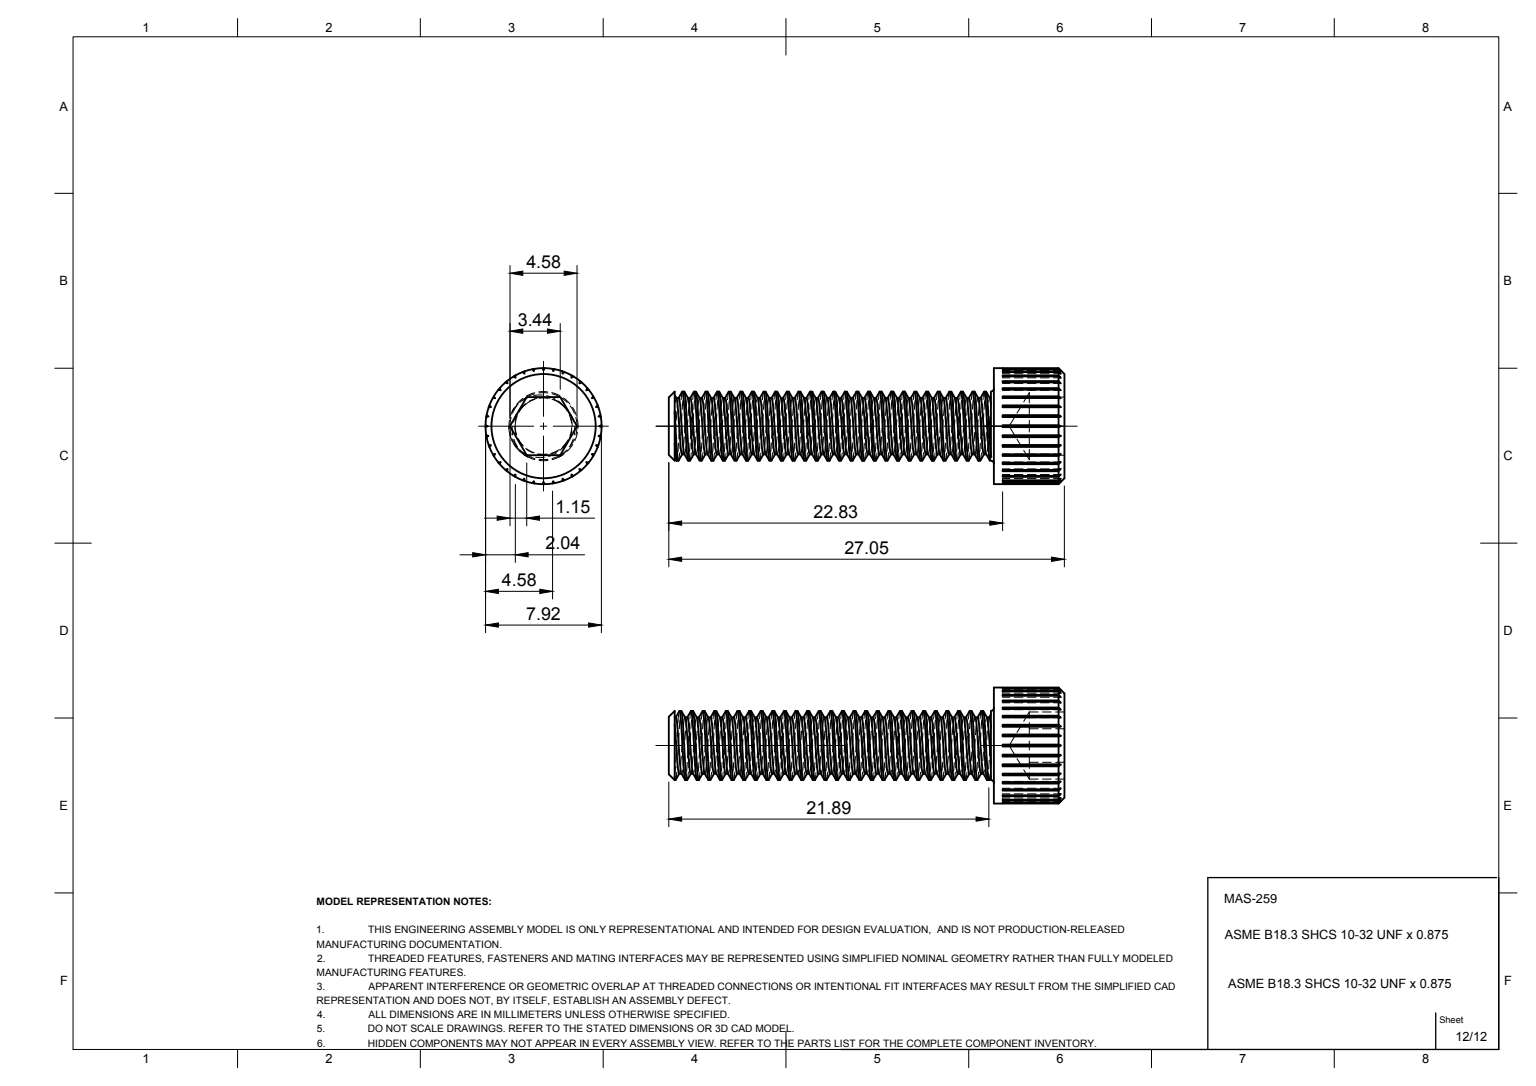
ISO-10303-21;
HEADER;
/* Generated by software containing ST-Developer
 * from STEP Tools, Inc. (www.steptools.com) 
 */

FILE_DESCRIPTION(
/* description */ (''),
/* implementation_level */ '2;1');

FILE_NAME(
/* name */ 'ASME B18.3 SHCS 10-32 UNF x 0.875.step',
/* time_stamp */ '2026-10-15T13:30:17-07:00',
/* author */ (''),
/* organization */ (''),
/* preprocessor_version */ 'ST-DEVELOPER v20.2',
/* originating_system */ 'Autodesk Translation Framework v15.15.0.0',
/* authorisation */ '');

FILE_SCHEMA (('AUTOMOTIVE_DESIGN { 1 0 10303 214 3 1 1 }'));
ENDSEC;

DATA;
#10=MECHANICAL_DESIGN_GEOMETRIC_PRESENTATION_REPRESENTATION('',(#1041),#71795);
#859=(
BOUNDED_CURVE()
B_SPLINE_CURVE(2,(#58913,#58914,#58915),.UNSPECIFIED.,.F.,.F.)
B_SPLINE_CURVE_WITH_KNOTS((3,3),(0.,0.0213887827154485),.UNSPECIFIED.)
CURVE()
GEOMETRIC_REPRESENTATION_ITEM()
RATIONAL_B_SPLINE_CURVE((1.,1.0006145366538,1.00078646015806))
REPRESENTATION_ITEM('')
);
#860=(
BOUNDED_CURVE()
B_SPLINE_CURVE(2,(#58918,#58919,#58920),.UNSPECIFIED.,.F.,.F.)
B_SPLINE_CURVE_WITH_KNOTS((3,3),(0.0380048027322743,0.0593935854477577),
 .UNSPECIFIED.)
CURVE()
GEOMETRIC_REPRESENTATION_ITEM()
RATIONAL_B_SPLINE_CURVE((1.00078646015726,1.00061453665318,1.))
REPRESENTATION_ITEM('')
);
#861=(
BOUNDED_CURVE()
B_SPLINE_CURVE(2,(#58929,#58930,#58931),.UNSPECIFIED.,.F.,.F.)
B_SPLINE_CURVE_WITH_KNOTS((3,3),(0.0380048027323083,0.0593935854477567),
 .UNSPECIFIED.)
CURVE()
GEOMETRIC_REPRESENTATION_ITEM()
RATIONAL_B_SPLINE_CURVE((1.00078646016055,1.00061453665575,1.))
REPRESENTATION_ITEM('')
);
#862=(
BOUNDED_CURVE()
B_SPLINE_CURVE(2,(#58935,#58936,#58937),.UNSPECIFIED.,.F.,.F.)
B_SPLINE_CURVE_WITH_KNOTS((3,3),(0.,0.0213887827154447),.UNSPECIFIED.)
CURVE()
GEOMETRIC_REPRESENTATION_ITEM()
RATIONAL_B_SPLINE_CURVE((1.,1.00061453665542,1.00078646016013))
REPRESENTATION_ITEM('')
);
#863=(
BOUNDED_CURVE()
B_SPLINE_CURVE(2,(#58939,#58940,#58941),.UNSPECIFIED.,.F.,.F.)
B_SPLINE_CURVE_WITH_KNOTS((3,3),(0.0380048027323192,0.0593935854477567),
 .UNSPECIFIED.)
CURVE()
GEOMETRIC_REPRESENTATION_ITEM()
RATIONAL_B_SPLINE_CURVE((1.0007864601593,1.00061453665477,1.))
REPRESENTATION_ITEM('')
);
#864=(
BOUNDED_CURVE()
B_SPLINE_CURVE(2,(#58945,#58946,#58947),.UNSPECIFIED.,.F.,.F.)
B_SPLINE_CURVE_WITH_KNOTS((3,3),(0.,0.0213887827154334),.UNSPECIFIED.)
CURVE()
GEOMETRIC_REPRESENTATION_ITEM()
RATIONAL_B_SPLINE_CURVE((1.,1.00061453665449,1.00078646015894))
REPRESENTATION_ITEM('')
);
#865=(
BOUNDED_CURVE()
B_SPLINE_CURVE(2,(#58949,#58950,#58951),.UNSPECIFIED.,.F.,.F.)
B_SPLINE_CURVE_WITH_KNOTS((3,3),(0.0380048027322763,0.0593935854477568),
 .UNSPECIFIED.)
CURVE()
GEOMETRIC_REPRESENTATION_ITEM()
RATIONAL_B_SPLINE_CURVE((1.00078646015818,1.00061453665389,1.))
REPRESENTATION_ITEM('')
);
#866=(
BOUNDED_CURVE()
B_SPLINE_CURVE(2,(#58955,#58956,#58957),.UNSPECIFIED.,.F.,.F.)
B_SPLINE_CURVE_WITH_KNOTS((3,3),(0.,0.0213887827154747),.UNSPECIFIED.)
CURVE()
GEOMETRIC_REPRESENTATION_ITEM()
RATIONAL_B_SPLINE_CURVE((1.,1.00061453665232,1.00078646015616))
REPRESENTATION_ITEM('')
);
#867=(
BOUNDED_CURVE()
B_SPLINE_CURVE(2,(#58959,#58960,#58961),.UNSPECIFIED.,.F.,.F.)
B_SPLINE_CURVE_WITH_KNOTS((3,3),(0.0380048027322871,0.0593935854477566),
 .UNSPECIFIED.)
CURVE()
GEOMETRIC_REPRESENTATION_ITEM()
RATIONAL_B_SPLINE_CURVE((1.00078646015913,1.00061453665464,1.))
REPRESENTATION_ITEM('')
);
#868=(
BOUNDED_CURVE()
B_SPLINE_CURVE(2,(#58965,#58966,#58967),.UNSPECIFIED.,.F.,.F.)
B_SPLINE_CURVE_WITH_KNOTS((3,3),(0.,0.0213887827154556),.UNSPECIFIED.)
CURVE()
GEOMETRIC_REPRESENTATION_ITEM()
RATIONAL_B_SPLINE_CURVE((1.,1.00061453665459,1.00078646015907))
REPRESENTATION_ITEM('')
);
#869=(
BOUNDED_CURVE()
B_SPLINE_CURVE(2,(#58969,#58970,#58971),.UNSPECIFIED.,.F.,.F.)
B_SPLINE_CURVE_WITH_KNOTS((3,3),(0.0380048027322698,0.0593935854477568),
 .UNSPECIFIED.)
CURVE()
GEOMETRIC_REPRESENTATION_ITEM()
RATIONAL_B_SPLINE_CURVE((1.000786460157,1.00061453665298,1.))
REPRESENTATION_ITEM('')
);
#870=(
BOUNDED_CURVE()
B_SPLINE_CURVE(2,(#58975,#58976,#58977),.UNSPECIFIED.,.F.,.F.)
B_SPLINE_CURVE_WITH_KNOTS((3,3),(0.,0.0213887827154226),.UNSPECIFIED.)
CURVE()
GEOMETRIC_REPRESENTATION_ITEM()
RATIONAL_B_SPLINE_CURVE((1.,1.00061453665557,1.00078646016033))
REPRESENTATION_ITEM('')
);
#871=(
BOUNDED_CURVE()
B_SPLINE_CURVE(2,(#58979,#58980,#58981),.UNSPECIFIED.,.F.,.F.)
B_SPLINE_CURVE_WITH_KNOTS((3,3),(0.0380048027322981,0.0593935854477561),
 .UNSPECIFIED.)
CURVE()
GEOMETRIC_REPRESENTATION_ITEM()
RATIONAL_B_SPLINE_CURVE((1.00078646015658,1.00061453665264,1.))
REPRESENTATION_ITEM('')
);
#872=(
BOUNDED_CURVE()
B_SPLINE_CURVE(2,(#58985,#58986,#58987),.UNSPECIFIED.,.F.,.F.)
B_SPLINE_CURVE_WITH_KNOTS((3,3),(0.,0.0213887827154885),.UNSPECIFIED.)
CURVE()
GEOMETRIC_REPRESENTATION_ITEM()
RATIONAL_B_SPLINE_CURVE((1.,1.00061453665414,1.00078646015849))
REPRESENTATION_ITEM('')
);
#873=(
BOUNDED_CURVE()
B_SPLINE_CURVE(2,(#58989,#58990,#58991),.UNSPECIFIED.,.F.,.F.)
B_SPLINE_CURVE_WITH_KNOTS((3,3),(0.0380048027323009,0.0593935854477566),
 .UNSPECIFIED.)
CURVE()
GEOMETRIC_REPRESENTATION_ITEM()
RATIONAL_B_SPLINE_CURVE((1.00078646015915,1.00061453665465,1.))
REPRESENTATION_ITEM('')
);
#874=(
BOUNDED_CURVE()
B_SPLINE_CURVE(2,(#58995,#58996,#58997),.UNSPECIFIED.,.F.,.F.)
B_SPLINE_CURVE_WITH_KNOTS((3,3),(0.,0.0213887827154357),.UNSPECIFIED.)
CURVE()
GEOMETRIC_REPRESENTATION_ITEM()
RATIONAL_B_SPLINE_CURVE((1.,1.00061453665688,1.000786460162))
REPRESENTATION_ITEM('')
);
#875=(
BOUNDED_CURVE()
B_SPLINE_CURVE(2,(#58999,#59000,#59001),.UNSPECIFIED.,.F.,.F.)
B_SPLINE_CURVE_WITH_KNOTS((3,3),(0.0380048027323154,0.059393585447756),
 .UNSPECIFIED.)
CURVE()
GEOMETRIC_REPRESENTATION_ITEM()
RATIONAL_B_SPLINE_CURVE((1.00078646016079,1.00061453665593,1.))
REPRESENTATION_ITEM('')
);
#876=(
BOUNDED_CURVE()
B_SPLINE_CURVE(2,(#59005,#59006,#59007),.UNSPECIFIED.,.F.,.F.)
B_SPLINE_CURVE_WITH_KNOTS((3,3),(0.,0.0213887827154912),.UNSPECIFIED.)
CURVE()
GEOMETRIC_REPRESENTATION_ITEM()
RATIONAL_B_SPLINE_CURVE((1.,1.00061453665086,1.0007864601543))
REPRESENTATION_ITEM('')
);
#877=(
BOUNDED_CURVE()
B_SPLINE_CURVE(2,(#59009,#59010,#59011),.UNSPECIFIED.,.F.,.F.)
B_SPLINE_CURVE_WITH_KNOTS((3,3),(0.0380048027322925,0.0593935854477561),
 .UNSPECIFIED.)
CURVE()
GEOMETRIC_REPRESENTATION_ITEM()
RATIONAL_B_SPLINE_CURVE((1.00078646015764,1.00061453665347,1.))
REPRESENTATION_ITEM('')
);
#878=(
BOUNDED_CURVE()
B_SPLINE_CURVE(2,(#59015,#59016,#59017),.UNSPECIFIED.,.F.,.F.)
B_SPLINE_CURVE_WITH_KNOTS((3,3),(0.,0.0213887827155107),.UNSPECIFIED.)
CURVE()
GEOMETRIC_REPRESENTATION_ITEM()
RATIONAL_B_SPLINE_CURVE((1.,1.00061453665119,1.00078646015471))
REPRESENTATION_ITEM('')
);
#879=(
BOUNDED_CURVE()
B_SPLINE_CURVE(2,(#59019,#59020,#59021),.UNSPECIFIED.,.F.,.F.)
B_SPLINE_CURVE_WITH_KNOTS((3,3),(0.038004802732295,0.0593935854477563),
 .UNSPECIFIED.)
CURVE()
GEOMETRIC_REPRESENTATION_ITEM()
RATIONAL_B_SPLINE_CURVE((1.00078646016111,1.00061453665618,1.))
REPRESENTATION_ITEM('')
);
#880=(
BOUNDED_CURVE()
B_SPLINE_CURVE(2,(#59025,#59026,#59027),.UNSPECIFIED.,.F.,.F.)
B_SPLINE_CURVE_WITH_KNOTS((3,3),(0.,0.0213887827154503),.UNSPECIFIED.)
CURVE()
GEOMETRIC_REPRESENTATION_ITEM()
RATIONAL_B_SPLINE_CURVE((1.,1.00061453665305,1.00078646015709))
REPRESENTATION_ITEM('')
);
#881=(
BOUNDED_CURVE()
B_SPLINE_CURVE(2,(#59029,#59030,#59031),.UNSPECIFIED.,.F.,.F.)
B_SPLINE_CURVE_WITH_KNOTS((3,3),(0.0380048027323246,0.059393585447756),
 .UNSPECIFIED.)
CURVE()
GEOMETRIC_REPRESENTATION_ITEM()
RATIONAL_B_SPLINE_CURVE((1.00078646015741,1.00061453665329,1.))
REPRESENTATION_ITEM('')
);
#882=(
BOUNDED_CURVE()
B_SPLINE_CURVE(2,(#59035,#59036,#59037),.UNSPECIFIED.,.F.,.F.)
B_SPLINE_CURVE_WITH_KNOTS((3,3),(0.,0.0213887827154455),.UNSPECIFIED.)
CURVE()
GEOMETRIC_REPRESENTATION_ITEM()
RATIONAL_B_SPLINE_CURVE((1.,1.00061453665435,1.00078646015877))
REPRESENTATION_ITEM('')
);
#883=(
BOUNDED_CURVE()
B_SPLINE_CURVE(2,(#59039,#59040,#59041),.UNSPECIFIED.,.F.,.F.)
B_SPLINE_CURVE_WITH_KNOTS((3,3),(0.0380048027322671,0.0593935854477559),
 .UNSPECIFIED.)
CURVE()
GEOMETRIC_REPRESENTATION_ITEM()
RATIONAL_B_SPLINE_CURVE((1.00078646015673,1.00061453665277,1.))
REPRESENTATION_ITEM('')
);
#884=(
BOUNDED_CURVE()
B_SPLINE_CURVE(2,(#59045,#59046,#59047),.UNSPECIFIED.,.F.,.F.)
B_SPLINE_CURVE_WITH_KNOTS((3,3),(0.,0.0213887827154328),.UNSPECIFIED.)
CURVE()
GEOMETRIC_REPRESENTATION_ITEM()
RATIONAL_B_SPLINE_CURVE((1.,1.0006145366569,1.00078646016203))
REPRESENTATION_ITEM('')
);
#885=(
BOUNDED_CURVE()
B_SPLINE_CURVE(2,(#59049,#59050,#59051),.UNSPECIFIED.,.F.,.F.)
B_SPLINE_CURVE_WITH_KNOTS((3,3),(0.0380048027322495,0.0593935854477564),
 .UNSPECIFIED.)
CURVE()
GEOMETRIC_REPRESENTATION_ITEM()
RATIONAL_B_SPLINE_CURVE((1.0007864601568,1.00061453665282,1.))
REPRESENTATION_ITEM('')
);
#886=(
BOUNDED_CURVE()
B_SPLINE_CURVE(2,(#59055,#59056,#59057),.UNSPECIFIED.,.F.,.F.)
B_SPLINE_CURVE_WITH_KNOTS((3,3),(0.,0.0213887827154736),.UNSPECIFIED.)
CURVE()
GEOMETRIC_REPRESENTATION_ITEM()
RATIONAL_B_SPLINE_CURVE((1.,1.0006145366516,1.00078646015525))
REPRESENTATION_ITEM('')
);
#887=(
BOUNDED_CURVE()
B_SPLINE_CURVE(2,(#59059,#59060,#59061),.UNSPECIFIED.,.F.,.F.)
B_SPLINE_CURVE_WITH_KNOTS((3,3),(0.0380048027322323,0.0593935854477557),
 .UNSPECIFIED.)
CURVE()
GEOMETRIC_REPRESENTATION_ITEM()
RATIONAL_B_SPLINE_CURVE((1.00078646015266,1.00061453664958,1.))
REPRESENTATION_ITEM('')
);
#888=(
BOUNDED_CURVE()
B_SPLINE_CURVE(2,(#59065,#59066,#59067),.UNSPECIFIED.,.F.,.F.)
B_SPLINE_CURVE_WITH_KNOTS((3,3),(0.,0.0213887827154861),.UNSPECIFIED.)
CURVE()
GEOMETRIC_REPRESENTATION_ITEM()
RATIONAL_B_SPLINE_CURVE((1.,1.00061453665221,1.00078646015603))
REPRESENTATION_ITEM('')
);
#889=(
BOUNDED_CURVE()
B_SPLINE_CURVE(2,(#59069,#59070,#59071),.UNSPECIFIED.,.F.,.F.)
B_SPLINE_CURVE_WITH_KNOTS((3,3),(0.038004802732259,0.0593935854477563),
 .UNSPECIFIED.)
CURVE()
GEOMETRIC_REPRESENTATION_ITEM()
RATIONAL_B_SPLINE_CURVE((1.00078646015598,1.00061453665218,1.))
REPRESENTATION_ITEM('')
);
#890=(
BOUNDED_CURVE()
B_SPLINE_CURVE(2,(#59075,#59076,#59077),.UNSPECIFIED.,.F.,.F.)
B_SPLINE_CURVE_WITH_KNOTS((3,3),(0.,0.0213887827154904),.UNSPECIFIED.)
CURVE()
GEOMETRIC_REPRESENTATION_ITEM()
RATIONAL_B_SPLINE_CURVE((1.,1.00061453665374,1.00078646015798))
REPRESENTATION_ITEM('')
);
#891=(
BOUNDED_CURVE()
B_SPLINE_CURVE(2,(#59079,#59080,#59081),.UNSPECIFIED.,.F.,.F.)
B_SPLINE_CURVE_WITH_KNOTS((3,3),(0.0380048027322369,0.0593935854477557),
 .UNSPECIFIED.)
CURVE()
GEOMETRIC_REPRESENTATION_ITEM()
RATIONAL_B_SPLINE_CURVE((1.00078646015409,1.0006145366507,1.))
REPRESENTATION_ITEM('')
);
#892=(
BOUNDED_CURVE()
B_SPLINE_CURVE(2,(#59085,#59086,#59087),.UNSPECIFIED.,.F.,.F.)
B_SPLINE_CURVE_WITH_KNOTS((3,3),(0.,0.0213887827154539),.UNSPECIFIED.)
CURVE()
GEOMETRIC_REPRESENTATION_ITEM()
RATIONAL_B_SPLINE_CURVE((1.,1.00061453665704,1.0007864601622))
REPRESENTATION_ITEM('')
);
#893=(
BOUNDED_CURVE()
B_SPLINE_CURVE(2,(#59089,#59090,#59091),.UNSPECIFIED.,.F.,.F.)
B_SPLINE_CURVE_WITH_KNOTS((3,3),(0.0380048027323148,0.0593935854477558),
 .UNSPECIFIED.)
CURVE()
GEOMETRIC_REPRESENTATION_ITEM()
RATIONAL_B_SPLINE_CURVE((1.00078646015925,1.00061453665473,1.))
REPRESENTATION_ITEM('')
);
#894=(
BOUNDED_CURVE()
B_SPLINE_CURVE(2,(#59095,#59096,#59097),.UNSPECIFIED.,.F.,.F.)
B_SPLINE_CURVE_WITH_KNOTS((3,3),(0.,0.0213887827154462),.UNSPECIFIED.)
CURVE()
GEOMETRIC_REPRESENTATION_ITEM()
RATIONAL_B_SPLINE_CURVE((1.,1.00061453665421,1.00078646015858))
REPRESENTATION_ITEM('')
);
#895=(
BOUNDED_CURVE()
B_SPLINE_CURVE(2,(#59099,#59100,#59101),.UNSPECIFIED.,.F.,.F.)
B_SPLINE_CURVE_WITH_KNOTS((3,3),(0.038004802732261,0.0593935854477558),
 .UNSPECIFIED.)
CURVE()
GEOMETRIC_REPRESENTATION_ITEM()
RATIONAL_B_SPLINE_CURVE((1.0007864601574,1.00061453665329,1.))
REPRESENTATION_ITEM('')
);
#896=(
BOUNDED_CURVE()
B_SPLINE_CURVE(2,(#59105,#59106,#59107),.UNSPECIFIED.,.F.,.F.)
B_SPLINE_CURVE_WITH_KNOTS((3,3),(0.,0.021388782715505),.UNSPECIFIED.)
CURVE()
GEOMETRIC_REPRESENTATION_ITEM()
RATIONAL_B_SPLINE_CURVE((1.,1.00061453665229,1.00078646015612))
REPRESENTATION_ITEM('')
);
#897=(
BOUNDED_CURVE()
B_SPLINE_CURVE(2,(#59109,#59110,#59111),.UNSPECIFIED.,.F.,.F.)
B_SPLINE_CURVE_WITH_KNOTS((3,3),(0.0380048027323058,0.0593935854477558),
 .UNSPECIFIED.)
CURVE()
GEOMETRIC_REPRESENTATION_ITEM()
RATIONAL_B_SPLINE_CURVE((1.00078646016102,1.00061453665611,1.))
REPRESENTATION_ITEM('')
);
#898=(
BOUNDED_CURVE()
B_SPLINE_CURVE(2,(#59116,#59117,#59118),.UNSPECIFIED.,.F.,.F.)
B_SPLINE_CURVE_WITH_KNOTS((3,3),(0.,0.0213887827154293),.UNSPECIFIED.)
CURVE()
GEOMETRIC_REPRESENTATION_ITEM()
RATIONAL_B_SPLINE_CURVE((1.,1.00061453665639,1.00078646016138))
REPRESENTATION_ITEM('')
);
#899=(
BOUNDED_CURVE()
B_SPLINE_CURVE(2,(#59120,#59121,#59122),.UNSPECIFIED.,.F.,.F.)
B_SPLINE_CURVE_WITH_KNOTS((3,3),(0.0380048027323149,0.0593935854477581),
 .UNSPECIFIED.)
CURVE()
GEOMETRIC_REPRESENTATION_ITEM()
RATIONAL_B_SPLINE_CURVE((1.00078646016138,1.0006145366564,1.))
REPRESENTATION_ITEM('')
);
#900=(
BOUNDED_CURVE()
B_SPLINE_CURVE(2,(#59126,#59127,#59128),.UNSPECIFIED.,.F.,.F.)
B_SPLINE_CURVE_WITH_KNOTS((3,3),(0.,0.0213887827154979),.UNSPECIFIED.)
CURVE()
GEOMETRIC_REPRESENTATION_ITEM()
RATIONAL_B_SPLINE_CURVE((1.,1.00061453665225,1.00078646015608))
REPRESENTATION_ITEM('')
);
#901=(
BOUNDED_CURVE()
B_SPLINE_CURVE(2,(#59130,#59131,#59132),.UNSPECIFIED.,.F.,.F.)
B_SPLINE_CURVE_WITH_KNOTS((3,3),(0.0380048027322422,0.059393585447758),
 .UNSPECIFIED.)
CURVE()
GEOMETRIC_REPRESENTATION_ITEM()
RATIONAL_B_SPLINE_CURVE((1.00078646015494,1.00061453665137,1.))
REPRESENTATION_ITEM('')
);
#902=(
BOUNDED_CURVE()
B_SPLINE_CURVE(2,(#59136,#59137,#59138),.UNSPECIFIED.,.F.,.F.)
B_SPLINE_CURVE_WITH_KNOTS((3,3),(0.,0.0213887827154959),.UNSPECIFIED.)
CURVE()
GEOMETRIC_REPRESENTATION_ITEM()
RATIONAL_B_SPLINE_CURVE((1.,1.00061453665238,1.00078646015624))
REPRESENTATION_ITEM('')
);
#903=(
BOUNDED_CURVE()
B_SPLINE_CURVE(2,(#59140,#59141,#59142),.UNSPECIFIED.,.F.,.F.)
B_SPLINE_CURVE_WITH_KNOTS((3,3),(0.0380048027323219,0.0593935854477577),
 .UNSPECIFIED.)
CURVE()
GEOMETRIC_REPRESENTATION_ITEM()
RATIONAL_B_SPLINE_CURVE((1.00078646016013,1.00061453665542,1.))
REPRESENTATION_ITEM('')
);
#904=(
BOUNDED_CURVE()
B_SPLINE_CURVE(2,(#59146,#59147,#59148),.UNSPECIFIED.,.F.,.F.)
B_SPLINE_CURVE_WITH_KNOTS((3,3),(0.,0.021388782715533),.UNSPECIFIED.)
CURVE()
GEOMETRIC_REPRESENTATION_ITEM()
RATIONAL_B_SPLINE_CURVE((1.,1.00061453664963,1.00078646015272))
REPRESENTATION_ITEM('')
);
#905=(
BOUNDED_CURVE()
B_SPLINE_CURVE(2,(#59150,#59151,#59152),.UNSPECIFIED.,.F.,.F.)
B_SPLINE_CURVE_WITH_KNOTS((3,3),(0.0380048027324089,0.0593935854477567),
 .UNSPECIFIED.)
CURVE()
GEOMETRIC_REPRESENTATION_ITEM()
RATIONAL_B_SPLINE_CURVE((1.00078646016585,1.00061453665989,1.))
REPRESENTATION_ITEM('')
);
#906=(
BOUNDED_CURVE()
B_SPLINE_CURVE(2,(#59156,#59157,#59158),.UNSPECIFIED.,.F.,.F.)
B_SPLINE_CURVE_WITH_KNOTS((3,3),(0.,0.0213887827154936),.UNSPECIFIED.)
CURVE()
GEOMETRIC_REPRESENTATION_ITEM()
RATIONAL_B_SPLINE_CURVE((1.,1.00061453665172,1.00078646015539))
REPRESENTATION_ITEM('')
);
#907=(
BOUNDED_CURVE()
B_SPLINE_CURVE(2,(#59160,#59161,#59162),.UNSPECIFIED.,.F.,.F.)
B_SPLINE_CURVE_WITH_KNOTS((3,3),(0.038004802732325,0.0593935854477579),
 .UNSPECIFIED.)
CURVE()
GEOMETRIC_REPRESENTATION_ITEM()
RATIONAL_B_SPLINE_CURVE((1.00078646016394,1.0006145366584,1.))
REPRESENTATION_ITEM('')
);
#908=(
BOUNDED_CURVE()
B_SPLINE_CURVE(2,(#59166,#59167,#59168),.UNSPECIFIED.,.F.,.F.)
B_SPLINE_CURVE_WITH_KNOTS((3,3),(0.,0.0213887827154531),.UNSPECIFIED.)
CURVE()
GEOMETRIC_REPRESENTATION_ITEM()
RATIONAL_B_SPLINE_CURVE((1.,1.00061453665483,1.00078646015938))
REPRESENTATION_ITEM('')
);
#909=(
BOUNDED_CURVE()
B_SPLINE_CURVE(2,(#59170,#59171,#59172),.UNSPECIFIED.,.F.,.F.)
B_SPLINE_CURVE_WITH_KNOTS((3,3),(0.03800480273219,0.0593935854477586),
 .UNSPECIFIED.)
CURVE()
GEOMETRIC_REPRESENTATION_ITEM()
RATIONAL_B_SPLINE_CURVE((1.00078646015297,1.00061453664982,1.))
REPRESENTATION_ITEM('')
);
#910=(
BOUNDED_CURVE()
B_SPLINE_CURVE(2,(#59176,#59177,#59178),.UNSPECIFIED.,.F.,.F.)
B_SPLINE_CURVE_WITH_KNOTS((3,3),(0.,0.0213887827154683),.UNSPECIFIED.)
CURVE()
GEOMETRIC_REPRESENTATION_ITEM()
RATIONAL_B_SPLINE_CURVE((1.,1.00061453665169,1.00078646015536))
REPRESENTATION_ITEM('')
);
#911=(
BOUNDED_CURVE()
B_SPLINE_CURVE(2,(#59180,#59181,#59182),.UNSPECIFIED.,.F.,.F.)
B_SPLINE_CURVE_WITH_KNOTS((3,3),(0.0380048027322755,0.0593935854477574),
 .UNSPECIFIED.)
CURVE()
GEOMETRIC_REPRESENTATION_ITEM()
RATIONAL_B_SPLINE_CURVE((1.00078646016181,1.00061453665673,1.))
REPRESENTATION_ITEM('')
);
#912=(
BOUNDED_CURVE()
B_SPLINE_CURVE(2,(#59186,#59187,#59188),.UNSPECIFIED.,.F.,.F.)
B_SPLINE_CURVE_WITH_KNOTS((3,3),(0.,0.0213887827154684),.UNSPECIFIED.)
CURVE()
GEOMETRIC_REPRESENTATION_ITEM()
RATIONAL_B_SPLINE_CURVE((1.,1.0006145366546,1.00078646015908))
REPRESENTATION_ITEM('')
);
#913=(
BOUNDED_CURVE()
B_SPLINE_CURVE(2,(#59190,#59191,#59192),.UNSPECIFIED.,.F.,.F.)
B_SPLINE_CURVE_WITH_KNOTS((3,3),(0.0380048027323105,0.0593935854477581),
 .UNSPECIFIED.)
CURVE()
GEOMETRIC_REPRESENTATION_ITEM()
RATIONAL_B_SPLINE_CURVE((1.00078646015979,1.00061453665516,1.))
REPRESENTATION_ITEM('')
);
#914=(
BOUNDED_CURVE()
B_SPLINE_CURVE(2,(#59196,#59197,#59198),.UNSPECIFIED.,.F.,.F.)
B_SPLINE_CURVE_WITH_KNOTS((3,3),(0.,0.0213887827154438),.UNSPECIFIED.)
CURVE()
GEOMETRIC_REPRESENTATION_ITEM()
RATIONAL_B_SPLINE_CURVE((1.,1.00061453665793,1.00078646016334))
REPRESENTATION_ITEM('')
);
#915=(
BOUNDED_CURVE()
B_SPLINE_CURVE(2,(#59200,#59201,#59202),.UNSPECIFIED.,.F.,.F.)
B_SPLINE_CURVE_WITH_KNOTS((3,3),(0.0380048027322779,0.0593935854477573),
 .UNSPECIFIED.)
CURVE()
GEOMETRIC_REPRESENTATION_ITEM()
RATIONAL_B_SPLINE_CURVE((1.00078646015484,1.00061453665129,1.))
REPRESENTATION_ITEM('')
);
#916=(
BOUNDED_CURVE()
B_SPLINE_CURVE(2,(#59206,#59207,#59208),.UNSPECIFIED.,.F.,.F.)
B_SPLINE_CURVE_WITH_KNOTS((3,3),(0.,0.0213887827154012),.UNSPECIFIED.)
CURVE()
GEOMETRIC_REPRESENTATION_ITEM()
RATIONAL_B_SPLINE_CURVE((1.,1.00061453665908,1.00078646016482))
REPRESENTATION_ITEM('')
);
#917=(
BOUNDED_CURVE()
B_SPLINE_CURVE(2,(#59210,#59211,#59212),.UNSPECIFIED.,.F.,.F.)
B_SPLINE_CURVE_WITH_KNOTS((3,3),(0.0380048027322933,0.0593935854477573),
 .UNSPECIFIED.)
CURVE()
GEOMETRIC_REPRESENTATION_ITEM()
RATIONAL_B_SPLINE_CURVE((1.00078646015827,1.00061453665397,1.))
REPRESENTATION_ITEM('')
);
#918=(
BOUNDED_CURVE()
B_SPLINE_CURVE(2,(#59216,#59217,#59218),.UNSPECIFIED.,.F.,.F.)
B_SPLINE_CURVE_WITH_KNOTS((3,3),(0.,0.0213887827154559),.UNSPECIFIED.)
CURVE()
GEOMETRIC_REPRESENTATION_ITEM()
RATIONAL_B_SPLINE_CURVE((1.,1.00061453665602,1.0007864601609))
REPRESENTATION_ITEM('')
);
#919=(
BOUNDED_CURVE()
B_SPLINE_CURVE(2,(#59220,#59221,#59222),.UNSPECIFIED.,.F.,.F.)
B_SPLINE_CURVE_WITH_KNOTS((3,3),(0.038004802732396,0.0593935854477571),
 .UNSPECIFIED.)
CURVE()
GEOMETRIC_REPRESENTATION_ITEM()
RATIONAL_B_SPLINE_CURVE((1.00078646016815,1.00061453666168,1.))
REPRESENTATION_ITEM('')
);
#920=(
BOUNDED_CURVE()
B_SPLINE_CURVE(2,(#59226,#59227,#59228),.UNSPECIFIED.,.F.,.F.)
B_SPLINE_CURVE_WITH_KNOTS((3,3),(0.,0.0213887827154657),.UNSPECIFIED.)
CURVE()
GEOMETRIC_REPRESENTATION_ITEM()
RATIONAL_B_SPLINE_CURVE((1.,1.00061453665296,1.00078646015698))
REPRESENTATION_ITEM('')
);
#921=(
BOUNDED_CURVE()
B_SPLINE_CURVE(2,(#59230,#59231,#59232),.UNSPECIFIED.,.F.,.F.)
B_SPLINE_CURVE_WITH_KNOTS((3,3),(0.0380048027322985,0.059393585447757),
 .UNSPECIFIED.)
CURVE()
GEOMETRIC_REPRESENTATION_ITEM()
RATIONAL_B_SPLINE_CURVE((1.00078646016081,1.00061453665595,1.))
REPRESENTATION_ITEM('')
);
#922=(
BOUNDED_CURVE()
B_SPLINE_CURVE(2,(#59236,#59237,#59238),.UNSPECIFIED.,.F.,.F.)
B_SPLINE_CURVE_WITH_KNOTS((3,3),(0.,0.0213887827154679),.UNSPECIFIED.)
CURVE()
GEOMETRIC_REPRESENTATION_ITEM()
RATIONAL_B_SPLINE_CURVE((1.,1.00061453665517,1.00078646015981))
REPRESENTATION_ITEM('')
);
#923=(
BOUNDED_CURVE()
B_SPLINE_CURVE(2,(#59240,#59241,#59242),.UNSPECIFIED.,.F.,.F.)
B_SPLINE_CURVE_WITH_KNOTS((3,3),(0.0380048027322456,0.0593935854477571),
 .UNSPECIFIED.)
CURVE()
GEOMETRIC_REPRESENTATION_ITEM()
RATIONAL_B_SPLINE_CURVE((1.00078646015223,1.00061453664925,1.))
REPRESENTATION_ITEM('')
);
#924=(
BOUNDED_CURVE()
B_SPLINE_CURVE(2,(#59246,#59247,#59248),.UNSPECIFIED.,.F.,.F.)
B_SPLINE_CURVE_WITH_KNOTS((3,3),(0.,0.0213887827154763),.UNSPECIFIED.)
CURVE()
GEOMETRIC_REPRESENTATION_ITEM()
RATIONAL_B_SPLINE_CURVE((1.,1.00061453665236,1.00078646015621))
REPRESENTATION_ITEM('')
);
#925=(
BOUNDED_CURVE()
B_SPLINE_CURVE(2,(#59250,#59251,#59252),.UNSPECIFIED.,.F.,.F.)
B_SPLINE_CURVE_WITH_KNOTS((3,3),(0.0380048027323043,0.0593935854477561),
 .UNSPECIFIED.)
CURVE()
GEOMETRIC_REPRESENTATION_ITEM()
RATIONAL_B_SPLINE_CURVE((1.00078646015985,1.0006145366552,1.))
REPRESENTATION_ITEM('')
);
#926=(
BOUNDED_CURVE()
B_SPLINE_CURVE(2,(#59256,#59257,#59258),.UNSPECIFIED.,.F.,.F.)
B_SPLINE_CURVE_WITH_KNOTS((3,3),(0.,0.0213887827154303),.UNSPECIFIED.)
CURVE()
GEOMETRIC_REPRESENTATION_ITEM()
RATIONAL_B_SPLINE_CURVE((1.,1.00061453665563,1.0007864601604))
REPRESENTATION_ITEM('')
);
#927=(
BOUNDED_CURVE()
B_SPLINE_CURVE(2,(#59260,#59261,#59262),.UNSPECIFIED.,.F.,.F.)
B_SPLINE_CURVE_WITH_KNOTS((3,3),(0.0380048027323154,0.0593935854477565),
 .UNSPECIFIED.)
CURVE()
GEOMETRIC_REPRESENTATION_ITEM()
RATIONAL_B_SPLINE_CURVE((1.00078646015761,1.00061453665345,1.))
REPRESENTATION_ITEM('')
);
#928=(
BOUNDED_CURVE()
B_SPLINE_CURVE(2,(#59266,#59267,#59268),.UNSPECIFIED.,.F.,.F.)
B_SPLINE_CURVE_WITH_KNOTS((3,3),(0.,0.0213887827154477),.UNSPECIFIED.)
CURVE()
GEOMETRIC_REPRESENTATION_ITEM()
RATIONAL_B_SPLINE_CURVE((1.,1.00061453665389,1.00078646015818))
REPRESENTATION_ITEM('')
);
#929=(
BOUNDED_CURVE()
B_SPLINE_CURVE(2,(#59270,#59271,#59272),.UNSPECIFIED.,.F.,.F.)
B_SPLINE_CURVE_WITH_KNOTS((3,3),(0.0380048027322823,0.0593935854477568),
 .UNSPECIFIED.)
CURVE()
GEOMETRIC_REPRESENTATION_ITEM()
RATIONAL_B_SPLINE_CURVE((1.00078646015752,1.00061453665338,1.))
REPRESENTATION_ITEM('')
);
#930=(
BOUNDED_CURVE()
B_SPLINE_CURVE(2,(#59275,#59276,#59277),.UNSPECIFIED.,.F.,.F.)
B_SPLINE_CURVE_WITH_KNOTS((3,3),(0.,0.0213887827154623),.UNSPECIFIED.)
CURVE()
GEOMETRIC_REPRESENTATION_ITEM()
RATIONAL_B_SPLINE_CURVE((1.,1.00061453665359,1.00078646015779))
REPRESENTATION_ITEM('')
);
#1004=TOROIDAL_SURFACE('',#14398,2.56347,0.2);
#1008=B_SPLINE_SURFACE_WITH_KNOTS('',3,3,((#57303,#57304,#57305,#57306,
#57307,#57308,#57309,#57310,#57311,#57312,#57313,#57314,#57315,#57316,#57317,
#57318,#57319,#57320,#57321,#57322,#57323,#57324,#57325,#57326,#57327,#57328,
#57329,#57330,#57331,#57332,#57333,#57334,#57335,#57336,#57337,#57338,#57339,
#57340,#57341,#57342,#57343,#57344,#57345,#57346,#57347,#57348,#57349,#57350,
#57351,#57352,#57353,#57354,#57355,#57356,#57357,#57358,#57359,#57360,#57361,
#57362,#57363,#57364,#57365,#57366,#57367,#57368,#57369,#57370,#57371,#57372,
#57373,#57374,#57375,#57376,#57377,#57378,#57379,#57380,#57381,#57382,#57383,
#57384,#57385,#57386,#57387,#57388,#57389,#57390,#57391,#57392,#57393,#57394,
#57395,#57396,#57397,#57398,#57399,#57400,#57401,#57402,#57403,#57404,#57405,
#57406,#57407,#57408,#57409,#57410,#57411,#57412,#57413,#57414,#57415,#57416,
#57417,#57418,#57419,#57420,#57421,#57422,#57423,#57424,#57425,#57426,#57427,
#57428,#57429,#57430,#57431,#57432,#57433,#57434,#57435,#57436,#57437,#57438,
#57439,#57440,#57441,#57442,#57443,#57444,#57445,#57446,#57447,#57448,#57449,
#57450,#57451,#57452,#57453,#57454,#57455,#57456,#57457,#57458,#57459,#57460,
#57461,#57462,#57463,#57464,#57465,#57466,#57467,#57468,#57469,#57470,#57471,
#57472,#57473,#57474,#57475,#57476,#57477,#57478,#57479),(#57480,#57481,
#57482,#57483,#57484,#57485,#57486,#57487,#57488,#57489,#57490,#57491,#57492,
#57493,#57494,#57495,#57496,#57497,#57498,#57499,#57500,#57501,#57502,#57503,
#57504,#57505,#57506,#57507,#57508,#57509,#57510,#57511,#57512,#57513,#57514,
#57515,#57516,#57517,#57518,#57519,#57520,#57521,#57522,#57523,#57524,#57525,
#57526,#57527,#57528,#57529,#57530,#57531,#57532,#57533,#57534,#57535,#57536,
#57537,#57538,#57539,#57540,#57541,#57542,#57543,#57544,#57545,#57546,#57547,
#57548,#57549,#57550,#57551,#57552,#57553,#57554,#57555,#57556,#57557,#57558,
#57559,#57560,#57561,#57562,#57563,#57564,#57565,#57566,#57567,#57568,#57569,
#57570,#57571,#57572,#57573,#57574,#57575,#57576,#57577,#57578,#57579,#57580,
#57581,#57582,#57583,#57584,#57585,#57586,#57587,#57588,#57589,#57590,#57591,
#57592,#57593,#57594,#57595,#57596,#57597,#57598,#57599,#57600,#57601,#57602,
#57603,#57604,#57605,#57606,#57607,#57608,#57609,#57610,#57611,#57612,#57613,
#57614,#57615,#57616,#57617,#57618,#57619,#57620,#57621,#57622,#57623,#57624,
#57625,#57626,#57627,#57628,#57629,#57630,#57631,#57632,#57633,#57634,#57635,
#57636,#57637,#57638,#57639,#57640,#57641,#57642,#57643,#57644,#57645,#57646,
#57647,#57648,#57649,#57650,#57651,#57652,#57653,#57654,#57655,#57656),
(#57657,#57658,#57659,#57660,#57661,#57662,#57663,#57664,#57665,#57666,
#57667,#57668,#57669,#57670,#57671,#57672,#57673,#57674,#57675,#57676,#57677,
#57678,#57679,#57680,#57681,#57682,#57683,#57684,#57685,#57686,#57687,#57688,
#57689,#57690,#57691,#57692,#57693,#57694,#57695,#57696,#57697,#57698,#57699,
#57700,#57701,#57702,#57703,#57704,#57705,#57706,#57707,#57708,#57709,#57710,
#57711,#57712,#57713,#57714,#57715,#57716,#57717,#57718,#57719,#57720,#57721,
#57722,#57723,#57724,#57725,#57726,#57727,#57728,#57729,#57730,#57731,#57732,
#57733,#57734,#57735,#57736,#57737,#57738,#57739,#57740,#57741,#57742,#57743,
#57744,#57745,#57746,#57747,#57748,#57749,#57750,#57751,#57752,#57753,#57754,
#57755,#57756,#57757,#57758,#57759,#57760,#57761,#57762,#57763,#57764,#57765,
#57766,#57767,#57768,#57769,#57770,#57771,#57772,#57773,#57774,#57775,#57776,
#57777,#57778,#57779,#57780,#57781,#57782,#57783,#57784,#57785,#57786,#57787,
#57788,#57789,#57790,#57791,#57792,#57793,#57794,#57795,#57796,#57797,#57798,
#57799,#57800,#57801,#57802,#57803,#57804,#57805,#57806,#57807,#57808,#57809,
#57810,#57811,#57812,#57813,#57814,#57815,#57816,#57817,#57818,#57819,#57820,
#57821,#57822,#57823,#57824,#57825,#57826,#57827,#57828,#57829,#57830,#57831,
#57832,#57833),(#57834,#57835,#57836,#57837,#57838,#57839,#57840,#57841,
#57842,#57843,#57844,#57845,#57846,#57847,#57848,#57849,#57850,#57851,#57852,
#57853,#57854,#57855,#57856,#57857,#57858,#57859,#57860,#57861,#57862,#57863,
#57864,#57865,#57866,#57867,#57868,#57869,#57870,#57871,#57872,#57873,#57874,
#57875,#57876,#57877,#57878,#57879,#57880,#57881,#57882,#57883,#57884,#57885,
#57886,#57887,#57888,#57889,#57890,#57891,#57892,#57893,#57894,#57895,#57896,
#57897,#57898,#57899,#57900,#57901,#57902,#57903,#57904,#57905,#57906,#57907,
#57908,#57909,#57910,#57911,#57912,#57913,#57914,#57915,#57916,#57917,#57918,
#57919,#57920,#57921,#57922,#57923,#57924,#57925,#57926,#57927,#57928,#57929,
#57930,#57931,#57932,#57933,#57934,#57935,#57936,#57937,#57938,#57939,#57940,
#57941,#57942,#57943,#57944,#57945,#57946,#57947,#57948,#57949,#57950,#57951,
#57952,#57953,#57954,#57955,#57956,#57957,#57958,#57959,#57960,#57961,#57962,
#57963,#57964,#57965,#57966,#57967,#57968,#57969,#57970,#57971,#57972,#57973,
#57974,#57975,#57976,#57977,#57978,#57979,#57980,#57981,#57982,#57983,#57984,
#57985,#57986,#57987,#57988,#57989,#57990,#57991,#57992,#57993,#57994,#57995,
#57996,#57997,#57998,#57999,#58000,#58001,#58002,#58003,#58004,#58005,#58006,
#58007,#58008,#58009,#58010)),.UNSPECIFIED.,.F.,.F.,.F.,(4,4),(4,1,1,1,
1,1,1,1,1,1,1,1,1,1,1,1,1,1,1,1,1,1,1,1,1,1,1,1,1,1,1,1,1,1,1,1,1,1,1,1,
1,1,1,1,1,1,1,1,1,1,1,1,1,1,1,1,1,1,1,1,1,1,1,1,1,1,1,1,1,1,1,1,1,1,1,1,
1,1,1,1,1,1,1,1,1,1,1,1,1,1,1,1,1,1,1,1,1,1,1,1,1,1,1,1,1,1,1,1,1,1,1,1,
1,1,1,1,1,1,1,1,1,1,1,1,1,1,1,1,1,1,1,1,1,1,1,1,1,1,1,1,1,1,1,1,1,1,1,1,
1,1,1,1,1,1,1,1,1,1,1,1,1,1,1,1,1,1,1,1,1,1,1,1,1,1,4),(-0.000395455933507198,
0.0505042896976108),(8.33359626324614,9.32879578175085,10.3239953002556,
11.3191948187603,12.314394337265,13.3095938557697,14.3047933742744,15.2999928927791,
16.2951924112838,17.2903919297885,18.2855914482932,19.2807909667979,20.2759904853026,
21.2711900038073,22.2663895223121,23.2615890408168,24.2567885593215,25.2519880778262,
26.2471875963309,27.2423871148356,28.2375866333403,29.232786151845,30.2279856703497,
31.2231851888544,32.2183847073591,33.2135842258639,34.2087837443686,35.2039832628733,
36.199182781378,37.1943822998827,38.1895818183874,39.1847813368921,40.1799808553968,
41.1751803739015,42.1703798924062,43.1655794109109,44.1607789294156,45.1559784479203,
46.1511779664251,47.1463774849298,48.1415770034345,49.1367765219392,50.1319760404439,
51.1271755589486,52.1223750774533,53.117574595958,54.1127741144627,55.1079736329674,
56.1031731514721,57.0983726699769,58.0935721884816,59.0887717069863,60.083971225491,
61.0791707439957,62.0743702625004,63.0695697810051,64.0647692995098,65.0599688180145,
66.0551683365192,67.0503678550239,68.0455673735286,69.0407668920334,70.0359664105381,
71.0311659290428,72.0263654475475,73.0215649660522,74.0167644845569,75.0119640030616,
76.0071635215663,77.002363040071,77.9975625585757,78.9927620770804,79.9879615955851,
80.9831611140899,81.9783606325946,82.9735601510993,83.968759669604,84.9639591881087,
85.9591587066134,86.9543582251181,87.9495577436228,88.9447572621275,89.9399567806322,
90.9351562991369,91.9303558176416,92.9255553361464,93.9207548546511,94.9159543731558,
95.9111538916605,96.9063534101652,97.9015529286699,98.8967524471746,99.8919519656793,
100.887151484184,101.882351002689,102.877550521193,103.872750039698,104.867949558203,
105.863149076708,106.858348595212,107.853548113717,108.848747632222,109.843947150726,
110.839146669231,111.834346187736,112.829545706241,113.824745224745,114.81994474325,
115.815144261755,116.810343780259,117.805543298764,118.800742817269,119.795942335773,
120.791141854278,121.786341372783,122.781540891288,123.776740409792,124.771939928297,
125.767139446802,126.762338965306,127.757538483811,128.752738002316,129.747937520821,
130.743137039325,131.73833655783,132.733536076335,133.728735594839,134.723935113344,
135.719134631849,136.714334150354,137.709533668858,138.704733187363,139.699932705868,
140.695132224372,141.690331742877,142.685531261382,143.680730779886,144.675930298391,
145.671129816896,146.666329335401,147.661528853905,148.65672837241,149.651927890915,
150.647127409419,151.642326927924,152.637526446429,153.632725964934,154.627925483438,
155.623125001943,156.618324520448,157.613524038952,158.608723557457,159.603923075962,
160.599122594467,161.594322112971,162.589521631476,163.584721149981,164.579920668485,
165.57512018699,166.570319705495,167.565519224,168.560718742504,169.555918261009,
170.551117779514,171.546317298018,172.541516816523,173.536716335028,174.531915853532,
175.527115372037,176.522314890542,177.517514409047,178.512713927551,179.507913446056,
180.503112964561,181.498707938999),.UNSPECIFIED.);
#1009=B_SPLINE_SURFACE_WITH_KNOTS('',3,3,((#58181,#58182,#58183,#58184,
#58185,#58186,#58187,#58188,#58189,#58190,#58191,#58192,#58193,#58194,#58195,
#58196,#58197,#58198,#58199,#58200,#58201,#58202,#58203,#58204,#58205,#58206,
#58207,#58208,#58209,#58210,#58211,#58212,#58213,#58214,#58215,#58216,#58217,
#58218,#58219,#58220,#58221,#58222,#58223,#58224,#58225,#58226,#58227,#58228,
#58229,#58230,#58231,#58232,#58233,#58234,#58235,#58236,#58237,#58238,#58239,
#58240,#58241,#58242,#58243,#58244,#58245,#58246,#58247,#58248,#58249,#58250,
#58251,#58252,#58253,#58254,#58255,#58256,#58257,#58258,#58259,#58260,#58261,
#58262,#58263,#58264,#58265,#58266,#58267,#58268,#58269,#58270,#58271,#58272,
#58273,#58274,#58275,#58276,#58277,#58278,#58279,#58280,#58281,#58282,#58283,
#58284,#58285,#58286,#58287,#58288,#58289,#58290,#58291,#58292,#58293,#58294,
#58295,#58296,#58297,#58298,#58299,#58300,#58301,#58302,#58303,#58304,#58305,
#58306,#58307,#58308,#58309,#58310,#58311,#58312,#58313,#58314,#58315,#58316,
#58317,#58318,#58319,#58320,#58321,#58322,#58323,#58324,#58325,#58326,#58327,
#58328,#58329,#58330,#58331,#58332,#58333,#58334,#58335,#58336,#58337,#58338,
#58339,#58340,#58341,#58342,#58343,#58344,#58345,#58346,#58347,#58348,#58349,
#58350,#58351,#58352,#58353,#58354,#58355,#58356,#58357),(#58358,#58359,
#58360,#58361,#58362,#58363,#58364,#58365,#58366,#58367,#58368,#58369,#58370,
#58371,#58372,#58373,#58374,#58375,#58376,#58377,#58378,#58379,#58380,#58381,
#58382,#58383,#58384,#58385,#58386,#58387,#58388,#58389,#58390,#58391,#58392,
#58393,#58394,#58395,#58396,#58397,#58398,#58399,#58400,#58401,#58402,#58403,
#58404,#58405,#58406,#58407,#58408,#58409,#58410,#58411,#58412,#58413,#58414,
#58415,#58416,#58417,#58418,#58419,#58420,#58421,#58422,#58423,#58424,#58425,
#58426,#58427,#58428,#58429,#58430,#58431,#58432,#58433,#58434,#58435,#58436,
#58437,#58438,#58439,#58440,#58441,#58442,#58443,#58444,#58445,#58446,#58447,
#58448,#58449,#58450,#58451,#58452,#58453,#58454,#58455,#58456,#58457,#58458,
#58459,#58460,#58461,#58462,#58463,#58464,#58465,#58466,#58467,#58468,#58469,
#58470,#58471,#58472,#58473,#58474,#58475,#58476,#58477,#58478,#58479,#58480,
#58481,#58482,#58483,#58484,#58485,#58486,#58487,#58488,#58489,#58490,#58491,
#58492,#58493,#58494,#58495,#58496,#58497,#58498,#58499,#58500,#58501,#58502,
#58503,#58504,#58505,#58506,#58507,#58508,#58509,#58510,#58511,#58512,#58513,
#58514,#58515,#58516,#58517,#58518,#58519,#58520,#58521,#58522,#58523,#58524,
#58525,#58526,#58527,#58528,#58529,#58530,#58531,#58532,#58533,#58534),
(#58535,#58536,#58537,#58538,#58539,#58540,#58541,#58542,#58543,#58544,
#58545,#58546,#58547,#58548,#58549,#58550,#58551,#58552,#58553,#58554,#58555,
#58556,#58557,#58558,#58559,#58560,#58561,#58562,#58563,#58564,#58565,#58566,
#58567,#58568,#58569,#58570,#58571,#58572,#58573,#58574,#58575,#58576,#58577,
#58578,#58579,#58580,#58581,#58582,#58583,#58584,#58585,#58586,#58587,#58588,
#58589,#58590,#58591,#58592,#58593,#58594,#58595,#58596,#58597,#58598,#58599,
#58600,#58601,#58602,#58603,#58604,#58605,#58606,#58607,#58608,#58609,#58610,
#58611,#58612,#58613,#58614,#58615,#58616,#58617,#58618,#58619,#58620,#58621,
#58622,#58623,#58624,#58625,#58626,#58627,#58628,#58629,#58630,#58631,#58632,
#58633,#58634,#58635,#58636,#58637,#58638,#58639,#58640,#58641,#58642,#58643,
#58644,#58645,#58646,#58647,#58648,#58649,#58650,#58651,#58652,#58653,#58654,
#58655,#58656,#58657,#58658,#58659,#58660,#58661,#58662,#58663,#58664,#58665,
#58666,#58667,#58668,#58669,#58670,#58671,#58672,#58673,#58674,#58675,#58676,
#58677,#58678,#58679,#58680,#58681,#58682,#58683,#58684,#58685,#58686,#58687,
#58688,#58689,#58690,#58691,#58692,#58693,#58694,#58695,#58696,#58697,#58698,
#58699,#58700,#58701,#58702,#58703,#58704,#58705,#58706,#58707,#58708,#58709,
#58710,#58711),(#58712,#58713,#58714,#58715,#58716,#58717,#58718,#58719,
#58720,#58721,#58722,#58723,#58724,#58725,#58726,#58727,#58728,#58729,#58730,
#58731,#58732,#58733,#58734,#58735,#58736,#58737,#58738,#58739,#58740,#58741,
#58742,#58743,#58744,#58745,#58746,#58747,#58748,#58749,#58750,#58751,#58752,
#58753,#58754,#58755,#58756,#58757,#58758,#58759,#58760,#58761,#58762,#58763,
#58764,#58765,#58766,#58767,#58768,#58769,#58770,#58771,#58772,#58773,#58774,
#58775,#58776,#58777,#58778,#58779,#58780,#58781,#58782,#58783,#58784,#58785,
#58786,#58787,#58788,#58789,#58790,#58791,#58792,#58793,#58794,#58795,#58796,
#58797,#58798,#58799,#58800,#58801,#58802,#58803,#58804,#58805,#58806,#58807,
#58808,#58809,#58810,#58811,#58812,#58813,#58814,#58815,#58816,#58817,#58818,
#58819,#58820,#58821,#58822,#58823,#58824,#58825,#58826,#58827,#58828,#58829,
#58830,#58831,#58832,#58833,#58834,#58835,#58836,#58837,#58838,#58839,#58840,
#58841,#58842,#58843,#58844,#58845,#58846,#58847,#58848,#58849,#58850,#58851,
#58852,#58853,#58854,#58855,#58856,#58857,#58858,#58859,#58860,#58861,#58862,
#58863,#58864,#58865,#58866,#58867,#58868,#58869,#58870,#58871,#58872,#58873,
#58874,#58875,#58876,#58877,#58878,#58879,#58880,#58881,#58882,#58883,#58884,
#58885,#58886,#58887,#58888)),.UNSPECIFIED.,.F.,.F.,.F.,(4,4),(4,1,1,1,
1,1,1,1,1,1,1,1,1,1,1,1,1,1,1,1,1,1,1,1,1,1,1,1,1,1,1,1,1,1,1,1,1,1,1,1,
1,1,1,1,1,1,1,1,1,1,1,1,1,1,1,1,1,1,1,1,1,1,1,1,1,1,1,1,1,1,1,1,1,1,1,1,
1,1,1,1,1,1,1,1,1,1,1,1,1,1,1,1,1,1,1,1,1,1,1,1,1,1,1,1,1,1,1,1,1,1,1,1,
1,1,1,1,1,1,1,1,1,1,1,1,1,1,1,1,1,1,1,1,1,1,1,1,1,1,1,1,1,1,1,1,1,1,1,1,
1,1,1,1,1,1,1,1,1,1,1,1,1,1,1,1,1,1,1,1,1,1,1,1,1,1,4),(-0.000351020118781134,
0.0505486889477217),(11.6721348619008,12.6677298061693,13.662929324674,
14.6581288431788,15.6533283616835,16.6485278801882,17.6437273986929,18.6389269171976,
19.6341264357023,20.629325954207,21.6245254727117,22.6197249912164,23.6149245097211,
24.6101240282258,25.6053235467305,26.6005230652353,27.59572258374,28.5909221022447,
29.5861216207494,30.5813211392541,31.5765206577588,32.5717201762635,33.5669196947682,
34.5621192132729,35.5573187317776,36.5525182502823,37.5477177687871,38.5429172872918,
39.5381168057965,40.5333163243012,41.5285158428059,42.5237153613106,43.5189148798153,
44.51411439832,45.5093139168247,46.5045134353294,47.4997129538341,48.4949124723388,
49.4901119908436,50.4853115093483,51.480511027853,52.4757105463577,53.4709100648624,
54.4661095833671,55.4613091018718,56.4565086203765,57.4517081388812,58.4469076573859,
59.4421071758906,60.4373066943953,61.4325062129001,62.4277057314048,63.4229052499095,
64.4181047684142,65.4133042869189,66.4085038054236,67.4037033239283,68.398902842433,
69.3941023609377,70.3893018794424,71.3845013979471,72.3797009164519,73.3749004349566,
74.3700999534613,75.365299471966,76.3604989904707,77.3556985089754,78.3508980274801,
79.3460975459848,80.3412970644895,81.3364965829942,82.3316961014989,83.3268956200036,
84.3220951385084,85.3172946570131,86.3124941755178,87.3076936940225,88.3028932125272,
89.2980927310319,90.2932922495366,91.2884917680413,92.283691286546,93.2788908050507,
94.2740903235554,95.2692898420601,96.2644893605649,97.2596888790696,98.2548883975743,
99.250087916079,100.245287434584,101.240486953088,102.235686471593,103.230885990098,
104.226085508603,105.221285027107,106.216484545612,107.211684064117,108.206883582621,
109.202083101126,110.197282619631,111.192482138135,112.18768165664,113.182881175145,
114.17808069365,115.173280212154,116.168479730659,117.163679249164,118.158878767668,
119.154078286173,120.149277804678,121.144477323183,122.139676841687,123.134876360192,
124.130075878697,125.125275397201,126.120474915706,127.115674434211,128.110873952716,
129.10607347122,130.101272989725,131.09647250823,132.091672026734,133.086871545239,
134.082071063744,135.077270582249,136.072470100753,137.067669619258,138.062869137763,
139.058068656267,140.053268174772,141.048467693277,142.043667211781,143.038866730286,
144.034066248791,145.029265767296,146.0244652858,147.019664804305,148.01486432281,
149.010063841314,150.005263359819,151.000462878324,151.995662396829,152.990861915333,
153.986061433838,154.981260952343,155.976460470847,156.971659989352,157.966859507857,
158.962059026361,159.957258544866,160.952458063371,161.947657581876,162.94285710038,
163.938056618885,164.93325613739,165.928455655894,166.923655174399,167.918854692904,
168.914054211409,169.909253729913,170.904453248418,171.899652766923,172.894852285427,
173.890051803932,174.885251322437,175.880450840942,176.875650359446,177.870849877951,
178.866049396456,179.86124891496,180.856448433465,181.85164795197,182.846847470474,
183.842046988979,184.837597527603),.UNSPECIFIED.);
#1021=SHAPE_REPRESENTATION_RELATIONSHIP('SRR','None',#72025,#1031);
#1031=ADVANCED_BREP_SHAPE_REPRESENTATION('',(#1051),#71793);
#1041=STYLED_ITEM('',(#72084),#1051);
#1051=MANIFOLD_SOLID_BREP('Body1',#13643);
#1097=CONICAL_SURFACE('',#14403,2.16347,0.785398163397448);
#1098=CONICAL_SURFACE('',#14410,3.7624,0.785398163397448);
#1099=CONICAL_SURFACE('',#14603,1.14567944042316,1.02974425867665);
#1250=B_SPLINE_CURVE_WITH_KNOTS('',3,(#37380,#37381,#37382,#37383,#37384,
#37385,#37386,#37387,#37388,#37389,#37390,#37391,#37392,#37393,#37394,#37395,
#37396,#37397,#37398,#37399,#37400,#37401,#37402,#37403,#37404,#37405,#37406,
#37407,#37408,#37409,#37410,#37411,#37412,#37413,#37414,#37415,#37416,#37417,
#37418,#37419,#37420,#37421,#37422,#37423,#37424,#37425,#37426,#37427,#37428,
#37429,#37430,#37431,#37432,#37433,#37434,#37435,#37436,#37437,#37438,#37439,
#37440,#37441,#37442,#37443,#37444,#37445,#37446,#37447,#37448,#37449,#37450,
#37451,#37452,#37453,#37454,#37455,#37456,#37457,#37458,#37459,#37460,#37461,
#37462,#37463,#37464,#37465,#37466,#37467,#37468,#37469,#37470,#37471,#37472,
#37473,#37474,#37475,#37476,#37477,#37478,#37479,#37480,#37481,#37482,#37483,
#37484,#37485,#37486,#37487,#37488,#37489,#37490,#37491,#37492,#37493,#37494,
#37495,#37496,#37497,#37498,#37499,#37500,#37501,#37502,#37503,#37504,#37505,
#37506,#37507,#37508,#37509),.UNSPECIFIED.,.F.,.F.,(4,3,3,3,3,3,3,3,3,3,
3,3,3,3,3,3,3,3,3,3,3,3,3,3,3,3,3,3,3,3,3,3,3,3,3,3,3,3,3,3,3,3,3,4),(10.3186182874641,
10.3239953002556,10.4300038943101,10.5411527598664,10.6468733851658,10.7525295886974,
10.8581575555237,10.9637934277648,11.0695404627179,11.1753522010957,11.2813394755448,
11.3191948187603,11.4252459288507,11.5363894799025,11.6421623944753,11.74787433385,
11.8535614052088,11.9592596763638,12.065073665625,12.1709550724332,12.2770154594751,
12.314394337265,12.4201373345448,12.5257192007202,12.6311751710519,12.7365642163835,
12.8419229525085,12.9472879499407,13.0527650948566,13.1583061525316,13.2640283089846,
13.3095938557697,13.4154942679295,13.5266566562226,13.6322701065976,13.7378198081219,
13.8433421239847,13.9488733752784,14.0545180315408,14.1602285717525,14.2661173730005,
14.3047933742744,14.4106730427761,14.457190242259),.UNSPECIFIED.);
#1251=B_SPLINE_CURVE_WITH_KNOTS('',3,(#37512,#37513,#37514,#37515,#37516,
#37517,#37518,#37519,#37520,#37521,#37522,#37523,#37524,#37525,#37526,#37527,
#37528,#37529,#37530,#37531,#37532,#37533,#37534,#37535,#37536,#37537,#37538,
#37539,#37540,#37541,#37542,#37543,#37544,#37545,#37546,#37547,#37548,#37549,
#37550,#37551,#37552,#37553,#37554,#37555,#37556,#37557,#37558,#37559,#37560,
#37561,#37562,#37563,#37564,#37565,#37566,#37567,#37568,#37569,#37570,#37571,
#37572,#37573,#37574,#37575,#37576,#37577,#37578,#37579,#37580,#37581,#37582,
#37583,#37584,#37585,#37586,#37587,#37588,#37589,#37590,#37591,#37592,#37593,
#37594,#37595,#37596),.UNSPECIFIED.,.F.,.F.,(4,3,3,3,3,3,3,3,3,3,3,3,3,
3,3,3,3,3,3,3,3,3,3,3,3,3,3,3,4),(11.6725302876646,11.7808330913471,11.8916951806998,
11.9999183950615,12.1081436308134,12.2164003956853,12.3292327483063,12.4377217360197,
12.5463108432516,12.6550959203905,12.6677298061693,12.7725797148627,12.8772543949575,
12.9817864245415,13.0862414773316,13.1906574122375,13.295072030404,13.3995935079154,
13.5041742946929,13.6089390469749,13.662929324674,13.768906453379,13.8747386674348,
13.9804623817128,14.0861138807601,14.1917607912468,14.297403516148,14.4031294877355,
14.4560348278906),.UNSPECIFIED.);
#1252=B_SPLINE_CURVE_WITH_KNOTS('',3,(#37602,#37603,#37604,#37605,#37606,
#37607,#37608,#37609,#37610,#37611,#37612,#37613,#37614,#37615,#37616,#37617,
#37618,#37619,#37620,#37621,#37622,#37623,#37624,#37625,#37626,#37627,#37628,
#37629,#37630,#37631,#37632,#37633,#37634,#37635,#37636,#37637,#37638,#37639,
#37640,#37641,#37642,#37643,#37644,#37645,#37646,#37647,#37648,#37649,#37650,
#37651,#37652,#37653,#37654,#37655,#37656,#37657,#37658,#37659,#37660,#37661,
#37662,#37663,#37664,#37665,#37666,#37667,#37668,#37669,#37670,#37671,#37672,
#37673,#37674,#37675,#37676,#37677,#37678,#37679,#37680,#37681,#37682,#37683,
#37684,#37685,#37686,#37687,#37688,#37689,#37690,#37691,#37692,#37693,#37694,
#37695,#37696,#37697,#37698,#37699,#37700,#37701,#37702,#37703,#37704,#37705,
#37706,#37707,#37708,#37709,#37710,#37711,#37712,#37713,#37714,#37715,#37716,
#37717,#37718,#37719,#37720,#37721,#37722,#37723,#37724,#37725,#37726,#37727,
#37728,#37729,#37730,#37731,#37732,#37733,#37734,#37735,#37736,#37737,#37738,
#37739,#37740,#37741,#37742,#37743,#37744,#37745,#37746,#37747,#37748,#37749,
#37750,#37751,#37752,#37753,#37754,#37755),.UNSPECIFIED.,.F.,.F.,(4,3,3,
3,3,3,3,3,3,3,3,3,3,3,3,3,3,3,3,3,3,3,3,3,3,3,3,3,3,3,3,3,3,3,3,3,3,3,3,
3,3,3,3,3,3,3,3,3,3,3,3,4),(15.707963267949,15.8151330995317,15.9223517262571,
16.0297361942916,16.1372132458269,16.2449080240999,16.2951924112838,16.4010712431056,
16.5122363289409,16.6178281121499,16.7233561737618,16.8288569113081,16.9343666802768,
17.0399901377781,17.1456796180955,17.2515477643943,17.2903919297885,17.3962679028274,
17.5074333460106,17.6130223227781,17.7185476047815,17.8240455940151,17.9295526504612,
18.0351734668675,18.1408603442465,18.2467259693383,18.2855914482932,18.3914628384719,
18.5026288545127,18.6082130240858,18.7137334296441,18.8192264806583,18.924728544519,
19.0303443187165,19.1360261191755,19.241886662104,19.2807909667979,19.3866656920306,
19.4978312911896,19.6034189078599,19.7089427922628,19.814439348484,19.9199449385594,
20.0255642478333,20.1312495927124,20.2371136612566,20.2759904853026,20.3818694039373,
20.4875658530965,20.5931570867173,20.698678083258,20.7399394645196),
 .UNSPECIFIED.);
#1253=B_SPLINE_CURVE_WITH_KNOTS('',3,(#37756,#37757,#37758,#37759,#37760,
#37761,#37762,#37763,#37764,#37765,#37766,#37767,#37768,#37769,#37770,#37771,
#37772,#37773,#37774,#37775,#37776,#37777,#37778,#37779,#37780,#37781,#37782,
#37783,#37784,#37785,#37786,#37787,#37788,#37789,#37790,#37791,#37792),
 .UNSPECIFIED.,.F.,.F.,(4,3,3,3,3,3,3,3,3,3,3,3,4),(14.457190242259,14.562854862703,
14.6684337986202,14.7739634667209,14.8794802188877,14.9850965746116,15.0907591877488,
15.1966208740822,15.2999928927791,15.4167046733531,15.5330578786748,15.6488271475791,
15.7079632676211),.UNSPECIFIED.);
#1254=B_SPLINE_CURVE_WITH_KNOTS('',3,(#37794,#37795,#37796,#37797,#37798,
#37799,#37800,#37801,#37802,#37803,#37804,#37805,#37806,#37807,#37808,#37809,
#37810,#37811,#37812,#37813,#37814,#37815,#37816,#37817,#37818,#37819,#37820,
#37821,#37822,#37823,#37824,#37825,#37826,#37827,#37828,#37829,#37830,#37831,
#37832,#37833),.UNSPECIFIED.,.F.,.F.,(4,3,3,3,3,3,3,3,3,3,3,3,3,4),(14.4560348278906,
14.562000547318,14.6581288431788,14.7641800030469,14.8753235478765,14.9810965159128,
15.0868085099609,15.1924956371218,15.2981939651273,15.4040080124557,15.509889478102,
15.6159499246049,15.6533283616835,15.707963267949),.UNSPECIFIED.);
#1255=B_SPLINE_CURVE_WITH_KNOTS('',3,(#37834,#37835,#37836,#37837,#37838,
#37839,#37840,#37841,#37842,#37843,#37844,#37845,#37846,#37847,#37848,#37849,
#37850,#37851,#37852,#37853,#37854,#37855,#37856,#37857,#37858,#37859,#37860,
#37861,#37862,#37863,#37864,#37865,#37866,#37867,#37868,#37869,#37870,#37871,
#37872,#37873,#37874,#37875,#37876,#37877,#37878,#37879,#37880,#37881,#37882,
#37883,#37884,#37885,#37886,#37887,#37888,#37889,#37890,#37891,#37892,#37893,
#37894,#37895,#37896,#37897,#37898,#37899,#37900,#37901,#37902,#37903,#37904,
#37905,#37906,#37907,#37908,#37909,#37910,#37911,#37912,#37913,#37914,#37915,
#37916,#37917,#37918,#37919,#37920,#37921,#37922,#37923,#37924,#37925,#37926,
#37927,#37928,#37929,#37930,#37931,#37932,#37933,#37934,#37935,#37936,#37937,
#37938,#37939,#37940,#37941,#37942,#37943,#37944,#37945,#37946,#37947,#37948,
#37949,#37950,#37951,#37952,#37953,#37954,#37955,#37956,#37957,#37958,#37959,
#37960,#37961,#37962,#37963,#37964,#37965,#37966,#37967,#37968,#37969,#37970,
#37971,#37972,#37973,#37974,#37975,#37976,#37977,#37978,#37979,#37980,#37981,
#37982,#37983,#37984,#37985,#37986,#37987,#37988,#37989,#37990,#37991,#37992,
#37993,#37994,#37995,#37996,#37997,#37998,#37999,#38000,#38001,#38002,#38003,
#38004,#38005,#38006,#38007,#38008,#38009,#38010,#38011),.UNSPECIFIED.,
 .F.,.F.,(4,2,2,2,2,2,2,2,2,2,2,2,2,2,2,2,2,2,2,2,2,2,2,2,2,2,2,2,2,2,2,
2,2,2,2,2,2,2,2,2,2,2,2,2,2,2,2,2,2,2,2,2,2,2,2,2,2,2,2,2,2,2,2,2,2,2,2,
2,2,2,2,2,2,2,2,2,2,2,2,2,2,2,2,2,2,2,2,2,4),(-2.43133029467023,-2.38045001641935,
-2.35582585487554,-2.34996458315354,-2.34737231509244,-2.34544514087839,
-2.34364787513912,-2.34117544414635,-2.33486585233081,-2.28574937995146,
-2.26320221662845,-2.25641259847009,-2.25337582158693,-2.25165987492902,
-2.25015458445799,-2.24908376645736,-2.24807298134615,-2.24639599349135,
-2.2420617591264,-2.20459396018532,-2.20325870874998,-2.16114216120753,
-2.15647733790003,-2.15409971006157,-2.15220279008586,-2.15002604328546,
-2.14630497841577,-2.1327292995895,-2.12305786403638,-2.0723386663915,-2.06093177442003,
-2.05865927109117,-2.05740262436177,-2.0563309285897,-2.05497533199509,
-2.05221788883994,-2.03150830505557,-1.99827162636792,-1.97841989445824,
-1.96681044873025,-1.96343346403003,-1.96133520783537,-1.95940855322915,
-1.95693657970761,-1.95286438517933,-1.92477504883846,-1.87686021439252,
-1.86815836690016,-1.86606893828926,-1.86485555255859,-1.86378135222052,
-1.86239428053879,-1.86008446922467,-1.84548994150369,-1.84188271978142,
-1.83737314524978,-1.78735171086278,-1.77449287947572,-1.77099907195111,
-1.76887677773858,-1.76695963469935,-1.76450247220002,-1.76056358161632,
-1.73709776247759,-1.68729728933206,-1.67596246878737,-1.67370142540451,
-1.67245099739686,-1.67138219433715,-1.67002849029079,-1.66727639878152,
-1.63428435466996,-1.60904546014541,-1.58569358874201,-1.57997665320094,
-1.57739888543641,-1.57546262700068,-1.5736423375891,-1.57111494340174,
-1.56453208978344,-1.51953315279275,-1.49439804095941,-1.48351717476073,
-1.48127975245331,-1.48003320198764,-1.47896300189892,-1.47760087849872,
-1.47480684896619,-1.45825318070351),.UNSPECIFIED.);
#1256=B_SPLINE_CURVE_WITH_KNOTS('',3,(#38017,#38018,#38019,#38020,#38021,
#38022,#38023,#38024,#38025,#38026,#38027,#38028,#38029,#38030,#38031,#38032,
#38033,#38034,#38035,#38036,#38037,#38038,#38039,#38040,#38041,#38042,#38043,
#38044,#38045,#38046,#38047,#38048,#38049,#38050,#38051,#38052,#38053,#38054,
#38055,#38056,#38057,#38058,#38059,#38060,#38061,#38062,#38063,#38064,#38065,
#38066,#38067,#38068,#38069,#38070,#38071,#38072,#38073,#38074,#38075,#38076,
#38077,#38078,#38079,#38080,#38081,#38082,#38083,#38084,#38085,#38086,#38087,
#38088,#38089,#38090,#38091,#38092,#38093,#38094,#38095,#38096,#38097,#38098,
#38099,#38100,#38101,#38102,#38103,#38104,#38105,#38106,#38107,#38108,#38109,
#38110,#38111,#38112,#38113,#38114,#38115,#38116,#38117,#38118,#38119,#38120,
#38121,#38122,#38123,#38124,#38125,#38126,#38127,#38128,#38129,#38130,#38131,
#38132,#38133,#38134,#38135,#38136,#38137,#38138,#38139,#38140,#38141,#38142,
#38143,#38144,#38145,#38146,#38147,#38148,#38149,#38150,#38151,#38152,#38153,
#38154,#38155,#38156,#38157,#38158,#38159,#38160,#38161,#38162,#38163,#38164,
#38165,#38166,#38167,#38168,#38169,#38170,#38171,#38172,#38173,#38174,#38175,
#38176,#38177,#38178,#38179,#38180,#38181,#38182,#38183,#38184,#38185,#38186,
#38187,#38188,#38189,#38190,#38191,#38192,#38193,#38194,#38195,#38196,#38197,
#38198,#38199,#38200),.UNSPECIFIED.,.F.,.F.,(4,2,2,2,2,2,2,2,2,2,2,2,2,
2,2,2,2,2,2,2,2,2,2,2,2,2,2,2,2,2,2,2,2,2,2,2,2,2,2,2,2,2,2,2,2,2,2,2,2,
2,2,2,2,2,2,2,2,2,2,2,2,2,2,2,2,2,2,2,2,2,2,2,2,2,2,2,2,2,2,2,2,2,2,2,2,
2,2,2,2,2,2,4),(-0.973731012778231,-0.955750958635197,-0.927909947755372,
-0.923844024993355,-0.921373817980455,-0.919447326652216,-0.917348026432846,
-0.913966681351581,-0.902316084334358,-0.882364141007552,-0.846990293236625,
-0.842697461103928,-0.828114535608816,-0.825803131074563,-0.824414718568904,
-0.82333944937632,-0.822125063138687,-0.820033087835368,-0.811307980630995,
-0.763285194946165,-0.735403154309707,-0.731336423695054,-0.728866047581838,
-0.726939616766068,-0.724840576847746,-0.721460080022725,-0.709816718998952,
-0.689882362547447,-0.670522457648294,-0.63846656759735,-0.634012125360898,
-0.632315970877924,-0.631301323134629,-0.630204156020763,-0.628653925132381,
-0.624810025087573,-0.605890794874009,-0.580447336426393,-0.569174825301193,
-0.542898176919398,-0.538863974553914,-0.536403146008452,-0.534478019893663,
-0.53237416812308,-0.528972086168774,-0.517113257272782,-0.467748584387895,
-0.443502234065478,-0.440697060970407,-0.439332560367093,-0.438262155148899,
-0.437017434643968,-0.434787607278837,-0.424028574732282,-0.39939235477578,
-0.353670719479631,-0.347123507531396,-0.344601732751843,-0.342782934594833,
-0.34084590276073,-0.338263073718374,-0.332518166164782,-0.324799974382857,
-0.304815429683866,-0.260585220866742,-0.250183900526884,-0.248090563291109,
-0.246752913181188,-0.245684319785793,-0.244419147477469,-0.242095000800413,
-0.229725171460215,-0.197764680691731,-0.160971399894507,-0.154554730935017,
-0.152053934683415,-0.150240545456253,-0.148300202652094,-0.146394599564277,
-0.142044179569303,-0.118569620754311,-0.0985583869616866,-0.0813296821625467,
-0.0793844099193463,-0.0584312395777052,-0.0556646330183186,-0.0543077968269223,
-0.0532380215325895,-0.051987825727483,-0.0497327075339078,-0.0469305815507994,
-0.000564225491686792),.UNSPECIFIED.);
#1257=B_SPLINE_CURVE_WITH_KNOTS('',3,(#38201,#38202,#38203,#38204,#38205,
#38206,#38207,#38208,#38209,#38210,#38211,#38212,#38213,#38214,#38215,#38216,
#38217,#38218,#38219,#38220,#38221,#38222,#38223,#38224,#38225,#38226,#38227,
#38228,#38229,#38230,#38231,#38232,#38233,#38234,#38235,#38236,#38237),
 .UNSPECIFIED.,.F.,.F.,(4,3,3,3,3,3,3,3,3,3,3,3,4),(20.7399394645196,20.8454343576969,
20.9518732692245,21.0575111976985,21.1643506007529,21.2711900038073,21.3761014635548,
21.480866411635,21.5855227766783,21.6901309418475,21.7947058019396,21.8993450709265,
21.9911485751286),.UNSPECIFIED.);
#1258=B_SPLINE_CURVE_WITH_KNOTS('',3,(#38238,#38239,#38240,#38241,#38242,
#38243,#38244,#38245,#38246,#38247,#38248,#38249,#38250,#38251,#38252,#38253,
#38254,#38255,#38256,#38257,#38258,#38259,#38260,#38261,#38262,#38263,#38264,
#38265,#38266,#38267,#38268,#38269,#38270,#38271,#38272,#38273,#38274,#38275,
#38276,#38277,#38278,#38279,#38280,#38281,#38282,#38283,#38284,#38285,#38286,
#38287,#38288,#38289,#38290,#38291,#38292,#38293,#38294,#38295,#38296,#38297,
#38298,#38299,#38300,#38301,#38302,#38303,#38304,#38305,#38306,#38307,#38308,
#38309,#38310,#38311,#38312,#38313,#38314,#38315,#38316,#38317,#38318,#38319,
#38320,#38321,#38322,#38323,#38324,#38325,#38326,#38327,#38328,#38329,#38330,
#38331,#38332,#38333,#38334,#38335,#38336,#38337,#38338,#38339,#38340,#38341,
#38342,#38343,#38344,#38345,#38346,#38347,#38348,#38349,#38350,#38351,#38352,
#38353,#38354,#38355,#38356,#38357,#38358,#38359,#38360,#38361,#38362,#38363,
#38364,#38365,#38366,#38367,#38368,#38369,#38370,#38371,#38372,#38373,#38374,
#38375,#38376,#38377,#38378,#38379,#38380,#38381,#38382,#38383,#38384,#38385,
#38386,#38387,#38388,#38389,#38390,#38391,#38392,#38393,#38394,#38395,#38396,
#38397,#38398,#38399,#38400,#38401,#38402,#38403,#38404,#38405,#38406,#38407,
#38408,#38409,#38410,#38411,#38412,#38413,#38414,#38415,#38416,#38417,#38418,
#38419,#38420,#38421,#38422,#38423,#38424,#38425,#38426,#38427,#38428,#38429,
#38430,#38431,#38432,#38433,#38434,#38435,#38436,#38437,#38438,#38439,#38440,
#38441,#38442,#38443,#38444,#38445,#38446,#38447),.UNSPECIFIED.,.F.,.F.,
(4,2,2,2,2,2,2,2,2,2,2,2,2,2,2,2,2,2,2,2,2,2,2,2,2,2,2,2,2,2,2,2,2,2,2,
2,2,2,2,2,2,2,2,2,2,2,2,2,2,2,2,2,2,2,2,2,2,2,2,2,2,2,2,2,2,2,2,2,2,2,2,
2,2,2,2,2,2,2,2,2,2,2,2,2,2,2,2,2,2,2,2,2,2,2,2,2,2,2,2,2,2,2,2,2,4),(-1.45825318070351,
-1.45156178778247,-1.42090792497479,-1.40102276261981,-1.38939887848518,
-1.38602083639596,-1.38392262513754,-1.38199648791495,-1.37952584138216,
-1.37545724963582,-1.34748120068021,-1.29950333832415,-1.29079437424628,
-1.28870398222319,-1.28749014757655,-1.28641514699885,-1.28502680057963,
-1.28271489394581,-1.2681049786494,-1.26053267416157,-1.21637831561782,
-1.19820627391089,-1.19452940480568,-1.19215069055576,-1.19023982714425,
-1.18806589020858,-1.18434464466145,-1.16872170824729,-1.10977602424721,
-1.09873956671539,-1.0966071259162,-1.09525768936263,-1.09418855470572,
-1.0929330402689,-1.09065330185538,-1.07901753526725,-1.02564218440679,
-1.00579633564512,-1.00202362975111,-0.999615218290805,-0.997701221088182,
-0.995545782674325,-0.991910100888293,-0.977418749284369,-0.949515751727793,
-0.909099786448388,-0.904865961813497,-0.903205015183827,-0.902197083093176,
-0.901094145324588,-0.899513702299606,-0.895479460004572,-0.874680517282409,
-0.832977281385335,-0.813300926898741,-0.809536708368696,-0.807130920758082,
-0.805217220821617,-0.803060222208958,-0.799417318693306,-0.784834337890712,
-0.73530540501547,-0.714355716199509,-0.711589300202888,-0.710232547595368,
-0.709162826002879,-0.7079126754028,-0.705657631261806,-0.694465257317898,
-0.646214321686994,-0.621179007803346,-0.617190326586427,-0.614716520525246,
-0.612795209862247,-0.610677226762678,-0.607210898824432,-0.594682526475048,
-0.54429322378361,-0.541775326839909,-0.534962483064637,-0.521403817291864,
-0.519138492929374,-0.517763632053185,-0.516690000901088,-0.515467352430039,
-0.513338033538654,-0.504109563266951,-0.455558614375983,-0.428725696984432,
-0.424685281485952,-0.422222638518982,-0.420297280843739,-0.418194382487543,
-0.41479652381461,-0.402979963969508,-0.353683036759244,-0.329323022126649,
-0.326516834600987,-0.325152143085468,-0.324081736938291,-0.32283718818749,
-0.320608075622083,-0.309860402849404,-0.285269174135166,-0.242759173181297),
 .UNSPECIFIED.);
#1259=B_SPLINE_CURVE_WITH_KNOTS('',3,(#38452,#38453,#38454,#38455,#38456,
#38457,#38458,#38459,#38460,#38461,#38462,#38463,#38464,#38465,#38466,#38467,
#38468,#38469,#38470,#38471,#38472,#38473,#38474,#38475,#38476,#38477,#38478,
#38479,#38480,#38481,#38482,#38483,#38484,#38485,#38486,#38487,#38488,#38489,
#38490,#38491,#38492,#38493,#38494,#38495,#38496,#38497,#38498,#38499,#38500,
#38501,#38502,#38503,#38504,#38505,#38506,#38507,#38508,#38509,#38510,#38511,
#38512,#38513,#38514,#38515,#38516,#38517,#38518,#38519,#38520,#38521,#38522,
#38523,#38524,#38525,#38526,#38527,#38528,#38529,#38530,#38531,#38532,#38533,
#38534,#38535,#38536,#38537,#38538,#38539,#38540,#38541,#38542,#38543,#38544,
#38545,#38546,#38547,#38548,#38549,#38550,#38551,#38552,#38553,#38554,#38555,
#38556,#38557,#38558,#38559,#38560,#38561,#38562,#38563,#38564,#38565,#38566,
#38567,#38568,#38569,#38570,#38571,#38572,#38573,#38574,#38575,#38576,#38577,
#38578,#38579,#38580,#38581,#38582,#38583,#38584,#38585,#38586,#38587,#38588,
#38589,#38590,#38591,#38592,#38593,#38594,#38595,#38596,#38597,#38598,#38599,
#38600,#38601,#38602,#38603,#38604,#38605,#38606,#38607,#38608,#38609,#38610,
#38611,#38612,#38613,#38614,#38615,#38616,#38617,#38618,#38619,#38620,#38621,
#38622,#38623,#38624,#38625,#38626,#38627,#38628,#38629,#38630,#38631,#38632,
#38633,#38634,#38635,#38636,#38637,#38638,#38639,#38640,#38641,#38642,#38643,
#38644,#38645,#38646,#38647,#38648,#38649,#38650,#38651,#38652,#38653,#38654,
#38655,#38656,#38657,#38658,#38659,#38660,#38661,#38662,#38663,#38664,#38665,
#38666,#38667,#38668,#38669,#38670,#38671,#38672,#38673,#38674,#38675,#38676,
#38677,#38678,#38679),.UNSPECIFIED.,.F.,.F.,(4,2,2,2,2,2,2,2,2,2,2,2,2,
2,2,2,2,2,2,2,2,2,2,2,2,2,2,2,2,2,2,2,2,2,2,2,2,2,2,2,2,2,2,2,2,2,2,2,2,
2,2,2,2,2,2,2,2,2,2,2,2,2,2,2,2,2,2,2,2,2,2,2,2,2,2,2,2,2,2,2,2,2,2,2,2,
2,2,2,2,2,2,2,2,2,2,2,2,2,2,2,2,2,2,2,2,2,2,2,2,2,2,2,2,4),(-2.18907843185636,
-2.1839306013294,-2.17485020575198,-2.17273199547205,-2.17151200523755,
-2.17043821167424,-2.1690599687162,-2.16678258086056,-2.15298325962618,
-2.14407336322025,-2.09404474057858,-2.08113083700294,-2.07762964538173,
-2.07550427092731,-2.07358523571058,-2.07112686624626,-2.06718845219888,
-2.04352277838749,-1.99392469203216,-1.98260702366587,-1.9803451476513,
-1.97909365696134,-1.97802428852795,-1.97666991122767,-1.97391466295616,
-1.94102259251772,-1.91596288141848,-1.8923771341101,-1.88663055052084,
-1.88404773803523,-1.88211102295667,-1.88029273909076,-1.87777202276496,
-1.87122963832237,-1.82541566561039,-1.80082765372363,-1.79008210236407,
-1.7878533619564,-1.78660902981171,-1.78553881750097,-1.78417438900382,
-1.78136876502146,-1.75699340207282,-1.70774602364499,-1.69594469696769,
-1.69254873306982,-1.69044647398244,-1.68852134558622,-1.68605850477318,
-1.68201668517563,-1.65511711555205,-1.60638806299799,-1.59735403843273,
-1.59523899949626,-1.5940195897443,-1.59294547489239,-1.59156575312678,
-1.5892837254437,-1.57538620389586,-1.53753193309329,-1.5052955359033,-1.50087091112575,
-1.49854547458503,-1.49663774468201,-1.49442304134062,-1.49061937817887,
-1.47559385812967,-1.46762063018482,-1.4297860559281,-1.41322955288997,
-1.40479868284896,-1.40272975314678,-1.40152054116425,-1.40044422584235,
-1.39904717505007,-1.39670603320875,-1.38135480916071,-1.34231200871113,
-1.31548288268737,-1.30933359090502,-1.30667934594091,-1.3047306205867,
-1.30293049425767,-1.30048066331338,-1.29436616552681,-1.24352118243223,
-1.22232034260141,-1.21576905562745,-1.21148236839234,-1.20981285835396,
-1.20880331644811,-1.20770183331242,-1.20612900255011,-1.20214357010386,
-1.18183778006478,-1.14511941468412,-1.12031081678326,-1.11632887885858,
-1.11385702466666,-1.11193586457025,-1.10981666469395,-1.10634518918034,
-1.09376300387386,-1.04341552098978,-1.03992207094416,-1.03518427337638,
-1.02062666848119,-1.01831619305407,-1.0169280136395,-1.01585272486253,
-1.01463809124073,-1.01254517944843,-1.00380882148382,-0.973731012778231),
 .UNSPECIFIED.);
#1260=B_SPLINE_CURVE_WITH_KNOTS('',3,(#38681,#38682,#38683,#38684,#38685,
#38686,#38687,#38688,#38689,#38690,#38691,#38692,#38693,#38694,#38695,#38696,
#38697,#38698,#38699,#38700,#38701,#38702,#38703,#38704,#38705,#38706,#38707,
#38708,#38709,#38710,#38711,#38712,#38713,#38714,#38715,#38716,#38717,#38718,
#38719,#38720,#38721,#38722,#38723,#38724,#38725,#38726,#38727,#38728,#38729,
#38730,#38731,#38732,#38733,#38734,#38735,#38736),.UNSPECIFIED.,.F.,.F.,
(4,2,2,2,2,2,2,2,2,2,2,2,2,2,2,2,2,2,2,2,2,2,2,2,2,2,2,4),(-0.242759173181297,
-0.239484908413729,-0.232942998134359,-0.230422100898547,-0.228603562991515,
-0.226666463115397,-0.224134462219529,-0.218612162294353,-0.211204854271706,
-0.192410102059554,-0.15099184128989,-0.136420870478374,-0.134109912752697,
-0.132721617013,-0.131646344922579,-0.130431850700236,-0.128339453177511,
-0.119609190654219,-0.0749861339708847,-0.0622325535010866,-0.0431063276215727,
-0.0393705230611759,-0.036973320299747,-0.0350602865874416,-0.0332660364412645,
-0.0311437737735425,-0.0280691132243875,-0.000562207713922817),
 .UNSPECIFIED.);
#1261=B_SPLINE_CURVE_WITH_KNOTS('',3,(#38737,#38738,#38739,#38740,#38741,
#38742,#38743,#38744,#38745,#38746,#38747,#38748,#38749,#38750,#38751,#38752,
#38753,#38754,#38755,#38756,#38757,#38758,#38759,#38760,#38761,#38762,#38763,
#38764,#38765,#38766,#38767,#38768,#38769,#38770,#38771,#38772,#38773,#38774,
#38775,#38776,#38777,#38778,#38779,#38780,#38781,#38782,#38783,#38784,#38785,
#38786,#38787,#38788,#38789,#38790,#38791,#38792,#38793,#38794,#38795,#38796,
#38797,#38798,#38799,#38800,#38801,#38802,#38803,#38804,#38805,#38806,#38807,
#38808,#38809,#38810,#38811,#38812,#38813,#38814,#38815,#38816,#38817,#38818,
#38819,#38820,#38821,#38822,#38823,#38824,#38825,#38826,#38827,#38828,#38829,
#38830,#38831,#38832,#38833,#38834,#38835,#38836,#38837,#38838,#38839,#38840,
#38841,#38842,#38843,#38844,#38845,#38846,#38847,#38848,#38849,#38850,#38851,
#38852,#38853,#38854,#38855,#38856,#38857,#38858,#38859,#38860,#38861,#38862,
#38863,#38864,#38865,#38866,#38867,#38868,#38869,#38870,#38871,#38872,#38873,
#38874,#38875,#38876,#38877,#38878,#38879,#38880,#38881,#38882,#38883,#38884,
#38885,#38886,#38887,#38888,#38889,#38890,#38891,#38892,#38893,#38894,#38895,
#38896,#38897,#38898,#38899,#38900,#38901,#38902,#38903,#38904,#38905,#38906,
#38907,#38908),.UNSPECIFIED.,.F.,.F.,(4,2,2,2,2,2,2,2,2,2,2,2,2,2,2,2,2,
2,2,2,2,2,2,2,2,2,2,2,2,2,2,2,2,2,2,2,2,2,2,2,2,2,2,2,2,2,2,2,2,2,2,2,2,
2,2,2,2,2,2,2,2,2,2,2,2,2,2,2,2,2,2,2,2,2,2,2,2,2,2,2,2,2,2,2,2,4),(-2.43106450421894,
-2.39856083670546,-2.37674236244877,-2.37260994751277,-2.37101451032931,
-2.36990877942184,-2.36890423794777,-2.36726031490655,-2.36312756464469,
-2.32129209831977,-2.29974641558412,-2.28724398588586,-2.27896222066677,
-2.27605490535705,-2.27426731044241,-2.27234199218159,-2.26987731557179,
-2.2658290795459,-2.23915429692451,-2.19091947104382,-2.18126430669329,
-2.17910533358957,-2.17787627917333,-2.17680395021957,-2.17541678511089,
-2.17315947718651,-2.15975564875051,-2.11477183353478,-2.09118845382734,
-2.08544213871858,-2.08285935469182,-2.0809226242386,-2.07910429922532,
-2.07658348332363,-2.07004059226666,-2.02422976751882,-1.9996387147458,
-1.98889233519711,-1.98666352473376,-1.9854191676788,-1.98434894271607,
-1.98298450976323,-1.9801789165061,-1.95581080779381,-1.90655821994549,
-1.89475388316804,-1.89135759085117,-1.8892552415537,-1.887330105921,-1.88486735962884,
-1.88082591679901,-1.85394312515226,-1.80526015606077,-1.79616893882391,
-1.79404968714631,-1.79282933765577,-1.79175538811095,-1.79037715036878,
-1.78810019381254,-1.77431691885455,-1.76539662913765,-1.71538404556458,
-1.70243737393402,-1.69893281989934,-1.69680646879669,-1.69488723702736,
-1.69242956686465,-1.6884941987051,-1.66525029266196,-1.61524846150961,
-1.6038931854412,-1.60162891305741,-1.60037676902164,-1.59930725544581,
-1.59795322331895,-1.59520041140823,-1.56220203872801,-1.53696107782019,
-1.51359987938577,-1.50788181747465,-1.50530390649304,-1.50336769639834,
-1.50154757213365,-1.49902060750673,-1.49244015029847,-1.45788973492034),
 .UNSPECIFIED.);
#1262=B_SPLINE_CURVE_WITH_KNOTS('',3,(#38914,#38915,#38916,#38917,#38918,
#38919,#38920,#38921,#38922,#38923,#38924,#38925,#38926,#38927,#38928,#38929,
#38930,#38931,#38932,#38933,#38934,#38935,#38936,#38937,#38938,#38939,#38940,
#38941,#38942,#38943,#38944,#38945,#38946,#38947,#38948,#38949,#38950,#38951,
#38952,#38953,#38954,#38955,#38956,#38957,#38958,#38959,#38960,#38961,#38962,
#38963,#38964,#38965,#38966,#38967,#38968,#38969,#38970,#38971,#38972,#38973,
#38974,#38975,#38976,#38977,#38978,#38979,#38980,#38981,#38982,#38983,#38984,
#38985,#38986,#38987,#38988,#38989,#38990,#38991,#38992,#38993,#38994,#38995,
#38996,#38997,#38998,#38999,#39000,#39001,#39002,#39003,#39004,#39005,#39006,
#39007,#39008,#39009,#39010,#39011,#39012,#39013,#39014,#39015,#39016,#39017,
#39018,#39019,#39020,#39021,#39022,#39023,#39024,#39025,#39026,#39027,#39028,
#39029,#39030,#39031,#39032,#39033,#39034,#39035,#39036,#39037,#39038,#39039,
#39040,#39041,#39042,#39043,#39044,#39045,#39046,#39047,#39048,#39049,#39050,
#39051,#39052,#39053,#39054,#39055,#39056,#39057,#39058,#39059,#39060,#39061,
#39062,#39063,#39064,#39065,#39066,#39067,#39068,#39069,#39070,#39071,#39072,
#39073,#39074,#39075,#39076,#39077,#39078,#39079,#39080,#39081,#39082,#39083,
#39084,#39085,#39086,#39087,#39088,#39089,#39090,#39091,#39092,#39093,#39094,
#39095,#39096,#39097,#39098,#39099,#39100,#39101,#39102,#39103,#39104,#39105,
#39106,#39107,#39108,#39109,#39110,#39111,#39112,#39113,#39114,#39115,#39116,
#39117,#39118,#39119,#39120,#39121,#39122,#39123,#39124,#39125,#39126,#39127,
#39128,#39129,#39130,#39131,#39132,#39133,#39134,#39135,#39136,#39137),
 .UNSPECIFIED.,.F.,.F.,(4,2,2,2,2,2,2,2,2,2,2,2,2,2,2,2,2,2,2,2,2,2,2,2,
2,2,2,2,2,2,2,2,2,2,2,2,2,2,2,2,2,2,2,2,2,2,2,2,2,2,2,2,2,2,2,2,2,2,2,2,
2,2,2,2,2,2,2,2,2,2,2,2,2,2,2,2,2,2,2,2,2,2,2,2,2,2,2,2,2,2,2,2,2,2,2,2,
2,2,2,2,2,2,2,2,2,2,2,2,2,2,2,4),(-0.974049502300515,-0.939668666783827,
-0.902923410451016,-0.898553856892679,-0.896870898180754,-0.895858753339227,
-0.894759439644448,-0.893198082359334,-0.889285261111349,-0.86969915682471,
-0.844667352004037,-0.83514015638519,-0.807510274807168,-0.803449377040111,
-0.800980594572217,-0.799054239182555,-0.796954101036965,-0.793569227282947,
-0.781884496908835,-0.76184752887367,-0.723102133264661,-0.707765142038601,
-0.705424196294939,-0.704027102049918,-0.702950652573362,-0.701741163373514,
-0.699671497935943,-0.691233737908456,-0.674660025196731,-0.636815037360663,
-0.628950834903638,-0.613886812162755,-0.610079586229558,-0.607863844696181,
-0.605955842977444,-0.603630854330446,-0.599209479812135,-0.567162280502796,
-0.527685699697228,-0.515040673177024,-0.512820090426797,-0.511443784707103,
-0.510372303045744,-0.509135641296099,-0.506942831513843,-0.496781460444001,
-0.474445634807406,-0.425382181390631,-0.419088858583707,-0.416608623625157,
-0.414800587748342,-0.412856970027851,-0.410233845880524,-0.404263746921691,
-0.378908104764982,-0.338480098460455,-0.322748848151743,-0.320166781566477,
-0.318830188286942,-0.317761660335839,-0.316495652641563,-0.314167567347622,
-0.301598113336664,-0.270736343622129,-0.230053644983765,-0.225940254321415,
-0.223456038041966,-0.221527427290404,-0.221482185472768,-0.221442324415341,
-0.221407200191162,-0.221376245849259,-0.221348962512488,-0.221324912356767,
-0.221303710325948,-0.221285015497597,-0.221262112677871,-0.221239852690074,
-0.221218216089607,-0.221197183392619,-0.221176735743261,-0.221156854892689,
-0.221137524412802,-0.221118728486339,-0.221100448669947,-0.221082669150805,
-0.221065374626108,-0.221048550273309,-0.221032181853345,-0.218813215100687,
-0.214830735898025,-0.209901542601693,-0.199420047216925,-0.168749462403717,
-0.132935679079068,-0.128539983970839,-0.126852896933998,-0.12583996423875,
-0.124741321061993,-0.123183460576993,-0.119292453273063,-0.0999190980505376,
-0.0617594859685334,-0.049449157600044,-0.0360612075894408,-0.0323616080679501,
-0.0301919801619317,-0.0284710675814616,-0.0266505210595801,-0.0244014998863868,
-0.0210199944006751,-0.000563417466375508),.UNSPECIFIED.);
#1263=B_SPLINE_CURVE_WITH_KNOTS('',3,(#39138,#39139,#39140,#39141,#39142,
#39143,#39144,#39145,#39146,#39147,#39148,#39149,#39150,#39151,#39152,#39153,
#39154,#39155,#39156,#39157,#39158,#39159,#39160,#39161,#39162,#39163,#39164,
#39165,#39166,#39167,#39168,#39169,#39170,#39171,#39172,#39173,#39174,#39175,
#39176,#39177,#39178,#39179,#39180,#39181,#39182,#39183,#39184,#39185,#39186,
#39187,#39188,#39189,#39190,#39191,#39192,#39193,#39194,#39195,#39196,#39197,
#39198,#39199,#39200,#39201,#39202,#39203,#39204,#39205,#39206,#39207,#39208,
#39209,#39210,#39211,#39212,#39213,#39214,#39215,#39216,#39217),
 .UNSPECIFIED.,.F.,.F.,(4,2,2,2,2,2,2,2,2,2,2,2,2,2,2,2,2,2,2,2,2,2,2,2,
2,2,2,2,2,2,2,2,2,2,2,2,2,2,2,4),(-2.43093834628344,-2.39397070051664,-2.37058048796982,
-2.36630170697331,-2.36468428417007,-2.36357423807792,-2.36257404593918,
-2.3609530259101,-2.35695582068091,-2.31400700300329,-2.29197204327885,
-2.28032579948885,-2.27501349318285,-2.27079475016954,-2.26851854724156,
-2.26850354307076,-2.26848760853789,-2.26847067571557,-2.26845267052536,
-2.26843351207262,-2.26841311178053,-2.26839137246683,-2.26836818735123,
-2.26834343885347,-2.26831699720751,-2.2682887188571,-2.26825844457562,
-2.26822599736379,-2.26819117997167,-2.26815377194733,-2.26811352626145,
-2.26807016525541,-2.26803603321207,-2.26798677368753,-2.2679150619848,
-2.26598972177671,-2.26352362362469,-2.25947007117894,-2.23261266108948,
-2.18907843185636),.UNSPECIFIED.);
#1264=B_SPLINE_CURVE_WITH_KNOTS('',3,(#39218,#39219,#39220,#39221,#39222,
#39223,#39224,#39225,#39226,#39227,#39228,#39229,#39230,#39231,#39232,#39233,
#39234,#39235,#39236,#39237,#39238,#39239,#39240,#39241,#39242,#39243,#39244,
#39245,#39246,#39247,#39248,#39249,#39250,#39251,#39252,#39253,#39254,#39255,
#39256,#39257,#39258,#39259,#39260,#39261,#39262,#39263,#39264,#39265,#39266,
#39267,#39268,#39269,#39270,#39271,#39272,#39273,#39274,#39275,#39276,#39277,
#39278,#39279,#39280,#39281,#39282,#39283,#39284,#39285,#39286,#39287,#39288,
#39289,#39290,#39291,#39292,#39293,#39294,#39295,#39296,#39297,#39298,#39299,
#39300,#39301,#39302,#39303,#39304,#39305,#39306,#39307,#39308,#39309,#39310,
#39311,#39312,#39313,#39314,#39315,#39316,#39317,#39318,#39319,#39320,#39321,
#39322,#39323,#39324,#39325,#39326,#39327,#39328,#39329,#39330,#39331,#39332,
#39333,#39334,#39335,#39336,#39337,#39338,#39339,#39340,#39341,#39342,#39343,
#39344,#39345,#39346,#39347,#39348,#39349,#39350,#39351,#39352,#39353,#39354,
#39355,#39356,#39357,#39358,#39359,#39360,#39361,#39362,#39363,#39364,#39365,
#39366,#39367,#39368,#39369,#39370,#39371,#39372,#39373,#39374,#39375,#39376,
#39377,#39378,#39379,#39380,#39381,#39382,#39383,#39384,#39385,#39386,#39387,
#39388,#39389,#39390,#39391,#39392,#39393,#39394,#39395,#39396,#39397,#39398,
#39399,#39400,#39401,#39402,#39403,#39404,#39405,#39406,#39407,#39408,#39409,
#39410,#39411,#39412,#39413,#39414,#39415,#39416,#39417,#39418,#39419,#39420,
#39421,#39422,#39423,#39424,#39425,#39426,#39427,#39428,#39429,#39430,#39431,
#39432,#39433,#39434,#39435,#39436,#39437,#39438,#39439,#39440,#39441,#39442,
#39443,#39444,#39445,#39446,#39447),.UNSPECIFIED.,.F.,.F.,(4,2,2,2,2,2,
2,2,2,2,2,2,2,2,2,2,2,2,2,2,2,2,2,2,2,2,2,2,2,2,2,2,2,2,2,2,2,2,2,2,2,2,
2,2,2,2,2,2,2,2,2,2,2,2,2,2,2,2,2,2,2,2,2,2,2,2,2,2,2,2,2,2,2,2,2,2,2,2,
2,2,2,2,2,2,2,2,2,2,2,2,2,2,2,2,2,2,2,2,2,2,2,2,2,2,2,2,2,2,2,2,2,2,2,2,
4),(-1.45788973492034,-1.44728121954649,-1.42221084849868,-1.41134474520948,
-1.40910854636243,-1.40786245858797,-1.40679223899318,-1.40542973937949,
-1.40263457398283,-1.37934069475602,-1.34776007851332,-1.32850668156247,
-1.31713696169503,-1.31378416547413,-1.31169109939208,-1.30976257782796,
-1.30727897943553,-1.30316766916123,-1.27332662366873,-1.24564104468246,
-1.2372790077656,-1.22094418203882,-1.21738131340196,-1.21587764868769,
-1.21478874498355,-1.21361746837589,-1.21171940356069,-1.20517837232685,
-1.19380092690107,-1.16600778296183,-1.12688622356108,-1.12274113106383,
-1.12024767241467,-1.118317729489,-1.11622933928657,-1.11289754020751,-1.10172889385284,
-1.08296142385611,-1.04164101264389,-1.03783609150706,-1.02662417221638,
-1.02447889653974,-1.02312541105238,-1.02205586028173,-1.02080312246978,
-1.01853640295204,-1.00713899693282,-0.95665389978429,-0.945426749053942,
-0.932671842151801,-0.929034758466654,-0.926878944805138,-0.925156315206015,
-0.922839388460946,-0.918456085130867,-0.888030943507583,-0.851998564480172,
-0.848374980401106,-0.834363354910915,-0.832076060398842,-0.830694727931788,
-0.829620337708081,-0.828401715525089,-0.826290571027713,-0.817310809208004,
-0.76855785615866,-0.741649187938735,-0.737606931111413,-0.735143775907819,
-0.733218384570893,-0.731115821977663,-0.727719333659612,-0.715916034779185,
-0.666641219987156,-0.642244417329993,-0.639437952269776,-0.63807322854585,
-0.637002842435684,-0.635758366491829,-0.633529526385042,-0.622785929600139,
-0.598210684958713,-0.552407673828893,-0.545865416441603,-0.543344486491743,
-0.541525957326011,-0.539588896706328,-0.537005487422589,-0.531257023365038,
-0.507657095268978,-0.482576703113886,-0.449664012275572,-0.446907720230216,
-0.445552982054528,-0.444483405761475,-0.443231754005791,-0.440969806764859,
-0.429655661080284,-0.38009810743266,-0.356425316092589,-0.352477419128838,
-0.350015888108703,-0.348096098033331,-0.345971635337019,-0.342475977572016,
-0.329629296459239,-0.279504223382021,-0.270580722951042,-0.256753974007734,
-0.254474890966415,-0.253095979900508,-0.252021886514772,-0.250801794960802,
-0.24868397461504,-0.242450017710487),.UNSPECIFIED.);
#1265=B_SPLINE_CURVE_WITH_KNOTS('',3,(#39452,#39453,#39454,#39455,#39456,
#39457,#39458,#39459,#39460,#39461,#39462,#39463,#39464,#39465,#39466,#39467,
#39468,#39469,#39470,#39471,#39472,#39473,#39474,#39475,#39476,#39477,#39478,
#39479,#39480,#39481,#39482,#39483,#39484,#39485,#39486,#39487,#39488,#39489,
#39490,#39491,#39492,#39493,#39494,#39495,#39496,#39497,#39498,#39499,#39500,
#39501,#39502,#39503,#39504,#39505,#39506,#39507,#39508,#39509,#39510,#39511,
#39512,#39513,#39514,#39515,#39516,#39517,#39518,#39519,#39520,#39521,#39522,
#39523,#39524,#39525,#39526,#39527,#39528,#39529,#39530,#39531,#39532,#39533,
#39534,#39535,#39536,#39537,#39538,#39539,#39540,#39541,#39542,#39543,#39544,
#39545,#39546,#39547,#39548,#39549,#39550,#39551,#39552,#39553,#39554,#39555,
#39556,#39557,#39558,#39559,#39560,#39561,#39562,#39563,#39564,#39565,#39566,
#39567,#39568,#39569,#39570,#39571,#39572,#39573,#39574,#39575,#39576,#39577,
#39578,#39579,#39580,#39581,#39582,#39583,#39584,#39585,#39586,#39587,#39588,
#39589,#39590,#39591,#39592,#39593,#39594,#39595,#39596,#39597,#39598,#39599,
#39600,#39601,#39602,#39603,#39604,#39605,#39606,#39607,#39608,#39609,#39610,
#39611,#39612,#39613,#39614,#39615,#39616,#39617,#39618,#39619,#39620,#39621,
#39622,#39623,#39624,#39625,#39626,#39627,#39628,#39629,#39630,#39631,#39632,
#39633,#39634,#39635,#39636,#39637,#39638,#39639,#39640,#39641,#39642,#39643,
#39644,#39645,#39646,#39647,#39648,#39649,#39650,#39651,#39652,#39653,#39654,
#39655,#39656,#39657,#39658,#39659,#39660,#39661,#39662,#39663,#39664,#39665,
#39666,#39667,#39668,#39669,#39670,#39671,#39672,#39673,#39674,#39675,#39676,
#39677,#39678,#39679,#39680,#39681,#39682,#39683,#39684,#39685),
 .UNSPECIFIED.,.F.,.F.,(4,2,2,2,2,2,2,2,2,2,2,2,2,2,2,2,2,2,2,2,2,2,2,2,
2,2,2,2,2,2,2,2,2,2,2,2,2,2,2,2,2,2,2,2,2,2,2,2,2,2,2,2,2,2,2,2,2,2,2,2,
2,2,2,2,2,2,2,2,2,2,2,2,2,2,2,2,2,2,2,2,2,2,2,2,2,2,2,2,2,2,2,2,2,2,2,2,
2,2,2,2,2,2,2,2,2,2,2,2,2,2,2,2,2,2,2,2,4),(-2.18935248187665,-2.18060066749766,
-2.15694016658323,-2.15118407272377,-2.14859960122188,-2.14666268406757,
-2.14484496893962,-2.14232624925915,-2.13579608245308,-2.08978493478155,
-2.06533993589874,-2.05463044068599,-2.05240392987667,-2.05116011334871,
-2.05008988780738,-2.04872485222336,-2.0459159945143,-2.01731507032644,
-1.96501096126273,-1.95884776140898,-1.95619137442189,-1.95424252348692,
-1.95244329808938,-1.94999625583526,-1.94389681699885,-1.89293421326724,
-1.87181669331227,-1.86199324095131,-1.85982296362902,-1.85859145419472,
-1.85751956066189,-1.8561363427705,-1.85389212123688,-1.84075767891242,
-1.83663677628878,-1.79739848954192,-1.77890347580332,-1.76784751087897,
-1.76452805143229,-1.76244264719452,-1.76051222081093,-1.7580135702108,
-1.75384981185473,-1.71962175099484,-1.69700106213779,-1.67043416967073,
-1.6677376184964,-1.66639499276351,-1.66532638013963,-1.66406581435144,
-1.66182497834639,-1.65217686663973,-1.64668268224548,-1.64343190088964,
-1.6071309288505,-1.58718087532719,-1.57553045135644,-1.57214954096179,
-1.57005058069742,-1.56812444738517,-1.56565476177136,-1.5615897988422,
-1.53377242182849,-1.48567445613213,-1.47692957908397,-1.47483618816815,
-1.47362155248537,-1.47254644189409,-1.47115873906295,-1.46884957918566,
-1.45431683617923,-1.41310881236197,-1.3941816503753,-1.38294619856559,
-1.37960763855067,-1.37751789578559,-1.37558866205773,-1.37309886484303,
-1.36896580734986,-1.32913662252565,-1.29758323813264,-1.28487092155145,
-1.28253604786515,-1.28126868035578,-1.28020038155685,-1.27886581316868,
-1.27678224874297,-1.26652794218534,-1.26169040461733,-1.25848401248425,
-1.21625766280637,-1.19236615165704,-1.18841185403942,-1.18594838990454,
-1.18402835893277,-1.18190492033105,-1.17841391748335,-1.1656183993103,
-1.1154512933227,-1.10655266306099,-1.09769458274199,-1.09160171006255,
-1.08967988583714,-1.08850333668462,-1.08741668501776,-1.08592632933243,
-1.08244081493993,-1.07756942812815,-1.0641969279115,-1.01260095594681,
-0.998688442087327,-0.994983744058309,-0.992791771793684,-0.990882235579823,
-0.988527333152801,-0.983960819019553,-0.974049502300515),.UNSPECIFIED.);
#1266=B_SPLINE_CURVE_WITH_KNOTS('',3,(#39687,#39688,#39689,#39690,#39691,
#39692,#39693,#39694,#39695,#39696,#39697,#39698,#39699,#39700,#39701,#39702,
#39703,#39704,#39705,#39706,#39707,#39708,#39709,#39710,#39711,#39712,#39713,
#39714,#39715,#39716,#39717,#39718,#39719,#39720,#39721,#39722,#39723,#39724,
#39725,#39726,#39727,#39728),.UNSPECIFIED.,.F.,.F.,(4,2,2,2,2,2,2,2,2,2,
2,2,2,2,2,2,2,2,2,2,4),(-0.242450017710487,-0.239613473062178,-0.190935717053101,
-0.164054434004285,-0.160012895157732,-0.157549959845364,-0.155624609592036,
-0.153836590607114,-0.150925281606183,-0.142625917540657,-0.130083569029777,
-0.108179587073087,-0.0668015315072034,-0.0626017132925774,-0.0609463002630057,
-0.0599394409044324,-0.0588355042916628,-0.0572500557751757,-0.0531838315658337,
-0.0320590766620085,-0.000564309293417658),.UNSPECIFIED.);
#1267=B_SPLINE_CURVE_WITH_KNOTS('',3,(#39729,#39730,#39731,#39732,#39733,
#39734,#39735,#39736,#39737,#39738,#39739,#39740,#39741,#39742,#39743,#39744,
#39745,#39746,#39747,#39748,#39749,#39750,#39751,#39752,#39753,#39754,#39755,
#39756,#39757,#39758,#39759,#39760,#39761,#39762,#39763,#39764,#39765,#39766,
#39767,#39768,#39769,#39770,#39771,#39772,#39773,#39774,#39775,#39776,#39777,
#39778,#39779,#39780,#39781,#39782,#39783,#39784,#39785,#39786,#39787,#39788,
#39789,#39790,#39791,#39792,#39793,#39794,#39795,#39796,#39797,#39798,#39799,
#39800,#39801,#39802,#39803,#39804,#39805,#39806,#39807,#39808,#39809,#39810,
#39811,#39812,#39813,#39814,#39815,#39816,#39817,#39818,#39819,#39820,#39821,
#39822,#39823,#39824,#39825,#39826,#39827,#39828,#39829,#39830,#39831,#39832,
#39833,#39834,#39835,#39836,#39837,#39838,#39839,#39840,#39841,#39842,#39843,
#39844,#39845,#39846,#39847,#39848,#39849,#39850,#39851,#39852,#39853,#39854,
#39855,#39856,#39857,#39858,#39859,#39860,#39861,#39862,#39863,#39864,#39865,
#39866,#39867,#39868,#39869,#39870,#39871,#39872,#39873,#39874,#39875,#39876,
#39877,#39878,#39879,#39880,#39881,#39882,#39883,#39884,#39885,#39886,#39887,
#39888,#39889,#39890,#39891,#39892,#39893,#39894,#39895,#39896,#39897,#39898,
#39899,#39900,#39901,#39902,#39903,#39904,#39905,#39906,#39907,#39908,#39909,
#39910),.UNSPECIFIED.,.F.,.F.,(4,2,2,2,2,2,2,2,2,2,2,2,2,2,2,2,2,2,2,2,
2,2,2,2,2,2,2,2,2,2,2,2,2,2,2,2,2,2,2,2,2,2,2,2,2,2,2,2,2,2,2,2,2,2,2,2,
2,2,2,2,2,2,2,2,2,2,2,2,2,2,2,2,2,2,2,2,2,2,2,2,2,2,2,2,2,2,2,2,2,2,4),
(-2.43147070535632,-2.40300556094277,-2.39963156188484,-2.39738592739693,
-2.39556668374874,-2.39367853485371,-2.39144549981715,-2.38756058344078,
-2.37147569928083,-2.36550631723452,-2.35221906982282,-2.31294397103424,
-2.3021952056922,-2.29996651027028,-2.29872230187077,-2.29765225773529,
-2.29628812360843,-2.29348337379555,-2.26427055269208,-2.23793401837194,
-2.21916095273017,-2.21175959069598,-2.20624169758611,-2.20371034602944,
-2.20177374242271,-2.19995566421347,-2.19743539402241,-2.19089510865308,
-2.14508228266071,-2.12049602366336,-2.10975125662286,-2.10752268455289,
-2.10627844725858,-2.10520831710629,-2.10384399431071,-2.10103859108146,
-2.07666592890003,-2.02742166491021,-2.01562086601409,-2.0122251247061,
-2.01012301841169,-2.00819803996524,-2.00573540483696,-2.00169395249485,
-1.97479880611712,-1.92608023587121,-1.91703857223042,-1.91492308250195,
-1.91370363088909,-1.91262962485615,-1.91125022976533,-1.90896912756493,
-1.89508957154718,-1.85425176992584,-1.82760849123504,-1.82148173486223,
-1.81883154172982,-1.81688365480492,-1.81508279798496,-1.81262965525182,
-1.80649483109552,-1.75584471168521,-1.73452469544941,-1.72464410995741,
-1.72246991923611,-1.72123749704616,-1.72016565358985,-1.71878360770034,
-1.71654346073459,-1.70349530646087,-1.69586373357149,-1.65962603782693,
-1.63479319467049,-1.62888809174351,-1.62627671094222,-1.62433525630996,
-1.62252453751998,-1.62003325829708,-1.61367269863085,-1.56534582288567,
-1.54249751157193,-1.53220006802035,-1.52999877622483,-1.52876036673041,
-1.5276892968553,-1.52631603775879,-1.52410525764287,-1.51164787092179,
-1.50692332461291,-1.46352326967845,-1.45811225063465),.UNSPECIFIED.);
#1268=B_SPLINE_CURVE_WITH_KNOTS('',3,(#39916,#39917,#39918,#39919,#39920,
#39921,#39922,#39923,#39924,#39925,#39926,#39927,#39928,#39929,#39930,#39931,
#39932,#39933,#39934,#39935,#39936,#39937,#39938,#39939,#39940,#39941,#39942,
#39943,#39944,#39945,#39946,#39947,#39948,#39949,#39950,#39951,#39952,#39953,
#39954,#39955,#39956,#39957,#39958,#39959,#39960,#39961,#39962,#39963,#39964,
#39965,#39966,#39967,#39968,#39969,#39970,#39971,#39972,#39973,#39974,#39975,
#39976,#39977,#39978,#39979,#39980,#39981,#39982,#39983,#39984,#39985,#39986,
#39987,#39988,#39989,#39990,#39991,#39992,#39993,#39994,#39995,#39996,#39997,
#39998,#39999,#40000,#40001,#40002,#40003,#40004,#40005,#40006,#40007,#40008,
#40009,#40010,#40011,#40012,#40013,#40014,#40015,#40016,#40017,#40018,#40019,
#40020,#40021,#40022,#40023,#40024,#40025,#40026,#40027,#40028,#40029,#40030,
#40031,#40032,#40033,#40034,#40035,#40036,#40037,#40038,#40039,#40040,#40041,
#40042,#40043,#40044,#40045,#40046,#40047,#40048,#40049,#40050,#40051,#40052,
#40053,#40054,#40055,#40056,#40057,#40058,#40059,#40060,#40061,#40062,#40063,
#40064,#40065,#40066,#40067,#40068,#40069,#40070,#40071,#40072,#40073,#40074,
#40075,#40076,#40077,#40078,#40079,#40080,#40081,#40082,#40083,#40084,#40085,
#40086,#40087,#40088,#40089,#40090,#40091,#40092,#40093,#40094,#40095,#40096,
#40097,#40098,#40099,#40100,#40101,#40102,#40103,#40104,#40105),
 .UNSPECIFIED.,.F.,.F.,(4,2,2,2,2,2,2,2,2,2,2,2,2,2,2,2,2,2,2,2,2,2,2,2,
2,2,2,2,2,2,2,2,2,2,2,2,2,2,2,2,2,2,2,2,2,2,2,2,2,2,2,2,2,2,2,2,2,2,2,2,
2,2,2,2,2,2,2,2,2,2,2,2,2,2,2,2,2,2,2,2,2,2,2,2,2,2,2,2,2,2,2,2,2,2,4),
(-0.973880464698564,-0.972269911093484,-0.969457378845782,-0.968091411426718,
-0.967020867405405,-0.96577714487014,-0.963551956960564,-0.952870471028589,
-0.928543279543384,-0.882387778249055,-0.875866516807864,-0.873348841111349,
-0.871531099753036,-0.869593431561668,-0.867006721865821,-0.861240473108374,
-0.837503321861841,-0.805408902237263,-0.779763040997667,-0.776947041813183,
-0.775580422480422,-0.774509861087641,-0.773266683782313,-0.771043858624368,
-0.760400345293145,-0.736222472933244,-0.689859125910439,-0.683351558937275,
-0.680836131057608,-0.679019024004365,-0.677081113987435,-0.674492499333955,
-0.668715352300812,-0.64489232770314,-0.612518230785388,-0.587253647670481,
-0.584440197257536,-0.583074112974796,-0.582003634870122,-0.580760169417441,
-0.578535884619285,-0.567867258045739,-0.543589536267181,-0.497370624181562,
-0.490854124820034,-0.488337326480139,-0.486519906768528,-0.484582292073066,
-0.481995155339175,-0.476225861051315,-0.452463280515828,-0.420277869357716,
-0.416501889836401,-0.394702732168843,-0.391925571083226,-0.390566707532061,
-0.389496856009609,-0.388248321095346,-0.386000598833899,-0.37493474536427,
-0.349041885940512,-0.305052298328393,-0.298418648747195,-0.295883577305447,
-0.294061405077351,-0.292126509122557,-0.289556322752951,-0.283880113573802,
-0.260836545559236,-0.235320547067467,-0.202177715473949,-0.199426441543799,
-0.198072752606125,-0.19702906937169,-0.195814034912246,-0.194510415399186,
-0.192500346305293,-0.188709621849118,-0.177852689857685,-0.123605809715138,
-0.10807550640261,-0.104233390007135,-0.102009954033067,-0.100102833316269,
-0.0977882547111115,-0.0934150861284736,-0.0633686667400292,-0.0132863794194273,
-0.00797944871388667,-0.0061591313381461,-0.00512003665360846,-0.00408773129344569,
-0.00302632206325726,-0.00169493168175966,-0.000563682644051655),
 .UNSPECIFIED.);
#1269=B_SPLINE_CURVE_WITH_KNOTS('',3,(#40106,#40107,#40108,#40109,#40110,
#40111,#40112,#40113,#40114,#40115,#40116,#40117,#40118,#40119,#40120,#40121,
#40122,#40123,#40124,#40125,#40126,#40127,#40128,#40129,#40130,#40131,#40132,
#40133,#40134,#40135,#40136,#40137,#40138,#40139,#40140,#40141,#40142,#40143,
#40144,#40145,#40146,#40147,#40148,#40149,#40150,#40151,#40152,#40153,#40154,
#40155,#40156,#40157,#40158,#40159,#40160,#40161,#40162,#40163,#40164,#40165,
#40166,#40167,#40168,#40169,#40170,#40171,#40172,#40173,#40174,#40175,#40176,
#40177,#40178,#40179,#40180,#40181,#40182,#40183,#40184,#40185),
 .UNSPECIFIED.,.F.,.F.,(4,2,2,2,2,2,2,2,2,2,2,2,2,2,2,2,2,2,2,2,2,2,2,2,
2,2,2,2,2,2,2,2,2,2,2,2,2,2,2,4),(-2.4313535774442,-2.42510807129326,-2.39735431592081,
-2.37085249543322,-2.34904123187566,-2.34352840192528,-2.34098866370796,
-2.33905874223842,-2.33722792421159,-2.33414261554579,-2.32583364557825,
-2.32481127129679,-2.27582979560085,-2.24834597515755,-2.24625271318251,
-2.24491477371547,-2.24367413235542,-2.24366896022422,-2.24366374095101,
-2.24365847351217,-2.24365315693452,-2.24364779010072,-2.24364237193938,
-2.24363690125186,-2.24363137687909,-2.24362579761802,-2.2436201623626,
-2.24361446970691,-2.2436087184551,-2.24360290725867,-2.24359703462071,
-2.24359109923169,-2.24358509947373,-2.24357903387616,-2.24357290098285,
-2.24253144952348,-2.24115684924962,-2.23845773220675,-2.20560943320674,
-2.18935248187665),.UNSPECIFIED.);
#1270=B_SPLINE_CURVE_WITH_KNOTS('',3,(#40186,#40187,#40188,#40189,#40190,
#40191,#40192,#40193,#40194,#40195,#40196,#40197,#40198,#40199,#40200,#40201,
#40202,#40203,#40204,#40205,#40206,#40207,#40208,#40209,#40210,#40211,#40212,
#40213,#40214,#40215,#40216,#40217,#40218,#40219,#40220,#40221,#40222,#40223,
#40224,#40225,#40226,#40227,#40228,#40229,#40230,#40231,#40232,#40233,#40234,
#40235,#40236,#40237,#40238,#40239,#40240,#40241,#40242,#40243,#40244,#40245,
#40246,#40247,#40248,#40249,#40250,#40251,#40252,#40253,#40254,#40255,#40256,
#40257,#40258,#40259,#40260,#40261,#40262,#40263,#40264,#40265,#40266,#40267,
#40268,#40269,#40270,#40271,#40272,#40273,#40274,#40275,#40276,#40277,#40278,
#40279,#40280,#40281,#40282,#40283,#40284,#40285,#40286,#40287,#40288,#40289,
#40290,#40291,#40292,#40293,#40294,#40295,#40296,#40297,#40298,#40299,#40300,
#40301,#40302,#40303,#40304,#40305,#40306,#40307,#40308,#40309,#40310,#40311,
#40312,#40313,#40314,#40315,#40316,#40317,#40318,#40319,#40320,#40321,#40322,
#40323,#40324,#40325,#40326,#40327,#40328,#40329,#40330,#40331,#40332,#40333,
#40334,#40335,#40336,#40337,#40338,#40339,#40340,#40341,#40342,#40343,#40344,
#40345,#40346,#40347,#40348,#40349,#40350,#40351,#40352,#40353,#40354,#40355,
#40356,#40357,#40358,#40359,#40360,#40361,#40362,#40363,#40364,#40365,#40366,
#40367,#40368,#40369,#40370,#40371,#40372,#40373,#40374,#40375,#40376,#40377,
#40378,#40379,#40380,#40381,#40382,#40383,#40384,#40385,#40386,#40387,#40388,
#40389,#40390,#40391,#40392,#40393,#40394,#40395,#40396,#40397,#40398,#40399,
#40400,#40401,#40402,#40403,#40404,#40405,#40406,#40407,#40408,#40409,#40410,
#40411,#40412,#40413),.UNSPECIFIED.,.F.,.F.,(4,2,2,2,2,2,2,2,2,2,2,2,2,
2,2,2,2,2,2,2,2,2,2,2,2,2,2,2,2,2,2,2,2,2,2,2,2,2,2,2,2,2,2,2,2,2,2,2,2,
2,2,2,2,2,2,2,2,2,2,2,2,2,2,2,2,2,2,2,2,2,2,2,2,2,2,2,2,2,2,2,2,2,2,2,2,
2,2,2,2,2,2,2,2,2,2,2,2,2,2,2,2,2,2,2,2,2,2,2,2,2,2,2,2,4),(-1.45811225063465,
-1.44170082180132,-1.43618582134325,-1.43364528846694,-1.43171484819826,
-1.42988360138484,-1.42679772386231,-1.41848826947098,-1.4165222193944,
-1.36594710220237,-1.34827985806994,-1.33948849992986,-1.33739143884113,
-1.33617592121108,-1.33510087351288,-1.33371433877708,-1.33140938767511,
-1.3169826198997,-1.31323902374403,-1.30961068878169,-1.26511237152881,
-1.24656587566988,-1.24265254902188,-1.24043611814186,-1.23872004850519,
-1.23647768428818,-1.23255374644359,-1.21593802447899,-1.1793488152984,
-1.16009498377915,-1.14762034011282,-1.145408571095,-1.14403499457011,-1.14296386468914,
-1.14172559042497,-1.13952504904511,-1.12923985212111,-1.10644047917935,
-1.05807986143029,-1.05172470419247,-1.04923426983626,-1.04742372312006,
-1.04548203791393,-1.04286963059341,-1.03695912812163,-1.0120807065289,
-0.975526007447791,-0.968861951198427,-0.955222582590498,-0.952952885198095,
-0.951576775429746,-0.950503058319238,-0.949281334180986,-0.947155945638413,
-0.937980459394101,-0.889391010616536,-0.862543504115506,-0.858502987268429,
-0.85604041671282,-0.854115196466913,-0.852012530416708,-0.848615230141997,
-0.836802501174192,-0.787514522134391,-0.763146661402301,-0.760340605634563,
-0.758976008164643,-0.757905686150994,-0.756661244654995,-0.754432367584388,
-0.743686675979851,-0.719102034132714,-0.67331664825625,-0.666773868535854,
-0.664252939054944,-0.662434474839119,-0.66049754325791,-0.657914408952143,
-0.652166987107334,-0.628573976464478,-0.603490708992825,-0.570577345053661,
-0.567821288068995,-0.566466641813923,-0.565397126535096,-0.564145532806228,
-0.561883656827096,-0.550569161633893,-0.501003570372116,-0.47734334827208,
-0.473396000960714,-0.470934706787354,-0.469015036185457,-0.466890639150764,
-0.463394936107679,-0.450546324335389,-0.400426224341905,-0.37809074440209,
-0.375302693741566,-0.373941669709287,-0.372871649728039,-0.37162468239229,
-0.369384164216112,-0.358441940004316,-0.333061062736163,-0.288376260763831,
-0.281774636441631,-0.279244502087781,-0.27742363244446,-0.275488048658781,
-0.272913409092824,-0.267212729661355,-0.243981066307571,-0.242694324494143),
 .UNSPECIFIED.);
#1271=B_SPLINE_CURVE_WITH_KNOTS('',3,(#40418,#40419,#40420,#40421,#40422,
#40423,#40424,#40425,#40426,#40427,#40428,#40429,#40430,#40431,#40432,#40433,
#40434,#40435,#40436,#40437,#40438,#40439,#40440,#40441,#40442,#40443,#40444,
#40445,#40446,#40447,#40448,#40449,#40450,#40451,#40452,#40453,#40454,#40455,
#40456,#40457,#40458,#40459,#40460,#40461,#40462,#40463,#40464,#40465,#40466,
#40467,#40468,#40469,#40470,#40471,#40472,#40473,#40474,#40475,#40476,#40477,
#40478,#40479,#40480,#40481,#40482,#40483,#40484,#40485,#40486,#40487,#40488,
#40489,#40490,#40491,#40492,#40493,#40494,#40495,#40496,#40497,#40498,#40499,
#40500,#40501,#40502,#40503,#40504,#40505,#40506,#40507,#40508,#40509,#40510,
#40511,#40512,#40513,#40514,#40515,#40516,#40517,#40518,#40519,#40520,#40521,
#40522,#40523,#40524,#40525,#40526,#40527,#40528,#40529,#40530,#40531,#40532,
#40533,#40534,#40535,#40536,#40537,#40538,#40539,#40540,#40541,#40542,#40543,
#40544,#40545,#40546,#40547,#40548,#40549,#40550,#40551,#40552,#40553,#40554,
#40555,#40556,#40557,#40558,#40559,#40560,#40561,#40562,#40563,#40564,#40565,
#40566,#40567,#40568,#40569,#40570,#40571,#40572,#40573,#40574,#40575,#40576,
#40577,#40578,#40579,#40580,#40581,#40582,#40583,#40584,#40585,#40586,#40587,
#40588,#40589,#40590,#40591,#40592,#40593,#40594,#40595,#40596,#40597,#40598,
#40599,#40600,#40601,#40602,#40603,#40604,#40605,#40606,#40607,#40608,#40609,
#40610,#40611,#40612,#40613,#40614,#40615,#40616,#40617,#40618,#40619,#40620,
#40621,#40622,#40623,#40624,#40625,#40626,#40627,#40628,#40629,#40630,#40631,
#40632,#40633),.UNSPECIFIED.,.F.,.F.,(4,2,2,2,2,2,2,2,2,2,2,2,2,2,2,2,2,
2,2,2,2,2,2,2,2,2,2,2,2,2,2,2,2,2,2,2,2,2,2,2,2,2,2,2,2,2,2,2,2,2,2,2,2,
2,2,2,2,2,2,2,2,2,2,2,2,2,2,2,2,2,2,2,2,2,2,2,2,2,2,2,2,2,2,2,2,2,2,2,2,
2,2,2,2,2,2,2,2,2,2,2,2,2,2,2,2,2,2,4),(-2.18940658193359,-2.16144257327339,
-2.13712099329524,-2.12644165044395,-2.12421662887569,-2.12297297834277,
-2.1219024780941,-2.12053655223453,-2.11772404374133,-2.0925695938446,-2.06014355461465,
-2.03630392865665,-2.03052412119434,-2.02793495096009,-2.02599687479963,
-2.02417978858807,-2.02166466999551,-2.01515955612574,-1.96870351955098,
-1.94455905100501,-1.93392429751389,-1.93170188152769,-1.9304587522863,
-1.92938811365604,-1.92802125155263,-1.92520425142244,-1.89935050708435,
-1.8703445606534,-1.84420648875698,-1.83813988678378,-1.83549970273249,
-1.8335530958362,-1.83174912232173,-1.82928508310506,-1.8230881048389,-1.77299492340303,
-1.75448464401906,-1.74160149573924,-1.73925804394325,-1.73798866066294,
-1.73692021949006,-1.73558742889287,-1.73351017519861,-1.72335655509252,
-1.68067243928948,-1.6490806007065,-1.64466924860686,-1.64234623579676,
-1.64043817531106,-1.63822046295688,-1.63440514597119,-1.61924535681772,
-1.61150245729804,-1.57361820968498,-1.55702718568849,-1.54858416943477,
-1.5465139282218,-1.54530423929898,-1.5442276986449,-1.54283061388871,-1.54048996215428,
-1.52516330792117,-1.51783757855562,-1.46768342936896,-1.4548923192832,
-1.45140132442633,-1.44927764382689,-1.44735723351125,-1.44489305927805,
-1.44093713374117,-1.41702272421784,-1.38100908984842,-1.36446838835635,
-1.35604213761666,-1.35397328633343,-1.35276393683969,-1.35168737320398,
-1.35028983644486,-1.34794753345849,-1.33257510891003,-1.2918535263551,
-1.27319073354756,-1.2620639423948,-1.25873635117821,-1.25664875288808,
-1.25471828327463,-1.25222237371355,-1.24806930345205,-1.21578564165102,
-1.19326211510147,-1.16479918968955,-1.16198137568129,-1.16061433404227,
-1.15954366092882,-1.15830060481519,-1.15607861145084,-1.14545084611257,
-1.12133637463227,-1.07487668668413,-1.06837469763743,-1.06586004743169,
-1.0640430517866,-1.06210484214885,-1.05951510558615,-1.05373241602226,
-1.0298677757197,-0.997378655514071,-0.973880464698564),.UNSPECIFIED.);
#1272=B_SPLINE_CURVE_WITH_KNOTS('',3,(#40635,#40636,#40637,#40638,#40639,
#40640,#40641,#40642,#40643,#40644,#40645,#40646,#40647,#40648,#40649,#40650,
#40651,#40652,#40653,#40654,#40655,#40656,#40657,#40658,#40659,#40660,#40661,
#40662,#40663,#40664,#40665,#40666,#40667,#40668,#40669,#40670,#40671,#40672,
#40673,#40674,#40675,#40676,#40677,#40678,#40679,#40680,#40681,#40682,#40683,
#40684,#40685,#40686,#40687,#40688,#40689,#40690,#40691,#40692,#40693,#40694,
#40695,#40696),.UNSPECIFIED.,.F.,.F.,(4,2,2,2,2,2,2,2,2,2,2,2,2,2,2,2,2,
2,2,2,2,2,2,2,2,2,2,2,2,2,4),(-0.242694324494143,-0.218605650932494,-0.185552121754827,
-0.182797511274354,-0.181443159544478,-0.180406009161524,-0.180400810290624,
-0.180395681461162,-0.180390621373856,-0.180385628707869,-0.180380702107863,
-0.180375840415643,-0.18037104225267,-0.180366306480232,-0.180361631974136,
-0.180357017665444,-0.179123693304752,-0.177796221260034,-0.175728472628226,
-0.1717832401797,-0.161960968930813,-0.115026663723998,-0.103806571378454,
-0.0910204854260511,-0.087380530540636,-0.0852242461373569,-0.0835019252520926,
-0.0811862994677313,-0.0768084010236629,-0.0465816149829859,-0.000564402028610045),
 .UNSPECIFIED.);
#1273=B_SPLINE_CURVE_WITH_KNOTS('',3,(#40697,#40698,#40699,#40700,#40701,
#40702,#40703,#40704,#40705,#40706,#40707,#40708,#40709,#40710,#40711,#40712,
#40713,#40714,#40715,#40716,#40717,#40718,#40719,#40720,#40721,#40722,#40723,
#40724,#40725,#40726,#40727,#40728,#40729,#40730,#40731,#40732,#40733,#40734,
#40735,#40736,#40737,#40738,#40739,#40740,#40741,#40742,#40743,#40744,#40745,
#40746,#40747,#40748,#40749,#40750,#40751,#40752,#40753,#40754,#40755,#40756,
#40757,#40758,#40759,#40760,#40761,#40762,#40763,#40764,#40765,#40766,#40767,
#40768,#40769,#40770,#40771,#40772,#40773,#40774,#40775,#40776,#40777,#40778,
#40779,#40780,#40781,#40782,#40783,#40784,#40785,#40786,#40787,#40788,#40789,
#40790,#40791,#40792,#40793,#40794,#40795,#40796,#40797,#40798,#40799,#40800,
#40801,#40802,#40803,#40804,#40805,#40806,#40807,#40808,#40809,#40810,#40811,
#40812,#40813,#40814,#40815,#40816,#40817,#40818,#40819,#40820,#40821,#40822,
#40823,#40824,#40825,#40826,#40827,#40828,#40829,#40830,#40831,#40832,#40833,
#40834,#40835,#40836,#40837,#40838,#40839,#40840,#40841,#40842,#40843,#40844,
#40845,#40846,#40847,#40848,#40849,#40850,#40851,#40852,#40853,#40854,#40855,
#40856,#40857,#40858,#40859,#40860,#40861,#40862,#40863,#40864,#40865,#40866,
#40867,#40868,#40869,#40870,#40871,#40872,#40873,#40874,#40875,#40876,#40877,
#40878,#40879,#40880,#40881,#40882,#40883,#40884,#40885,#40886,#40887,#40888,
#40889,#40890),.UNSPECIFIED.,.F.,.F.,(4,2,2,2,2,2,2,2,2,2,2,2,2,2,2,2,2,
2,2,2,2,2,2,2,2,2,2,2,2,2,2,2,2,2,2,2,2,2,2,2,2,2,2,2,2,2,2,2,2,2,2,2,2,
2,2,2,2,2,2,2,2,2,2,2,2,2,2,2,2,2,2,2,2,2,2,2,2,2,2,2,2,2,2,2,2,2,2,2,2,
2,2,2,2,2,2,2,4),(-2.4317062866866,-2.42631946932063,-2.42284242681522,
-2.42138712823313,-2.42030635631367,-2.41929078546131,-2.41827619804741,
-2.41658068528834,-2.412131014088,-2.4042631093833,-2.35755483301902,-2.33076585912172,
-2.32648682003991,-2.32419183435477,-2.32230310789888,-2.32006893514292,
-2.31618089233947,-2.30006479595078,-2.29414997942651,-2.25400673339955,
-2.23851616165929,-2.2331462770639,-2.2305711188579,-2.22848372097956,-2.22728189948522,
-2.2272783209793,-2.22727472446683,-2.22727111019277,-2.22726707779843,
-2.22726295734438,-2.22627413439945,-2.2249248760073,-2.22219608205174,
-2.20297217965708,-2.16689246046896,-2.14785413817739,-2.13657261230876,
-2.13322903487839,-2.1311380516908,-2.12920896144971,-2.12672115297072,
-2.12259531964831,-2.09204332782668,-2.06523540897104,-2.04143514287707,
-2.0371183630271,-2.03549492471133,-2.03438335856718,-2.03338376108912,
-2.03176742393232,-2.02780017460041,-1.98463327652318,-1.94618210521712,
-1.94165667913121,-1.93931021770443,-1.93740119453352,-1.93520279048105,
-1.93147034085856,-1.91724937590887,-1.90784956577158,-1.85723685355633,
-1.84582687396493,-1.84355937852569,-1.84230645713313,-1.8412368955595,
-1.8398835907454,-1.83713483704096,-1.80394389373345,-1.77834739718764,
-1.75543209513847,-1.74977179704114,-1.74720425223577,-1.74526949748954,
-1.74344609704551,-1.74090712924979,-1.73424975188637,-1.69074788332287,
-1.66445024573998,-1.65328764777817,-1.65103403222151,-1.64978408218889,
-1.64871416178508,-1.64735668774601,-1.64458723953504,-1.62351387319986,
-1.57412066204767,-1.55955581103137,-1.55591398846505,-1.55375701717094,
-1.55184296172285,-1.54943621994816,-1.5456694924275,-1.52595351827851,
-1.4842401133961,-1.46343816530266,-1.4594035702923,-1.45835777854406),
 .UNSPECIFIED.);
#1274=B_SPLINE_CURVE_WITH_KNOTS('',3,(#40896,#40897,#40898,#40899,#40900,
#40901,#40902,#40903,#40904,#40905,#40906,#40907,#40908,#40909,#40910,#40911,
#40912,#40913,#40914,#40915,#40916,#40917,#40918,#40919,#40920,#40921,#40922,
#40923,#40924,#40925,#40926,#40927,#40928,#40929,#40930,#40931,#40932,#40933,
#40934,#40935,#40936,#40937,#40938,#40939,#40940,#40941,#40942,#40943,#40944,
#40945,#40946,#40947,#40948,#40949,#40950,#40951,#40952,#40953,#40954,#40955,
#40956,#40957,#40958,#40959,#40960,#40961,#40962,#40963,#40964,#40965,#40966,
#40967,#40968,#40969,#40970,#40971,#40972,#40973,#40974,#40975,#40976,#40977,
#40978,#40979,#40980,#40981,#40982,#40983,#40984,#40985,#40986,#40987,#40988,
#40989,#40990,#40991,#40992,#40993,#40994,#40995,#40996,#40997,#40998,#40999,
#41000,#41001,#41002,#41003,#41004,#41005,#41006,#41007,#41008,#41009,#41010,
#41011,#41012,#41013,#41014,#41015,#41016,#41017,#41018,#41019,#41020,#41021,
#41022,#41023,#41024,#41025,#41026,#41027,#41028,#41029,#41030,#41031,#41032,
#41033,#41034,#41035,#41036,#41037,#41038,#41039,#41040,#41041,#41042,#41043,
#41044,#41045,#41046,#41047,#41048,#41049,#41050,#41051,#41052,#41053,#41054,
#41055,#41056,#41057,#41058,#41059,#41060,#41061,#41062,#41063,#41064,#41065,
#41066,#41067,#41068,#41069,#41070,#41071),.UNSPECIFIED.,.F.,.F.,(4,2,2,
2,2,2,2,2,2,2,2,2,2,2,2,2,2,2,2,2,2,2,2,2,2,2,2,2,2,2,2,2,2,2,2,2,2,2,2,
2,2,2,2,2,2,2,2,2,2,2,2,2,2,2,2,2,2,2,2,2,2,2,2,2,2,2,2,2,2,2,2,2,2,2,2,
2,2,2,2,2,2,2,2,2,2,2,2,4),(-0.973977657370886,-0.973066225395767,-0.96462553205897,
-0.949890383429859,-0.946108799913681,-0.943898938423955,-0.941990547568084,
-0.939658230341248,-0.93520175623725,-0.901423061709051,-0.864052893434362,
-0.851119013078597,-0.848884067143519,-0.847503440760412,-0.846431544150649,
-0.845197744158303,-0.843018001083116,-0.833057749166896,-0.811456952073632,
-0.761268981829781,-0.755085959307637,-0.752624381878774,-0.75082112682837,
-0.748874263048361,-0.746231906474935,-0.740152187499536,-0.685673665951278,
-0.65907084035136,-0.656250944266086,-0.654883472690943,-0.65381273992442,
-0.652569931773576,-0.650349158675844,-0.639742052545,-0.615709127911285,
-0.569131526530966,-0.562637200983748,-0.560123747126126,-0.558307036457941,
-0.556368592141944,-0.553777612379373,-0.547988227727931,-0.524071730661645,
-0.491451887208981,-0.466531110152501,-0.463719962171692,-0.462354248606782,
-0.461283703094992,-0.460039749030071,-0.457813582313128,-0.447116515032338,
-0.422727974885078,-0.376658171476533,-0.370130551098277,-0.367611826710242,
-0.365793782987993,-0.363856214310271,-0.361270363610149,-0.355509076252417,
-0.331811084214977,-0.299860253176341,-0.274023829522888,-0.271206733979273,
-0.269839878994731,-0.268769274689338,-0.267526209836558,-0.265303983616606,
-0.254670951810799,-0.230534782273424,-0.184107317859786,-0.177605661939579,
-0.175091146612725,-0.173274250402615,-0.171388887920209,-0.168909579784115,
-0.166151510114064,-0.161541700153478,-0.152000034598465,-0.124139661679705,
-0.0836544184238998,-0.0794162098931193,-0.0777545015696333,-0.076746390053646,
-0.0756434506032181,-0.0740634455314549,-0.0700327318928364,-0.0492720935334833,
-0.000564379274226552),.UNSPECIFIED.);
#1275=B_SPLINE_CURVE_WITH_KNOTS('',3,(#41072,#41073,#41074,#41075,#41076,
#41077,#41078,#41079,#41080,#41081,#41082,#41083,#41084,#41085,#41086,#41087,
#41088,#41089,#41090,#41091,#41092,#41093,#41094,#41095,#41096,#41097,#41098,
#41099,#41100,#41101,#41102,#41103,#41104,#41105,#41106,#41107,#41108,#41109,
#41110,#41111,#41112,#41113,#41114,#41115,#41116,#41117,#41118,#41119,#41120,
#41121,#41122,#41123,#41124,#41125,#41126,#41127,#41128,#41129,#41130,#41131),
 .UNSPECIFIED.,.F.,.F.,(4,2,2,2,2,2,2,2,2,2,2,2,2,2,2,2,2,2,2,2,2,2,2,2,
2,2,2,2,2,4),(-2.43155191913647,-2.42280426928896,-2.41717915570413,-2.41472977602384,
-2.4128483970087,-2.4110144659602,-2.40919597385053,-2.40667538762493,-2.4001357854956,
-2.38765704245933,-2.34967338981676,-2.32867441764294,-2.31888358202122,
-2.31671515539217,-2.31548388580663,-2.31441167645972,-2.31302736228571,
-2.31078000750653,-2.29758812567188,-2.2901962096612,-2.24000035791993,
-2.23033265395902,-2.22567929295,-2.22290341575571,-2.22039871392486,-2.21849988363351,
-2.21668231804465,-2.21416509433217,-2.20764625756361,-2.18940658193359),
 .UNSPECIFIED.);
#1276=B_SPLINE_CURVE_WITH_KNOTS('',3,(#41132,#41133,#41134,#41135,#41136,
#41137,#41138,#41139,#41140,#41141,#41142,#41143,#41144,#41145,#41146,#41147,
#41148,#41149,#41150,#41151,#41152,#41153,#41154,#41155,#41156,#41157,#41158,
#41159,#41160,#41161,#41162,#41163,#41164,#41165,#41166,#41167,#41168,#41169,
#41170,#41171,#41172,#41173,#41174,#41175,#41176,#41177,#41178,#41179,#41180,
#41181,#41182,#41183,#41184,#41185,#41186,#41187,#41188,#41189,#41190,#41191,
#41192,#41193,#41194,#41195,#41196,#41197,#41198,#41199,#41200,#41201,#41202,
#41203,#41204,#41205,#41206,#41207,#41208,#41209,#41210,#41211,#41212,#41213,
#41214,#41215,#41216,#41217,#41218,#41219,#41220,#41221,#41222,#41223,#41224,
#41225,#41226,#41227,#41228,#41229,#41230,#41231,#41232,#41233,#41234,#41235,
#41236,#41237,#41238,#41239,#41240,#41241,#41242,#41243,#41244,#41245,#41246,
#41247,#41248,#41249,#41250,#41251,#41252,#41253,#41254,#41255,#41256,#41257,
#41258,#41259,#41260,#41261,#41262,#41263,#41264,#41265,#41266,#41267,#41268,
#41269,#41270,#41271,#41272,#41273,#41274,#41275,#41276,#41277,#41278,#41279,
#41280,#41281,#41282,#41283,#41284,#41285,#41286,#41287,#41288,#41289,#41290,
#41291,#41292,#41293,#41294,#41295,#41296,#41297,#41298,#41299,#41300,#41301,
#41302,#41303,#41304,#41305,#41306,#41307,#41308,#41309,#41310,#41311,#41312,
#41313,#41314,#41315,#41316,#41317,#41318,#41319,#41320,#41321,#41322,#41323,
#41324,#41325,#41326,#41327,#41328,#41329,#41330,#41331,#41332,#41333,#41334,
#41335,#41336,#41337,#41338,#41339,#41340,#41341,#41342,#41343,#41344,#41345,
#41346,#41347,#41348,#41349),.UNSPECIFIED.,.F.,.F.,(4,2,2,2,2,2,2,2,2,2,
2,2,2,2,2,2,2,2,2,2,2,2,2,2,2,2,2,2,2,2,2,2,2,2,2,2,2,2,2,2,2,2,2,2,2,2,
2,2,2,2,2,2,2,2,2,2,2,2,2,2,2,2,2,2,2,2,2,2,2,2,2,2,2,2,2,2,2,2,2,2,2,2,
2,2,2,2,2,2,2,2,2,2,2,2,2,2,2,2,2,2,2,2,2,2,2,2,2,2,4),(-1.45835777854406,
-1.45782292134003,-1.45671982849219,-1.45571180378477,-1.45405068696945,
-1.44981633975645,-1.40941409136322,-1.38151665039056,-1.36702465517826,
-1.36338856292279,-1.36123282708679,-1.35931853250336,-1.35690970377132,
-1.35313623226168,-1.33328607259331,-1.2916715978068,-1.27091053315857,
-1.26687992104755,-1.2652998732437,-1.26419688058157,-1.26318870015759,
-1.26152684151105,-1.25728805457661,-1.21645982195293,-1.17610577553567,
-1.17199274716033,-1.16950859901695,-1.16757995187486,-1.1654870523497,
-1.16213518611104,-1.15077524554465,-1.13154304754217,-1.1093393364444,
-1.07653295911687,-1.07377260196959,-1.07241697662387,-1.0713472429167,
-1.07009603487008,-1.06783646579505,-1.05656721586208,-1.00750575847676,
-0.983309320391648,-0.979345735708968,-0.976879356296229,-0.974958817363028,
-0.972836611528421,-0.969351756039008,-0.956625709477781,-0.906395563822677,
-0.899001585570265,-0.883708004291678,-0.881368651676051,-0.879972002196811,
-0.878895586663093,-0.877685788952901,-0.875614827186638,-0.867161218921143,
-0.850539790563458,-0.81262176389978,-0.805139220166297,-0.78985891896541,
-0.78603554928505,-0.783816063930652,-0.781908216251608,-0.779587630864457,
-0.775187516610344,-0.744082816337828,-0.699986725742051,-0.690597403163341,
-0.688376255545713,-0.687119929725613,-0.686050573033518,-0.684701493744927,
-0.681974206919407,-0.652315578287309,-0.600933311411062,-0.594876274383381,
-0.592438712173165,-0.590641471414158,-0.58868996983462,-0.586021344200863,
-0.579790268987491,-0.55227256029989,-0.532096881767296,-0.498876658231994,
-0.496127792706804,-0.494774448438069,-0.493704865817538,-0.492451924507258,
-0.490184417884345,-0.478774147393955,-0.428145293785074,-0.405566535049798,
-0.401655738212274,-0.399205269930749,-0.397286622876708,-0.395155746347279,
-0.391631723900853,-0.378471888084394,-0.328593100266154,-0.319666177026502,
-0.30594849068588,-0.303673254608417,-0.302295404604407,-0.301221344249222,
-0.300000385996226,-0.297878987119962,-0.288761531407757,-0.242729697819112),
 .UNSPECIFIED.);
#1277=B_SPLINE_CURVE_WITH_KNOTS('',3,(#41354,#41355,#41356,#41357,#41358,
#41359,#41360,#41361,#41362,#41363,#41364,#41365,#41366,#41367,#41368,#41369,
#41370,#41371,#41372,#41373,#41374,#41375,#41376,#41377,#41378,#41379,#41380,
#41381,#41382,#41383,#41384,#41385,#41386,#41387,#41388,#41389,#41390,#41391,
#41392,#41393,#41394,#41395,#41396,#41397,#41398,#41399,#41400,#41401,#41402,
#41403,#41404,#41405,#41406,#41407,#41408,#41409,#41410,#41411,#41412,#41413,
#41414,#41415,#41416,#41417,#41418,#41419,#41420,#41421,#41422,#41423,#41424,
#41425,#41426,#41427,#41428,#41429,#41430,#41431,#41432,#41433,#41434,#41435,
#41436,#41437,#41438,#41439,#41440,#41441,#41442,#41443,#41444,#41445,#41446,
#41447,#41448,#41449,#41450,#41451,#41452,#41453,#41454,#41455,#41456,#41457,
#41458,#41459,#41460,#41461,#41462,#41463,#41464,#41465,#41466,#41467,#41468,
#41469,#41470,#41471,#41472,#41473,#41474,#41475,#41476,#41477,#41478,#41479,
#41480,#41481,#41482,#41483,#41484,#41485,#41486,#41487,#41488,#41489,#41490,
#41491,#41492,#41493,#41494,#41495,#41496,#41497,#41498,#41499,#41500,#41501,
#41502,#41503,#41504,#41505,#41506,#41507,#41508,#41509,#41510,#41511,#41512,
#41513,#41514,#41515,#41516,#41517,#41518,#41519,#41520,#41521,#41522,#41523,
#41524,#41525,#41526,#41527,#41528,#41529,#41530,#41531,#41532,#41533,#41534,
#41535,#41536,#41537,#41538,#41539,#41540,#41541,#41542,#41543,#41544,#41545,
#41546,#41547,#41548,#41549,#41550,#41551,#41552,#41553,#41554,#41555,#41556,
#41557,#41558,#41559,#41560,#41561),.UNSPECIFIED.,.F.,.F.,(4,2,2,2,2,2,
2,2,2,2,2,2,2,2,2,2,2,2,2,2,2,2,2,2,2,2,2,2,2,2,2,2,2,2,2,2,2,2,2,2,2,2,
2,2,2,2,2,2,2,2,2,2,2,2,2,2,2,2,2,2,2,2,2,2,2,2,2,2,2,2,2,2,2,2,2,2,2,2,
2,2,2,2,2,2,2,2,2,2,2,2,2,2,2,2,2,2,2,2,2,2,2,2,2,4),(-2.18956623962693,
-2.18041265317692,-2.13479112283698,-2.11558000051423,-2.10806267563156,
-2.10249362892436,-2.09991061012686,-2.09797378248252,-2.09615542362863,
-2.09363465227258,-2.08709241093975,-2.04127798422216,-2.01668662835424,
-2.00593999991555,-2.00371111203506,-2.00246670807316,-2.0013964405585,
-2.00003195016963,-1.99722622749472,-1.97285484915736,-1.92360185617187,
-1.91179798530528,-1.90840165225533,-1.90629924087623,-1.90437402379684,
-1.90191113941125,-1.89786939745731,-1.87097988132194,-1.82227944897952,
-1.81320701320005,-1.81108907851394,-1.80986899017584,-1.80879493893445,
-1.80741614584906,-1.80513739766206,-1.7913846509769,-1.78245491750448,
-1.73248156176817,-1.71948358905235,-1.71597432518676,-1.71384687906953,
-1.71192779210242,-1.70947187810071,-1.70554249779532,-1.68249449319403,
-1.6323005931622,-1.62092793367482,-1.61866262219051,-1.61741022173571,
-1.61634068419027,-1.61498687122962,-1.61223532245761,-1.57918186518307,
-1.55384116306093,-1.53060519866613,-1.52490326666873,-1.52232822463779,
-1.52039240101882,-1.51857134679561,-1.51604102130604,-1.50943936924016,
-1.46469168750852,-1.43029296130569,-1.42682568940314,-1.42533842521348,
-1.42425221684062,-1.42307425013789,-1.42114633521858,-1.41500392814279,
-1.36095873132179,-1.33797549667318,-1.33230655794222,-1.32973757283408,
-1.32780273420643,-1.32597998967863,-1.32344311596424,-1.3167986002539,
-1.2729999316692,-1.24692916359499,-1.23582081263044,-1.23357045616619,
-1.23232128218876,-1.23125138826584,-1.22989312832399,-1.2277321321533,
-1.21620561414111,-1.16169534723097,-1.14295010261025,-1.1392392790364,
-1.13684979219599,-1.1349375347666,-1.13276982262447,-1.12907855463261,
-1.1138696923037,-1.05923312898293,-1.04382162424118,-1.04147786111809,
-1.04007993791724,-1.0390033692011,-1.03779432903114,-1.03572672259374,
-1.02731503206474,-1.01082014887421,-0.973977657370886),.UNSPECIFIED.);
#1278=B_SPLINE_CURVE_WITH_KNOTS('',3,(#41563,#41564,#41565,#41566,#41567,
#41568,#41569,#41570,#41571,#41572,#41573,#41574,#41575,#41576,#41577,#41578,
#41579,#41580,#41581,#41582,#41583,#41584,#41585,#41586,#41587,#41588,#41589,
#41590,#41591,#41592,#41593,#41594,#41595,#41596,#41597,#41598,#41599,#41600,
#41601,#41602,#41603,#41604,#41605,#41606,#41607,#41608,#41609,#41610,#41611,
#41612,#41613,#41614,#41615,#41616),.UNSPECIFIED.,.F.,.F.,(4,2,2,2,2,2,
2,2,2,2,2,2,2,2,2,2,2,2,2,2,2,2,2,2,2,2,4),(-0.242729697819112,-0.240116437798231,
-0.213250307360193,-0.209206621585435,-0.206742923171201,-0.204871176334209,
-0.202830447661773,-0.200707670511219,-0.197631835711563,-0.192234493795022,
-0.152249128627421,-0.116231805408894,-0.111837027572666,-0.11014999390269,
-0.109137008829852,-0.108038232994759,-0.106480058163093,-0.102587620031566,
-0.0832020359993201,-0.0292996200280103,-0.0187066474130954,-0.0153142652421365,
-0.0132125172705519,-0.0113620376163737,-0.00949737249079776,-0.00709833961708263,
-0.000563576427226659),.UNSPECIFIED.);
#1279=B_SPLINE_CURVE_WITH_KNOTS('',3,(#41617,#41618,#41619,#41620,#41621,
#41622,#41623,#41624,#41625,#41626,#41627,#41628,#41629,#41630,#41631,#41632,
#41633,#41634,#41635,#41636,#41637,#41638,#41639,#41640,#41641,#41642,#41643,
#41644,#41645,#41646,#41647,#41648,#41649,#41650,#41651,#41652,#41653,#41654,
#41655,#41656,#41657,#41658,#41659,#41660,#41661,#41662,#41663,#41664,#41665,
#41666,#41667,#41668,#41669,#41670,#41671,#41672,#41673,#41674,#41675,#41676,
#41677,#41678,#41679,#41680,#41681,#41682,#41683,#41684,#41685,#41686,#41687,
#41688,#41689,#41690,#41691,#41692,#41693,#41694,#41695,#41696,#41697,#41698,
#41699,#41700,#41701,#41702,#41703,#41704,#41705,#41706,#41707,#41708,#41709,
#41710,#41711,#41712,#41713,#41714,#41715,#41716,#41717,#41718,#41719,#41720,
#41721,#41722,#41723,#41724,#41725,#41726,#41727,#41728,#41729,#41730,#41731,
#41732,#41733,#41734,#41735,#41736,#41737,#41738,#41739,#41740,#41741,#41742,
#41743,#41744,#41745,#41746,#41747,#41748,#41749,#41750,#41751,#41752,#41753,
#41754,#41755,#41756,#41757,#41758,#41759,#41760,#41761,#41762,#41763,#41764,
#41765,#41766,#41767,#41768,#41769,#41770,#41771,#41772,#41773,#41774,#41775,
#41776,#41777,#41778,#41779,#41780,#41781,#41782,#41783,#41784,#41785,#41786,
#41787,#41788,#41789,#41790,#41791,#41792),.UNSPECIFIED.,.F.,.F.,(4,2,2,
2,2,2,2,2,2,2,2,2,2,2,2,2,2,2,2,2,2,2,2,2,2,2,2,2,2,2,2,2,2,2,2,2,2,2,2,
2,2,2,2,2,2,2,2,2,2,2,2,2,2,2,2,2,2,2,2,2,2,2,2,2,2,2,2,2,2,2,2,2,2,2,2,
2,2,2,2,2,2,2,2,2,2,2,2,4),(-2.43098705841732,-2.37325618589629,-2.35138393235581,
-2.34875985260428,-2.34743194285922,-2.34646736735063,-2.3452364712295,
-2.34312480058049,-2.33501171342135,-2.27302956465628,-2.26259037357187,
-2.25767556453552,-2.25479368631527,-2.25228619365899,-2.25038948750831,
-2.24860670909135,-2.2457786052043,-2.23907951341181,-2.19696091665691,
-2.18432879521766,-2.16671728089558,-2.15794472848786,-2.15584958042758,
-2.15463474084651,-2.15356000158624,-2.15217348935786,-2.14986779371891,
-2.13540917988652,-2.13123953293945,-2.09601883338496,-2.07583864161764,
-2.06409693795727,-2.06070716390939,-2.05860642407425,-2.05668114419651,
-2.05421598368269,-2.05016581307431,-2.02329630499217,-1.97460122937902,
-1.96553340523322,-1.96341604761062,-1.96219621060087,-1.96112232655666,
-1.95974367908389,-1.95746502960675,-1.94363919822089,-1.93474313249465,
-1.88468173806665,-1.87180449230982,-1.86830651259571,-1.8661817859668,
-1.86426249635717,-1.86180263470978,-1.85785946586743,-1.834341149538,-1.7846128941192,
-1.77328309330995,-1.77102045824447,-1.76976876684499,-1.76869936167858,
-1.76734511062723,-1.76459068609666,-1.73166584694355,-1.70655132012922,
-1.68303418847249,-1.67729631933894,-1.67471501209352,-1.67277846273196,
-1.67095963252408,-1.66843703924917,-1.66188321649084,-1.61625853492399,
-1.59153190985087,-1.58075152837653,-1.57852062830689,-1.57727579023372,
-1.57620558036129,-1.57484172014555,-1.57203916236646,-1.54800005779068,
-1.49855239847719,-1.48662910198961,-1.48322097845794,-1.48111597163792,
-1.479191501112,-1.47673385895048,-1.47270984440081,-1.45772415786055),
 .UNSPECIFIED.);
#1280=B_SPLINE_CURVE_WITH_KNOTS('',3,(#41798,#41799,#41800,#41801,#41802,
#41803,#41804,#41805,#41806,#41807,#41808,#41809,#41810,#41811,#41812,#41813,
#41814,#41815,#41816,#41817,#41818,#41819,#41820,#41821,#41822,#41823,#41824,
#41825,#41826,#41827,#41828,#41829,#41830,#41831,#41832,#41833,#41834,#41835,
#41836,#41837,#41838,#41839,#41840,#41841,#41842,#41843,#41844,#41845,#41846,
#41847,#41848,#41849,#41850,#41851,#41852,#41853,#41854,#41855,#41856,#41857,
#41858,#41859,#41860,#41861,#41862,#41863,#41864,#41865,#41866,#41867,#41868,
#41869,#41870,#41871,#41872,#41873,#41874,#41875,#41876,#41877,#41878,#41879,
#41880,#41881,#41882,#41883,#41884,#41885,#41886,#41887,#41888,#41889,#41890,
#41891,#41892,#41893,#41894,#41895,#41896,#41897,#41898,#41899,#41900,#41901,
#41902,#41903,#41904,#41905,#41906,#41907,#41908,#41909,#41910,#41911,#41912,
#41913,#41914,#41915,#41916,#41917,#41918,#41919,#41920,#41921,#41922,#41923,
#41924,#41925,#41926,#41927,#41928,#41929,#41930,#41931,#41932,#41933,#41934,
#41935,#41936,#41937,#41938,#41939,#41940,#41941,#41942,#41943,#41944,#41945,
#41946,#41947,#41948,#41949,#41950,#41951,#41952,#41953,#41954,#41955,#41956,
#41957,#41958,#41959,#41960,#41961,#41962,#41963,#41964,#41965,#41966,#41967,
#41968,#41969,#41970,#41971,#41972,#41973,#41974,#41975,#41976,#41977,#41978,
#41979),.UNSPECIFIED.,.F.,.F.,(4,2,2,2,2,2,2,2,2,2,2,2,2,2,2,2,2,2,2,2,
2,2,2,2,2,2,2,2,2,2,2,2,2,2,2,2,2,2,2,2,2,2,2,2,2,2,2,2,2,2,2,2,2,2,2,2,
2,2,2,2,2,2,2,2,2,2,2,2,2,2,2,2,2,2,2,2,2,2,2,2,2,2,2,2,2,2,2,2,2,2,4),
(-0.97400982262004,-0.939077207573621,-0.923181086866272,-0.920592913881418,
-0.919255111714498,-0.918186661183434,-0.916921971078261,-0.914599507770575,
-0.902139044537373,-0.869753821135637,-0.830541542481921,-0.826400310588078,
-0.823908117647993,-0.821978531220479,-0.819889906012371,-0.816556386446665,
-0.805369159224853,-0.786555882087239,-0.745091495181054,-0.730596384167335,
-0.728288657443566,-0.726901365223826,-0.725826291228361,-0.724611365664025,
-0.722516746509033,-0.713755870225364,-0.696186004762857,-0.666729273318793,
-0.637976146905596,-0.633889137744435,-0.631412792417983,-0.629485492526718,
-0.6273893194661,-0.624021829572349,-0.612506891380457,-0.592891960217706,
-0.551826433120587,-0.538073516635675,-0.535794992344142,-0.534416253167552,
-0.533342189652874,-0.532122013407345,-0.530003774144425,-0.520927345024398,
-0.472255137139017,-0.445376108802911,-0.441334664061433,-0.438871769675417,
-0.436946441493308,-0.434843804970809,-0.431446879756632,-0.419638807746116,
-0.370357049030402,-0.345974416967848,-0.343168126153214,-0.341803450348783,
-0.340733084123659,-0.339488610814658,-0.337259724835709,-0.326514921370215,
-0.301934525120386,-0.256146755451947,-0.249599617232489,-0.247077940087878,
-0.245259234433548,-0.243322321543413,-0.240739686153191,-0.235184684216764,
-0.22768443090503,-0.208537529894372,-0.176131543099938,-0.169617438007437,
-0.153220540271922,-0.150613800178691,-0.149271979345731,-0.148203282914577,
-0.146941770713721,-0.145599792217739,-0.140316164913045,-0.117843485008567,
-0.0976712951451026,-0.0872716329576706,-0.0603973523829484,-0.0563558450857691,
-0.0538928630504517,-0.051967436578634,-0.0498646624896345,-0.0477046383277412,
-0.0445379818388593,-0.0338137111492761,-0.000563923203056516),
 .UNSPECIFIED.);
#1281=B_SPLINE_CURVE_WITH_KNOTS('',3,(#41980,#41981,#41982,#41983,#41984,
#41985,#41986,#41987,#41988,#41989,#41990,#41991,#41992,#41993,#41994,#41995,
#41996,#41997,#41998,#41999,#42000,#42001,#42002,#42003,#42004,#42005,#42006,
#42007,#42008,#42009,#42010,#42011,#42012,#42013,#42014,#42015,#42016,#42017,
#42018,#42019,#42020,#42021,#42022,#42023,#42024,#42025,#42026,#42027,#42028,
#42029,#42030,#42031,#42032,#42033,#42034,#42035),.UNSPECIFIED.,.F.,.F.,
(4,2,2,2,2,2,2,2,2,2,2,2,2,2,2,2,2,2,2,2,2,2,2,2,2,2,2,4),(-2.43140076039871,
-2.39440475956086,-2.39129067200828,-2.38954019459536,-2.38799018084422,
-2.38689320294571,-2.38587875790501,-2.38418299704171,-2.37972988241132,
-2.34792437241353,-2.32909866248134,-2.30836358721486,-2.29682048211597,
-2.29431824636313,-2.29197312934567,-2.29006450344343,-2.28786578274992,
-2.28413092789478,-2.26987859822957,-2.26054060536068,-2.20991829103546,
-2.19852196334369,-2.19629771777738,-2.1950285003781,-2.19396036929867,
-2.1926281795813,-2.19055224883826,-2.18956623962693),.UNSPECIFIED.);
#1282=B_SPLINE_CURVE_WITH_KNOTS('',3,(#42036,#42037,#42038,#42039,#42040,
#42041,#42042,#42043,#42044,#42045,#42046,#42047,#42048,#42049,#42050,#42051,
#42052,#42053,#42054,#42055,#42056,#42057,#42058,#42059,#42060,#42061,#42062,
#42063,#42064,#42065,#42066,#42067,#42068,#42069,#42070,#42071,#42072,#42073,
#42074,#42075,#42076,#42077,#42078,#42079,#42080,#42081,#42082,#42083,#42084,
#42085,#42086,#42087,#42088,#42089,#42090,#42091,#42092,#42093,#42094,#42095,
#42096,#42097,#42098,#42099,#42100,#42101,#42102,#42103,#42104,#42105,#42106,
#42107,#42108,#42109,#42110,#42111,#42112,#42113,#42114,#42115,#42116,#42117,
#42118,#42119,#42120,#42121,#42122,#42123,#42124,#42125,#42126,#42127,#42128,
#42129,#42130,#42131,#42132,#42133,#42134,#42135,#42136,#42137,#42138,#42139,
#42140,#42141,#42142,#42143,#42144,#42145,#42146,#42147,#42148,#42149,#42150,
#42151,#42152,#42153,#42154,#42155,#42156,#42157,#42158,#42159,#42160,#42161,
#42162,#42163,#42164,#42165,#42166,#42167,#42168,#42169,#42170,#42171,#42172,
#42173,#42174,#42175,#42176,#42177,#42178,#42179,#42180,#42181,#42182,#42183,
#42184,#42185,#42186,#42187,#42188,#42189,#42190,#42191,#42192,#42193,#42194,
#42195,#42196,#42197,#42198,#42199,#42200,#42201,#42202,#42203,#42204,#42205,
#42206,#42207,#42208,#42209,#42210,#42211,#42212,#42213,#42214,#42215,#42216,
#42217,#42218,#42219,#42220,#42221,#42222,#42223,#42224,#42225,#42226,#42227,
#42228,#42229,#42230,#42231,#42232,#42233,#42234,#42235,#42236,#42237,#42238,
#42239,#42240,#42241,#42242,#42243,#42244,#42245,#42246,#42247,#42248,#42249,
#42250,#42251),.UNSPECIFIED.,.F.,.F.,(4,2,2,2,2,2,2,2,2,2,2,2,2,2,2,2,2,
2,2,2,2,2,2,2,2,2,2,2,2,2,2,2,2,2,2,2,2,2,2,2,2,2,2,2,2,2,2,2,2,2,2,2,2,
2,2,2,2,2,2,2,2,2,2,2,2,2,2,2,2,2,2,2,2,2,2,2,2,2,2,2,2,2,2,2,2,2,2,2,2,
2,2,2,2,2,2,2,2,2,2,2,2,2,2,2,2,2,2,4),(-1.45772415786055,-1.44648434475585,
-1.43513039397568,-1.40967403196687,-1.39074676278327,-1.38690250508643,
-1.38535233027771,-1.38425527651423,-1.38324079143602,-1.38154502484505,
-1.37709224739574,-1.3449684202107,-1.31108999243359,-1.29486807041862,
-1.29110383623707,-1.28892025104236,-1.28701015439179,-1.28464439998024,
-1.28101018914932,-1.26346220473926,-1.2155886220444,-1.21093664919579,
-1.19636012794277,-1.19404918426374,-1.1926609905796,-1.19158585557495,
-1.1903715819739,-1.1882797105454,-1.17955374255117,-1.1315309774056,-1.1036593126324,
-1.09959323249244,-1.09712319924799,-1.09519700462702,-1.09309819062394,
-1.08971798837394,-1.07807494897275,-1.05814031916614,-1.04074491082258,
-1.00670630617543,-1.00227142637631,-1.00057839813368,-0.999564432201041,
-0.998466938314348,-0.996914481307998,-0.993056149466106,-0.973996176335221,
-0.948646457345167,-0.937299141324565,-0.911151612309999,-0.907129967764425,
-0.904672987294396,-0.902748572346378,-0.900643156020368,-0.897233322069521,
-0.885293358341514,-0.835797164451535,-0.81178497768871,-0.808982338963741,
-0.807618426931977,-0.806548173500303,-0.805303273309203,-0.803072247896647,
-0.792290346122666,-0.7675604210291,-0.721978599471011,-0.715424152550581,
-0.712901398121786,-0.711082469351578,-0.709145831571899,-0.706564443645755,
-0.700826566101351,-0.677307378585801,-0.652167948477815,-0.619222189382195,
-0.616467190145176,-0.615112764116153,-0.614043276000622,-0.612791544283018,
-0.610528992148389,-0.599202139297834,-0.549499317175386,-0.525982640659287,
-0.522039541800048,-0.519579543467754,-0.517660048940116,-0.515534994928404,
-0.512036246785498,-0.499153791500606,-0.449062050911271,-0.440125765073548,
-0.426324651551249,-0.424046827146197,-0.42266833520035,-0.421594353973553,
-0.420374145751427,-0.418255563646169,-0.409173297016571,-0.360509019333671,
-0.33363333921505,-0.329592172348819,-0.327129433694186,-0.325204219123834,
-0.323101698460661,-0.319704942270411,-0.308665781953824,-0.289895743865608,
-0.242394817054379),.UNSPECIFIED.);
#1283=B_SPLINE_CURVE_WITH_KNOTS('',3,(#42256,#42257,#42258,#42259,#42260,
#42261,#42262,#42263,#42264,#42265,#42266,#42267,#42268,#42269,#42270,#42271,
#42272,#42273,#42274,#42275,#42276,#42277,#42278,#42279,#42280,#42281,#42282,
#42283,#42284,#42285,#42286,#42287,#42288,#42289,#42290,#42291,#42292,#42293,
#42294,#42295,#42296,#42297,#42298,#42299,#42300,#42301,#42302,#42303,#42304,
#42305,#42306,#42307,#42308,#42309,#42310,#42311,#42312,#42313,#42314,#42315,
#42316,#42317,#42318,#42319,#42320,#42321,#42322,#42323,#42324,#42325,#42326,
#42327,#42328,#42329,#42330,#42331,#42332,#42333,#42334,#42335,#42336,#42337,
#42338,#42339,#42340,#42341,#42342,#42343,#42344,#42345,#42346,#42347,#42348,
#42349,#42350,#42351,#42352,#42353,#42354,#42355,#42356,#42357,#42358,#42359,
#42360,#42361,#42362,#42363,#42364,#42365,#42366,#42367,#42368,#42369,#42370,
#42371,#42372,#42373,#42374,#42375,#42376,#42377,#42378,#42379,#42380,#42381,
#42382,#42383,#42384,#42385,#42386,#42387,#42388,#42389,#42390,#42391,#42392,
#42393,#42394,#42395,#42396,#42397,#42398,#42399,#42400,#42401,#42402,#42403,
#42404,#42405,#42406,#42407,#42408,#42409,#42410,#42411,#42412,#42413,#42414,
#42415,#42416,#42417,#42418,#42419,#42420,#42421,#42422,#42423,#42424,#42425,
#42426,#42427,#42428,#42429,#42430,#42431,#42432,#42433,#42434,#42435,#42436,
#42437,#42438,#42439,#42440,#42441,#42442,#42443,#42444,#42445,#42446,#42447,
#42448,#42449,#42450,#42451,#42452,#42453,#42454,#42455,#42456,#42457,#42458,
#42459,#42460,#42461,#42462,#42463,#42464,#42465,#42466,#42467,#42468,#42469,
#42470,#42471,#42472,#42473,#42474,#42475,#42476,#42477,#42478,#42479,#42480,
#42481,#42482,#42483),.UNSPECIFIED.,.F.,.F.,(4,2,2,2,2,2,2,2,2,2,2,2,2,
2,2,2,2,2,2,2,2,2,2,2,2,2,2,2,2,2,2,2,2,2,2,2,2,2,2,2,2,2,2,2,2,2,2,2,2,
2,2,2,2,2,2,2,2,2,2,2,2,2,2,2,2,2,2,2,2,2,2,2,2,2,2,2,2,2,2,2,2,2,2,2,2,
2,2,2,2,2,2,2,2,2,2,2,2,2,2,2,2,2,2,2,2,2,2,2,2,2,2,2,2,4),(-2.18931141726403,
-2.17971667832203,-2.1740160498697,-2.17144169112358,-2.16950641917689,
-2.16768591172043,-2.16515639046521,-2.15855710585837,-2.11381318737296,
-2.08845504588565,-2.07751962371634,-2.07527973837221,-2.07403303835293,
-2.07296319011424,-2.07160231875026,-2.06881434908441,-2.04651619031018,
-1.99647970394439,-1.98357334229189,-1.98007276618586,-1.97794748921928,
-1.97602836410324,-1.97356963236718,-1.96963013729441,-1.94623392849253,
-1.89638959941177,-1.88504946072947,-1.88278627299703,-1.88153447453714,
-1.88046509985247,-1.87911104334982,-1.87635752577091,-1.84340404869804,
-1.81823856230869,-1.79478852897057,-1.78905936872617,-1.78647966632284,
-1.78454339589489,-1.78272415279415,-1.78019990948715,-1.77363543732423,
-1.72820385303824,-1.70333934205701,-1.69252478179074,-1.69029187121616,
-1.68904660853373,-1.68797646898426,-1.68661326000842,-1.68381392304517,
-1.66009019981957,-1.62676371955206,-1.60247045374809,-1.5966332703778,
-1.59403400930359,-1.59209453001447,-1.59028057654964,-1.58777683567353,
-1.581340693591,-1.53394559694203,-1.51046266617043,-1.49999852998953,-1.49778680719362,
-1.49654611858245,-1.49547534836201,-1.49410542088859,-1.49190568130833,
-1.47966149467538,-1.47672048794915,-1.4356436480993,-1.41692899715293,
-1.40578127281034,-1.40245184674131,-1.40036407711228,-1.39843411649277,
-1.39593980305544,-1.3917914385534,-1.35985865087689,-1.35502115868795,
-1.33287401204694,-1.31050544791138,-1.30632060236034,-1.30471701458361,
-1.30360952762794,-1.30260636232229,-1.30097041016749,-1.29688593766107,
-1.25474407604486,-1.21610189115401,-1.21116629859234,-1.20873697248221,
-1.20682091850222,-1.20467841387701,-1.20110095985851,-1.18731908359201,
-1.13793039812803,-1.1297063610522,-1.12806946511162,-1.11543397322218,
-1.11321409396405,-1.11183809978535,-1.11076678014907,-1.10953021389148,
-1.10733735324484,-1.09717180774499,-1.07481837312228,-1.02579318475135,
-1.01949783413441,-1.01701745831222,-1.0152095509318,-1.01326628957882,
-1.01064402995532,-1.00467757573562,-0.979348183379391,-0.97400982262004),
 .UNSPECIFIED.);
#1284=B_SPLINE_CURVE_WITH_KNOTS('',3,(#42485,#42486,#42487,#42488,#42489,
#42490,#42491,#42492,#42493,#42494,#42495,#42496,#42497,#42498,#42499,#42500,
#42501,#42502,#42503,#42504,#42505,#42506,#42507,#42508,#42509,#42510,#42511,
#42512,#42513,#42514,#42515,#42516,#42517,#42518,#42519,#42520,#42521,#42522,
#42523,#42524,#42525,#42526,#42527,#42528,#42529,#42530,#42531,#42532,#42533,
#42534,#42535,#42536,#42537,#42538,#42539,#42540),.UNSPECIFIED.,.F.,.F.,
(4,2,2,2,2,2,2,2,2,2,2,2,2,2,2,2,2,2,2,2,2,2,2,2,2,2,2,4),(-0.242394817054379,
-0.239477933129532,-0.232834969013898,-0.230848793020402,-0.229657925746363,
-0.228576461818301,-0.227148180620264,-0.224012380099846,-0.21970251570913,
-0.208538470225524,-0.176092779368492,-0.141350239810987,-0.137184531408027,
-0.134685091467156,-0.132754290951723,-0.130668717402813,-0.1273494967973,
-0.116541451371545,-0.0910614130852629,-0.0701399243704446,-0.0417834508299576,
-0.0389659377043969,-0.0375990719874846,-0.0365285510021365,-0.035285688115564,
-0.0339701702088994,-0.0319313914060394,-0.000563637760111814),
 .UNSPECIFIED.);
#1285=B_SPLINE_CURVE_WITH_KNOTS('',3,(#42541,#42542,#42543,#42544,#42545,
#42546,#42547,#42548,#42549,#42550,#42551,#42552,#42553,#42554,#42555,#42556,
#42557,#42558,#42559,#42560,#42561,#42562,#42563,#42564,#42565,#42566,#42567,
#42568,#42569,#42570,#42571,#42572,#42573,#42574,#42575,#42576,#42577,#42578,
#42579,#42580,#42581,#42582,#42583,#42584,#42585,#42586,#42587,#42588,#42589,
#42590,#42591,#42592,#42593,#42594,#42595,#42596,#42597,#42598,#42599,#42600,
#42601,#42602,#42603,#42604,#42605,#42606,#42607,#42608,#42609,#42610,#42611,
#42612,#42613,#42614,#42615,#42616,#42617,#42618,#42619,#42620,#42621,#42622,
#42623,#42624,#42625,#42626,#42627,#42628,#42629,#42630,#42631,#42632,#42633,
#42634,#42635,#42636,#42637,#42638,#42639,#42640,#42641,#42642,#42643,#42644,
#42645,#42646,#42647,#42648,#42649,#42650,#42651,#42652,#42653,#42654,#42655,
#42656,#42657,#42658,#42659,#42660,#42661,#42662,#42663,#42664,#42665,#42666,
#42667,#42668,#42669,#42670,#42671,#42672,#42673,#42674,#42675,#42676,#42677,
#42678,#42679,#42680,#42681,#42682,#42683,#42684,#42685,#42686,#42687,#42688,
#42689,#42690,#42691,#42692,#42693,#42694,#42695,#42696,#42697,#42698,#42699,
#42700,#42701,#42702,#42703,#42704,#42705,#42706,#42707,#42708,#42709,#42710,
#42711,#42712,#42713,#42714,#42715,#42716,#42717,#42718,#42719,#42720),
 .UNSPECIFIED.,.F.,.F.,(4,2,2,2,2,2,2,2,2,2,2,2,2,2,2,2,2,2,2,2,2,2,2,2,
2,2,2,2,2,2,2,2,2,2,2,2,2,2,2,2,2,2,2,2,2,2,2,2,2,2,2,2,2,2,2,2,2,2,2,2,
2,2,2,2,2,2,2,2,2,2,2,2,2,2,2,2,2,2,2,2,2,2,2,2,2,2,2,2,2,4),(-2.43111332147802,
-2.38917177521858,-2.37884381470538,-2.37580751112802,-2.37308011772945,
-2.37111920558706,-2.36933623067966,-2.36650413856717,-2.35976992812447,
-2.32022875543692,-2.29877245339659,-2.28568114122789,-2.27850715033665,
-2.27654687080474,-2.27553356051292,-2.27446559778252,-2.2731247373101,
-2.27051997682063,-2.25413707293724,-2.21586026107291,-2.19633288980105,
-2.18488724238658,-2.18150859397224,-2.17941088462658,-2.17748579658507,
-2.17501730932659,-2.17095401451103,-2.14312784627585,-2.09507485649955,
-2.08634084768317,-2.0842490787659,-2.08303521959261,-2.08196068488694,
-2.08057358187924,-2.07826512068986,-2.06372609292791,-2.06029014083134,
-2.02810348766952,-1.99442956914285,-1.98997799626856,-1.98764768423892,
-1.98575840755453,-1.98355640874775,-1.97980490657129,-1.96535729195556,
-1.95637900899021,-1.9187883770378,-1.9023298071914,-1.89393293524496,-1.89186744927816,
-1.89065939691659,-1.88958352682837,-1.88818629131251,-1.8858432234415,
-1.87041570169094,-1.83244271815857,-1.80480911101898,-1.79856606812766,
-1.79589652110466,-1.7939458995574,-1.79215054933956,-1.7892510245597,-1.78210809499121,
-1.78069897318267,-1.7142709818317,-1.70188807520945,-1.6995699185117,-1.6983063758211,
-1.69723817732583,-1.69589979053953,-1.69330788042781,-1.67729613578746,
-1.67070292700316,-1.62055405819952,-1.60779490314547,-1.60430804402985,
-1.60218598415125,-1.60026646040368,-1.59780261663732,-1.59384557993601,
-1.56983497879135,-1.52059092707837,-1.50930636683371,-1.50704653351831,
-1.50579556926187,-1.50472627945938,-1.50337152633243,-1.50061395219292,
-1.48014739334638,-1.45804903820686),.UNSPECIFIED.);
#1286=B_SPLINE_CURVE_WITH_KNOTS('',3,(#42726,#42727,#42728,#42729,#42730,
#42731,#42732,#42733,#42734,#42735,#42736,#42737,#42738,#42739,#42740,#42741,
#42742,#42743,#42744,#42745,#42746,#42747,#42748,#42749,#42750,#42751,#42752,
#42753,#42754,#42755,#42756,#42757,#42758,#42759,#42760,#42761,#42762,#42763,
#42764,#42765,#42766,#42767,#42768,#42769,#42770,#42771,#42772,#42773,#42774,
#42775,#42776,#42777,#42778,#42779,#42780,#42781,#42782,#42783,#42784,#42785,
#42786,#42787,#42788,#42789,#42790,#42791,#42792,#42793,#42794,#42795,#42796,
#42797,#42798,#42799,#42800,#42801,#42802,#42803,#42804,#42805,#42806,#42807,
#42808,#42809,#42810,#42811,#42812,#42813,#42814,#42815,#42816,#42817,#42818,
#42819,#42820,#42821,#42822,#42823,#42824,#42825,#42826,#42827,#42828,#42829,
#42830,#42831,#42832,#42833,#42834,#42835,#42836,#42837,#42838,#42839,#42840,
#42841,#42842,#42843,#42844,#42845,#42846,#42847,#42848,#42849,#42850,#42851,
#42852,#42853,#42854,#42855,#42856,#42857,#42858,#42859,#42860,#42861,#42862,
#42863,#42864,#42865,#42866,#42867,#42868,#42869,#42870,#42871,#42872,#42873,
#42874,#42875,#42876,#42877,#42878,#42879,#42880,#42881,#42882,#42883,#42884,
#42885,#42886,#42887,#42888,#42889,#42890,#42891,#42892,#42893,#42894,#42895,
#42896,#42897,#42898,#42899,#42900,#42901,#42902,#42903,#42904,#42905,#42906,
#42907),.UNSPECIFIED.,.F.,.F.,(4,2,2,2,2,2,2,2,2,2,2,2,2,2,2,2,2,2,2,2,
2,2,2,2,2,2,2,2,2,2,2,2,2,2,2,2,2,2,2,2,2,2,2,2,2,2,2,2,2,2,2,2,2,2,2,2,
2,2,2,2,2,2,2,2,2,2,2,2,2,2,2,2,2,2,2,2,2,2,2,2,2,2,2,2,2,2,2,2,2,2,4),
(-0.973731148246856,-0.951279812783102,-0.905142557312427,-0.898619654373167,
-0.896101639113266,-0.894283747865263,-0.892346008287853,-0.889759355501773,
-0.883993872523863,-0.86026380526683,-0.828197165487885,-0.802510932731893,
-0.799694562950635,-0.798327827824749,-0.797257206352008,-0.79601399436364,
-0.793791193224789,-0.783149442324522,-0.758979449522965,-0.712600691950234,
-0.706093629737283,-0.703578205223135,-0.701761038045641,-0.699823005805383,
-0.697234127711926,-0.691455971181448,-0.667626182897352,-0.635234174815842,
-0.609990764968893,-0.607177324877824,-0.605811199954283,-0.604740668152728,
-0.603497115284924,-0.601272612648773,-0.590601759538253,-0.566316174829597,
-0.520104127674435,-0.513586693973118,-0.511069668712476,-0.509252128619224,
-0.507314425935313,-0.504727241235337,-0.498958132026518,-0.475198112371053,
-0.443023778988662,-0.417481873302499,-0.414669410318262,-0.413303510126237,
-0.412233034873776,-0.410989410663569,-0.408764443935391,-0.39808489115552,
-0.373764168679482,-0.327604860820988,-0.321084461622554,-0.318567021058041,
-0.316749417787192,-0.314811867403475,-0.31222526435995,-0.306459040839527,
-0.282720685501049,-0.248079315716744,-0.224952367324629,-0.22215746487591,
-0.220795062430265,-0.219724907147974,-0.218503915405194,-0.216363456341239,
-0.21369578096127,-0.208053508523378,-0.191338861194781,-0.154619482139047,
-0.131651989982077,-0.127725350969118,-0.125270166743044,-0.123351054218838,
-0.121222969280775,-0.117711239986985,-0.104687879315528,-0.0677131483839322,
-0.0520824168507651,-0.0460575312679607,-0.03206964115021,-0.0297834579716761,
-0.0284024794595397,-0.0273281666610978,-0.0263227736782593,-0.0251172576095525,
-0.0233453054434443,-0.0170509377124757,-0.000563395908633966),
 .UNSPECIFIED.);
#1287=B_SPLINE_CURVE_WITH_KNOTS('',3,(#42908,#42909,#42910,#42911,#42912,
#42913,#42914,#42915,#42916,#42917,#42918,#42919,#42920,#42921,#42922,#42923,
#42924,#42925,#42926,#42927,#42928,#42929,#42930,#42931,#42932,#42933,#42934,
#42935,#42936,#42937,#42938,#42939,#42940,#42941,#42942,#42943,#42944,#42945,
#42946,#42947,#42948,#42949,#42950,#42951),.UNSPECIFIED.,.F.,.F.,(4,2,2,
2,2,2,2,2,2,2,2,2,2,2,2,2,2,2,2,2,2,4),(-2.43151735467866,-2.38290482253618,
-2.37358794232629,-2.36693454650074,-2.36419561173252,-2.3622317610133,
-2.36044974366734,-2.35762693889216,-2.35095445542579,-2.30791896744605,
-2.28692218296531,-2.27580139030319,-2.27150343763058,-2.26838780436255,
-2.26695602206332,-2.26587417418831,-2.26468527150582,-2.26270735505003,
-2.25613545544025,-2.25465941024578,-2.20294860238536,-2.18931141726403),
 .UNSPECIFIED.);
#1288=B_SPLINE_CURVE_WITH_KNOTS('',3,(#42952,#42953,#42954,#42955,#42956,
#42957,#42958,#42959,#42960,#42961,#42962,#42963,#42964,#42965,#42966,#42967,
#42968,#42969,#42970,#42971,#42972,#42973,#42974,#42975,#42976,#42977,#42978,
#42979,#42980,#42981,#42982,#42983,#42984,#42985,#42986,#42987,#42988,#42989,
#42990,#42991,#42992,#42993,#42994,#42995,#42996,#42997,#42998,#42999,#43000,
#43001,#43002,#43003,#43004,#43005,#43006,#43007,#43008,#43009,#43010,#43011,
#43012,#43013,#43014,#43015,#43016,#43017,#43018,#43019,#43020,#43021,#43022,
#43023,#43024,#43025,#43026,#43027,#43028,#43029,#43030,#43031,#43032,#43033,
#43034,#43035,#43036,#43037,#43038,#43039,#43040,#43041,#43042,#43043,#43044,
#43045,#43046,#43047,#43048,#43049,#43050,#43051,#43052,#43053,#43054,#43055,
#43056,#43057,#43058,#43059,#43060,#43061,#43062,#43063,#43064,#43065,#43066,
#43067,#43068,#43069,#43070,#43071,#43072,#43073,#43074,#43075,#43076,#43077,
#43078,#43079,#43080,#43081,#43082,#43083,#43084,#43085,#43086,#43087,#43088,
#43089,#43090,#43091,#43092,#43093,#43094,#43095,#43096,#43097,#43098,#43099,
#43100,#43101,#43102,#43103,#43104,#43105,#43106,#43107,#43108,#43109,#43110,
#43111,#43112,#43113,#43114,#43115,#43116,#43117,#43118,#43119,#43120,#43121,
#43122,#43123,#43124,#43125,#43126,#43127,#43128,#43129,#43130,#43131,#43132,
#43133,#43134,#43135,#43136,#43137,#43138,#43139,#43140,#43141,#43142,#43143,
#43144,#43145,#43146,#43147,#43148,#43149,#43150,#43151,#43152,#43153,#43154,
#43155,#43156,#43157,#43158,#43159,#43160,#43161,#43162,#43163,#43164,#43165,
#43166,#43167,#43168,#43169,#43170,#43171,#43172,#43173,#43174,#43175,#43176,
#43177),.UNSPECIFIED.,.F.,.F.,(4,2,2,2,2,2,2,2,2,2,2,2,2,2,2,2,2,2,2,2,
2,2,2,2,2,2,2,2,2,2,2,2,2,2,2,2,2,2,2,2,2,2,2,2,2,2,2,2,2,2,2,2,2,2,2,2,
2,2,2,2,2,2,2,2,2,2,2,2,2,2,2,2,2,2,2,2,2,2,2,2,2,2,2,2,2,2,2,2,2,2,2,2,
2,2,2,2,2,2,2,2,2,2,2,2,2,2,2,2,2,2,2,2,4),(-1.45804903820686,-1.44411603124442,
-1.41931364947825,-1.41341293944206,-1.41080266413045,-1.40886170535669,
-1.40705121483662,-1.40455988171319,-1.39819720383853,-1.34992058120615,
-1.32704990428333,-1.31674740446581,-1.31454611555658,-1.31330786400848,
-1.31223703005821,-1.31086420267533,-1.30865436736672,-1.29620903696286,
-1.29147679578464,-1.25491697527206,-1.22448400536502,-1.22010159717905,
-1.21778520182247,-1.21606298734725,-1.21390772642402,-1.21027164814994,
-1.19576936065448,-1.16782955717974,-1.12746451440361,-1.12323445350922,
-1.12157433395621,-1.12056671343561,-1.11946387646818,-1.11788328292449,
-1.11384713031036,-1.0930257268107,-1.05130305455471,-1.03167762524489,
-1.02791629846846,-1.02551156463125,-1.02359819413678,-1.02144102670644,
-1.01779652651438,-1.00318901473943,-0.95347066733627,-0.932750620208573,
-0.929985602457105,-0.928629224592126,-0.927559646597564,-0.926309486657909,
-0.924053979952481,-0.912850070776156,-0.864469000500925,-0.839580014824916,
-0.835596204323731,-0.833124017428689,-0.831203106510309,-0.829084695636985,
-0.825615686110968,-0.813055540777542,-0.762700454526518,-0.759610199259253,
-0.754164578701645,-0.739887822884978,-0.73758930351271,-0.736204759388913,
-0.735130087216258,-0.733913657859962,-0.731812017309895,-0.722957160454548,
-0.705090431905975,-0.676230134081205,-0.647297656289903,-0.643206856889482,
-0.640729480188029,-0.638802131026579,-0.63670666226202,-0.633341967401709,
-0.621853038839032,-0.602301877085459,-0.561006757549835,-0.54737630866855,
-0.545107171359372,-0.543731243198401,-0.542657568539581,-0.541435779445196,
-0.53931001710087,-0.530128889112639,-0.481545305103937,-0.454700250067968,
-0.450659873189332,-0.448197373453389,-0.446272199864192,-0.444169575928009,
-0.44077232405153,-0.428959561920595,-0.37967224122419,-0.355305788630056,
-0.352499805782322,-0.351135241544172,-0.350064944526133,-0.348820530864299,
-0.346591700623393,-0.335846176064526,-0.31126177525271,-0.265477914632111,
-0.258935259735816,-0.256414384522101,-0.254595961428509,-0.252659075479142,
-0.250076005176255,-0.244328738901846,-0.242792485946247),.UNSPECIFIED.);
#1289=B_SPLINE_CURVE_WITH_KNOTS('',3,(#43182,#43183,#43184,#43185,#43186,
#43187,#43188,#43189,#43190,#43191,#43192,#43193,#43194,#43195,#43196,#43197,
#43198,#43199,#43200,#43201,#43202,#43203,#43204,#43205,#43206,#43207,#43208,
#43209,#43210,#43211,#43212,#43213,#43214,#43215,#43216,#43217,#43218,#43219,
#43220,#43221,#43222,#43223,#43224,#43225,#43226,#43227,#43228,#43229,#43230,
#43231,#43232,#43233,#43234,#43235,#43236,#43237,#43238,#43239,#43240,#43241,
#43242,#43243,#43244,#43245,#43246,#43247,#43248,#43249,#43250,#43251,#43252,
#43253,#43254,#43255,#43256,#43257,#43258,#43259,#43260,#43261,#43262,#43263,
#43264,#43265,#43266,#43267,#43268,#43269,#43270,#43271,#43272,#43273,#43274,
#43275,#43276,#43277,#43278,#43279,#43280,#43281,#43282,#43283,#43284,#43285,
#43286,#43287,#43288,#43289,#43290,#43291,#43292,#43293,#43294,#43295,#43296,
#43297,#43298,#43299,#43300,#43301,#43302,#43303,#43304,#43305,#43306,#43307,
#43308,#43309,#43310,#43311,#43312,#43313,#43314,#43315,#43316,#43317,#43318,
#43319,#43320,#43321,#43322,#43323,#43324,#43325,#43326,#43327,#43328,#43329,
#43330,#43331,#43332,#43333,#43334,#43335,#43336,#43337,#43338,#43339,#43340,
#43341,#43342,#43343,#43344,#43345,#43346,#43347,#43348,#43349,#43350,#43351,
#43352,#43353,#43354,#43355,#43356,#43357,#43358,#43359,#43360,#43361,#43362,
#43363,#43364,#43365,#43366,#43367,#43368,#43369,#43370,#43371,#43372,#43373,
#43374,#43375,#43376,#43377,#43378,#43379,#43380,#43381,#43382,#43383,#43384,
#43385,#43386,#43387,#43388,#43389,#43390,#43391,#43392,#43393,#43394,#43395,
#43396,#43397,#43398,#43399,#43400,#43401,#43402,#43403,#43404,#43405,#43406,
#43407),.UNSPECIFIED.,.F.,.F.,(4,2,2,2,2,2,2,2,2,2,2,2,2,2,2,2,2,2,2,2,
2,2,2,2,2,2,2,2,2,2,2,2,2,2,2,2,2,2,2,2,2,2,2,2,2,2,2,2,2,2,2,2,2,2,2,2,
2,2,2,2,2,2,2,2,2,2,2,2,2,2,2,2,2,2,2,2,2,2,2,2,2,2,2,2,2,2,2,2,2,2,2,2,
2,2,2,2,2,2,2,2,2,2,2,2,2,2,2,2,2,2,2,2,4),(-2.1891488065354,-2.18407159117508,
-2.15979983031995,-2.14913383485187,-2.14690988386288,-2.14566659310058,
-2.14459625283958,-2.14323033751547,-2.1404171979368,-2.11511152414759,
-2.0828027222587,-2.05900520967905,-2.053231249635,-2.05064339136501,-2.04870577796628,
-2.0468887483205,-2.04437310819771,-2.03786320923401,-1.99150154532939,
-1.96730017783045,-1.95665173129801,-1.9544287463143,-1.95318561927294,
-1.95211518375039,-1.95074884127597,-1.94793379090312,-1.9223556952876,
-1.89024525756908,-1.86650790491974,-1.86074148965835,-1.85815489694462,
-1.85621738975707,-1.85439984798862,-1.85188252569995,-1.84536267515809,
-1.79916055671009,-1.77484177475619,-1.76416333267218,-1.76193843312834,
-1.76069484164971,-1.75962438649371,-1.75825851074869,-1.75544608042783,
-1.73028692675401,-1.69786638536991,-1.67402924025756,-1.66824986706944,
-1.66566084130567,-1.66372285341205,-1.66190583552197,-1.65939078855576,
-1.65288572872909,-1.60644531195937,-1.58229151716934,-1.5716545869198,
-1.5694321061222,-1.56818899521187,-1.5671184066517,-1.565751652834,-1.56293502569036,
-1.53713253224363,-1.50518579944361,-1.48149220271351,-1.47573106818268,
-1.47314523773344,-1.47120766213391,-1.46938959103355,-1.46687079517596,
-1.46034284864737,-1.41425149688032,-1.38984698160783,-1.3791463523992,
-1.37691991724136,-1.37567589707743,-1.37460534222759,-1.37323968742848,
-1.37105445594421,-1.35908847320552,-1.35390478039994,-1.31033055912168,
-1.28857470422758,-1.28306825710304,-1.28052907871686,-1.27859859569926,
-1.27676650936933,-1.27367727812995,-1.26575457493155,-1.21565024412149,
-1.18756778685796,-1.18474933794885,-1.18338212841215,-1.18231139074868,
-1.18106833635763,-1.17884653393905,-1.16822327014345,-1.14412742366844,
-1.09763702710024,-1.09113657392201,-1.08862209291068,-1.08680508048344,
-1.08486672374035,-1.0822765677241,-1.07649200246857,-1.05261382074484,
-1.02009029026644,-0.99502696360631,-0.992214634511519,-0.990848664520793,
-0.98977807000532,-0.988534233238302,-0.986308704469612,-0.975622953818306,
-0.973731148246856),.UNSPECIFIED.);
#1290=B_SPLINE_CURVE_WITH_KNOTS('',3,(#43409,#43410,#43411,#43412,#43413,
#43414,#43415,#43416,#43417,#43418,#43419,#43420,#43421,#43422,#43423,#43424,
#43425,#43426,#43427,#43428,#43429,#43430,#43431,#43432,#43433,#43434,#43435,
#43436,#43437,#43438,#43439,#43440,#43441,#43442,#43443,#43444,#43445,#43446,
#43447,#43448,#43449,#43450),.UNSPECIFIED.,.F.,.F.,(4,2,2,2,2,2,2,2,2,2,
2,2,2,2,2,2,2,2,2,2,4),(-0.242792485946247,-0.236606260475716,-0.216603844230613,
-0.177600472048637,-0.162467956475159,-0.160135070365004,-0.158740433278701,
-0.157664438586877,-0.156660436687939,-0.154845479375884,-0.14911953504362,
-0.139586203035983,-0.114635212441782,-0.0732474400545378,-0.0665302659882875,
-0.0636998826889005,-0.0619163984637437,-0.0599536284970733,-0.0572212430688076,
-0.0506087548470122,-0.000564233396250174),.UNSPECIFIED.);
#1291=B_SPLINE_CURVE_WITH_KNOTS('',3,(#43451,#43452,#43453,#43454,#43455,
#43456,#43457,#43458,#43459,#43460,#43461,#43462,#43463,#43464,#43465,#43466,
#43467,#43468,#43469,#43470,#43471,#43472,#43473,#43474,#43475,#43476,#43477,
#43478,#43479,#43480,#43481,#43482,#43483,#43484,#43485,#43486,#43487,#43488,
#43489,#43490,#43491,#43492,#43493,#43494,#43495,#43496,#43497,#43498,#43499,
#43500,#43501,#43502,#43503,#43504,#43505,#43506,#43507,#43508,#43509,#43510,
#43511,#43512,#43513,#43514,#43515,#43516,#43517,#43518,#43519,#43520,#43521,
#43522,#43523,#43524,#43525,#43526,#43527,#43528,#43529,#43530,#43531,#43532,
#43533,#43534,#43535,#43536,#43537,#43538,#43539,#43540,#43541,#43542,#43543,
#43544,#43545,#43546,#43547,#43548,#43549,#43550,#43551,#43552,#43553,#43554,
#43555,#43556,#43557,#43558,#43559,#43560,#43561,#43562,#43563,#43564,#43565,
#43566,#43567,#43568,#43569,#43570,#43571,#43572,#43573,#43574,#43575,#43576,
#43577,#43578,#43579,#43580,#43581,#43582,#43583,#43584,#43585,#43586,#43587,
#43588,#43589,#43590,#43591,#43592,#43593,#43594,#43595,#43596,#43597,#43598,
#43599,#43600,#43601,#43602,#43603,#43604,#43605,#43606,#43607,#43608,#43609,
#43610,#43611,#43612,#43613,#43614,#43615,#43616,#43617,#43618,#43619,#43620,
#43621,#43622,#43623,#43624,#43625,#43626),.UNSPECIFIED.,.F.,.F.,(4,2,2,
2,2,2,2,2,2,2,2,2,2,2,2,2,2,2,2,2,2,2,2,2,2,2,2,2,2,2,2,2,2,2,2,2,2,2,2,
2,2,2,2,2,2,2,2,2,2,2,2,2,2,2,2,2,2,2,2,2,2,2,2,2,2,2,2,2,2,2,2,2,2,2,2,
2,2,2,2,2,2,2,2,2,2,2,2,4),(-2.43144843030508,-2.40785000583015,-2.40081715584106,
-2.39898955012162,-2.39776127716115,-2.3967514418594,-2.3956810271092,-2.39431407568053,
-2.39149562376289,-2.36415626395074,-2.3429661710446,-2.31721727850622,
-2.3060587865771,-2.30270362049879,-2.30061026573823,-2.2986822823544,-2.29620049811193,
-2.29209461855544,-2.26247961134774,-2.21309749852176,-2.20704719263268,
-2.20523873696824,-2.20423118381301,-2.20315890103114,-2.20177342189852,
-2.1995220676231,-2.18630323603844,-2.17896668854862,-2.15998733635828,
-2.11753435018015,-2.11178986444075,-2.10920716907905,-2.10727021236919,
-2.10545146162796,-2.10292971542693,-2.09638241916073,-2.050624999603,-2.02598654668394,
-2.01522759358309,-2.01299778004289,-2.01175308504504,-2.01068270850339,
-2.00931826178519,-2.00651324271827,-1.98225073594355,-1.93292688948208,
-1.9210808995237,-1.91768012732984,-1.91557657668874,-1.91365138680606,
-1.91119000910201,-1.90715387836146,-1.88071562406883,-1.86976129225014,
-1.84451043018516,-1.82524940226418,-1.82137031370429,-1.81981441394241,
-1.81871618686855,-1.81770287689808,-1.81601363388956,-1.81160379997301,
-1.77640226859393,-1.73071783308773,-1.72611796769222,-1.72375628374654,
-1.72184635426832,-1.71965954041639,-1.7159769004447,-1.70230398963697,
-1.64234000250745,-1.63025924291869,-1.62795571378017,-1.62669498537163,
-1.62562607093029,-1.62428286458477,-1.62167018288379,-1.6051099103036,
-1.56739941498058,-1.54051901546667,-1.53436308508751,-1.53170741605176,
-1.5297581860298,-1.5279579738794,-1.52550861096656,-1.51939831583559,-1.46849685491709,
-1.45815955314769),.UNSPECIFIED.);
#1292=B_SPLINE_CURVE_WITH_KNOTS('',3,(#43632,#43633,#43634,#43635,#43636,
#43637,#43638,#43639,#43640,#43641,#43642,#43643,#43644,#43645,#43646,#43647,
#43648,#43649,#43650,#43651,#43652,#43653,#43654,#43655,#43656,#43657,#43658,
#43659,#43660,#43661,#43662,#43663,#43664,#43665,#43666,#43667,#43668,#43669,
#43670,#43671,#43672,#43673,#43674,#43675,#43676,#43677,#43678,#43679,#43680,
#43681,#43682,#43683,#43684,#43685,#43686,#43687,#43688,#43689,#43690,#43691,
#43692,#43693,#43694,#43695,#43696,#43697,#43698,#43699,#43700,#43701,#43702,
#43703,#43704,#43705,#43706,#43707,#43708,#43709,#43710,#43711,#43712,#43713,
#43714,#43715,#43716,#43717,#43718,#43719,#43720,#43721,#43722,#43723,#43724,
#43725,#43726,#43727,#43728,#43729,#43730,#43731,#43732,#43733,#43734,#43735,
#43736,#43737,#43738,#43739,#43740,#43741,#43742,#43743,#43744,#43745,#43746,
#43747,#43748,#43749,#43750,#43751,#43752,#43753,#43754,#43755,#43756,#43757,
#43758,#43759,#43760,#43761,#43762,#43763,#43764,#43765,#43766,#43767,#43768,
#43769,#43770,#43771,#43772,#43773,#43774,#43775,#43776,#43777,#43778,#43779,
#43780,#43781,#43782,#43783,#43784,#43785,#43786,#43787,#43788,#43789,#43790,
#43791,#43792,#43793,#43794,#43795,#43796,#43797,#43798,#43799,#43800,#43801,
#43802,#43803,#43804,#43805,#43806,#43807,#43808,#43809,#43810,#43811,#43812,
#43813,#43814,#43815,#43816,#43817),.UNSPECIFIED.,.F.,.F.,(4,2,2,2,2,2,
2,2,2,2,2,2,2,2,2,2,2,2,2,2,2,2,2,2,2,2,2,2,2,2,2,2,2,2,2,2,2,2,2,2,2,2,
2,2,2,2,2,2,2,2,2,2,2,2,2,2,2,2,2,2,2,2,2,2,2,2,2,2,2,2,2,2,2,2,2,2,2,2,
2,2,2,2,2,2,2,2,2,2,2,2,2,2,4),(-0.974056705393386,-0.970767599827482,-0.968248849743031,
-0.966430598933844,-0.964492634670361,-0.961905954975287,-0.956141557687982,
-0.932423006446969,-0.90040565164778,-0.874644663389221,-0.871827496807036,
-0.870460487489761,-0.869389705003979,-0.868146367639386,-0.865923493353298,
-0.855284282705457,-0.831126855210087,-0.784718647842081,-0.778212138159034,
-0.77569658979416,-0.773879222992864,-0.771940875529662,-0.769351399913293,
-0.763571167113192,-0.739728233207329,-0.707303473089765,-0.68209559271628,
-0.679282025970213,-0.677915759069537,-0.676845077488844,-0.675601306485995,
-0.67337630525633,-0.662700976143061,-0.638400270170196,-0.592197954215753,
-0.585678539654812,-0.583160985107273,-0.581343139305016,-0.579405181685472,
-0.576817778872307,-0.571048696888105,-0.547291951846117,-0.515135657007328,
-0.489564133311662,-0.486748260051386,-0.485381570228107,-0.484310890681449,
-0.483067504073187,-0.480844127845821,-0.470194587867565,-0.445995046599982,
-0.399654341647386,-0.393143278441079,-0.390627117579252,-0.388809682585953,
-0.386871609996702,-0.384283100823115,-0.378507546406061,-0.354699458675277,
-0.322375054238652,-0.297033738475139,-0.294219448791694,-0.292853103622761,
-0.291782491249627,-0.290538950233659,-0.28831472761058,-0.277650190713819,
-0.25339073855881,-0.207134540309728,-0.200620242929509,-0.197880099369848,
-0.195947412270461,-0.194001118338801,-0.192026745997686,-0.186780676933051,
-0.179902354445663,-0.163049726484927,-0.137558298351062,-0.104416941036746,
-0.101666486621136,-0.100312839959541,-0.0992432537594365,-0.0979905807456046,
-0.0957242462049522,-0.084334456591408,-0.0339378912075332,-0.0199576090708968,
-0.0140702961719974,-0.00792603025400796,-0.00525623048890964,-0.00332710256047799,
-0.00169315958314438,-0.000563811939861371),.UNSPECIFIED.);
#1293=B_SPLINE_CURVE_WITH_KNOTS('',3,(#43818,#43819,#43820,#43821,#43822,
#43823,#43824,#43825,#43826,#43827,#43828,#43829,#43830,#43831,#43832,#43833,
#43834,#43835,#43836,#43837,#43838,#43839,#43840,#43841,#43842,#43843,#43844,
#43845,#43846,#43847,#43848,#43849,#43850,#43851,#43852,#43853,#43854,#43855,
#43856,#43857,#43858,#43859),.UNSPECIFIED.,.F.,.F.,(4,2,2,2,2,2,2,2,2,2,
2,2,2,2,2,2,2,2,2,2,4),(-2.43117239107418,-2.4290930149489,-2.42472570548591,
-2.40006531117722,-2.3614222198719,-2.34391340408118,-2.34022028516732,
-2.33869485427737,-2.33760229782761,-2.33658159640704,-2.33485398169207,
-2.33019147478549,-2.28681939009497,-2.2531026138123,-2.24618984956439,
-2.24347381374301,-2.24152886814728,-2.23958583461733,-2.23684613990076,
-2.23033209340117,-2.1891488065354),.UNSPECIFIED.);
#1294=B_SPLINE_CURVE_WITH_KNOTS('',3,(#43860,#43861,#43862,#43863,#43864,
#43865,#43866,#43867,#43868,#43869,#43870,#43871,#43872,#43873,#43874,#43875,
#43876,#43877,#43878,#43879,#43880,#43881,#43882,#43883,#43884,#43885,#43886,
#43887,#43888,#43889,#43890,#43891,#43892,#43893,#43894,#43895,#43896,#43897,
#43898,#43899,#43900,#43901,#43902,#43903,#43904,#43905,#43906,#43907,#43908,
#43909,#43910,#43911,#43912,#43913,#43914,#43915,#43916,#43917,#43918,#43919,
#43920,#43921,#43922,#43923,#43924,#43925,#43926,#43927,#43928,#43929,#43930,
#43931,#43932,#43933,#43934,#43935,#43936,#43937,#43938,#43939,#43940,#43941,
#43942,#43943,#43944,#43945,#43946,#43947,#43948,#43949,#43950,#43951,#43952,
#43953,#43954,#43955,#43956,#43957,#43958,#43959,#43960,#43961,#43962,#43963,
#43964,#43965,#43966,#43967,#43968,#43969,#43970,#43971,#43972,#43973,#43974,
#43975,#43976,#43977,#43978,#43979,#43980,#43981,#43982,#43983,#43984,#43985,
#43986,#43987,#43988,#43989,#43990,#43991,#43992,#43993,#43994,#43995,#43996,
#43997,#43998,#43999,#44000,#44001,#44002,#44003,#44004,#44005,#44006,#44007,
#44008,#44009,#44010,#44011,#44012,#44013,#44014,#44015,#44016,#44017,#44018,
#44019,#44020,#44021,#44022,#44023,#44024,#44025,#44026,#44027,#44028,#44029,
#44030,#44031,#44032,#44033,#44034,#44035,#44036,#44037,#44038,#44039,#44040,
#44041,#44042,#44043,#44044,#44045,#44046,#44047,#44048,#44049,#44050,#44051,
#44052,#44053,#44054,#44055,#44056,#44057,#44058,#44059,#44060,#44061,#44062,
#44063,#44064,#44065,#44066,#44067,#44068,#44069,#44070,#44071,#44072,#44073,
#44074,#44075,#44076,#44077,#44078,#44079,#44080,#44081,#44082,#44083,#44084,
#44085,#44086,#44087,#44088,#44089),.UNSPECIFIED.,.F.,.F.,(4,2,2,2,2,2,
2,2,2,2,2,2,2,2,2,2,2,2,2,2,2,2,2,2,2,2,2,2,2,2,2,2,2,2,2,2,2,2,2,2,2,2,
2,2,2,2,2,2,2,2,2,2,2,2,2,2,2,2,2,2,2,2,2,2,2,2,2,2,2,2,2,2,2,2,2,2,2,2,
2,2,2,2,2,2,2,2,2,2,2,2,2,2,2,2,2,2,2,2,2,2,2,2,2,2,2,2,2,2,2,2,2,2,2,2,
4),(-1.45815955314769,-1.44732239483162,-1.4374815980845,-1.43530965035556,
-1.43407751885901,-1.43300529456673,-1.43162192643633,-1.42937800453873,
-1.41626097458002,-1.37521302751139,-1.34801416757412,-1.34182015784328,
-1.33915781988152,-1.33720733922246,-1.33540852808946,-1.33296499174635,
-1.32686946064739,-1.27577362846622,-1.25471878594145,-1.24491146276283,
-1.24274165989903,-1.24150995294707,-1.24043758552606,-1.23905335993059,
-1.2368067246399,-1.22363569591481,-1.21620278656998,-1.19055413225765,
-1.18075585925275,-1.1529041864578,-1.14883716538906,-1.14636632028527,
-1.14443934880887,-1.14233954307896,-1.13895742295031,-1.12730455185172,
-1.10734920133301,-1.0720558348165,-1.06769069478283,-1.05308523263596,
-1.05077249566933,-1.04938351750842,-1.04830795561214,-1.04709340405836,
-1.0450015131953,-1.03628206747524,-0.988270978654193,-0.960350687990752,
-0.956282198022534,-0.953810991505604,-0.951884055767852,-0.949784609839112,
-0.946403777433049,-0.934762463204984,-0.914835477492735,-0.888896014969876,
-0.86094318007732,-0.858124467330395,-0.856757192695807,-0.855686434128333,
-0.854443390088617,-0.852221691153655,-0.841600547227164,-0.817513338268695,
-0.771009110740899,-0.76450940249591,-0.761995017413554,-0.760178011403446,
-0.758239603075399,-0.75564927736428,-0.749863908874753,-0.725979799604828,
-0.693441324549237,-0.668398089841144,-0.665585869300714,-0.664219907676432,
-0.663149298508304,-0.661905420581649,-0.65967975904056,-0.648992234575457,
-0.624642378329538,-0.578513036397747,-0.571989464154865,-0.569471318334955,
-0.567653374251944,-0.565715616815219,-0.563129006459453,-0.557363896546726,
-0.533637087329864,-0.501583030661506,-0.475878850358701,-0.473062334996994,
-0.471695558087341,-0.470624917716716,-0.469381699807339,-0.467158927530579,
-0.456518072773769,-0.432351920759021,-0.385967102003845,-0.379459667396208,
-0.376944159485018,-0.375126951867793,-0.373188894923825,-0.370600015649461,
-0.364821990738335,-0.340993582725157,-0.308606257880663,-0.283354963533916,
-0.280541423394484,-0.279175265685267,-0.278104715785658,-0.276861150774939,
-0.274636648374459,-0.263966221290074,-0.242629061483656),.UNSPECIFIED.);
#1295=B_SPLINE_CURVE_WITH_KNOTS('',3,(#44094,#44095,#44096,#44097,#44098,
#44099,#44100,#44101,#44102,#44103,#44104,#44105,#44106,#44107,#44108,#44109,
#44110,#44111,#44112,#44113,#44114,#44115,#44116,#44117,#44118,#44119,#44120,
#44121,#44122,#44123,#44124,#44125,#44126,#44127,#44128,#44129,#44130,#44131,
#44132,#44133,#44134,#44135,#44136,#44137,#44138,#44139,#44140,#44141,#44142,
#44143,#44144,#44145,#44146,#44147,#44148,#44149,#44150,#44151,#44152,#44153,
#44154,#44155,#44156,#44157,#44158,#44159,#44160,#44161,#44162,#44163,#44164,
#44165,#44166,#44167,#44168,#44169,#44170,#44171,#44172,#44173,#44174,#44175,
#44176,#44177,#44178,#44179,#44180,#44181,#44182,#44183,#44184,#44185,#44186,
#44187,#44188,#44189,#44190,#44191,#44192,#44193,#44194,#44195,#44196,#44197,
#44198,#44199,#44200,#44201,#44202,#44203,#44204,#44205,#44206,#44207,#44208,
#44209,#44210,#44211,#44212,#44213,#44214,#44215,#44216,#44217,#44218,#44219,
#44220,#44221,#44222,#44223,#44224,#44225,#44226,#44227,#44228,#44229,#44230,
#44231,#44232,#44233,#44234,#44235,#44236,#44237,#44238,#44239,#44240,#44241,
#44242,#44243,#44244,#44245,#44246,#44247,#44248,#44249,#44250,#44251,#44252,
#44253,#44254,#44255,#44256,#44257,#44258,#44259,#44260,#44261,#44262,#44263,
#44264,#44265,#44266,#44267,#44268,#44269,#44270,#44271,#44272,#44273,#44274,
#44275,#44276,#44277,#44278,#44279,#44280,#44281,#44282,#44283,#44284,#44285,
#44286,#44287,#44288,#44289,#44290,#44291,#44292,#44293,#44294,#44295,#44296,
#44297,#44298,#44299,#44300,#44301,#44302,#44303,#44304,#44305),
 .UNSPECIFIED.,.F.,.F.,(4,2,2,2,2,2,2,2,2,2,2,2,2,2,2,2,2,2,2,2,2,2,2,2,
2,2,2,2,2,2,2,2,2,2,2,2,2,2,2,2,2,2,2,2,2,2,2,2,2,2,2,2,2,2,2,2,2,2,2,2,
2,2,2,2,2,2,2,2,2,2,2,2,2,2,2,2,2,2,2,2,2,2,2,2,2,2,2,2,2,2,2,2,2,2,2,2,
2,2,2,2,2,2,2,2,2,4),(-2.18988230660751,-2.18020862884737,-2.15522474485167,
-2.13149902818363,-2.12573340665907,-2.12314655975065,-2.12120861939381,
-2.11939049471598,-2.11687208411056,-2.11034779308784,-2.06417767717913,
-2.03982150278388,-2.02913245352607,-2.02690650664556,-2.0256624917424,
-2.02459177367733,-2.02322569379073,-2.02041328568376,-1.99604239516536,
-1.9467732584526,-1.93496561450914,-1.93156816678215,-1.92946505929063,
-1.9275392007042,-1.92507549006123,-1.92103238023235,-1.8941329993509,-1.84541388260516,
-1.83634145487599,-1.83422303722388,-1.83300259187793,-1.83192817379636,
-1.83054884247138,-1.82826906621039,-1.81443650002443,-1.80553599538707,
-1.75544982617297,-1.74256616896649,-1.73906644883103,-1.73694066510838,
-1.73502042061606,-1.73255933509714,-1.72861420416093,-1.70508409941534,
-1.65533141517052,-1.64399602008472,-1.64173226192497,-1.64047994836713,
-1.63941001106574,-1.63805508519747,-1.63529928491342,-1.60235842677999,
-1.57723192580991,-1.55370258545975,-1.54796179730585,-1.54537919422741,
-1.54344167957483,-1.54162194773606,-1.53909811186514,-1.53254110687688,
-1.48689272750605,-1.46215469980333,-1.45136918546287,-1.44913718945494,
-1.44789173510909,-1.44682099239685,-1.44545644904185,-1.44265247361283,
-1.41859883477889,-1.36912828860013,-1.35720003965533,-1.35379031711478,
-1.35168428436138,-1.34975885042809,-1.34729994298328,-1.34327378224955,
-1.31703011668517,-1.30567420457458,-1.28020291482538,-1.26126991671715,
-1.25742413169721,-1.2558732479088,-1.25477565994706,-1.25376065521533,
-1.25206396782874,-1.24760847225538,-1.21635576050806,-1.1698077613698,
-1.1633097746501,-1.16079547791974,-1.15897834638018,-1.1570396280807,-1.15444858428883,
-1.14866033077609,-1.1247563834069,-1.09217127843988,-1.06718673213728,
-1.06437463042073,-1.06300858835561,-1.06193784993263,-1.06069374575655,
-1.05846749233913,-1.04777351747286,-1.02340036986222,-0.977293775021958,
-0.974056705393386),.UNSPECIFIED.);
#1296=B_SPLINE_CURVE_WITH_KNOTS('',3,(#44307,#44308,#44309,#44310,#44311,
#44312,#44313,#44314,#44315,#44316,#44317,#44318,#44319,#44320,#44321,#44322,
#44323,#44324,#44325,#44326,#44327,#44328,#44329,#44330,#44331,#44332,#44333,
#44334,#44335,#44336,#44337,#44338,#44339,#44340,#44341,#44342,#44343,#44344,
#44345,#44346),.UNSPECIFIED.,.F.,.F.,(4,2,2,2,2,2,2,2,2,2,2,2,2,2,2,2,2,
2,2,4),(-0.242629061483656,-0.239682634531744,-0.1934641037118,-0.186947916218177,
-0.184431248901112,-0.182613783776822,-0.18074272676804,-0.178246011784779,
-0.175487868287805,-0.170877890135219,-0.13846529255783,-0.0991266652829539,
-0.0898702697162213,-0.0876598718599338,-0.0864060717597737,-0.0853365957900867,
-0.0839844673452894,-0.0812415895493274,-0.0491039633603923,-0.000564216032066522),
 .UNSPECIFIED.);
#1297=B_SPLINE_CURVE_WITH_KNOTS('',3,(#44347,#44348,#44349,#44350,#44351,
#44352,#44353,#44354,#44355,#44356,#44357,#44358,#44359,#44360,#44361,#44362,
#44363,#44364,#44365,#44366,#44367,#44368,#44369,#44370,#44371,#44372,#44373,
#44374,#44375,#44376,#44377,#44378,#44379,#44380,#44381,#44382,#44383,#44384,
#44385,#44386,#44387,#44388,#44389,#44390,#44391,#44392,#44393,#44394,#44395,
#44396,#44397,#44398,#44399,#44400,#44401,#44402,#44403,#44404,#44405,#44406,
#44407,#44408,#44409,#44410,#44411,#44412,#44413,#44414,#44415,#44416,#44417,
#44418,#44419,#44420,#44421,#44422,#44423,#44424,#44425,#44426,#44427,#44428,
#44429,#44430,#44431,#44432,#44433,#44434,#44435,#44436,#44437,#44438,#44439,
#44440,#44441,#44442,#44443,#44444,#44445,#44446,#44447,#44448,#44449,#44450,
#44451,#44452,#44453,#44454,#44455,#44456,#44457,#44458,#44459,#44460,#44461,
#44462,#44463,#44464,#44465,#44466,#44467,#44468,#44469,#44470,#44471,#44472,
#44473,#44474,#44475,#44476,#44477,#44478,#44479,#44480,#44481,#44482,#44483,
#44484,#44485,#44486,#44487,#44488,#44489,#44490,#44491,#44492,#44493,#44494,
#44495,#44496,#44497,#44498,#44499,#44500,#44501,#44502,#44503,#44504,#44505,
#44506,#44507,#44508,#44509,#44510,#44511,#44512,#44513,#44514,#44515,#44516,
#44517,#44518,#44519,#44520,#44521,#44522,#44523,#44524,#44525,#44526),
 .UNSPECIFIED.,.F.,.F.,(4,2,2,2,2,2,2,2,2,2,2,2,2,2,2,2,2,2,2,2,2,2,2,2,
2,2,2,2,2,2,2,2,2,2,2,2,2,2,2,2,2,2,2,2,2,2,2,2,2,2,2,2,2,2,2,2,2,2,2,2,
2,2,2,2,2,2,2,2,2,2,2,2,2,2,2,2,2,2,2,2,2,2,2,2,2,2,2,2,2,4),(-2.43140689233801,
-2.42730802413046,-2.42384966764435,-2.42197678520656,-2.42013632541179,
-2.41805381072676,-2.41474657866191,-2.40482494816618,-2.35006798177995,
-2.33068438956821,-2.32679299369968,-2.32523527200865,-2.3241368317781,
-2.3231241666317,-2.32143768962451,-2.31704448475864,-2.28112899585354,
-2.24110509170697,-2.23570914056281,-2.23263405531163,-2.23051182522825,
-2.22847121329233,-2.22659964598011,-2.22413640967445,-2.22009303974486,
-2.1932117185811,-2.14452097237056,-2.13544349917663,-2.13332534236296,
-2.1321052809959,-2.13103135690177,-2.12965285963222,-2.12737487317794,
-2.1135662627697,-2.10465940377763,-2.05461570128677,-2.04171198600117,
-2.03821145889551,-2.03608608258357,-2.03416678461417,-2.03170771598067,
-2.02776744732415,-2.00410984452807,-1.95449874146468,-1.94317912566083,
-1.94091696075749,-1.93966532352435,-1.93859583811702,-1.93724132341471,
-1.93448583098649,-1.90158806500461,-1.87652216896889,-1.85293812903845,
-1.84719146553272,-1.84460846852694,-1.84267155586909,-1.84085304339472,
-1.83833194146579,-1.83178815509688,-1.78598031300878,-1.7613814106052,
-1.75063262164552,-1.74840351230983,-1.74715901618346,-1.74608868915105,
-1.74472414859095,-1.74191840928341,-1.71756171542954,-1.66829638977874,
-1.6564858775608,-1.65308875597319,-1.65098609224484,-1.64906080114486,
-1.64659803823337,-1.64255695708556,-1.61570163208136,-1.56709302049328,
-1.55790361113352,-1.55577708686118,-1.5545550599976,-1.55348130266044,
-1.55210544329499,-1.54983678596374,-1.53621703957684,-1.49492499433258,
-1.47538716047664,-1.46390196080592,-1.4605373999802,-1.45844179702659,
-1.45799153533436),.UNSPECIFIED.);
#1298=B_SPLINE_CURVE_WITH_KNOTS('',3,(#44532,#44533,#44534,#44535,#44536,
#44537,#44538,#44539,#44540,#44541,#44542,#44543,#44544,#44545,#44546,#44547,
#44548,#44549,#44550,#44551,#44552,#44553,#44554,#44555,#44556,#44557,#44558,
#44559,#44560,#44561,#44562,#44563,#44564,#44565,#44566,#44567,#44568,#44569,
#44570,#44571,#44572,#44573,#44574,#44575,#44576,#44577,#44578,#44579,#44580,
#44581,#44582,#44583,#44584,#44585,#44586,#44587,#44588,#44589,#44590,#44591,
#44592,#44593,#44594,#44595,#44596,#44597,#44598,#44599,#44600,#44601,#44602,
#44603,#44604,#44605,#44606,#44607,#44608,#44609,#44610,#44611,#44612,#44613,
#44614,#44615,#44616,#44617,#44618,#44619,#44620,#44621,#44622,#44623,#44624,
#44625,#44626,#44627,#44628,#44629,#44630,#44631,#44632,#44633,#44634,#44635,
#44636,#44637,#44638,#44639,#44640,#44641,#44642,#44643,#44644,#44645,#44646,
#44647,#44648,#44649,#44650,#44651,#44652,#44653,#44654,#44655,#44656,#44657,
#44658,#44659,#44660,#44661,#44662,#44663,#44664,#44665,#44666,#44667,#44668,
#44669,#44670,#44671,#44672,#44673,#44674,#44675,#44676,#44677,#44678,#44679,
#44680,#44681,#44682,#44683,#44684,#44685,#44686,#44687,#44688,#44689,#44690,
#44691,#44692,#44693,#44694,#44695,#44696,#44697,#44698,#44699,#44700,#44701,
#44702,#44703,#44704,#44705,#44706,#44707,#44708,#44709,#44710,#44711,#44712,
#44713,#44714,#44715,#44716,#44717,#44718,#44719,#44720,#44721,#44722,#44723,
#44724,#44725,#44726,#44727,#44728,#44729,#44730,#44731),.UNSPECIFIED.,
 .F.,.F.,(4,2,2,2,2,2,2,2,2,2,2,2,2,2,2,2,2,2,2,2,2,2,2,2,2,2,2,2,2,2,2,
2,2,2,2,2,2,2,2,2,2,2,2,2,2,2,2,2,2,2,2,2,2,2,2,2,2,2,2,2,2,2,2,2,2,2,2,
2,2,2,2,2,2,2,2,2,2,2,2,2,2,2,2,2,2,2,2,2,2,2,2,2,2,2,2,2,2,2,2,4),(-0.97398342740053,
-0.968789361277668,-0.965266725663231,-0.960570416671455,-0.946002141715252,
-0.943691261956634,-0.942302975570392,-0.941227687795161,-0.94001314994702,
-0.937920616691668,-0.929188913039654,-0.881145465576063,-0.853287025028794,
-0.849220735468894,-0.846750441118566,-0.84482396273153,-0.84272475851091,
-0.839343748850874,-0.82769612619938,-0.80775146912542,-0.77275384054031,
-0.768060200998447,-0.753492154119069,-0.751181382289118,-0.749793168302248,
-0.748717941271087,-0.747503477310026,-0.745411083233981,-0.736680131350044,
-0.688640198281378,-0.660782354850949,-0.656716274212725,-0.65424611436532,
-0.652319745407183,-0.65022066500978,-0.646839864898028,-0.635193065905695,
-0.615249941840422,-0.58027423357657,-0.575552480206659,-0.560992661202858,
-0.558682321382804,-0.557294274842584,-0.556219120642795,-0.555004674660426,
-0.552912166829224,-0.544178656171066,-0.496132215096054,-0.468288168448986,
-0.464222616924401,-0.461752686018684,-0.459826440263581,-0.457727438197202,
-0.454346640793039,-0.442698609209978,-0.422751877753202,-0.3822367226858,
-0.368432767544484,-0.366154858310516,-0.364776359165642,-0.363702399926604,
-0.362482247943189,-0.360363834948695,-0.351283378875099,-0.302619137294814,
-0.275743799216676,-0.271702727583868,-0.269240048974191,-0.26731488249938,
-0.265212415497841,-0.26181574843141,-0.250008412649237,-0.200730365289813,
-0.17635237101312,-0.173545085341349,-0.172180280486157,-0.171109983227981,
-0.171104885878602,-0.17109985722943,-0.171094896126241,-0.171090001282427,
-0.171085171468235,-0.171080405514773,-0.171075702294062,-0.171071060659346,
-0.169836383949264,-0.167670621475185,-0.164939434463173,-0.159107639417711,
-0.141509908166866,-0.112041215706876,-0.0833372334848896,-0.0792513797624821,
-0.0767753920112682,-0.0748481662874705,-0.0727518684183954,-0.069383726633986,
-0.0578620861435787,-0.0382304328438444,-0.000564480343473832),
 .UNSPECIFIED.);
#1299=B_SPLINE_CURVE_WITH_KNOTS('',3,(#44732,#44733,#44734,#44735,#44736,
#44737,#44738,#44739,#44740,#44741,#44742,#44743,#44744,#44745,#44746,#44747,
#44748,#44749,#44750,#44751,#44752,#44753,#44754,#44755,#44756,#44757,#44758,
#44759,#44760,#44761,#44762,#44763,#44764,#44765,#44766,#44767,#44768,#44769,
#44770,#44771,#44772,#44773,#44774,#44775,#44776,#44777,#44778,#44779,#44780,
#44781,#44782,#44783,#44784,#44785,#44786,#44787),.UNSPECIFIED.,.F.,.F.,
(4,2,2,2,2,2,2,2,2,2,2,2,2,2,2,2,2,2,2,2,2,2,2,2,2,2,2,4),(-2.43183342158011,
-2.41479196364183,-2.41296275867932,-2.41173372599316,-2.41072356638809,
-2.40965298480507,-2.40828648451585,-2.40609834958051,-2.39407687652996,
-2.3855012686747,-2.35151229207745,-2.33166344231834,-2.32005262071449,
-2.31667513422864,-2.31457657965056,-2.31264966593554,-2.31017738443359,
-2.30610472255568,-2.27800301443796,-2.23010211394347,-2.22433170748115,
-2.22162094479725,-2.2194489721092,-2.21822263232837,-2.21715280704875,
-2.21579726637834,-2.21303773047925,-2.18988230660751),.UNSPECIFIED.);
#1300=B_SPLINE_CURVE_WITH_KNOTS('',3,(#44788,#44789,#44790,#44791,#44792,
#44793,#44794,#44795,#44796,#44797,#44798,#44799,#44800,#44801,#44802,#44803,
#44804,#44805,#44806,#44807,#44808,#44809,#44810,#44811,#44812,#44813,#44814,
#44815,#44816,#44817,#44818,#44819,#44820,#44821,#44822,#44823,#44824,#44825,
#44826,#44827,#44828,#44829,#44830,#44831,#44832,#44833,#44834,#44835,#44836,
#44837,#44838,#44839,#44840,#44841,#44842,#44843,#44844,#44845,#44846,#44847,
#44848,#44849,#44850,#44851,#44852,#44853,#44854,#44855,#44856,#44857,#44858,
#44859,#44860,#44861,#44862,#44863,#44864,#44865,#44866,#44867,#44868,#44869,
#44870,#44871,#44872,#44873,#44874,#44875,#44876,#44877,#44878,#44879,#44880,
#44881,#44882,#44883,#44884,#44885,#44886,#44887,#44888,#44889,#44890,#44891,
#44892,#44893,#44894,#44895,#44896,#44897,#44898,#44899,#44900,#44901,#44902,
#44903,#44904,#44905,#44906,#44907,#44908,#44909,#44910,#44911,#44912,#44913,
#44914,#44915,#44916,#44917,#44918,#44919,#44920,#44921,#44922,#44923,#44924,
#44925,#44926,#44927,#44928,#44929,#44930,#44931,#44932,#44933,#44934,#44935,
#44936,#44937,#44938,#44939,#44940,#44941,#44942,#44943,#44944,#44945,#44946,
#44947,#44948,#44949,#44950,#44951,#44952,#44953,#44954,#44955,#44956,#44957,
#44958,#44959,#44960,#44961,#44962,#44963,#44964,#44965,#44966,#44967,#44968,
#44969,#44970,#44971,#44972,#44973,#44974,#44975,#44976,#44977,#44978,#44979,
#44980,#44981,#44982,#44983,#44984,#44985,#44986,#44987,#44988,#44989,#44990,
#44991,#44992,#44993,#44994,#44995,#44996,#44997,#44998,#44999,#45000,#45001,
#45002,#45003,#45004,#45005,#45006,#45007),.UNSPECIFIED.,.F.,.F.,(4,2,2,
2,2,2,2,2,2,2,2,2,2,2,2,2,2,2,2,2,2,2,2,2,2,2,2,2,2,2,2,2,2,2,2,2,2,2,2,
2,2,2,2,2,2,2,2,2,2,2,2,2,2,2,2,2,2,2,2,2,2,2,2,2,2,2,2,2,2,2,2,2,2,2,2,
2,2,2,2,2,2,2,2,2,2,2,2,2,2,2,2,2,2,2,2,2,2,2,2,2,2,2,2,2,2,2,2,2,2,4),
(-1.45799153533436,-1.45651417706466,-1.45403624613571,-1.44994405409045,
-1.42097709480293,-1.39209919572151,-1.36867732705061,-1.36439485985391,
-1.362776523103,-1.36166600052332,-1.3606654929809,-1.35904417830258,-1.3550473207155,
-1.312064391649,-1.28580827308421,-1.27660644739737,-1.27001644747882,-1.26728761919184,
-1.26532537659116,-1.26354098881585,-1.26070621604771,-1.25396336127136,
-1.21576901676488,-1.17622344647632,-1.17197318108443,-1.17030952396949,
-1.16930104917613,-1.168198464086,-1.16662023684018,-1.16260083811927,-1.14195464856034,
-1.10018730489828,-1.08040023259733,-1.07663015773493,-1.07422242216828,
-1.07230832110076,-1.07015208760232,-1.0665134259311,-1.05198792680941,
-1.02398010559419,-0.983675247784505,-0.979450802613525,-0.977791304773497,
-0.976783596635041,-0.975680235883655,-0.974098167166473,-0.970054359585526,
-0.921162681269848,-0.88856605718916,-0.884410662117065,-0.88191416045053,
-0.87998371854712,-0.877896633990358,-0.874570909331996,-0.863460421535659,
-0.844833376384835,-0.804420847416611,-0.788672332436125,-0.786089591973712,
-0.784752853919872,-0.783684319587785,-0.782418433068192,-0.780090907330598,
-0.767532812312541,-0.736725087439566,-0.695994912039856,-0.691871033066363,
-0.689383743796099,-0.687454677948254,-0.685363344218717,-0.682018387597583,
-0.670724481050623,-0.651653325621746,-0.612535221539828,-0.59619701944811,
-0.593592138557923,-0.592250623469297,-0.59118182495394,-0.589919787918668,
-0.587610145699826,-0.575409100155573,-0.513140824030563,-0.501526108351775,
-0.49801047818145,-0.495881615044767,-0.493962817257088,-0.49150944246179,
-0.48645173660807,-0.479883294958928,-0.464121348109848,-0.42038480522287,
-0.415022082955552,-0.403241580038739,-0.401066651294722,-0.399704232860486,
-0.398634098053535,-0.397388125173552,-0.395152186636372,-0.384287760935015,
-0.359224624415685,-0.314103749499636,-0.307524123919663,-0.304997410533382,
-0.3031774375461,-0.301241361157506,-0.298663590341235,-0.292945697496344,
-0.269581291711543,-0.244309336638491,-0.242475885032187),.UNSPECIFIED.);
#1301=B_SPLINE_CURVE_WITH_KNOTS('',3,(#45012,#45013,#45014,#45015,#45016,
#45017,#45018,#45019,#45020,#45021,#45022,#45023,#45024,#45025,#45026,#45027,
#45028,#45029,#45030,#45031,#45032,#45033,#45034,#45035,#45036,#45037,#45038,
#45039,#45040,#45041,#45042,#45043,#45044,#45045,#45046,#45047,#45048,#45049,
#45050,#45051,#45052,#45053,#45054,#45055,#45056,#45057,#45058,#45059,#45060,
#45061,#45062,#45063,#45064,#45065,#45066,#45067,#45068,#45069,#45070,#45071,
#45072,#45073,#45074,#45075,#45076,#45077,#45078,#45079,#45080,#45081,#45082,
#45083,#45084,#45085,#45086,#45087,#45088,#45089,#45090,#45091,#45092,#45093,
#45094,#45095,#45096,#45097,#45098,#45099,#45100,#45101,#45102,#45103,#45104,
#45105,#45106,#45107,#45108,#45109,#45110,#45111,#45112,#45113,#45114,#45115,
#45116,#45117,#45118,#45119,#45120,#45121,#45122,#45123,#45124,#45125,#45126,
#45127,#45128,#45129,#45130,#45131,#45132,#45133,#45134,#45135,#45136,#45137,
#45138,#45139,#45140,#45141,#45142,#45143,#45144,#45145,#45146,#45147,#45148,
#45149,#45150,#45151,#45152,#45153,#45154,#45155,#45156,#45157,#45158,#45159,
#45160,#45161,#45162,#45163,#45164,#45165,#45166,#45167,#45168,#45169,#45170,
#45171,#45172,#45173,#45174,#45175,#45176,#45177,#45178,#45179,#45180,#45181,
#45182,#45183,#45184,#45185,#45186,#45187,#45188,#45189,#45190,#45191,#45192,
#45193,#45194,#45195,#45196,#45197,#45198,#45199,#45200,#45201,#45202,#45203,
#45204,#45205,#45206,#45207,#45208,#45209,#45210,#45211,#45212,#45213,#45214,
#45215,#45216,#45217,#45218,#45219,#45220,#45221,#45222,#45223,#45224,#45225,
#45226,#45227),.UNSPECIFIED.,.F.,.F.,(4,2,2,2,2,2,2,2,2,2,2,2,2,2,2,2,2,
2,2,2,2,2,2,2,2,2,2,2,2,2,2,2,2,2,2,2,2,2,2,2,2,2,2,2,2,2,2,2,2,2,2,2,2,
2,2,2,2,2,2,2,2,2,2,2,2,2,2,2,2,2,2,2,2,2,2,2,2,2,2,2,2,2,2,2,2,2,2,2,2,
2,2,2,2,2,2,2,2,2,2,2,2,2,2,2,2,2,2,4),(-2.18954711984868,-2.18843508427736,
-2.18217025824943,-2.13183465909379,-2.11041638015107,-2.10062439548328,
-2.09839846759916,-2.09714683209159,-2.09607728962157,-2.09472262747542,
-2.09196658823948,-2.05908052686512,-2.03399035419614,-2.01041420920415,
-2.004668434598,-2.00208552494448,-2.000148553169,-1.99832989437154,-1.99580844475497,
-1.98926290823627,-1.9434473845648,-1.91885340361622,-1.90810563330579,
-1.90587650964589,-1.90463197419128,-1.90356159367554,-1.90219695933854,
-1.89939094106571,-1.8750170619244,-1.82575882625216,-1.81395368239914,
-1.81055698808115,-1.8084543541203,-1.80652893391879,-1.80406579064773,
-1.80002362590504,-1.77313142876445,-1.7244262815198,-1.71535236617163,
-1.71323416964948,-1.71201394404838,-1.71093978102919,-1.7095608560479,
-1.70728191373387,-1.69352812041669,-1.68459733085101,-1.63461952082228,
-1.62161915620125,-1.61810943021373,-1.61598173919837,-1.61406245397801,
-1.61160631766428,-1.60767664512738,-1.58463005044965,-1.53442712766417,
-1.5230529366638,-1.52078736744537,-1.51953483070341,-1.51846518057668,
-1.51711122998332,-1.51435941743451,-1.48130136576737,-1.45595594057811,
-1.43272012602413,-1.42701792996058,-1.42444267747988,-1.42250665901046,
-1.42068539468321,-1.41815473433718,-1.41155194896732,-1.36660946282598,
-1.34138433543342,-1.3304795426544,-1.32824082624815,-1.32699407969633,
-1.32592375764581,-1.32456172450014,-1.32176950947304,-1.298758299962,-1.26487566894333,
-1.24695088769403,-1.23977632115703,-1.2343519312359,-1.2318279227496,-1.22989946552966,
-1.2280621674189,-1.22494669344176,-1.21644189586132,-1.2159940573012,-1.20206001071282,
-1.17281884631323,-1.15957262311967,-1.13887344489183,-1.13610865929863,
-1.13475219517047,-1.13368245149794,-1.13243198490166,-1.13017564181538,
-1.11896171069095,-1.07048639413291,-1.04568353353247,-1.04170182323602,
-1.03923005824389,-1.03730893557505,-1.03518974466993,-1.03171821005687,
-1.01913498544038,-0.97398342740053),.UNSPECIFIED.);
#1302=B_SPLINE_CURVE_WITH_KNOTS('',3,(#45229,#45230,#45231,#45232,#45233,
#45234,#45235,#45236,#45237,#45238,#45239,#45240,#45241,#45242,#45243,#45244,
#45245,#45246,#45247,#45248,#45249,#45250,#45251,#45252,#45253,#45254,#45255,
#45256,#45257,#45258,#45259,#45260,#45261,#45262,#45263,#45264,#45265,#45266,
#45267,#45268,#45269,#45270,#45271,#45272,#45273,#45274,#45275,#45276,#45277,
#45278,#45279,#45280,#45281,#45282,#45283,#45284,#45285,#45286,#45287,#45288,
#45289,#45290,#45291,#45292,#45293,#45294,#45295,#45296,#45297,#45298,#45299,
#45300,#45301,#45302,#45303,#45304,#45305,#45306,#45307,#45308,#45309,#45310,
#45311,#45312,#45313,#45314,#45315,#45316,#45317,#45318,#45319,#45320,#45321,
#45322),.UNSPECIFIED.,.F.,.F.,(4,2,2,2,2,2,2,2,2,2,2,2,2,2,2,2,2,2,2,2,
2,2,2,2,2,2,2,2,2,2,2,2,2,2,2,2,2,2,2,2,2,2,2,2,2,2,4),(-0.242475885032187,
-0.211311516992314,-0.208556292319953,-0.207201817003389,-0.206208042780248,
-0.206203817915274,-0.206199683161047,-0.206195636544027,-0.206192019441469,
-0.206188420176096,-0.206184838611877,-0.206181274743271,-0.206177728430791,
-0.206174199566654,-0.206170688246241,-0.206167194404566,-0.206163717687113,
-0.20616025810502,-0.206156815386804,-0.206153389527791,-0.206149980554044,
-0.206146588168098,-0.204925604908831,-0.20276948903304,-0.200088336227301,
-0.194405976488265,-0.177506579186398,-0.159876697351341,-0.121865362242285,
-0.11512466485239,-0.112290320204464,-0.110506058339158,-0.108543830494773,
-0.105814801981801,-0.0992232583093638,-0.0900175597048242,-0.0637414610418433,
-0.030333017612405,-0.0224419710486729,-0.0186641397871498,-0.0160563233359045,
-0.0147142666500038,-0.0137075916180399,-0.0126989203002053,-0.0114764548261663,
-0.00966312529024703,-0.000563390165638188),.UNSPECIFIED.);
#1303=B_SPLINE_CURVE_WITH_KNOTS('',3,(#45323,#45324,#45325,#45326,#45327,
#45328,#45329,#45330,#45331,#45332,#45333,#45334,#45335,#45336,#45337,#45338,
#45339,#45340,#45341,#45342,#45343,#45344,#45345,#45346,#45347,#45348,#45349,
#45350,#45351,#45352,#45353,#45354,#45355,#45356,#45357,#45358,#45359,#45360,
#45361,#45362,#45363,#45364,#45365,#45366,#45367,#45368,#45369,#45370,#45371,
#45372,#45373,#45374,#45375,#45376,#45377,#45378,#45379,#45380,#45381,#45382,
#45383,#45384,#45385,#45386,#45387,#45388,#45389,#45390,#45391,#45392,#45393,
#45394,#45395,#45396,#45397,#45398,#45399,#45400,#45401,#45402,#45403,#45404,
#45405,#45406,#45407,#45408,#45409,#45410,#45411,#45412,#45413,#45414,#45415,
#45416,#45417,#45418,#45419,#45420,#45421,#45422,#45423,#45424,#45425,#45426,
#45427,#45428,#45429,#45430,#45431,#45432,#45433,#45434,#45435,#45436,#45437,
#45438,#45439,#45440,#45441,#45442,#45443,#45444,#45445,#45446,#45447,#45448,
#45449,#45450,#45451,#45452,#45453,#45454,#45455,#45456,#45457,#45458,#45459,
#45460,#45461,#45462,#45463,#45464,#45465,#45466,#45467,#45468,#45469,#45470,
#45471,#45472,#45473,#45474,#45475,#45476,#45477,#45478,#45479,#45480,#45481,
#45482,#45483,#45484,#45485,#45486,#45487,#45488,#45489,#45490,#45491,#45492,
#45493,#45494,#45495,#45496,#45497,#45498),.UNSPECIFIED.,.F.,.F.,(4,2,2,
2,2,2,2,2,2,2,2,2,2,2,2,2,2,2,2,2,2,2,2,2,2,2,2,2,2,2,2,2,2,2,2,2,2,2,2,
2,2,2,2,2,2,2,2,2,2,2,2,2,2,2,2,2,2,2,2,2,2,2,2,2,2,2,2,2,2,2,2,2,2,2,2,
2,2,2,2,2,2,2,2,2,2,2,2,4),(-2.43201023192336,-2.41829679723027,-2.36793049198057,
-2.35539612686519,-2.35192890121182,-2.34981050631577,-2.34788890998877,
-2.34541485945137,-2.34142600117818,-2.31640932036142,-2.27985334704831,
-2.26453959265631,-2.25920982259474,-2.25664833554951,-2.25459398025459,
-2.2533838605833,-2.25234705228238,-2.25098690718971,-2.24820391392017,
-2.22587235576064,-2.17578201699542,-2.16291765311221,-2.15942013393211,
-2.15729509797618,-2.15537514895323,-2.15291391380682,-2.14896747144052,
-2.125371311619,-2.07569592984939,-2.06436883949363,-2.062105862622,-2.06085386588979,
-2.05978412844462,-2.05842936515504,-2.05567359874798,-2.02276743251201,
-1.99769575491309,-1.97410569598012,-1.96835760453313,-1.9657739773459,
-1.96383659677978,-1.96201764838483,-1.95949594751044,-1.95295063806469,
-1.90713085053513,-1.88252667180167,-1.8717754558079,-1.86954581916108,
-1.86830102531784,-1.86723044015574,-1.86586556782549,-1.86305913731539,
-1.83869492073372,-1.78941868214392,-1.7776059289547,-1.7742080489118,-1.7721048918289,
-1.77017913307196,-1.76771575004489,-1.76367360461862,-1.73680818062124,
-1.68817847211972,-1.67899846068376,-1.67687226288339,-1.67565012657541,
-1.67457607582821,-1.67319958845993,-1.67092937937136,-1.65728919869154,
-1.61602007559205,-1.59646825030886,-1.58497652423159,-1.58161076819369,
-1.57951457513966,-1.5775865162642,-1.57510816548938,-1.57101559162511,
-1.5420689196837,-1.51317274152033,-1.49528784424624,-1.48642682118663,
-1.48432416439205,-1.48310723498795,-1.48203217347373,-1.48064720948833,
-1.47834817101076,-1.46407236322947,-1.45834644240502),.UNSPECIFIED.);
#1304=B_SPLINE_CURVE_WITH_KNOTS('',3,(#45504,#45505,#45506,#45507,#45508,
#45509,#45510,#45511,#45512,#45513,#45514,#45515,#45516,#45517,#45518,#45519,
#45520,#45521,#45522,#45523,#45524,#45525,#45526,#45527,#45528,#45529,#45530,
#45531,#45532,#45533,#45534,#45535,#45536,#45537,#45538,#45539,#45540,#45541,
#45542,#45543,#45544,#45545,#45546,#45547,#45548,#45549,#45550,#45551,#45552,
#45553,#45554,#45555,#45556,#45557,#45558,#45559,#45560,#45561,#45562,#45563,
#45564,#45565,#45566,#45567,#45568,#45569,#45570,#45571,#45572,#45573,#45574,
#45575,#45576,#45577,#45578,#45579,#45580,#45581,#45582,#45583,#45584,#45585,
#45586,#45587,#45588,#45589,#45590,#45591,#45592,#45593,#45594,#45595,#45596,
#45597,#45598,#45599,#45600,#45601,#45602,#45603,#45604,#45605,#45606,#45607,
#45608,#45609,#45610,#45611,#45612,#45613,#45614,#45615,#45616,#45617,#45618,
#45619,#45620,#45621,#45622,#45623,#45624,#45625,#45626,#45627,#45628,#45629,
#45630,#45631,#45632,#45633,#45634,#45635,#45636,#45637,#45638,#45639,#45640,
#45641,#45642,#45643,#45644,#45645,#45646,#45647,#45648,#45649,#45650,#45651,
#45652,#45653,#45654,#45655,#45656,#45657,#45658,#45659,#45660,#45661,#45662,
#45663,#45664,#45665,#45666,#45667,#45668,#45669,#45670,#45671,#45672,#45673,
#45674,#45675,#45676,#45677,#45678,#45679,#45680,#45681),.UNSPECIFIED.,
 .F.,.F.,(4,2,2,2,2,2,2,2,2,2,2,2,2,2,2,2,2,2,2,2,2,2,2,2,2,2,2,2,2,2,2,
2,2,2,2,2,2,2,2,2,2,2,2,2,2,2,2,2,2,2,2,2,2,2,2,2,2,2,2,2,2,2,2,2,2,2,2,
2,2,2,2,2,2,2,2,2,2,2,2,2,2,2,2,2,2,2,2,2,4),(-0.973746388460305,-0.964026499357242,
-0.925008914880137,-0.920865169477403,-0.918372219975626,-0.916442493527153,
-0.914354160686515,-0.911022069794456,-0.899848797001676,-0.88106940061312,
-0.839700173427234,-0.833881447720076,-0.824522836744943,-0.822304412055297,
-0.821048852704035,-0.819979656117997,-0.81863015094139,-0.815899968897619,
-0.785792992478453,-0.734974663461587,-0.728860798445624,-0.726411095616516,
-0.724611015576052,-0.722662294579658,-0.720007982801653,-0.713858226769834,
-0.687021263813445,-0.64776263229401,-0.632581134377751,-0.630246352083531,
-0.628851155971027,-0.627775081247309,-0.626564790244736,-0.624491037538719,
-0.615999144676198,-0.599259944139691,-0.562511411147729,-0.539607283698179,
-0.535682879100219,-0.533228434301822,-0.531309492542256,-0.529181179666661,
-0.525668107005635,-0.512628410796253,-0.462660004739359,-0.45370597408244,
-0.439975617433199,-0.437699381671416,-0.43632131094361,-0.435247319506291,
-0.434026713992213,-0.431906557439573,-0.422804055243892,-0.374152722725726,
-0.3472814055064,-0.343240129129532,-0.340777274139774,-0.338851938760359,
-0.336749255803814,-0.333352169891232,-0.321732819678866,-0.301779703417091,
-0.257494562288134,-0.247107054256051,-0.245014733199427,-0.243677455637427,
-0.242608974608807,-0.241343720371571,-0.23901884340004,-0.226644628619756,
-0.194653327343986,-0.160038725792635,-0.15207563127623,-0.149041812479143,
-0.147220511019105,-0.14528495563211,-0.143388340674838,-0.139122847388627,
-0.113835882725883,-0.0937843897785946,-0.0578023244281912,-0.0534078898783422,
-0.0517209993357558,-0.0507081033863247,-0.0496094269939885,-0.0480513976124226,
-0.0462896458552489,-0.0431471780912219,-0.000564085736078712),
 .UNSPECIFIED.);
#1305=B_SPLINE_CURVE_WITH_KNOTS('',3,(#45682,#45683,#45684,#45685,#45686,
#45687,#45688,#45689,#45690,#45691,#45692,#45693,#45694,#45695,#45696,#45697,
#45698,#45699,#45700,#45701,#45702,#45703,#45704,#45705,#45706,#45707,#45708,
#45709,#45710,#45711,#45712,#45713,#45714,#45715,#45716,#45717,#45718,#45719,
#45720,#45721,#45722,#45723,#45724,#45725,#45726,#45727,#45728,#45729,#45730,
#45731,#45732,#45733,#45734,#45735),.UNSPECIFIED.,.F.,.F.,(4,2,2,2,2,2,
2,2,2,2,2,2,2,2,2,2,2,2,2,2,2,2,2,2,2,2,4),(-2.43166641639941,-2.4035822623252,
-2.39321099227628,-2.39010269405064,-2.38796676598012,-2.38588059230468,
-2.38395033182375,-2.38145313275954,-2.37729450241099,-2.34422996694495,
-2.32249358193877,-2.29712234873137,-2.29217173168749,-2.29085510082182,
-2.28961152279337,-2.28854122649356,-2.28717574386714,-2.28436476465057,
-2.25935341469091,-2.23098557959375,-2.21075322911876,-2.20297145278707,
-2.19723601869153,-2.19466096879313,-2.19271686184005,-2.19091029731729,
-2.18954711984868),.UNSPECIFIED.);
#1306=B_SPLINE_CURVE_WITH_KNOTS('',3,(#45736,#45737,#45738,#45739,#45740,
#45741,#45742,#45743,#45744,#45745,#45746,#45747,#45748,#45749,#45750,#45751,
#45752,#45753,#45754,#45755,#45756,#45757,#45758,#45759,#45760,#45761,#45762,
#45763,#45764,#45765,#45766,#45767,#45768,#45769,#45770,#45771,#45772,#45773,
#45774,#45775,#45776,#45777,#45778,#45779,#45780,#45781,#45782,#45783,#45784,
#45785,#45786,#45787,#45788,#45789,#45790,#45791,#45792,#45793,#45794,#45795,
#45796,#45797,#45798,#45799,#45800,#45801,#45802,#45803,#45804,#45805,#45806,
#45807,#45808,#45809,#45810,#45811,#45812,#45813,#45814,#45815,#45816,#45817,
#45818,#45819,#45820,#45821,#45822,#45823,#45824,#45825,#45826,#45827,#45828,
#45829,#45830,#45831,#45832,#45833,#45834,#45835,#45836,#45837,#45838,#45839,
#45840,#45841,#45842,#45843,#45844,#45845,#45846,#45847,#45848,#45849,#45850,
#45851,#45852,#45853,#45854,#45855,#45856,#45857,#45858,#45859,#45860,#45861,
#45862,#45863,#45864,#45865,#45866,#45867,#45868,#45869,#45870,#45871,#45872,
#45873,#45874,#45875,#45876,#45877,#45878,#45879,#45880,#45881,#45882,#45883,
#45884,#45885,#45886,#45887,#45888,#45889,#45890,#45891,#45892,#45893,#45894,
#45895,#45896,#45897,#45898,#45899,#45900,#45901,#45902,#45903,#45904,#45905,
#45906,#45907,#45908,#45909,#45910,#45911,#45912,#45913,#45914,#45915,#45916,
#45917,#45918,#45919,#45920,#45921,#45922,#45923,#45924,#45925,#45926,#45927,
#45928,#45929,#45930,#45931,#45932,#45933,#45934,#45935,#45936,#45937,#45938,
#45939,#45940,#45941,#45942,#45943),.UNSPECIFIED.,.F.,.F.,(4,2,2,2,2,2,
2,2,2,2,2,2,2,2,2,2,2,2,2,2,2,2,2,2,2,2,2,2,2,2,2,2,2,2,2,2,2,2,2,2,2,2,
2,2,2,2,2,2,2,2,2,2,2,2,2,2,2,2,2,2,2,2,2,2,2,2,2,2,2,2,2,2,2,2,2,2,2,2,
2,2,2,2,2,2,2,2,2,2,2,2,2,2,2,2,2,2,2,2,2,2,2,2,2,4),(-1.45834644240502,
-1.42374471371173,-1.39700114213766,-1.39086112834712,-1.38820797082164,
-1.38625894713713,-1.38445777320206,-1.38200532844103,-1.37587813168322,
-1.3251133445948,-1.3222390361035,-1.29486859212337,-1.29216182246573,-1.29081674281652,
-1.28974749362049,-1.28848771402035,-1.28625195090993,-1.27667900905391,
-1.216226484536,-1.20075922531249,-1.19692105602227,-1.1946980654169,-1.19279023294875,
-1.19047343204715,-1.18609194423199,-1.15576595879912,-1.12851542892481,
-1.10243564931261,-1.09961715089813,-1.09824993184173,-1.09717919368131,
-1.09593614685932,-1.09371437808789,-1.08309166203224,-1.05899798684945,
-1.01250427586629,-1.00600402375574,-1.00348957544059,-1.00167257192859,
-0.999734211052079,-0.997144026022698,-0.991359297349661,-0.967479841021998,
-0.934952977495644,-0.909894206510875,-0.907081910778686,-0.905715947616078,
-0.904645353996951,-0.90340151334074,-0.901175965658991,-0.890489896755449,
-0.866145513954071,-0.820009780551091,-0.813486763016654,-0.810968729891711,
-0.809150834333133,-0.807213098156615,-0.804626463728066,-0.798861080013256,
-0.775131789383233,-0.743067991407038,-0.717377792553701,-0.714561399194917,
-0.713194659663292,-0.712124038135746,-0.710880830152675,-0.708658046312723,
-0.698016575058588,-0.673847703047412,-0.627467128808157,-0.620960165856165,
-0.618444757656858,-0.616627595116704,-0.614689561211031,-0.6121006695439,
-0.606322435305216,-0.582492043188745,-0.550098296407065,-0.524857081595505,
-0.52204365583862,-0.52067753398953,-0.519607002770865,-0.518363448664692,
-0.516138939268841,-0.505467969160891,-0.481181940966927,-0.434971472167958,
-0.4284531672314,-0.425936003306884,-0.424118427322185,-0.42218074601925,
-0.419593692658138,-0.413825308436699,-0.39007094459325,-0.365100651915328,
-0.332263432392804,-0.329504468238845,-0.328149175243173,-0.327079531844555,
-0.325828230566595,-0.323567994022054,-0.312284983825815,-0.263069673735912,
-0.242708007470264),.UNSPECIFIED.);
#1307=B_SPLINE_CURVE_WITH_KNOTS('',3,(#45948,#45949,#45950,#45951,#45952,
#45953,#45954,#45955,#45956,#45957,#45958,#45959,#45960,#45961,#45962,#45963,
#45964,#45965,#45966,#45967,#45968,#45969,#45970,#45971,#45972,#45973,#45974,
#45975,#45976,#45977,#45978,#45979,#45980,#45981,#45982,#45983,#45984,#45985,
#45986,#45987,#45988,#45989,#45990,#45991,#45992,#45993,#45994,#45995,#45996,
#45997,#45998,#45999,#46000,#46001,#46002,#46003,#46004,#46005,#46006,#46007,
#46008,#46009,#46010,#46011,#46012,#46013,#46014,#46015,#46016,#46017,#46018,
#46019,#46020,#46021,#46022,#46023,#46024,#46025,#46026,#46027,#46028,#46029,
#46030,#46031,#46032,#46033,#46034,#46035,#46036,#46037,#46038,#46039,#46040,
#46041,#46042,#46043,#46044,#46045,#46046,#46047,#46048,#46049,#46050,#46051,
#46052,#46053,#46054,#46055,#46056,#46057,#46058,#46059,#46060,#46061,#46062,
#46063,#46064,#46065,#46066,#46067,#46068,#46069,#46070,#46071,#46072,#46073,
#46074,#46075,#46076,#46077,#46078,#46079,#46080,#46081,#46082,#46083,#46084,
#46085,#46086,#46087,#46088,#46089,#46090,#46091,#46092,#46093,#46094,#46095,
#46096,#46097,#46098,#46099,#46100,#46101,#46102,#46103,#46104,#46105,#46106,
#46107,#46108,#46109,#46110,#46111,#46112,#46113,#46114,#46115,#46116,#46117,
#46118,#46119,#46120,#46121,#46122,#46123,#46124,#46125,#46126,#46127,#46128,
#46129,#46130,#46131,#46132,#46133,#46134,#46135,#46136,#46137,#46138,#46139,
#46140,#46141,#46142,#46143,#46144,#46145,#46146,#46147,#46148,#46149,#46150,
#46151,#46152,#46153,#46154,#46155,#46156,#46157,#46158,#46159,#46160,#46161,
#46162,#46163,#46164,#46165,#46166,#46167,#46168,#46169,#46170,#46171,#46172,
#46173,#46174,#46175,#46176,#46177),.UNSPECIFIED.,.F.,.F.,(4,2,2,2,2,2,
2,2,2,2,2,2,2,2,2,2,2,2,2,2,2,2,2,2,2,2,2,2,2,2,2,2,2,2,2,2,2,2,2,2,2,2,
2,2,2,2,2,2,2,2,2,2,2,2,2,2,2,2,2,2,2,2,2,2,2,2,2,2,2,2,2,2,2,2,2,2,2,2,
2,2,2,2,2,2,2,2,2,2,2,2,2,2,2,2,2,2,2,2,2,2,2,2,2,2,2,2,2,2,2,2,2,2,2,2,
4),(-2.18892388094417,-2.1843488704546,-2.17199046622995,-2.16967335405779,
-2.16840995352589,-2.16734162029971,-2.16600274244,-2.16340894683327,-2.14735269665759,
-2.1407038627092,-2.09031069828951,-2.07783695997642,-2.07437631571477,
-2.07225991018016,-2.07033879336962,-2.06786349888921,-2.06386881771297,
-2.03877015875202,-1.99057038181363,-1.97938330526312,-1.97712884419471,
-1.97587897099879,-1.97480945309321,-1.97345292163124,-1.97068682159884,
-1.94992345679077,-1.91985680301451,-1.88711406842814,-1.88267922302751,
-1.88035180266203,-1.87844416353084,-1.87623150446256,-1.87243612394093,
-1.85752223922304,-1.84935861118924,-1.81155852248697,-1.78976721460458,
-1.78563730698772,-1.78404221216232,-1.78293651519665,-1.78193185046896,
-1.78028742345155,-1.77615192579642,-1.73433178542166,-1.69480400245381,
-1.69026818711351,-1.68791986831109,-1.68601108594607,-1.68381490241827,
-1.68009089967871,-1.66595926189511,-1.65640861839957,-1.60585411835963,
-1.59445066798587,-1.59218386973542,-1.59093125500479,-1.58986190700698,
-1.5885088105629,-1.58576027760468,-1.55259324215636,-1.52703410495093,
-1.5040829436025,-1.49841850040637,-1.49585051131698,-1.49391600210762,
-1.49209325908414,-1.48955589128635,-1.4829069899875,-1.43923754022666,
-1.41307723349706,-1.40194816402122,-1.3996968001989,-1.39844749429663,
-1.39737775150074,-1.39602002263345,-1.39324846733114,-1.37205880270645,
-1.33841266162355,-1.31911370763122,-1.3077258025411,-1.30437137600113,
-1.30227810235601,-1.30034993680233,-1.29786755992181,-1.29375992426504,
-1.26407275131254,-1.23619952520191,-1.2277150158654,-1.21569054920526,
-1.2090190516832,-1.2070297305276,-1.20583820086272,-1.2047570216075,-1.20330108139657,
-1.20001032803684,-1.19548653160004,-1.18350163005669,-1.14508698648702,
-1.11734597306032,-1.11328274193258,-1.11081342320432,-1.10888717753662,
-1.10678769304258,-1.10340505283826,-1.09173993784322,-1.07175099433473,
-1.03349084653365,-1.01764228267197,-1.01505590478967,-1.01371847762994,
-1.01265003097012,-1.01138499820538,-1.0090609999237,-0.996570127006823,
-0.973746388460305),.UNSPECIFIED.);
#1308=B_SPLINE_CURVE_WITH_KNOTS('',3,(#46179,#46180,#46181,#46182,#46183,
#46184,#46185,#46186,#46187,#46188,#46189,#46190,#46191,#46192,#46193,#46194,
#46195,#46196,#46197,#46198,#46199,#46200,#46201,#46202,#46203,#46204,#46205,
#46206,#46207,#46208,#46209,#46210,#46211,#46212,#46213,#46214,#46215,#46216,
#46217,#46218,#46219,#46220,#46221,#46222,#46223,#46224,#46225,#46226,#46227,
#46228,#46229,#46230,#46231,#46232,#46233,#46234,#46235,#46236),
 .UNSPECIFIED.,.F.,.F.,(4,2,2,2,2,2,2,2,2,2,2,2,2,2,2,2,2,2,2,2,2,2,2,2,
2,2,2,2,4),(-0.242708007470264,-0.239038576650452,-0.235080102347808,-0.232615348612138,
-0.230695119825303,-0.228905579258431,-0.225960965083586,-0.217282374486274,
-0.203984666361365,-0.173075737777023,-0.142287490478921,-0.137838005971676,
-0.136142596534498,-0.135128081889868,-0.13403077769428,-0.13247988995464,
-0.128632028598946,-0.112421686013435,-0.0933912558259936,-0.0727848811857325,
-0.0467009348712936,-0.0426806923945847,-0.0402239591333887,-0.03829937000933,
-0.0365110374283958,-0.0344440954814045,-0.0315055729894532,-0.0221457821256158,
-0.000563535122424079),.UNSPECIFIED.);
#1309=B_SPLINE_CURVE_WITH_KNOTS('',3,(#46237,#46238,#46239,#46240,#46241,
#46242,#46243,#46244,#46245,#46246,#46247,#46248,#46249,#46250,#46251,#46252,
#46253,#46254,#46255,#46256,#46257,#46258,#46259,#46260,#46261,#46262,#46263,
#46264,#46265,#46266,#46267,#46268,#46269,#46270,#46271,#46272,#46273,#46274,
#46275,#46276,#46277,#46278,#46279,#46280,#46281,#46282,#46283,#46284,#46285,
#46286,#46287,#46288,#46289,#46290,#46291,#46292,#46293,#46294,#46295,#46296,
#46297,#46298,#46299,#46300,#46301,#46302,#46303,#46304,#46305,#46306,#46307,
#46308,#46309,#46310,#46311,#46312,#46313,#46314,#46315,#46316,#46317,#46318,
#46319,#46320,#46321,#46322,#46323,#46324,#46325,#46326,#46327,#46328,#46329,
#46330,#46331,#46332,#46333,#46334,#46335,#46336,#46337,#46338,#46339,#46340,
#46341,#46342,#46343,#46344,#46345,#46346,#46347,#46348,#46349,#46350,#46351,
#46352,#46353,#46354,#46355,#46356,#46357,#46358,#46359,#46360,#46361,#46362,
#46363,#46364,#46365,#46366,#46367,#46368,#46369,#46370,#46371,#46372,#46373,
#46374,#46375,#46376,#46377,#46378,#46379,#46380,#46381,#46382,#46383,#46384,
#46385,#46386,#46387,#46388,#46389,#46390,#46391,#46392,#46393,#46394,#46395,
#46396,#46397,#46398,#46399,#46400,#46401,#46402,#46403,#46404,#46405,#46406,
#46407,#46408,#46409,#46410,#46411,#46412),.UNSPECIFIED.,.F.,.F.,(4,2,2,
2,2,2,2,2,2,2,2,2,2,2,2,2,2,2,2,2,2,2,2,2,2,2,2,2,2,2,2,2,2,2,2,2,2,2,2,
2,2,2,2,2,2,2,2,2,2,2,2,2,2,2,2,2,2,2,2,2,2,2,2,2,2,2,2,2,2,2,2,2,2,2,2,
2,2,2,2,2,2,2,2,2,2,2,2,4),(-2.43194619973958,-2.38643680506946,-2.38052321123352,
-2.37647803904974,-2.37489573106975,-2.37379230532373,-2.37278461431682,
-2.37112529738533,-2.36690211191859,-2.32662888658048,-2.306188174032,-2.28517197525235,
-2.28102647635352,-2.27914198623931,-2.27721235382981,-2.27537824489537,
-2.27227871178857,-2.26388014691298,-2.26313491361184,-2.26123166742741,
-2.22060196103296,-2.19600030640739,-2.1852500502366,-2.18302058437965,
-2.18177588197233,-2.18070537300041,-2.17934059463958,-2.1765343467141,
-2.1521699206584,-2.1028983301243,-2.09108713368274,-2.08768956717104,-2.08558657596555,
-2.08366095032344,-2.08119771174316,-2.07715574821591,-2.05028796985693,
-2.00165062761665,-1.99248499313785,-1.9903599399778,-1.98913810992845,
-1.98806409468184,-1.98668735416955,-1.98441611556206,-1.97075747964463,
-1.9616618011355,-1.91156201494552,-1.89870278912326,-1.89520553501889,
-1.89308044058222,-1.89116029706932,-1.88869861559295,-1.88475105782276,
-1.86112640155451,-1.81147215585378,-1.80014639200279,-1.79788334906934,
-1.79663127219778,-1.79556143949831,-1.79420652127494,-1.79145032717075,
-1.75853536815557,-1.73345028878398,-1.70987286559356,-1.70412616749733,
-1.7015426591062,-1.69960516512639,-1.69778596271455,-1.69526367446354,
-1.68871546402137,-1.64293149103429,-1.61829670759328,-1.60753744098217,
-1.60530718476164,-1.60406219037432,-1.60299152366787,-1.60162666482692,
-1.59882065663587,-1.5745261215384,-1.52520397167212,-1.51336406308118,
-1.50996329741003,-1.50785938644611,-1.50593362436087,-1.50347118179144,
-1.49943259432383,-1.47272844074429,-1.45847283624988),.UNSPECIFIED.);
#1310=B_SPLINE_CURVE_WITH_KNOTS('',3,(#46418,#46419,#46420,#46421,#46422,
#46423,#46424,#46425,#46426,#46427,#46428,#46429,#46430,#46431,#46432,#46433,
#46434,#46435,#46436,#46437,#46438,#46439,#46440,#46441,#46442,#46443,#46444,
#46445,#46446,#46447,#46448,#46449,#46450,#46451,#46452,#46453,#46454,#46455,
#46456,#46457,#46458,#46459,#46460,#46461,#46462,#46463,#46464,#46465,#46466,
#46467,#46468,#46469,#46470,#46471,#46472,#46473,#46474,#46475,#46476,#46477,
#46478,#46479,#46480,#46481,#46482,#46483,#46484,#46485,#46486,#46487,#46488,
#46489,#46490,#46491,#46492,#46493,#46494,#46495,#46496,#46497,#46498,#46499,
#46500,#46501,#46502,#46503,#46504,#46505,#46506,#46507,#46508,#46509,#46510,
#46511,#46512,#46513,#46514,#46515,#46516,#46517,#46518,#46519,#46520,#46521,
#46522,#46523,#46524,#46525,#46526,#46527,#46528,#46529,#46530,#46531,#46532,
#46533,#46534,#46535,#46536,#46537,#46538,#46539,#46540,#46541,#46542,#46543,
#46544,#46545,#46546,#46547,#46548,#46549,#46550,#46551,#46552,#46553,#46554,
#46555,#46556,#46557,#46558,#46559,#46560,#46561,#46562,#46563,#46564,#46565,
#46566,#46567,#46568),.UNSPECIFIED.,.F.,.F.,(4,3,3,3,3,3,3,3,3,3,3,3,3,
3,3,3,3,3,3,3,3,3,3,3,3,3,3,3,3,3,3,3,3,3,3,3,3,3,3,3,3,3,3,3,3,3,3,3,3,
3,4),(135.088484104361,135.19457077706,135.300665273228,135.406886595447,
135.513169775309,135.619670278263,135.719134631849,135.825008513915,135.93617421847,
136.041760973883,136.147283992731,136.25277968045,136.358284400424,136.463902842808,
136.569587321621,136.67545053338,136.714334150354,136.82020803242,136.931373736974,
137.036960492388,137.142483511235,137.247979198954,137.353483918929,137.459102361313,
137.564786840126,137.670650051885,137.709533668858,137.815407550924,137.926573255479,
138.032160010892,138.13768302974,138.243178717459,138.348683437433,138.454301879818,
138.55998635863,138.66584957039,138.704733187363,138.810607069429,138.921772773984,
139.027359529397,139.132882548245,139.238378235964,139.343882955938,139.449501398322,
139.555185877135,139.661049088894,139.699932705868,139.805771670952,139.911472047979,
140.017065096305,140.120587878827),.UNSPECIFIED.);
#1311=B_SPLINE_CURVE_WITH_KNOTS('',3,(#46569,#46570,#46571,#46572,#46573,
#46574,#46575,#46576,#46577,#46578,#46579,#46580,#46581,#46582,#46583,#46584,
#46585,#46586,#46587,#46588,#46589,#46590,#46591,#46592,#46593,#46594,#46595,
#46596,#46597,#46598,#46599,#46600,#46601,#46602,#46603,#46604,#46605,#46606,
#46607,#46608,#46609,#46610),.UNSPECIFIED.,.F.,.F.,(4,2,2,2,2,2,2,2,2,2,
2,2,2,2,2,2,2,2,2,2,4),(-2.43085120260907,-2.4218930692744,-2.3732304159689,
-2.36414340232433,-2.36202507088455,-2.36080524156356,-2.35973174341889,
-2.35835407650429,-2.35607804526844,-2.34229979991363,-2.33357368029187,
-2.29450145198639,-2.27936350646572,-2.27297675430417,-2.2680761656219,
-2.26566166773466,-2.26381204113711,-2.26197018280592,-2.25882689403973,
-2.25012351517351,-2.18892388094417),.UNSPECIFIED.);
#1312=B_SPLINE_CURVE_WITH_KNOTS('',3,(#46611,#46612,#46613,#46614,#46615,
#46616,#46617,#46618,#46619,#46620,#46621,#46622,#46623,#46624,#46625,#46626,
#46627,#46628,#46629,#46630,#46631,#46632,#46633,#46634,#46635,#46636,#46637,
#46638,#46639,#46640,#46641,#46642,#46643,#46644,#46645,#46646,#46647,#46648,
#46649,#46650,#46651,#46652,#46653,#46654,#46655,#46656,#46657,#46658,#46659,
#46660,#46661,#46662,#46663,#46664,#46665,#46666,#46667,#46668,#46669,#46670,
#46671,#46672,#46673,#46674,#46675,#46676,#46677,#46678,#46679,#46680,#46681,
#46682,#46683,#46684,#46685,#46686,#46687,#46688,#46689,#46690,#46691,#46692,
#46693,#46694,#46695,#46696,#46697,#46698,#46699,#46700,#46701,#46702,#46703,
#46704,#46705,#46706,#46707,#46708,#46709,#46710,#46711,#46712,#46713,#46714,
#46715,#46716,#46717,#46718,#46719,#46720,#46721,#46722,#46723,#46724,#46725,
#46726,#46727,#46728,#46729,#46730,#46731,#46732,#46733,#46734,#46735,#46736,
#46737,#46738,#46739,#46740,#46741,#46742,#46743,#46744,#46745,#46746,#46747,
#46748,#46749,#46750,#46751,#46752,#46753,#46754,#46755,#46756,#46757,#46758,
#46759,#46760,#46761,#46762,#46763,#46764,#46765,#46766,#46767,#46768,#46769,
#46770,#46771,#46772,#46773,#46774,#46775,#46776,#46777,#46778,#46779,#46780,
#46781,#46782,#46783,#46784,#46785,#46786,#46787,#46788,#46789,#46790,#46791,
#46792,#46793,#46794,#46795,#46796,#46797,#46798,#46799,#46800,#46801,#46802,
#46803,#46804,#46805,#46806,#46807,#46808,#46809,#46810,#46811,#46812,#46813,
#46814,#46815,#46816,#46817,#46818,#46819,#46820,#46821,#46822,#46823,#46824,
#46825,#46826,#46827,#46828,#46829,#46830,#46831,#46832,#46833,#46834,#46835,
#46836,#46837,#46838),.UNSPECIFIED.,.F.,.F.,(4,2,2,2,2,2,2,2,2,2,2,2,2,
2,2,2,2,2,2,2,2,2,2,2,2,2,2,2,2,2,2,2,2,2,2,2,2,2,2,2,2,2,2,2,2,2,2,2,2,
2,2,2,2,2,2,2,2,2,2,2,2,2,2,2,2,2,2,2,2,2,2,2,2,2,2,2,2,2,2,2,2,2,2,2,2,
2,2,2,2,2,2,2,2,2,2,2,2,2,2,2,2,2,2,2,2,2,2,2,2,2,2,2,2,4),(-1.45847283624988,
-1.42448104976427,-1.41480729857782,-1.41264633664841,-1.41141648204844,
-1.41034366997905,-1.40895616369512,-1.40669886288321,-1.39331110372,-1.38939161230587,
-1.35220191876228,-1.33235836169835,-1.32074869529503,-1.31737074171904,
-1.3152717257304,-1.31334427360727,-1.31087114249934,-1.30679673990829,
-1.27865968173235,-1.23076682075486,-1.22209487069045,-1.22000632946136,
-1.21879237462672,-1.21771641841138,-1.21632575396059,-1.21330956422072,
-1.18514208765776,-1.13244841661113,-1.12655765196056,-1.12414557315679,
-1.12235435477634,-1.12039696035579,-1.11769762176706,-1.11128841518579,
-1.08223935854675,-1.04294581977014,-1.03014229915132,-1.02791330905034,
-1.02653425910949,-1.02546223213671,-1.02422674637145,-1.0220403522293,
-1.01198545223261,-0.990045532705057,-0.94035466596778,-0.934117946781772,
-0.931646853860487,-0.929840811876034,-0.927894911801151,-0.925260896532167,
-0.919231601188733,-0.893401491294308,-0.852753394268094,-0.847835417932028,
-0.837305384501196,-0.835203382475635,-0.83386287443638,-0.832793836131314,
-0.831530294760042,-0.829214734453587,-0.81690711207722,-0.752415906348205,
-0.750508920171359,-0.742220614031927,-0.739137165946123,-0.737306079560877,
-0.735374861676985,-0.732831725764556,-0.727304785851107,-0.705395560581283,
-0.662189960510224,-0.658083806982385,-0.644917449006924,-0.642670973943648,
-0.641286796220091,-0.640214428578387,-0.63898266929941,-0.636812666993299,
-0.627002141650751,-0.60593849674924,-0.554897578235623,-0.548799145697978,
-0.546355118445305,-0.54455616808783,-0.54260575003587,-0.539943890108808,
-0.533752805864446,-0.50657520393874,-0.469630588248447,-0.465537757261919,
-0.452356649907539,-0.450109552699725,-0.448725228570267,-0.447652898983027,
-0.446421354464429,-0.444252135798799,-0.434452030859449,-0.413424504584609,
-0.362328485355368,-0.356238497188287,-0.353795949088853,-0.35199743903901,
-0.350046874928202,-0.347383695745733,-0.34118442484052,-0.313936337359388,
-0.286171739665607,-0.260335079083255,-0.257517883491338,-0.256150979568555,
-0.255080336776874,-0.253837227238005,-0.251614921289972,-0.242510440294479),
 .UNSPECIFIED.);
#1313=B_SPLINE_CURVE_WITH_KNOTS('',3,(#46844,#46845,#46846,#46847,#46848,
#46849,#46850,#46851,#46852,#46853,#46854,#46855,#46856,#46857,#46858,#46859,
#46860,#46861,#46862,#46863,#46864,#46865,#46866,#46867,#46868,#46869,#46870,
#46871,#46872,#46873,#46874,#46875,#46876,#46877,#46878,#46879,#46880,#46881,
#46882,#46883,#46884,#46885,#46886,#46887,#46888,#46889,#46890,#46891,#46892,
#46893,#46894,#46895,#46896,#46897,#46898,#46899,#46900,#46901,#46902,#46903,
#46904,#46905,#46906,#46907,#46908,#46909,#46910,#46911,#46912,#46913,#46914,
#46915,#46916,#46917,#46918,#46919,#46920,#46921,#46922,#46923,#46924,#46925,
#46926,#46927,#46928,#46929,#46930,#46931,#46932,#46933,#46934,#46935,#46936,
#46937,#46938,#46939,#46940,#46941,#46942,#46943,#46944,#46945,#46946,#46947,
#46948,#46949,#46950,#46951,#46952,#46953,#46954,#46955,#46956,#46957,#46958,
#46959,#46960,#46961,#46962,#46963,#46964,#46965,#46966,#46967,#46968,#46969,
#46970,#46971,#46972,#46973,#46974,#46975,#46976,#46977,#46978,#46979,#46980,
#46981,#46982,#46983,#46984,#46985,#46986,#46987,#46988,#46989,#46990,#46991,
#46992,#46993,#46994,#46995,#46996,#46997,#46998,#46999,#47000,#47001,#47002,
#47003,#47004,#47005,#47006,#47007,#47008,#47009,#47010,#47011,#47012,#47013,
#47014,#47015,#47016,#47017,#47018,#47019,#47020,#47021,#47022,#47023,#47024,
#47025),.UNSPECIFIED.,.F.,.F.,(4,2,2,2,2,2,2,2,2,2,2,2,2,2,2,2,2,2,2,2,
2,2,2,2,2,2,2,2,2,2,2,2,2,2,2,2,2,2,2,2,2,2,2,2,2,2,2,2,2,2,2,2,2,2,2,2,
2,2,2,2,2,2,2,2,2,2,2,2,2,2,2,2,2,2,2,2,2,2,2,2,2,2,2,2,2,2,2,2,2,2,4),
(-0.97396649970557,-0.963160677049242,-0.936493329974217,-0.932456435089873,
-0.92999466299771,-0.928069219250143,-0.925965447727417,-0.922564446150021,
-0.910719168795666,-0.861372828057179,-0.837082522994241,-0.834276636619951,
-0.832911899907758,-0.831841362256304,-0.830596547743831,-0.828366701262137,
-0.817610474823226,-0.792987604902333,-0.747238785022208,-0.740691912692005,
-0.73817001886883,-0.736351054949499,-0.734413772548259,-0.731830482143081,
-0.726084016251074,-0.702502908975983,-0.677401453655629,-0.644473610654205,
-0.641717208988461,-0.64036232220085,-0.639292582175733,-0.638040684943666,
-0.63577815854317,-0.624458264319718,-0.57484907492696,-0.55121838206422,
-0.547271206301607,-0.544809692621628,-0.542889649515154,-0.540764634857739,
-0.537267442119368,-0.524407900964139,-0.474283930768112,-0.465354681437526,
-0.451533540689114,-0.449254447227754,-0.447875421872581,-0.44680117185509,
-0.445580825225109,-0.44346238522139,-0.434386540518391,-0.38570445419734,
-0.358836444568864,-0.354785521745208,-0.35231961929378,-0.350393601061566,
-0.348291895541077,-0.344900210592264,-0.333148490768363,-0.31294369840165,
-0.277719852171861,-0.273534786846673,-0.259052848455541,-0.256745409839309,
-0.255358096443446,-0.254282885854908,-0.253067669961399,-0.250972243616042,
-0.242203552825536,-0.224610651414523,-0.175037354543392,-0.173210348356956,
-0.171921917447971,-0.170072966897399,-0.163187272095047,-0.160329254175153,
-0.158540649031897,-0.156725911650928,-0.154172490534364,-0.14854749344977,
-0.140942067916782,-0.121393663295704,-0.0800739361752444,-0.0664513076675939,
-0.064182412995454,-0.0628064564478728,-0.0617326493067222,-0.0605105833603781,
-0.0583840487260259,-0.0491950908041694,-0.000564353419034184),
 .UNSPECIFIED.);
#1314=B_SPLINE_CURVE_WITH_KNOTS('',3,(#47026,#47027,#47028,#47029,#47030,
#47031,#47032,#47033,#47034,#47035,#47036,#47037,#47038,#47039,#47040,#47041,
#47042,#47043,#47044,#47045,#47046,#47047,#47048,#47049,#47050,#47051,#47052,
#47053,#47054,#47055,#47056,#47057,#47058,#47059,#47060,#47061,#47062,#47063,
#47064,#47065),.UNSPECIFIED.,.F.,.F.,(4,3,3,3,3,3,3,3,3,3,3,3,3,4),(140.120587878827,
140.226084307905,140.331587186861,140.437202184293,140.542880897559,140.648740549922,
140.695132224372,140.800694341929,140.906103434911,141.011396551526,141.116620100793,
141.221803227789,141.327013037885,141.371669411541),.UNSPECIFIED.);
#1315=B_SPLINE_CURVE_WITH_KNOTS('',3,(#47067,#47068,#47069,#47070,#47071,
#47072,#47073,#47074,#47075,#47076,#47077,#47078,#47079,#47080,#47081,#47082,
#47083,#47084,#47085,#47086,#47087,#47088,#47089,#47090,#47091,#47092,#47093,
#47094,#47095,#47096,#47097,#47098,#47099,#47100,#47101,#47102,#47103,#47104,
#47105,#47106,#47107,#47108),.UNSPECIFIED.,.F.,.F.,(4,2,2,2,2,2,2,2,2,2,
2,2,2,2,2,2,2,2,2,2,4),(-0.242510440294479,-0.240981513752686,-0.21684452742106,
-0.169409698756096,-0.163471707480922,-0.161115789464972,-0.15916083636883,
-0.157365049449781,-0.15482361530898,-0.148704683956145,-0.140251434050436,
-0.117292739366224,-0.0803531418467185,-0.0672818280338345,-0.0650402297128775,
-0.0636576336542719,-0.0625855799040149,-0.0613531507775264,-0.0591795220341944,
-0.0493108473116508,-0.000564367400856858),.UNSPECIFIED.);
#1316=B_SPLINE_CURVE_WITH_KNOTS('',3,(#47109,#47110,#47111,#47112,#47113,
#47114,#47115,#47116,#47117,#47118,#47119,#47120,#47121,#47122,#47123,#47124,
#47125,#47126,#47127,#47128,#47129,#47130,#47131,#47132,#47133,#47134,#47135,
#47136,#47137,#47138,#47139,#47140,#47141,#47142,#47143,#47144,#47145,#47146,
#47147,#47148,#47149,#47150,#47151,#47152,#47153,#47154,#47155,#47156,#47157,
#47158,#47159,#47160,#47161,#47162,#47163,#47164,#47165,#47166,#47167,#47168,
#47169,#47170,#47171,#47172,#47173,#47174,#47175,#47176,#47177,#47178,#47179,
#47180,#47181,#47182,#47183,#47184,#47185,#47186,#47187,#47188,#47189,#47190,
#47191,#47192,#47193,#47194,#47195,#47196,#47197,#47198,#47199,#47200,#47201,
#47202,#47203,#47204,#47205,#47206,#47207,#47208,#47209,#47210,#47211,#47212,
#47213,#47214,#47215,#47216,#47217,#47218,#47219,#47220,#47221,#47222,#47223,
#47224,#47225,#47226,#47227,#47228,#47229,#47230,#47231,#47232,#47233,#47234,
#47235,#47236,#47237,#47238,#47239,#47240,#47241,#47242,#47243,#47244,#47245,
#47246,#47247,#47248,#47249,#47250,#47251,#47252,#47253,#47254,#47255,#47256,
#47257,#47258,#47259,#47260,#47261,#47262,#47263,#47264,#47265,#47266,#47267,
#47268,#47269,#47270,#47271,#47272,#47273,#47274,#47275,#47276,#47277,#47278,
#47279,#47280,#47281,#47282,#47283,#47284,#47285,#47286,#47287,#47288,#47289,
#47290,#47291,#47292,#47293,#47294,#47295,#47296,#47297,#47298,#47299,#47300,
#47301,#47302,#47303,#47304,#47305,#47306,#47307,#47308,#47309,#47310,#47311,
#47312,#47313,#47314,#47315,#47316,#47317,#47318,#47319,#47320,#47321,#47322,
#47323,#47324,#47325,#47326,#47327,#47328,#47329,#47330,#47331,#47332,#47333,
#47334,#47335,#47336,#47337,#47338),.UNSPECIFIED.,.F.,.F.,(4,2,2,2,2,2,
2,2,2,2,2,2,2,2,2,2,2,2,2,2,2,2,2,2,2,2,2,2,2,2,2,2,2,2,2,2,2,2,2,2,2,2,
2,2,2,2,2,2,2,2,2,2,2,2,2,2,2,2,2,2,2,2,2,2,2,2,2,2,2,2,2,2,2,2,2,2,2,2,
2,2,2,2,2,2,2,2,2,2,2,2,2,2,2,2,2,2,2,2,2,2,2,2,2,2,2,2,2,2,2,2,2,2,2,2,
4),(-2.43130179521416,-2.40521661328843,-2.40210741262236,-2.39997151240219,
-2.3981760791286,-2.39626619950669,-2.39389373123154,-2.39023600490332,
-2.37230348877159,-2.35969568972471,-2.31584478156482,-2.30511357571031,
-2.30288634235593,-2.30164264811573,-2.30057285711815,-2.29920880146605,
-2.29640339207263,-2.27193528943643,-2.25973863257918,-2.2275793913354,
-2.2171313737183,-2.21221386664805,-2.20824241610447,-2.20602490885012,
-2.20600881579687,-2.20599227243346,-2.20597526443617,-2.20595777695779,
-2.20593979463704,-2.20592130162841,-2.20590228038918,-2.20588271280846,
-2.2058625834411,-2.20584187399575,-2.20582056545482,-2.20579863810674,
-2.20577607186008,-2.20575886829018,-2.20573933453463,-2.20571715025449,
-2.20569195021371,-2.20566332153779,-2.20563079088278,-2.20559381851842,
-2.20555178906137,-2.20362595385859,-2.20115553039861,-2.19708694822443,
-2.16926467954086,-2.12119390049976,-2.11245615078168,-2.11036367085829,
-2.10914943017043,-2.10807457879296,-2.10668709414727,-2.10437805449337,
-2.08983741058363,-2.08559487402455,-2.07411127348399,-2.05073267941089,
-2.0304300153756,-2.01863966990622,-2.01524501322652,-2.01314317408843,
-2.01121817092183,-2.008755133366,-2.00471222892042,-1.97781857453458,-1.92909608301112,
-1.92006057449843,-1.91794556695003,-1.91672623711903,-1.91565223400078,
-1.9142727089416,-1.91199111632163,-1.89809976450573,-1.85728076763408,
-1.83763625946661,-1.82610867045518,-1.82274023405638,-1.82064405160731,
-1.81871713202263,-1.81624181394433,-1.81215762847284,-1.7835168878772,
-1.75406980019526,-1.73638282186629,-1.72758586797076,-1.72548868611437,
-1.72427330133332,-1.72319850816391,-1.72181247819941,-1.71950873369246,
-1.70510219572368,-1.70099261770262,-1.66547840417381,-1.6382961237278,
-1.63210507254481,-1.62944377751171,-1.62749397557211,-1.62569573055,-1.62325287152882,
-1.61715853509714,-1.56608715218077,-1.54503470288607,-1.53522934655712,
-1.53306018122405,-1.53182886676045,-1.53075686085098,-1.52937312788663,
-1.52712734324978,-1.51396277641544,-1.51293567800882,-1.47638090775202,
-1.45815515730985),.UNSPECIFIED.);
#1317=B_SPLINE_CURVE_WITH_KNOTS('',3,(#47343,#47344,#47345,#47346,#47347,
#47348,#47349,#47350,#47351,#47352,#47353,#47354,#47355,#47356,#47357,#47358,
#47359,#47360,#47361,#47362,#47363,#47364,#47365,#47366,#47367,#47368,#47369,
#47370,#47371,#47372,#47373,#47374,#47375,#47376,#47377,#47378,#47379,#47380,
#47381,#47382,#47383,#47384,#47385,#47386,#47387,#47388,#47389,#47390,#47391,
#47392,#47393,#47394,#47395,#47396,#47397,#47398,#47399,#47400,#47401,#47402,
#47403,#47404,#47405,#47406,#47407,#47408,#47409,#47410,#47411,#47412,#47413,
#47414,#47415,#47416,#47417,#47418,#47419,#47420,#47421,#47422,#47423,#47424,
#47425,#47426,#47427,#47428,#47429,#47430,#47431,#47432,#47433,#47434,#47435,
#47436,#47437,#47438,#47439,#47440,#47441,#47442,#47443,#47444,#47445,#47446,
#47447,#47448,#47449,#47450,#47451,#47452,#47453,#47454,#47455,#47456,#47457,
#47458,#47459,#47460,#47461,#47462,#47463,#47464,#47465,#47466,#47467,#47468,
#47469,#47470,#47471,#47472,#47473,#47474,#47475,#47476,#47477,#47478,#47479,
#47480,#47481,#47482,#47483,#47484,#47485,#47486,#47487,#47488,#47489,#47490,
#47491,#47492,#47493,#47494,#47495,#47496,#47497,#47498,#47499,#47500,#47501,
#47502,#47503,#47504,#47505,#47506,#47507,#47508,#47509,#47510,#47511,#47512,
#47513,#47514,#47515,#47516,#47517,#47518,#47519,#47520,#47521,#47522,#47523,
#47524,#47525,#47526,#47527,#47528,#47529,#47530,#47531,#47532,#47533,#47534,
#47535,#47536,#47537,#47538,#47539,#47540,#47541,#47542,#47543,#47544,#47545,
#47546,#47547,#47548,#47549,#47550,#47551,#47552,#47553,#47554,#47555,#47556,
#47557,#47558,#47559,#47560,#47561,#47562,#47563,#47564,#47565,#47566,#47567,
#47568),.UNSPECIFIED.,.F.,.F.,(4,2,2,2,2,2,2,2,2,2,2,2,2,2,2,2,2,2,2,2,
2,2,2,2,2,2,2,2,2,2,2,2,2,2,2,2,2,2,2,2,2,2,2,2,2,2,2,2,2,2,2,2,2,2,2,2,
2,2,2,2,2,2,2,2,2,2,2,2,2,2,2,2,2,2,2,2,2,2,2,2,2,2,2,2,2,2,2,2,2,2,2,2,
2,2,2,2,2,2,2,2,2,2,2,2,2,2,2,2,2,2,2,2,4),(-2.18949906292891,-2.1838650089922,
-2.18163622273672,-2.18039187561649,-2.17932165705407,-2.17795722915846,
-2.17515163526715,-2.15078142330274,-2.10153065279031,-2.08972730276351,
-2.08633112314776,-2.08422880749848,-2.08230367858015,-2.07984090766426,
-2.07579935338851,-2.04891117986127,-2.00021327939007,-1.99114088668074,
-1.98902302161969,-1.98780298306768,-1.98672898210937,-1.98535026184121,
-1.98307165100038,-1.96925110501733,-1.96033552537047,-1.91024334543028,
-1.89739515281065,-1.89389953573463,-1.89177517123471,-1.88985551632921,
-1.88739422344208,-1.8834468060302,-1.85979651054343,-1.81018684308953,
-1.79886699722579,-1.79660473021298,-1.79535302900298,-1.79428348427921,
-1.79292888830024,-1.79017321020061,-1.75727490009547,-1.73220967725323,
-1.70862182618849,-1.70287452413093,-1.70029132676813,-1.69835429837472,
-1.69653570234955,-1.69401452457364,-1.68747077470464,-1.64165405685319,
-1.6170585313395,-1.60631034109623,-1.60408118071565,-1.60283663173836,
-1.60176624395849,-1.60040160600074,-1.59759559923776,-1.57322502826008,
-1.52396442077986,-1.51215791530036,-1.5087610695415,-1.50665839230684,
-1.50473296609692,-1.50226986140283,-1.49822785870703,-1.47134306991988,
-1.42265799690053,-1.41355905152598,-1.41143901428331,-1.41021837699256,
-1.40914428396779,-1.40776600229934,-1.40548926104755,-1.39175626157772,
-1.38282361888464,-1.34832797823272,-1.33030636996907,-1.32310576586014,
-1.31766596056196,-1.31513921693266,-1.31321053141478,-1.31137441314844,
-1.30826436637587,-1.29979490709798,-1.29925333107365,-1.25003776607155,
-1.22305935265615,-1.21967214806597,-1.21819883416083,-1.2171148038492,
-1.21607845635969,-1.21427264755552,-1.20857237311552,-1.19919355257488,
-1.15742761264654,-1.1291123391115,-1.12503472450797,-1.12256091445563,
-1.12063370358738,-1.11853572832477,-1.11516116513808,-1.10358047589121,
-1.08380399239698,-1.0440534653287,-1.04245188977587,-1.0291650673599,-1.02691289616834,
-1.02552706368613,-1.02445459794764,-1.02322406119448,-1.02105937004265,
-1.01132613546075,-0.97396649970557),.UNSPECIFIED.);
#1318=B_SPLINE_CURVE_WITH_KNOTS('',3,(#47569,#47570,#47571,#47572,#47573,
#47574,#47575,#47576,#47577,#47578,#47579,#47580,#47581,#47582,#47583,#47584,
#47585,#47586,#47587,#47588,#47589,#47590,#47591,#47592,#47593,#47594,#47595,
#47596,#47597,#47598,#47599,#47600,#47601,#47602,#47603,#47604,#47605,#47606,
#47607,#47608,#47609,#47610,#47611,#47612,#47613,#47614,#47615,#47616,#47617,
#47618,#47619,#47620,#47621,#47622,#47623,#47624,#47625,#47626,#47627,#47628,
#47629,#47630,#47631,#47632,#47633,#47634,#47635,#47636,#47637,#47638,#47639,
#47640,#47641,#47642,#47643,#47644,#47645,#47646,#47647,#47648,#47649,#47650,
#47651,#47652,#47653,#47654,#47655,#47656,#47657,#47658,#47659,#47660,#47661,
#47662,#47663,#47664,#47665,#47666,#47667,#47668,#47669,#47670,#47671,#47672,
#47673,#47674,#47675,#47676,#47677,#47678,#47679,#47680,#47681,#47682,#47683,
#47684,#47685,#47686,#47687,#47688,#47689,#47690,#47691,#47692,#47693,#47694,
#47695,#47696,#47697,#47698,#47699,#47700,#47701,#47702,#47703,#47704,#47705,
#47706,#47707,#47708,#47709,#47710,#47711,#47712,#47713,#47714,#47715,#47716,
#47717,#47718,#47719,#47720,#47721,#47722,#47723,#47724,#47725,#47726,#47727,
#47728,#47729,#47730,#47731,#47732,#47733,#47734,#47735,#47736,#47737,#47738,
#47739,#47740,#47741,#47742,#47743,#47744,#47745,#47746,#47747,#47748,#47749,
#47750,#47751,#47752,#47753,#47754,#47755,#47756,#47757,#47758,#47759,#47760,
#47761,#47762,#47763,#47764,#47765,#47766,#47767,#47768,#47769,#47770,#47771,
#47772,#47773,#47774,#47775,#47776,#47777,#47778,#47779,#47780,#47781,#47782,
#47783,#47784,#47785,#47786,#47787,#47788,#47789,#47790),.UNSPECIFIED.,
 .F.,.F.,(4,2,2,2,2,2,2,2,2,2,2,2,2,2,2,2,2,2,2,2,2,2,2,2,2,2,2,2,2,2,2,
2,2,2,2,2,2,2,2,2,2,2,2,2,2,2,2,2,2,2,2,2,2,2,2,2,2,2,2,2,2,2,2,2,2,2,2,
2,2,2,2,2,2,2,2,2,2,2,2,2,2,2,2,2,2,2,2,2,2,2,2,2,2,2,2,2,2,2,2,2,2,2,2,
2,2,2,2,2,2,2,4),(-1.45815515730985,-1.44311106714501,-1.43866533437122,
-1.43633552712416,-1.43461173462009,-1.43246533009513,-1.42887016732215,
-1.41651973983777,-1.36941026717677,-1.35148688200421,-1.34261472047773,
-1.34051166933253,-1.33929488460142,-1.33822020196588,-1.33683604894193,
-1.33453902675744,-1.32029853381343,-1.31483766688885,-1.26395783223085,
-1.24919663170449,-1.24553987342171,-1.24337987025709,-1.2414667039106,
-1.23906584830869,-1.23531757631766,-1.21597119432106,-1.16386542523579,
-1.15073996967145,-1.14849586366893,-1.14711256823274,-1.14604051464259,
-1.14480869864457,-1.14263760631898,-1.13280530404366,-1.11166108054614,
-1.06076806319143,-1.05466226608335,-1.05221390748264,-1.05041414743598,
-1.0484651328367,-1.04580927574224,-1.03965074470046,-1.01274074458945,
-0.975751174046082,-0.972106143030279,-0.958288283245352,-0.956009703561393,
-0.954630986116154,-0.953556974136883,-0.952336896014332,-0.950218917922291,
-0.94114499006314,-0.892473640758535,-0.865595297937176,-0.861554049098209,
-0.859091280809838,-0.857166055288193,-0.855063535065136,-0.851666807129734,
-0.839859519543243,-0.790580579910545,-0.766198655561951,-0.763392508246637,
-0.762027904358827,-0.760957595598691,-0.759713190493695,-0.757484430253501,
-0.746740305406103,-0.722161659370576,-0.676369047836385,-0.669826827451264,
-0.667306007928953,-0.665487589227804,-0.663550674810742,-0.66096750956867,
-0.655219793739925,-0.63162419573825,-0.606543529041573,-0.573631955430268,
-0.570875896002742,-0.569521260885908,-0.568451760439797,-0.567200191055959,
-0.564938376631638,-0.553624558266521,-0.504065332566312,-0.480399575278229,
-0.476452113126949,-0.473990802682898,-0.472071153495024,-0.469946814942489,
-0.466451288270663,-0.453604246946545,-0.403483737066874,-0.381147891239907,
-0.378359998669721,-0.376999017612909,-0.37592901488986,-0.37468204864494,
-0.372441485254584,-0.361498098158943,-0.336112164974224,-0.291435410883938,
-0.284833521049669,-0.282303367205749,-0.280482509045716,-0.278546960999872,
-0.275972409223171,-0.270272090904166,-0.247042911606363,-0.242695174128374),
 .UNSPECIFIED.);
#1319=B_SPLINE_CURVE_WITH_KNOTS('',3,(#47796,#47797,#47798,#47799,#47800,
#47801,#47802,#47803,#47804,#47805,#47806,#47807,#47808,#47809,#47810,#47811,
#47812,#47813,#47814,#47815,#47816,#47817,#47818,#47819,#47820,#47821,#47822,
#47823,#47824,#47825,#47826,#47827,#47828,#47829,#47830,#47831,#47832,#47833,
#47834,#47835,#47836,#47837,#47838,#47839,#47840,#47841,#47842,#47843,#47844,
#47845,#47846,#47847,#47848,#47849,#47850,#47851,#47852,#47853,#47854,#47855,
#47856,#47857,#47858,#47859,#47860,#47861,#47862,#47863,#47864,#47865,#47866,
#47867,#47868,#47869,#47870,#47871,#47872,#47873,#47874,#47875,#47876,#47877,
#47878,#47879,#47880,#47881,#47882,#47883,#47884,#47885,#47886,#47887,#47888,
#47889,#47890,#47891,#47892,#47893,#47894,#47895,#47896,#47897,#47898,#47899,
#47900,#47901,#47902,#47903,#47904,#47905,#47906,#47907,#47908,#47909,#47910,
#47911,#47912,#47913,#47914,#47915,#47916,#47917,#47918,#47919,#47920,#47921,
#47922,#47923,#47924,#47925,#47926,#47927,#47928,#47929,#47930,#47931,#47932,
#47933,#47934,#47935,#47936,#47937,#47938,#47939,#47940,#47941,#47942,#47943,
#47944,#47945,#47946,#47947,#47948,#47949,#47950,#47951,#47952,#47953,#47954,
#47955,#47956,#47957,#47958,#47959,#47960,#47961,#47962,#47963,#47964,#47965,
#47966,#47967,#47968,#47969,#47970,#47971,#47972,#47973,#47974,#47975,#47976,
#47977),.UNSPECIFIED.,.F.,.F.,(4,2,2,2,2,2,2,2,2,2,2,2,2,2,2,2,2,2,2,2,
2,2,2,2,2,2,2,2,2,2,2,2,2,2,2,2,2,2,2,2,2,2,2,2,2,2,2,2,2,2,2,2,2,2,2,2,
2,2,2,2,2,2,2,2,2,2,2,2,2,2,2,2,2,2,2,2,2,2,2,2,2,2,2,2,2,2,2,2,2,2,4),
(-0.974174670753132,-0.9634387478963,-0.922534947998271,-0.908680419082317,
-0.906395898254317,-0.905015325265116,-0.903940954268919,-0.902721703837313,
-0.900607987060405,-0.89159499936821,-0.842865170768955,-0.815964168702849,
-0.811921841013154,-0.809458563378312,-0.80753302865571,-0.805430261039978,
-0.802033333848669,-0.790227404450901,-0.740946061260547,-0.716552111482368,
-0.713745467792079,-0.712380644009616,-0.711310173068138,-0.710065591037871,
-0.707836542352759,-0.697091576444547,-0.67251230267429,-0.626708770399057,
-0.620165826363481,-0.617644669076387,-0.615825987798593,-0.613888776131545,
-0.611305184223749,-0.605556392203509,-0.581955589606329,-0.556872547144106,
-0.523956906786774,-0.521200410334773,-0.519845567067463,-0.518775905501424,
-0.517524151110571,-0.515262011105729,-0.503946744883425,-0.454382696229716,
-0.430710883651648,-0.426762757290848,-0.424301055522499,-0.422381115143407,
-0.420256468606168,-0.416760467897113,-0.403912057978495,-0.353783679746306,
-0.344859167237714,-0.331031955283378,-0.328752719201692,-0.327373706518535,
-0.326299528299217,-0.32507933374179,-0.322961319235643,-0.313889751013021,
-0.265208494141045,-0.238325315169799,-0.23428346188979,-0.231820332296355,
-0.229894828515189,-0.228106666535456,-0.225163619444972,-0.216726004108841,
-0.203920218771785,-0.172858848314652,-0.158376967495467,-0.152739973468462,
-0.149077644592055,-0.138231396142488,-0.13611016384228,-0.134764044901729,
-0.133695047108698,-0.132436819832506,-0.130144541429449,-0.118274896887299,
-0.0813224857394244,-0.0677146962907497,-0.0597956969094492,-0.0447636751811699,
-0.0409592442672668,-0.0387442253970217,-0.0368363035725809,-0.0350092001075732,
-0.0327352983580613,-0.0292939652422515,-0.00056352101036781),
 .UNSPECIFIED.);
#1320=B_SPLINE_CURVE_WITH_KNOTS('',3,(#47978,#47979,#47980,#47981,#47982,
#47983,#47984,#47985,#47986,#47987,#47988,#47989,#47990,#47991,#47992,#47993,
#47994,#47995,#47996,#47997,#47998,#47999,#48000,#48001,#48002,#48003,#48004,
#48005,#48006,#48007,#48008,#48009,#48010,#48011,#48012,#48013,#48014,#48015,
#48016,#48017,#48018,#48019,#48020,#48021,#48022,#48023),.UNSPECIFIED.,
 .F.,.F.,(4,2,2,2,2,2,2,2,2,2,2,2,2,2,2,2,2,2,2,2,2,2,4),(-2.43136994263749,
-2.38857942322587,-2.37646857526415,-2.37416389819509,-2.37290310662602,
-2.37183447809935,-2.37049206108053,-2.36838263494433,-2.35772255734863,
-2.31573744321584,-2.294466988112,-2.28642387945132,-2.28054678715594,-2.27800435161223,
-2.27604735945959,-2.27425783159587,-2.27139336340267,-2.26446612094389,
-2.2627043812287,-2.26099926603054,-2.21920140266554,-2.19461115105961,
-2.18949906292891),.UNSPECIFIED.);
#1321=B_SPLINE_CURVE_WITH_KNOTS('',3,(#48025,#48026,#48027,#48028,#48029,
#48030,#48031,#48032,#48033,#48034,#48035,#48036,#48037,#48038,#48039,#48040,
#48041,#48042,#48043,#48044,#48045,#48046,#48047,#48048,#48049,#48050,#48051,
#48052,#48053,#48054,#48055,#48056,#48057,#48058,#48059,#48060,#48061,#48062,
#48063,#48064,#48065,#48066,#48067,#48068,#48069,#48070,#48071,#48072,#48073,
#48074,#48075,#48076,#48077,#48078,#48079,#48080,#48081,#48082,#48083,#48084),
 .UNSPECIFIED.,.F.,.F.,(4,2,2,2,2,2,2,2,2,2,2,2,2,2,2,2,2,2,2,2,2,2,2,2,
2,2,2,2,2,4),(-0.242695174128374,-0.221667875824946,-0.188612152567491,
-0.185857636448818,-0.184503315098143,-0.183464484460551,-0.183459264182677,
-0.183454111818551,-0.183449026147903,-0.183444005663323,-0.183439049352269,
-0.18343415586448,-0.183429324011531,-0.183424552649247,-0.183419840616554,
-0.183415186829067,-0.182181080759297,-0.180852488616711,-0.178781995938101,
-0.174829325467977,-0.128017800485001,-0.0957595023227357,-0.0916081614258372,
-0.0891131162241835,-0.0871832241910747,-0.0850961611120692,-0.0817692317479223,
-0.0706430063604701,-0.0519763481601277,-0.000564321818699808),
 .UNSPECIFIED.);
#1322=B_SPLINE_CURVE_WITH_KNOTS('',3,(#48085,#48086,#48087,#48088,#48089,
#48090,#48091,#48092,#48093,#48094,#48095,#48096,#48097,#48098,#48099,#48100,
#48101,#48102,#48103,#48104,#48105,#48106,#48107,#48108,#48109,#48110,#48111,
#48112,#48113,#48114,#48115,#48116,#48117,#48118,#48119,#48120,#48121,#48122,
#48123,#48124,#48125,#48126,#48127,#48128,#48129,#48130,#48131,#48132,#48133,
#48134,#48135,#48136,#48137,#48138,#48139,#48140,#48141,#48142,#48143,#48144,
#48145,#48146,#48147,#48148,#48149,#48150,#48151,#48152,#48153,#48154,#48155,
#48156,#48157,#48158,#48159,#48160,#48161,#48162,#48163,#48164,#48165,#48166,
#48167,#48168,#48169,#48170,#48171,#48172,#48173,#48174,#48175,#48176,#48177,
#48178,#48179,#48180,#48181,#48182,#48183,#48184,#48185,#48186,#48187,#48188,
#48189,#48190,#48191,#48192,#48193,#48194,#48195,#48196,#48197,#48198,#48199,
#48200,#48201,#48202,#48203,#48204,#48205,#48206,#48207,#48208,#48209,#48210,
#48211,#48212,#48213,#48214,#48215,#48216,#48217,#48218,#48219,#48220,#48221,
#48222,#48223,#48224,#48225,#48226,#48227,#48228,#48229,#48230,#48231,#48232,
#48233,#48234,#48235,#48236,#48237,#48238,#48239,#48240,#48241),
 .UNSPECIFIED.,.F.,.F.,(4,3,3,3,3,3,3,3,3,3,3,3,3,3,3,3,3,3,3,3,3,3,3,3,
3,3,3,3,3,3,3,3,3,3,3,3,3,3,3,3,3,3,3,3,3,3,3,3,3,3,3,3,4),(153.9380400259,
153.986061433838,154.091935315901,154.203101020456,154.308687775867,154.414210794711,
154.519706482428,154.625211202399,154.730829644781,154.836514123591,154.942377335347,
154.981260952343,155.087134834418,155.198300538972,155.303887294394,155.409410313251,
155.51490600098,155.620410720963,155.726029163356,155.831713642178,155.937576853946,
155.976460470847,156.082334352903,156.19350005746,156.299086812864,156.404609831702,
156.510105519413,156.615610239378,156.721228681754,156.826913160558,156.932776372309,
156.971659989352,157.077533871402,157.188699575959,157.294286331357,157.399809350189,
157.505305037892,157.610809757851,157.716428200219,157.822112679016,157.92797589076,
157.966859507857,158.07273338999,158.183899094536,158.289485850017,158.395008868932,
158.500504556718,158.606009276758,158.711627719208,158.817312198086,158.923175409909,
158.962059026361,158.969960932636),.UNSPECIFIED.);
#1323=B_SPLINE_CURVE_WITH_KNOTS('',3,(#48246,#48247,#48248,#48249,#48250,
#48251,#48252,#48253,#48254,#48255,#48256,#48257,#48258,#48259,#48260,#48261,
#48262,#48263,#48264,#48265,#48266,#48267,#48268,#48269,#48270,#48271,#48272,
#48273,#48274,#48275,#48276,#48277,#48278,#48279,#48280,#48281,#48282,#48283,
#48284,#48285,#48286,#48287,#48288,#48289,#48290,#48291,#48292,#48293,#48294,
#48295,#48296,#48297,#48298,#48299,#48300,#48301,#48302,#48303,#48304,#48305,
#48306,#48307,#48308,#48309,#48310,#48311,#48312,#48313,#48314,#48315,#48316,
#48317,#48318,#48319,#48320,#48321,#48322,#48323,#48324,#48325,#48326,#48327,
#48328,#48329,#48330,#48331,#48332,#48333,#48334,#48335,#48336,#48337,#48338,
#48339,#48340,#48341,#48342,#48343,#48344,#48345,#48346,#48347,#48348,#48349,
#48350,#48351,#48352,#48353,#48354,#48355,#48356,#48357,#48358,#48359,#48360,
#48361,#48362,#48363,#48364,#48365,#48366,#48367,#48368,#48369,#48370,#48371,
#48372,#48373,#48374,#48375,#48376,#48377,#48378,#48379,#48380,#48381,#48382,
#48383,#48384,#48385,#48386,#48387,#48388,#48389,#48390,#48391,#48392,#48393,
#48394,#48395,#48396,#48397,#48398,#48399,#48400,#48401,#48402,#48403,#48404,
#48405,#48406,#48407,#48408,#48409,#48410,#48411,#48412,#48413,#48414,#48415,
#48416,#48417,#48418,#48419,#48420,#48421,#48422,#48423,#48424,#48425,#48426,
#48427,#48428,#48429,#48430,#48431,#48432,#48433,#48434,#48435,#48436,#48437,
#48438,#48439,#48440,#48441,#48442,#48443,#48444,#48445,#48446,#48447,#48448,
#48449,#48450,#48451,#48452,#48453,#48454,#48455,#48456,#48457,#48458,#48459,
#48460,#48461,#48462,#48463,#48464,#48465,#48466,#48467,#48468,#48469,#48470,
#48471,#48472,#48473,#48474,#48475),.UNSPECIFIED.,.F.,.F.,(4,2,2,2,2,2,
2,2,2,2,2,2,2,2,2,2,2,2,2,2,2,2,2,2,2,2,2,2,2,2,2,2,2,2,2,2,2,2,2,2,2,2,
2,2,2,2,2,2,2,2,2,2,2,2,2,2,2,2,2,2,2,2,2,2,2,2,2,2,2,2,2,2,2,2,2,2,2,2,
2,2,2,2,2,2,2,2,2,2,2,2,2,2,2,2,2,2,2,2,2,2,2,2,2,2,2,2,2,2,2,2,2,2,2,2,
4),(-2.18940064281308,-2.17324077329001,-2.16143901298114,-2.15804337874734,
-2.15594141928606,-2.15401662894101,-2.15155430825681,-2.14751352942863,
-2.12063290814333,-2.07195154041407,-2.06287088315446,-2.0607526661771,
-2.05953268093726,-2.05845889606584,-2.05708067089078,-2.05480332804314,
-2.04106172224337,-2.02899930501495,-1.99673047286814,-1.97294744453886,
-1.96717565764364,-1.96458837116913,-1.9626510260713,-1.96083413186644,
-1.95831849451821,-1.95180754209415,-1.90549285637228,-1.88126409108669,
-1.87060922949552,-1.86838603843297,-1.86714295435572,-1.86607265609163,
-1.8647066178964,-1.86189262734673,-1.83643587887034,-1.8042409334404,-1.78048012410981,
-1.77471102086373,-1.77212412516464,-1.77018674989406,-1.7683695927781,
-1.76585321828434,-1.75933821327124,-1.71307730131563,-1.68880685303427,
-1.67814116167038,-1.67591722009928,-1.67467392709753,-1.67360358004846,
-1.6722376499123,-1.66942445955091,-1.64411367538752,-1.61180827260133,
-1.58801179027351,-1.58223794572398,-1.57965009899405,-1.57771247826308,
-1.57589543013712,-1.57337974598009,-1.56686962725001,-1.52052379582618,
-1.49630993073737,-1.48565828834039,-1.48343509997932,-1.4821919240161,
-1.4811214868796,-1.47975519484316,-1.47756743927912,-1.46554922553989,
-1.46041753794372,-1.42183749947843,-1.39590787138247,-1.38986717267425,
-1.38723180943733,-1.3852862970197,-1.38348159235791,-1.38101384680097,
-1.37479343072953,-1.32495224273226,-1.30630021147244,-1.29336314441733,
-1.29101746019944,-1.28974773989311,-1.28867952837314,-1.28734766856046,
-1.28527302782054,-1.2751548719539,-1.23243264931515,-1.21630057327133,
-1.20006270971042,-1.19616594145952,-1.19392979701521,-1.19221358907431,
-1.18999115510297,-1.18605015542787,-1.16702391464143,-1.11964043772659,
-1.11560984042451,-1.10120413887445,-1.09889995817399,-1.09751363668171,
-1.09643859637109,-1.09522289538876,-1.09312510277461,-1.08432429177742,
-1.066629920425,-1.03722858135862,-1.0085775388757,-1.00449249691808,-1.0020166049989,
-1.00008921775498,-0.99799250647038,-0.994623178058371,-0.983092297038724,
-0.974174670753132),.UNSPECIFIED.);
#1324=B_SPLINE_CURVE_WITH_KNOTS('',3,(#48477,#48478,#48479,#48480,#48481,
#48482,#48483,#48484,#48485,#48486,#48487,#48488,#48489,#48490,#48491,#48492,
#48493,#48494,#48495,#48496,#48497,#48498,#48499,#48500,#48501,#48502,#48503,
#48504,#48505,#48506,#48507,#48508,#48509,#48510,#48511,#48512,#48513),
 .UNSPECIFIED.,.F.,.F.,(4,3,3,3,3,3,3,3,3,3,3,3,4),(158.969960932636,159.075821542289,
159.186001167611,159.291582644725,159.397102766328,159.502597933955,159.608104509553,
159.713726266565,159.819416195121,159.925282860653,159.957258544866,160.090976876507,
160.22122533308),.UNSPECIFIED.);
#1325=B_SPLINE_CURVE_WITH_KNOTS('',3,(#48514,#48515,#48516,#48517,#48518,
#48519,#48520,#48521,#48522,#48523,#48524,#48525,#48526,#48527,#48528,#48529,
#48530,#48531,#48532,#48533,#48534,#48535,#48536,#48537,#48538,#48539,#48540,
#48541,#48542,#48543,#48544,#48545,#48546,#48547,#48548,#48549,#48550,#48551,
#48552,#48553,#48554,#48555,#48556,#48557,#48558,#48559,#48560,#48561,#48562,
#48563,#48564,#48565,#48566,#48567,#48568,#48569,#48570,#48571,#48572,#48573,
#48574,#48575,#48576,#48577,#48578,#48579,#48580,#48581,#48582,#48583,#48584,
#48585,#48586,#48587,#48588,#48589,#48590,#48591,#48592,#48593,#48594,#48595,
#48596,#48597,#48598,#48599,#48600,#48601,#48602,#48603,#48604,#48605,#48606,
#48607,#48608,#48609,#48610,#48611,#48612,#48613,#48614,#48615,#48616,#48617,
#48618,#48619,#48620,#48621,#48622,#48623,#48624,#48625,#48626,#48627,#48628,
#48629,#48630,#48631,#48632,#48633,#48634,#48635,#48636,#48637,#48638,#48639,
#48640,#48641,#48642,#48643,#48644,#48645,#48646,#48647,#48648,#48649,#48650,
#48651,#48652,#48653,#48654,#48655,#48656,#48657,#48658,#48659,#48660,#48661,
#48662,#48663,#48664,#48665,#48666,#48667,#48668,#48669,#48670,#48671,#48672,
#48673,#48674,#48675,#48676,#48677,#48678,#48679,#48680,#48681,#48682,#48683,
#48684,#48685,#48686,#48687,#48688,#48689,#48690,#48691,#48692,#48693),
 .UNSPECIFIED.,.F.,.F.,(4,2,2,2,2,2,2,2,2,2,2,2,2,2,2,2,2,2,2,2,2,2,2,2,
2,2,2,2,2,2,2,2,2,2,2,2,2,2,2,2,2,2,2,2,2,2,2,2,2,2,2,2,2,2,2,2,2,2,2,2,
2,2,2,2,2,2,2,2,2,2,2,2,2,2,2,2,2,2,2,2,2,2,2,2,2,2,2,2,2,4),(-2.43128894848558,
-2.40402165749699,-2.39373143610476,-2.39061926341053,-2.38848190111966,
-2.38639485731439,-2.38446536562597,-2.381971374362,-2.37782292549865,-2.34580085899753,
-2.32528912137062,-2.30423921586788,-2.29362190367919,-2.29139181401887,
-2.29014733693218,-2.28907738036556,-2.28771376932007,-2.28491147647599,
-2.2608355911699,-2.21142526738758,-2.20355201278584,-2.19776263617866,
-2.19517879997975,-2.19323359120059,-2.19142993049838,-2.18896479492237,
-2.18275705001053,-2.1324153038027,-2.11095636463804,-2.10118862433269,
-2.09892725589144,-2.09767596541003,-2.09660671859089,-2.09525243215069,
-2.09249716145065,-2.05961979425454,-2.03453719648145,-2.01096712398314,
-2.00522287890918,-2.00264067241323,-2.00070423422888,-1.9988860810328,
-1.99636533978075,-1.98982168574514,-1.94401719922651,-1.91943099357456,
-1.90868643179094,-1.90645793826304,-1.90521374980516,-1.90414366480947,
-1.90277940364899,-1.89997414073687,-1.87560501050664,-1.82636135044212,
-1.81456011900504,-1.81116442769963,-1.80906238900794,-1.80713749688047,
-1.80467500577902,-1.80063386151756,-1.77374535134339,-1.72504381292472,
-1.71598427736919,-1.71386753606527,-1.71264783961755,-1.71157393599248,
-1.71019507990167,-1.7079157081721,-1.69408155483174,-1.65317816574383,
-1.6335503869198,-1.62202963000177,-1.6186619369908,-1.61656594808735,-1.61463902552569,
-1.61216345251823,-1.60807830527806,-1.57939167990488,-1.54989364667247,
-1.53228040212644,-1.5235069661649,-1.52141160076482,-1.52019663410166,
-1.51912178188801,-1.51773512312131,-1.51542918186865,-1.50096896070186,
-1.49602903682948,-1.46162491485128,-1.45803638872278),.UNSPECIFIED.);
#1326=B_SPLINE_CURVE_WITH_KNOTS('',3,(#48699,#48700,#48701,#48702,#48703,
#48704,#48705,#48706,#48707,#48708,#48709,#48710,#48711,#48712,#48713,#48714,
#48715,#48716,#48717,#48718,#48719,#48720,#48721,#48722,#48723,#48724,#48725,
#48726,#48727,#48728,#48729,#48730,#48731,#48732,#48733,#48734,#48735,#48736,
#48737,#48738,#48739,#48740,#48741,#48742,#48743,#48744,#48745,#48746,#48747,
#48748,#48749,#48750,#48751,#48752,#48753,#48754,#48755,#48756,#48757,#48758,
#48759,#48760,#48761,#48762,#48763,#48764,#48765,#48766,#48767,#48768,#48769,
#48770,#48771,#48772,#48773,#48774,#48775,#48776,#48777,#48778,#48779,#48780,
#48781,#48782,#48783,#48784,#48785,#48786,#48787,#48788,#48789,#48790,#48791,
#48792,#48793,#48794,#48795,#48796,#48797,#48798,#48799,#48800,#48801,#48802,
#48803,#48804,#48805,#48806,#48807,#48808,#48809,#48810,#48811,#48812,#48813,
#48814,#48815,#48816,#48817,#48818,#48819,#48820,#48821,#48822,#48823,#48824,
#48825,#48826,#48827,#48828,#48829,#48830,#48831,#48832,#48833,#48834,#48835,
#48836,#48837,#48838,#48839,#48840,#48841,#48842,#48843,#48844,#48845,#48846,
#48847,#48848,#48849,#48850,#48851,#48852,#48853,#48854,#48855,#48856,#48857,
#48858,#48859,#48860,#48861,#48862,#48863,#48864,#48865,#48866,#48867,#48868,
#48869,#48870,#48871,#48872,#48873,#48874,#48875,#48876,#48877,#48878,#48879,
#48880,#48881,#48882,#48883,#48884,#48885,#48886,#48887,#48888,#48889,#48890,
#48891,#48892,#48893,#48894,#48895,#48896,#48897,#48898,#48899,#48900,#48901,
#48902,#48903,#48904),.UNSPECIFIED.,.F.,.F.,(4,2,2,2,2,2,2,2,2,2,2,2,2,
2,2,2,2,2,2,2,2,2,2,2,2,2,2,2,2,2,2,2,2,2,2,2,2,2,2,2,2,2,2,2,2,2,2,2,2,
2,2,2,2,2,2,2,2,2,2,2,2,2,2,2,2,2,2,2,2,2,2,2,2,2,2,2,2,2,2,2,2,2,2,2,2,
2,2,2,2,2,2,2,2,2,2,2,2,2,2,2,2,2,4),(-0.973787058187152,-0.971801940687298,
-0.960595339333787,-0.912180463585337,-0.887328913404492,-0.883346693228246,
-0.880875193661627,-0.878954635845838,-0.876836432945466,-0.873367354718714,
-0.86080253907915,-0.810461687935693,-0.807784069226913,-0.801407631248591,
-0.787603698148841,-0.785326082540803,-0.783947804096976,-0.782873995668262,
-0.781653932042932,-0.77953575922172,-0.770457641318477,-0.721794527897309,
-0.694920470067691,-0.690879506929976,-0.688416876728683,-0.686491736509972,
-0.684389285437468,-0.680992612966264,-0.669184854826154,-0.619903294147924,
-0.59553936461531,-0.592733518051818,-0.591368985761278,-0.590298723959279,
-0.589054378667964,-0.586825602932509,-0.576078994605386,-0.551488665258547,
-0.505721719980875,-0.499179053126231,-0.496658315310316,-0.4948400368633,
-0.492903347186302,-0.49032061117294,-0.484574393320205,-0.460988384462475,
-0.435903714829837,-0.402990880561689,-0.400235401362543,-0.398880976192795,
-0.397811604865909,-0.396560145736941,-0.394298429990437,-0.382983009438961,
-0.333398190501279,-0.309766546414575,-0.305820446084308,-0.303359692352746,
-0.301440297380349,-0.299316056740722,-0.29582026906562,-0.282967424203672,
-0.23285865727467,-0.210527785598441,-0.207739529436496,-0.206378568735993,
-0.20538523922618,-0.205380733840351,-0.205376324848768,-0.205372010222191,
-0.205367788043043,-0.205363656126608,-0.205359612456606,-0.205355996019009,
-0.205352397622671,-0.20534881725101,-0.205345254614244,-0.205341709628195,
-0.205338182293948,-0.204132906833308,-0.202029515594048,-0.199429825637415,
-0.193988040782058,-0.178178988109144,-0.136499636818045,-0.116920683751525,
-0.113161382794714,-0.110757150155002,-0.1088436693764,-0.106685836783518,
-0.10303889847966,-0.0884033904650566,-0.0384822875238028,-0.0286042439439895,
-0.020731486639263,-0.0161192246366164,-0.0143991075754617,-0.0133797956866168,
-0.0123611384337308,-0.0112848240284811,-0.00984155426457022,-0.00629937579403202,
-0.000566239655952785),.UNSPECIFIED.);
#1327=B_SPLINE_CURVE_WITH_KNOTS('',3,(#48905,#48906,#48907,#48908,#48909,
#48910,#48911,#48912,#48913,#48914,#48915,#48916,#48917,#48918,#48919,#48920,
#48921,#48922,#48923,#48924,#48925,#48926,#48927,#48928,#48929,#48930,#48931,
#48932,#48933,#48934,#48935,#48936,#48937,#48938,#48939,#48940,#48941,#48942,
#48943,#48944,#48945,#48946,#48947,#48948,#48949,#48950,#48951,#48952,#48953,
#48954,#48955,#48956,#48957,#48958,#48959,#48960,#48961,#48962,#48963,#48964,
#48965,#48966,#48967,#48968,#48969,#48970,#48971,#48972,#48973,#48974),
 .UNSPECIFIED.,.F.,.F.,(4,2,2,2,2,2,2,2,2,2,2,2,2,2,2,2,2,2,2,2,2,2,2,2,
2,2,2,2,2,2,2,2,2,2,4),(-2.43149354648851,-2.38992219825084,-2.35583090092751,
-2.35137061176593,-2.3490381223182,-2.34713050883852,-2.34492257878601,
-2.34114681995311,-2.32646952177799,-2.31789549330984,-2.27056566194237,
-2.26071202374391,-2.25675850045035,-2.25468785090749,-2.25335928637703,
-2.25212528419966,-2.25212070094854,-2.25211605802304,-2.25211135431886,
-2.25210658860967,-2.25210175976448,-2.25209686677358,-2.25209190816784,
-2.2520868826371,-2.25208178896488,-2.25207662590736,-2.25207139196767,
-2.2520660857715,-2.25206070583709,-2.25205525071632,-2.25101812014064,
-2.24965406848819,-2.24684966234465,-2.22248366788433,-2.18940064281308),
 .UNSPECIFIED.);
#1328=B_SPLINE_CURVE_WITH_KNOTS('',3,(#48975,#48976,#48977,#48978,#48979,
#48980,#48981,#48982,#48983,#48984,#48985,#48986,#48987,#48988,#48989,#48990,
#48991,#48992,#48993,#48994,#48995,#48996,#48997,#48998,#48999,#49000,#49001,
#49002,#49003,#49004,#49005,#49006,#49007,#49008,#49009,#49010,#49011,#49012,
#49013,#49014,#49015,#49016,#49017,#49018,#49019,#49020,#49021,#49022,#49023,
#49024,#49025,#49026,#49027,#49028,#49029,#49030,#49031,#49032,#49033,#49034,
#49035,#49036,#49037,#49038,#49039,#49040,#49041,#49042,#49043,#49044,#49045,
#49046,#49047,#49048,#49049,#49050,#49051,#49052,#49053,#49054,#49055,#49056,
#49057,#49058,#49059,#49060,#49061,#49062,#49063,#49064,#49065,#49066,#49067,
#49068,#49069,#49070,#49071,#49072,#49073,#49074,#49075,#49076,#49077,#49078,
#49079,#49080,#49081,#49082,#49083,#49084,#49085,#49086,#49087,#49088,#49089,
#49090,#49091,#49092,#49093,#49094,#49095,#49096,#49097,#49098,#49099,#49100,
#49101,#49102,#49103,#49104,#49105,#49106,#49107,#49108,#49109,#49110,#49111,
#49112,#49113,#49114,#49115,#49116,#49117,#49118,#49119,#49120,#49121,#49122,
#49123,#49124,#49125,#49126,#49127,#49128,#49129,#49130,#49131,#49132,#49133,
#49134,#49135,#49136,#49137,#49138,#49139,#49140,#49141,#49142,#49143,#49144,
#49145,#49146,#49147,#49148,#49149,#49150,#49151,#49152,#49153,#49154,#49155,
#49156,#49157,#49158,#49159,#49160,#49161,#49162,#49163,#49164,#49165,#49166,
#49167,#49168,#49169,#49170,#49171,#49172,#49173,#49174,#49175,#49176,#49177,
#49178,#49179,#49180,#49181,#49182,#49183,#49184,#49185,#49186,#49187,#49188,
#49189,#49190,#49191,#49192,#49193,#49194,#49195,#49196,#49197,#49198,#49199,
#49200),.UNSPECIFIED.,.F.,.F.,(4,2,2,2,2,2,2,2,2,2,2,2,2,2,2,2,2,2,2,2,
2,2,2,2,2,2,2,2,2,2,2,2,2,2,2,2,2,2,2,2,2,2,2,2,2,2,2,2,2,2,2,2,2,2,2,2,
2,2,2,2,2,2,2,2,2,2,2,2,2,2,2,2,2,2,2,2,2,2,2,2,2,2,2,2,2,2,2,2,2,2,2,2,
2,2,2,2,2,2,2,2,2,2,2,2,2,2,2,2,2,2,2,2,4),(-1.45803638872278,-1.44140955810846,
-1.4296534867198,-1.42626204032791,-1.42416078601136,-1.42223538283188,
-1.41977054438492,-1.41572192907757,-1.38905345093723,-1.34083188303034,
-1.33115650017217,-1.32899609162502,-1.32776669246211,-1.32669436926324,
-1.32530761571122,-1.32305177729499,-1.30967949560475,-1.27115914898039,
-1.24205315011539,-1.23563848956805,-1.23293901479649,-1.23098229959912,
-1.22919223408246,-1.22632517787012,-1.21938271153818,-1.21764312031094,
-1.21594715762074,-1.20052166719741,-1.15783440869433,-1.15376778767004,
-1.13935889970063,-1.13705478431023,-1.13566856520255,-1.13459364289385,
-1.13337811845707,-1.13128073068624,-1.12248307646172,-1.10479748624807,
-1.07538906341804,-1.04674257577078,-1.04265803567621,-1.04018243940552,
-1.03825527724496,-1.03615880572939,-1.0327898514745,-1.02126014157823,
-1.00160846489221,-0.960711118130644,-0.946850192664359,-0.944569636386252,
-0.943190312833635,-0.942116198371843,-0.940896425614768,-0.938779939005228,
-0.929726983933022,-0.881036635156126,-0.854150880649193,-0.850109336714403,
-0.847646441396319,-0.845721148342182,-0.843618586646655,-0.840221863469916,
-0.828415329485479,-0.779136643502452,-0.754750652140122,-0.75194438598397,
-0.750579733526155,-0.74950939152889,-0.748264953939066,-0.746036149132539,
-0.735292080389934,-0.71071426842235,-0.664917481742959,-0.658375171359847,
-0.655854289806948,-0.65403581763451,-0.652098838204596,-0.649515572455393,
-0.64376757539928,-0.620170461854027,-0.595089597553438,-0.56217733182469,
-0.559421166843357,-0.558066482533499,-0.556996940095799,-0.5557453144805,
-0.553483399505891,-0.542169078215479,-0.492606658186242,-0.46894245453169,
-0.46499491262841,-0.462533525070197,-0.460613798585893,-0.458489356844486,
-0.454993619330617,-0.442145320835569,-0.392023602689026,-0.369687981125468,
-0.366899631130225,-0.365538528973036,-0.364468487942502,-0.363221548241199,
-0.360981174973554,-0.350041577124906,-0.324671736470178,-0.279970060321373,
-0.273369105584581,-0.270839068375085,-0.269018219490698,-0.267082612598111,
-0.264507865315939,-0.258806630483864,-0.242686067170977),.UNSPECIFIED.);
#1329=B_SPLINE_CURVE_WITH_KNOTS('',3,(#49205,#49206,#49207,#49208,#49209,
#49210,#49211,#49212,#49213,#49214,#49215,#49216,#49217,#49218,#49219,#49220,
#49221,#49222,#49223,#49224,#49225,#49226,#49227,#49228,#49229,#49230,#49231,
#49232,#49233,#49234,#49235,#49236,#49237,#49238,#49239,#49240,#49241,#49242,
#49243,#49244,#49245,#49246,#49247,#49248,#49249,#49250,#49251,#49252,#49253,
#49254,#49255,#49256,#49257,#49258,#49259,#49260,#49261,#49262,#49263,#49264,
#49265,#49266,#49267,#49268,#49269,#49270,#49271,#49272,#49273,#49274,#49275,
#49276,#49277,#49278,#49279,#49280,#49281,#49282,#49283,#49284,#49285,#49286,
#49287,#49288,#49289,#49290,#49291,#49292,#49293,#49294,#49295,#49296,#49297,
#49298,#49299,#49300,#49301,#49302,#49303,#49304,#49305,#49306,#49307,#49308,
#49309,#49310,#49311,#49312,#49313,#49314,#49315,#49316,#49317,#49318,#49319,
#49320,#49321,#49322,#49323,#49324,#49325,#49326,#49327,#49328,#49329,#49330,
#49331,#49332,#49333,#49334,#49335,#49336,#49337,#49338,#49339,#49340,#49341,
#49342,#49343,#49344,#49345,#49346,#49347,#49348,#49349,#49350,#49351,#49352,
#49353,#49354,#49355,#49356,#49357,#49358,#49359,#49360,#49361,#49362,#49363,
#49364,#49365,#49366,#49367,#49368,#49369,#49370,#49371,#49372,#49373,#49374,
#49375,#49376,#49377,#49378,#49379,#49380,#49381,#49382,#49383,#49384,#49385,
#49386,#49387,#49388,#49389,#49390,#49391,#49392,#49393,#49394,#49395,#49396,
#49397,#49398,#49399,#49400,#49401,#49402,#49403,#49404,#49405,#49406,#49407,
#49408,#49409,#49410,#49411,#49412,#49413,#49414,#49415,#49416,#49417,#49418,
#49419,#49420,#49421,#49422,#49423,#49424,#49425,#49426,#49427,#49428,#49429,
#49430),.UNSPECIFIED.,.F.,.F.,(4,2,2,2,2,2,2,2,2,2,2,2,2,2,2,2,2,2,2,2,
2,2,2,2,2,2,2,2,2,2,2,2,2,2,2,2,2,2,2,2,2,2,2,2,2,2,2,2,2,2,2,2,2,2,2,2,
2,2,2,2,2,2,2,2,2,2,2,2,2,2,2,2,2,2,2,2,2,2,2,2,2,2,2,2,2,2,2,2,2,2,2,2,
2,2,2,2,2,2,2,2,2,2,2,2,2,2,2,2,2,2,2,2,4),(-2.18872254859161,-2.17002179167717,
-2.14518703702611,-2.13436880140523,-2.13213379750711,-2.13088725221948,
-2.1298202530721,-2.12846565382737,-2.12568523544807,-2.10286441602397,
-2.05273787376312,-2.04036827364099,-2.03693304534607,-2.0348319028284,
-2.03292456959959,-2.0304670764821,-2.02650167534777,-2.00157162747401,
-1.95288089662249,-1.94164785102387,-1.93940343155684,-1.93816201436535,
-1.93709567204078,-1.93574240420877,-1.93299254007081,-1.89988676028501,
-1.8744524822172,-1.85130855558775,-1.84561366357324,-1.84303709746159,
-1.84109817253612,-1.83927272957644,-1.83673388794344,-1.83009470939507,
-1.78675857011873,-1.76061031150067,-1.74948407283173,-1.74722745902251,
-1.74597424423193,-1.74490219310406,-1.74354187372541,-1.74137583650298,
-1.72977515162387,-1.72614881771714,-1.68511277778045,-1.65967148131973,
-1.65369141651281,-1.65106669689131,-1.64912295297693,-1.64731554730339,
-1.64483734031946,-1.63855528126412,-1.58929534984329,-1.56703951088787,
-1.55690152001526,-1.55471121639564,-1.55347563711939,-1.55240534684621,
-1.55103072082867,-1.54881253115325,-1.53617323809864,-1.53392130142186,
-1.52985906274059,-1.49432363324139,-1.47447130805812,-1.46286312171031,
-1.45948896163682,-1.45739307116101,-1.45546901860655,-1.45300100078151,
-1.44893669643834,-1.42102214697608,-1.3730010914805,-1.36426263461768,
-1.36217147279774,-1.36095827606882,-1.35988371443071,-1.3584964621511,
-1.35618846503178,-1.3416774818303,-1.33754025779713,-1.30077359602667,
-1.28164390005165,-1.27032487363905,-1.26697735413578,-1.26488545258997,
-1.26295655598157,-1.26047044261958,-1.25635052086089,-1.21563973324288,
-1.17521405567067,-1.1709811870584,-1.1693200889352,-1.16831190363125,-1.16720889430082,
-1.16562808483523,-1.16159118187243,-1.14076347097502,-1.09905033095437,
-1.07943385000551,-1.07567306488648,-1.07326852833733,-1.07135521780413,
-1.06919801497672,-1.06555320581034,-1.05094112500672,-1.0011947216004,
-0.980497079700009,-0.977732889705016,-0.976376773378501,-0.975307352126593,
-0.974057341062226,-0.973787058187152),.UNSPECIFIED.);
#1330=B_SPLINE_CURVE_WITH_KNOTS('',3,(#49432,#49433,#49434,#49435,#49436,
#49437,#49438,#49439,#49440,#49441,#49442,#49443,#49444,#49445,#49446,#49447,
#49448,#49449,#49450,#49451,#49452,#49453,#49454,#49455,#49456,#49457,#49458,
#49459,#49460,#49461,#49462,#49463,#49464,#49465,#49466,#49467,#49468,#49469,
#49470,#49471,#49472,#49473,#49474,#49475,#49476,#49477,#49478,#49479,#49480,
#49481,#49482,#49483),.UNSPECIFIED.,.F.,.F.,(4,2,2,2,2,2,2,2,2,2,2,2,2,
2,2,2,2,2,2,2,2,2,2,2,2,4),(-0.242686067170977,-0.235570833340653,-0.210241480296161,
-0.177143687126316,-0.174389806930583,-0.173035598851322,-0.17196612060904,
-0.171961294888966,-0.171956533088919,-0.171951833918979,-0.171947196490059,
-0.170712853535879,-0.168546913769349,-0.165816510750283,-0.159987017369551,
-0.142400060987175,-0.112933959948163,-0.0842115242191416,-0.0801252663193682,
-0.0776491721637786,-0.0757219466205869,-0.0736257326623009,-0.0702579098612493,
-0.0587391870800611,-0.0391146113794489,-0.000564882367464451),
 .UNSPECIFIED.);
#1331=B_SPLINE_CURVE_WITH_KNOTS('',3,(#49484,#49485,#49486,#49487,#49488,
#49489,#49490,#49491,#49492,#49493,#49494,#49495,#49496,#49497,#49498,#49499,
#49500,#49501,#49502,#49503,#49504,#49505,#49506,#49507,#49508,#49509,#49510,
#49511,#49512,#49513,#49514,#49515,#49516,#49517,#49518,#49519,#49520,#49521,
#49522,#49523,#49524,#49525,#49526,#49527,#49528,#49529,#49530,#49531,#49532,
#49533,#49534,#49535,#49536,#49537,#49538,#49539,#49540,#49541,#49542,#49543,
#49544,#49545,#49546,#49547,#49548,#49549,#49550,#49551,#49552,#49553,#49554,
#49555,#49556,#49557,#49558,#49559,#49560,#49561,#49562,#49563,#49564,#49565,
#49566,#49567,#49568,#49569,#49570,#49571,#49572,#49573,#49574,#49575,#49576,
#49577,#49578,#49579,#49580,#49581,#49582,#49583,#49584,#49585,#49586,#49587,
#49588,#49589,#49590,#49591,#49592,#49593,#49594,#49595,#49596,#49597,#49598,
#49599,#49600,#49601,#49602,#49603,#49604,#49605,#49606,#49607,#49608,#49609,
#49610,#49611,#49612,#49613,#49614,#49615,#49616,#49617,#49618,#49619,#49620,
#49621,#49622,#49623,#49624,#49625,#49626,#49627,#49628,#49629,#49630,#49631,
#49632,#49633,#49634),.UNSPECIFIED.,.F.,.F.,(4,3,3,3,3,3,3,3,3,3,3,3,3,
3,3,3,3,3,3,3,3,3,3,3,3,3,3,3,3,3,3,3,3,3,3,3,3,3,3,3,3,3,3,3,3,3,3,3,3,
3,4),(172.787595947439,172.894852285427,173.000727023252,173.111892620837,
173.217480244213,173.32300413316,173.428500691763,173.534006282056,173.639625588321,
173.745310928324,173.851174989247,173.890051803932,173.995923020582,174.107089058314,
174.212673151851,174.318193517071,174.423686563397,174.529188658208,174.63480451627,
174.740486431252,174.846347133457,174.885251322437,174.991127614625,175.102293017914,
175.207882130164,175.313407480416,175.418905470766,175.524412461228,175.63003311208,
175.735719766205,175.841585083887,175.880450840942,175.98632964872,176.097494737561,
176.203086517862,176.308614584271,176.414115334286,176.519625123373,176.625248612265,
176.730938130519,176.836806324186,176.875650359446,176.981508508061,177.0871824446,
177.192752734883,177.298255901997,177.403728384724,177.509271423133,177.61484564062,
177.720590257694,177.819192458502),.UNSPECIFIED.);
#1332=B_SPLINE_CURVE_WITH_KNOTS('',3,(#49638,#49639,#49640,#49641,#49642,
#49643,#49644,#49645,#49646,#49647,#49648,#49649,#49650,#49651,#49652,#49653,
#49654,#49655,#49656,#49657,#49658,#49659,#49660,#49661,#49662,#49663,#49664,
#49665,#49666,#49667,#49668,#49669,#49670,#49671,#49672,#49673,#49674,#49675,
#49676,#49677,#49678,#49679,#49680,#49681,#49682,#49683,#49684,#49685,#49686,
#49687,#49688,#49689,#49690,#49691,#49692,#49693,#49694,#49695,#49696,#49697,
#49698,#49699,#49700,#49701,#49702,#49703,#49704),.UNSPECIFIED.,.F.,.F.,
(4,3,3,3,3,3,3,3,3,3,3,3,3,3,3,3,3,3,3,3,3,3,4),(-4.03543298028442,-3.98079807401883,
-3.87997784099943,-3.77930285740571,-3.67874561621863,-3.57825284400111,
-3.47779351922475,-3.3773366620498,-3.27678386921224,-3.17618423154693,
-3.0754091542649,-2.98559855551413,-2.88484766263545,-2.78423921728324,
-2.68374404659775,-2.58331059978388,-2.48290779801925,-2.38250460150961,
-2.28200066564049,-2.18144732608841,-2.08071375859153,-1.99039903700942,
-1.98502202421793),.UNSPECIFIED.);
#1333=B_SPLINE_CURVE_WITH_KNOTS('',3,(#49708,#49709,#49710,#49711,#49712),
 .UNSPECIFIED.,.F.,.F.,(4,1,4),(0.,0.995199518504699,1.09118169752335),
 .UNSPECIFIED.);
#1334=B_SPLINE_CURVE_WITH_KNOTS('',3,(#49714,#49715,#49716,#49717,#49718,
#49719,#49720,#49721,#49722,#49723,#49724,#49725,#49726,#49727,#49728,#49729,
#49730,#49731,#49732,#49733,#49734,#49735,#49736,#49737,#49738,#49739,#49740,
#49741,#49742,#49743,#49744,#49745,#49746,#49747,#49748,#49749,#49750,#49751,
#49752,#49753,#49754,#49755,#49756,#49757,#49758,#49759,#49760,#49761,#49762,
#49763,#49764,#49765,#49766,#49767,#49768,#49769,#49770,#49771,#49772,#49773,
#49774,#49775,#49776,#49777,#49778,#49779,#49780,#49781,#49782,#49783,#49784,
#49785,#49786,#49787,#49788,#49789,#49790,#49791,#49792,#49793,#49794,#49795,
#49796,#49797,#49798,#49799,#49800,#49801,#49802,#49803,#49804,#49805,#49806,
#49807,#49808,#49809,#49810,#49811,#49812,#49813,#49814,#49815,#49816,#49817,
#49818,#49819,#49820,#49821,#49822,#49823,#49824,#49825,#49826,#49827,#49828,
#49829,#49830,#49831,#49832,#49833,#49834,#49835,#49836,#49837,#49838,#49839,
#49840,#49841,#49842,#49843,#49844,#49845,#49846,#49847,#49848,#49849,#49850,
#49851,#49852,#49853,#49854,#49855,#49856,#49857,#49858,#49859,#49860,#49861,
#49862,#49863,#49864,#49865,#49866,#49867,#49868,#49869,#49870,#49871,#49872,
#49873,#49874,#49875,#49876,#49877,#49878,#49879,#49880,#49881,#49882,#49883,
#49884,#49885,#49886,#49887,#49888,#49889,#49890,#49891,#49892,#49893,#49894,
#49895,#49896,#49897,#49898,#49899,#49900,#49901,#49902,#49903),
 .UNSPECIFIED.,.F.,.F.,(4,3,3,3,3,3,3,3,3,3,3,3,3,3,3,3,3,3,3,3,3,3,3,3,
3,3,3,3,3,3,3,3,3,3,3,3,3,3,3,3,3,3,3,3,3,3,3,3,3,3,3,3,3,3,3,3,3,3,3,3,
3,3,3,4),(1.09118169752335,1.18963615437418,1.28973151470358,1.38794123898432,
1.48609770063967,1.58423432078809,1.68577549984342,1.78403284001534,1.88721593851237,
1.99039903700941,2.09116037479013,2.19177691929166,2.29227662977098,2.39271244684173,
2.49311545338774,2.59351669119274,2.69401529414065,2.79456144284928,2.89528477765136,
2.98559855551411,3.08640030485475,3.18706082314412,3.28760969790442,3.38809782241632,
3.48855621210923,3.58901584426918,3.68957719963664,3.79018858726309,3.89098063411128,
3.98079807401882,4.08130696164147,4.18166936812423,4.28191363655008,4.38209334175167,
4.4822399338952,4.58238482155049,4.68262899353893,4.78292135853078,4.88339499444592,
4.97599759252353,5.07665610324085,5.17717000061932,5.27756785995971,5.37790236639782,
5.47820475574583,5.57850622331588,5.67890711758334,5.77935653576083,5.87998594870358,
5.97119711102824,6.07184943593958,6.17235746762015,6.27274997609054,6.3730794484051,
6.47337712835462,6.57367421953878,6.67407129617918,6.77451719672591,6.87514364485227,
6.96639662953295,7.077331363177,7.18794283858982,7.29800909371209,7.37436700431324),
 .UNSPECIFIED.);
#1335=B_SPLINE_CURVE_WITH_KNOTS('',3,(#49905,#49906,#49907,#49908,#49909,
#49910,#49911,#49912,#49913,#49914,#49915,#49916,#49917,#49918,#49919,#49920,
#49921,#49922,#49923,#49924,#49925,#49926,#49927,#49928,#49929,#49930,#49931,
#49932,#49933,#49934,#49935,#49936,#49937,#49938,#49939,#49940,#49941,#49942,
#49943,#49944,#49945,#49946,#49947,#49948,#49949,#49950,#49951,#49952,#49953,
#49954,#49955,#49956,#49957,#49958,#49959,#49960,#49961,#49962,#49963,#49964,
#49965,#49966,#49967,#49968,#49969,#49970,#49971,#49972,#49973,#49974,#49975,
#49976,#49977,#49978,#49979,#49980,#49981,#49982,#49983,#49984,#49985,#49986,
#49987,#49988,#49989,#49990,#49991,#49992,#49993,#49994,#49995,#49996,#49997,
#49998,#49999,#50000,#50001,#50002,#50003,#50004,#50005,#50006,#50007,#50008,
#50009,#50010,#50011,#50012,#50013,#50014,#50015,#50016,#50017,#50018,#50019,
#50020,#50021,#50022,#50023,#50024,#50025,#50026,#50027,#50028,#50029,#50030,
#50031,#50032,#50033,#50034,#50035,#50036,#50037,#50038,#50039,#50040,#50041,
#50042,#50043,#50044,#50045,#50046,#50047,#50048,#50049,#50050,#50051,#50052,
#50053,#50054,#50055,#50056,#50057,#50058,#50059,#50060,#50061,#50062,#50063,
#50064,#50065,#50066,#50067,#50068,#50069,#50070,#50071,#50072,#50073,#50074,
#50075,#50076,#50077,#50078,#50079,#50080,#50081,#50082,#50083,#50084,#50085,
#50086,#50087,#50088,#50089,#50090,#50091,#50092,#50093,#50094,#50095,#50096,
#50097),.UNSPECIFIED.,.F.,.F.,(4,3,3,3,3,3,3,3,3,3,3,3,3,3,3,3,3,3,3,3,
3,3,3,3,3,3,3,3,3,3,3,3,3,3,3,3,3,3,3,3,3,3,3,3,3,3,3,3,3,3,3,3,3,3,3,3,
3,3,3,3,3,3,3,3,4),(7.37436700470293,7.47623210060709,7.57814056338098,
7.68020247595503,7.78234477542899,7.88469717684685,7.96159614803766,8.06223414660923,
8.16272746632172,8.26310474994611,8.36341869192005,8.46370055755739,8.56398157169686,
8.66436226855847,8.76479159750012,8.86540134129867,8.95679566654237,9.05743094783625,
9.15792156441644,9.25829617966797,9.35860747576356,9.45888672184735,9.55916514661096,
9.65954332022051,9.75997015810087,9.86057749497037,9.95199518504709,10.0526261103251,
10.1531122834455,10.2534823443239,10.3537890205745,10.4540635877761,10.5543372809956,
10.6547106729914,10.7551326942182,10.8557352111616,10.9471947035518,11.0478287988039,
11.148318187236,11.2486915164575,11.3490014918313,11.4492793843046,11.54955642434,
11.6499331736749,11.7503585633559,11.8509644282025,11.9423942220565,12.0430276962745,
12.1435164614777,12.2438891671998,12.3441985192097,12.4444757893439,12.5447522089552,
12.6451283452818,12.7455531250382,12.8461583923753,12.9375937405612,13.0373122504327,
13.1368975488485,13.2363822102156,13.3357986874663,13.4352009865847,13.5345968719368,
13.6340503460223,13.6575523118825),.UNSPECIFIED.);
#1336=B_SPLINE_CURVE_WITH_KNOTS('',3,(#50099,#50100,#50101,#50102,#50103,
#50104,#50105,#50106,#50107,#50108,#50109,#50110,#50111,#50112,#50113,#50114,
#50115,#50116,#50117,#50118,#50119,#50120,#50121,#50122,#50123,#50124,#50125,
#50126,#50127,#50128,#50129,#50130,#50131,#50132,#50133,#50134,#50135,#50136,
#50137,#50138,#50139,#50140,#50141,#50142,#50143,#50144,#50145,#50146,#50147,
#50148,#50149,#50150,#50151,#50152,#50153,#50154,#50155,#50156,#50157,#50158,
#50159,#50160,#50161,#50162,#50163,#50164,#50165,#50166,#50167,#50168,#50169,
#50170,#50171,#50172,#50173,#50174,#50175,#50176,#50177,#50178,#50179,#50180,
#50181,#50182,#50183,#50184,#50185,#50186,#50187,#50188,#50189,#50190,#50191,
#50192,#50193,#50194,#50195,#50196,#50197,#50198,#50199,#50200,#50201,#50202,
#50203,#50204,#50205,#50206,#50207,#50208,#50209,#50210,#50211,#50212,#50213,
#50214,#50215,#50216,#50217,#50218,#50219,#50220,#50221,#50222,#50223,#50224,
#50225,#50226,#50227,#50228,#50229,#50230,#50231,#50232,#50233,#50234,#50235,
#50236,#50237,#50238,#50239,#50240,#50241,#50242,#50243,#50244,#50245,#50246,
#50247,#50248,#50249,#50250,#50251,#50252,#50253,#50254,#50255,#50256,#50257,
#50258,#50259,#50260,#50261,#50262,#50263,#50264,#50265,#50266,#50267,#50268,
#50269,#50270,#50271,#50272,#50273,#50274,#50275,#50276,#50277,#50278,#50279,
#50280,#50281,#50282,#50283,#50284,#50285,#50286,#50287,#50288,#50289,#50290,
#50291),.UNSPECIFIED.,.F.,.F.,(4,3,3,3,3,3,3,3,3,3,3,3,3,3,3,3,3,3,3,3,
3,3,3,3,3,3,3,3,3,3,3,3,3,3,3,3,3,3,3,3,3,3,3,3,3,3,3,3,3,3,3,3,3,3,3,3,
3,3,3,3,3,3,3,3,4),(13.6575523121158,13.7815219879644,13.9076259063269,
13.9327932590659,14.0334266816178,14.1339153909878,14.2342880348259,14.3345973212899,
14.4348745223014,14.5351508692947,14.6355269279752,14.7359516272088,14.8365568100598,
14.9279927775706,15.0286260828516,15.1291146740881,15.2294871990636,15.3297963662775,
15.4300734478205,15.5303496752957,15.6307256152235,15.7311501959341,15.8317552620445,
15.9231922960753,16.0238255491891,16.1243140869664,16.2246865567843,16.324995667831,
16.425272692275,16.525548861796,16.6259247428236,16.7263492640218,16.8269542702739,
16.9183918145801,17.019025128215,17.1195137274687,17.2198862599111,17.3201954342525,
17.4204725225729,17.5207487564637,17.6211247021888,17.7215492883672,17.8221543593193,
17.9135913330848,18.0142246266121,18.1147132055655,18.2150857175149,18.3153948712555,
18.4156719388965,18.5159481520584,18.6163240771223,18.7167486426438,18.8173536931884,
18.9087908515895,19.0094241403,19.1099127142906,19.2102852210797,19.3105943695423,
19.4108714317945,19.5111476394641,19.6115235589104,19.7119481187367,19.8125531635206,
19.9039903700942,19.9407376190621),.UNSPECIFIED.);
#1337=B_SPLINE_CURVE_WITH_KNOTS('',3,(#50293,#50294,#50295,#50296,#50297,
#50298,#50299,#50300,#50301,#50302,#50303,#50304,#50305,#50306,#50307,#50308,
#50309,#50310,#50311,#50312,#50313,#50314,#50315,#50316,#50317,#50318,#50319,
#50320,#50321,#50322,#50323,#50324,#50325,#50326,#50327,#50328,#50329,#50330,
#50331,#50332,#50333,#50334,#50335,#50336,#50337,#50338,#50339,#50340,#50341,
#50342,#50343,#50344,#50345,#50346,#50347,#50348,#50349,#50350,#50351,#50352,
#50353,#50354,#50355,#50356,#50357,#50358,#50359,#50360,#50361,#50362,#50363,
#50364,#50365,#50366,#50367,#50368,#50369,#50370,#50371,#50372,#50373,#50374,
#50375,#50376,#50377,#50378,#50379,#50380,#50381,#50382,#50383,#50384,#50385,
#50386,#50387,#50388,#50389,#50390,#50391,#50392,#50393,#50394,#50395,#50396,
#50397,#50398,#50399,#50400,#50401,#50402,#50403,#50404,#50405,#50406,#50407,
#50408,#50409,#50410,#50411,#50412,#50413,#50414,#50415,#50416,#50417,#50418,
#50419,#50420,#50421,#50422,#50423,#50424,#50425,#50426,#50427,#50428,#50429,
#50430,#50431,#50432,#50433,#50434,#50435,#50436,#50437,#50438,#50439,#50440,
#50441,#50442,#50443,#50444,#50445,#50446,#50447,#50448,#50449,#50450,#50451,
#50452,#50453,#50454,#50455,#50456,#50457,#50458,#50459,#50460,#50461,#50462,
#50463,#50464,#50465,#50466,#50467,#50468,#50469,#50470,#50471,#50472,#50473,
#50474,#50475,#50476,#50477,#50478,#50479,#50480,#50481,#50482),
 .UNSPECIFIED.,.F.,.F.,(4,3,3,3,3,3,3,3,3,3,3,3,3,3,3,3,3,3,3,3,3,3,3,3,
3,3,3,3,3,3,3,3,3,3,3,3,3,3,3,3,3,3,3,3,3,3,3,3,3,3,3,3,3,3,3,3,3,3,3,3,
3,3,3,4),(19.9407376193107,20.0407702233511,20.1406607870345,20.2404402949026,
20.3401604465629,20.4398532798881,20.539550795928,20.639349904067,20.739204086973,
20.8392274864441,20.8991898885989,20.9998231821237,21.1003117610257,21.2006842728501,
21.3009934264208,21.4012704938471,21.5015467067495,21.601922631485,21.7023471966396,
21.8029522467564,21.8943894071036,21.9950227003054,22.0955112788694,22.195883790334,
22.2961929435321,22.3964700105732,22.4967462230784,22.5971221474006,22.6975467121326,
22.7981517618153,22.8895889256083,22.990222219855,23.0907107994821,23.1910833120322,
23.2913924663288,23.3916695344803,23.4919457481059,23.5923216735563,23.6927462394227,
23.7933512902372,23.884788444113,23.9854217378588,24.0859103169787,24.1862828290149,
24.2865919827936,24.3868690504238,24.4871452635258,24.5875211884525,24.6879457537941,
24.7885508040885,24.8799879626177,24.9806212563667,25.0811098354885,25.1814823475244,
25.2817915013017,25.3820685689291,25.4823447820271,25.5827207069478,25.683145272282,
25.7837503225673,25.8751874811224,25.9913760242763,26.1076493578189,26.2239226913614),
 .UNSPECIFIED.);
#1338=B_SPLINE_CURVE_WITH_KNOTS('',3,(#50484,#50485,#50486,#50487,#50488,
#50489,#50490,#50491,#50492,#50493),.UNSPECIFIED.,.F.,.F.,(4,1,1,1,1,1,
1,4),(26.2239229262417,26.8703869996271,27.8655865181318,28.8607860366366,
29.8559855551413,30.851185073646,31.8463845921507,32.5071082334213),
 .UNSPECIFIED.);
#1339=B_SPLINE_CURVE_WITH_KNOTS('',3,(#50495,#50496,#50497,#50498,#50499,
#50500,#50501,#50502,#50503,#50504),.UNSPECIFIED.,.F.,.F.,(4,1,1,1,1,1,
1,4),(32.5071082334213,32.8415841106554,33.8367836291601,34.8319831476648,
35.8271826661695,36.8223821846742,37.8175817031789,38.7902935406009),
 .UNSPECIFIED.);
#1340=B_SPLINE_CURVE_WITH_KNOTS('',3,(#50506,#50507,#50508,#50509,#50510,
#50511,#50512,#50513,#50514,#50515,#50516),.UNSPECIFIED.,.F.,.F.,(4,1,1,
1,1,1,1,1,4),(38.7902935406009,38.8127812216836,39.8079807401883,40.803180258693,
41.7983797771977,42.7935792957025,43.7887788142072,44.7839783327119,45.0734788477805),
 .UNSPECIFIED.);
#1341=B_SPLINE_CURVE_WITH_KNOTS('',3,(#50518,#50519,#50520,#50521,#50522,
#50523,#50524,#50525,#50526,#50527),.UNSPECIFIED.,.F.,.F.,(4,1,1,1,1,1,
1,4),(45.0734788477805,45.7791778512166,46.7743773697213,47.769576888226,
48.7647764067307,49.7599759252354,50.7551754437401,51.35666415496),
 .UNSPECIFIED.);
#1342=B_SPLINE_CURVE_WITH_KNOTS('',3,(#50529,#50530,#50531,#50532,#50533,
#50534,#50535,#50536,#50537,#50538),.UNSPECIFIED.,.F.,.F.,(4,1,1,1,1,1,
1,4),(51.35666415496,51.7503749622449,52.7455744807496,53.7407739992543,
54.735973517759,55.7311730362637,56.7263725547684,57.6398494621397),
 .UNSPECIFIED.);
#1343=B_SPLINE_CURVE_WITH_KNOTS('',3,(#50540,#50541,#50542,#50543,#50544,
#50545,#50546,#50547,#50548,#50549,#50550),.UNSPECIFIED.,.F.,.F.,(4,1,1,
1,1,1,1,1,4),(57.6398494621397,57.7215720732731,58.7167715917778,59.7119711102825,
60.7071706287872,61.7023701472919,62.6975696657966,63.6927691843013,63.9230347693192),
 .UNSPECIFIED.);
#1344=B_SPLINE_CURVE_WITH_KNOTS('',3,(#50552,#50553,#50554,#50555,#50556,
#50557,#50558,#50559,#50560,#50561),.UNSPECIFIED.,.F.,.F.,(4,1,1,1,1,1,
1,4),(63.9230347693192,64.687968702806,65.6831682213108,66.6783677398155,
67.6735672583202,68.6687667768249,69.6639662953296,70.2062200764988),
 .UNSPECIFIED.);
#1345=B_SPLINE_CURVE_WITH_KNOTS('',3,(#50563,#50564,#50565,#50566,#50567,
#50568,#50569,#50570,#50571,#50572),.UNSPECIFIED.,.F.,.F.,(4,1,1,1,1,1,
1,4),(70.2062200764988,70.6591658138343,71.654365332339,72.6495648508437,
73.6447643693484,74.6399638878531,75.6351634063578,76.4893976728457),
 .UNSPECIFIED.);
#1346=B_SPLINE_CURVE_WITH_KNOTS('',3,(#50574,#50575,#50576,#50577,#50578,
#50579,#50580,#50581,#50582,#50583,#50584,#50585,#50586,#50587,#50588,#50589,
#50590,#50591,#50592,#50593,#50594,#50595,#50596,#50597,#50598,#50599,#50600,
#50601,#50602,#50603,#50604,#50605,#50606,#50607,#50608,#50609,#50610,#50611,
#50612,#50613,#50614,#50615,#50616,#50617,#50618,#50619,#50620,#50621,#50622,
#50623,#50624,#50625,#50626,#50627,#50628,#50629,#50630,#50631,#50632,#50633,
#50634,#50635,#50636,#50637,#50638,#50639,#50640,#50641,#50642,#50643,#50644,
#50645,#50646,#50647,#50648,#50649,#50650,#50651,#50652,#50653,#50654,#50655,
#50656,#50657,#50658,#50659,#50660,#50661,#50662,#50663,#50664,#50665,#50666,
#50667,#50668,#50669,#50670,#50671,#50672,#50673,#50674,#50675,#50676,#50677,
#50678,#50679,#50680,#50681,#50682,#50683,#50684,#50685,#50686,#50687,#50688,
#50689,#50690,#50691,#50692,#50693,#50694,#50695,#50696,#50697,#50698,#50699,
#50700,#50701,#50702,#50703,#50704,#50705,#50706,#50707,#50708,#50709,#50710,
#50711,#50712,#50713,#50714,#50715,#50716,#50717,#50718,#50719,#50720,#50721,
#50722,#50723,#50724,#50725,#50726,#50727,#50728,#50729,#50730,#50731,#50732,
#50733,#50734,#50735,#50736,#50737,#50738,#50739,#50740,#50741,#50742,#50743,
#50744,#50745,#50746,#50747,#50748,#50749,#50750,#50751,#50752,#50753,#50754,
#50755,#50756,#50757,#50758,#50759,#50760,#50761,#50762,#50763),
 .UNSPECIFIED.,.F.,.F.,(4,3,3,3,3,3,3,3,3,3,3,3,3,3,3,3,3,3,3,3,3,3,3,3,
3,3,3,3,3,3,3,3,3,3,3,3,3,3,3,3,3,3,3,3,3,3,3,3,3,3,3,3,3,3,3,3,3,3,3,3,
3,3,3,4),(76.4894053836784,76.6303629248626,76.7309962186831,76.8314847978778,
76.9318573099886,77.0321664638419,77.1324435315463,77.2327197447224,77.333095669722,
77.433520235136,77.534125285501,77.6255624433673,77.726195737188,77.826684316383,
77.9270568284941,78.0273659823476,78.1276430500524,78.2279192632286,78.3282951882285,
78.4287197536428,78.5293248040081,78.620761961872,78.7213952556924,78.8218838348872,
78.922256346998,79.0225655008513,79.1228425685558,79.2231187817318,79.3234947067314,
79.4239192721455,79.5245243225105,79.6159614803767,79.7165947741972,79.817083353392,
79.9174558655028,80.0177650193562,80.1180420870607,80.2183183002368,80.3186942252365,
80.4191187906506,80.5197238410157,80.6111609988814,80.711794292702,80.8122828718968,
80.9126553840076,81.0129645378611,81.1132416055656,81.2135178187418,81.3138937437415,
81.4143183091556,81.5149233595208,81.6063605173861,81.7069938112066,81.8074823904016,
81.9078549025124,82.0081640563658,82.1084411240703,82.2087173372464,82.309093262246,
82.4095178276602,82.5101228780253,82.6015600358908,82.7574881024976,82.772590690858),
 .UNSPECIFIED.);
#1347=B_SPLINE_CURVE_WITH_KNOTS('',3,(#50765,#50766,#50767,#50768,#50769,
#50770,#50771,#50772,#50773,#50774,#50775,#50776,#50777,#50778,#50779,#50780,
#50781,#50782,#50783,#50784,#50785,#50786,#50787,#50788,#50789,#50790,#50791,
#50792,#50793,#50794,#50795,#50796,#50797,#50798,#50799,#50800,#50801,#50802,
#50803,#50804,#50805,#50806,#50807,#50808,#50809,#50810,#50811,#50812,#50813,
#50814,#50815,#50816,#50817,#50818,#50819,#50820,#50821,#50822,#50823,#50824,
#50825,#50826,#50827,#50828,#50829,#50830,#50831,#50832,#50833,#50834,#50835,
#50836,#50837,#50838,#50839,#50840,#50841,#50842,#50843,#50844,#50845,#50846,
#50847,#50848,#50849,#50850,#50851,#50852,#50853,#50854,#50855,#50856,#50857,
#50858,#50859,#50860,#50861,#50862,#50863,#50864,#50865,#50866,#50867,#50868,
#50869,#50870,#50871,#50872,#50873,#50874,#50875,#50876,#50877,#50878,#50879,
#50880,#50881,#50882,#50883,#50884,#50885,#50886,#50887,#50888,#50889,#50890,
#50891,#50892,#50893,#50894,#50895,#50896,#50897,#50898,#50899,#50900,#50901,
#50902,#50903,#50904,#50905,#50906,#50907,#50908,#50909,#50910,#50911,#50912,
#50913,#50914,#50915,#50916,#50917,#50918,#50919,#50920,#50921,#50922,#50923,
#50924,#50925,#50926,#50927,#50928,#50929,#50930,#50931,#50932,#50933,#50934,
#50935,#50936,#50937,#50938,#50939,#50940,#50941,#50942,#50943,#50944,#50945,
#50946,#50947,#50948,#50949,#50950,#50951,#50952,#50953,#50954,#50955,#50956,
#50957),.UNSPECIFIED.,.F.,.F.,(4,3,3,3,3,3,3,3,3,3,3,3,3,3,3,3,3,3,3,3,
3,3,3,3,3,3,3,3,3,3,3,3,3,3,3,3,3,3,3,3,3,3,3,3,3,3,3,3,3,3,3,3,3,3,3,3,
3,3,3,3,3,3,3,3,4),(82.7725906911482,82.8756117990541,82.9744965836673,
83.0733239779893,83.1721269406444,83.2709383939143,83.3698510039825,83.4688238473439,
83.5679537129612,83.5967595543955,83.6973928482161,83.797881427411,83.8982539395219,
83.9985630933753,84.0988401610799,84.1991163742559,84.2994922992556,84.3999168646698,
84.500521915035,84.5919590729002,84.6925923667207,84.7930809459153,84.8934534580262,
84.9937626118795,85.0940396795841,85.19431589276,85.2946918177597,85.3951163831737,
85.4957214335389,85.5871585914049,85.6877918852255,85.7882804644204,85.8886529765312,
85.9889621303845,86.089239198089,86.1895154112653,86.2898913362649,86.390315901679,
86.4909209520441,86.5823581099096,86.6829914037301,86.7834799829251,86.8838524950361,
86.9841616488894,87.0844387165938,87.1847149297701,87.2850908547698,87.385515420184,
87.4861204705492,87.5775576284143,87.6781909222347,87.7786795014294,87.8790520135402,
87.9793611673935,88.0796382350979,88.1799144482744,88.280290373274,88.3807149386882,
88.4813199890532,88.572757146919,88.679242924783,88.7854091588012,88.8913805263008,
88.9970953238284,89.0557759977323),.UNSPECIFIED.);
#1348=B_SPLINE_CURVE_WITH_KNOTS('',3,(#50959,#50960,#50961,#50962,#50963,
#50964,#50965,#50966,#50967,#50968,#50969,#50970,#50971,#50972,#50973,#50974,
#50975,#50976,#50977,#50978,#50979,#50980,#50981,#50982,#50983,#50984,#50985,
#50986,#50987,#50988,#50989,#50990,#50991,#50992,#50993,#50994,#50995,#50996,
#50997,#50998,#50999,#51000,#51001,#51002,#51003,#51004,#51005,#51006,#51007,
#51008,#51009,#51010,#51011,#51012,#51013,#51014,#51015,#51016,#51017,#51018,
#51019,#51020,#51021,#51022,#51023,#51024,#51025,#51026,#51027,#51028,#51029,
#51030,#51031,#51032,#51033,#51034,#51035,#51036,#51037,#51038,#51039,#51040,
#51041,#51042,#51043,#51044,#51045,#51046,#51047,#51048,#51049,#51050,#51051,
#51052,#51053,#51054,#51055,#51056,#51057,#51058,#51059,#51060,#51061,#51062,
#51063,#51064,#51065,#51066,#51067,#51068,#51069,#51070,#51071,#51072,#51073,
#51074,#51075,#51076,#51077,#51078,#51079,#51080,#51081,#51082,#51083,#51084,
#51085,#51086,#51087,#51088,#51089,#51090,#51091,#51092,#51093,#51094,#51095,
#51096,#51097,#51098,#51099,#51100,#51101,#51102,#51103,#51104,#51105,#51106,
#51107,#51108,#51109,#51110,#51111,#51112,#51113,#51114,#51115,#51116,#51117,
#51118,#51119,#51120,#51121,#51122,#51123,#51124,#51125,#51126,#51127,#51128,
#51129,#51130,#51131,#51132,#51133,#51134,#51135,#51136,#51137,#51138,#51139,
#51140,#51141,#51142,#51143,#51144,#51145,#51146,#51147,#51148),
 .UNSPECIFIED.,.F.,.F.,(4,3,3,3,3,3,3,3,3,3,3,3,3,3,3,3,3,3,3,3,3,3,3,3,
3,3,3,3,3,3,3,3,3,3,3,3,3,3,3,3,3,3,3,3,3,3,3,3,3,3,3,3,3,3,3,3,3,3,3,3,
3,3,3,4),(89.0557759980376,89.1601699110528,89.264818149268,89.3695947912726,
89.4746481648271,89.5679566654238,89.6685899592442,89.7690785384391,89.8694510505499,
89.9697602044032,90.0700372721077,90.1703134852838,90.2706894102834,90.3711139756975,
90.4717190260625,90.5631561839285,90.6637894777491,90.764278056944,90.8646505690549,
90.9649597229083,91.0652367906129,91.1655130037891,91.2658889287888,91.366313494203,
91.4669185445681,91.5583557024332,91.6589889962538,91.7594775754488,91.8598500875596,
91.960159241413,92.0604363091175,92.1607125222936,92.2610884472932,92.3615130127074,
92.4621180630725,92.5535552209379,92.6541885147583,92.7546770939531,92.8550496060639,
92.9553587599173,93.0556358276219,93.155912040798,93.2562879657976,93.3567125312118,
93.4573175815769,93.5487547394426,93.6493880332632,93.7498766124577,93.8502491245687,
93.9505582784219,94.0508353461266,94.1511115593032,94.2514874843028,94.3519120497171,
94.4525171000822,94.5439542579473,94.6433301388161,94.7423600398394,94.841295548215,
94.9401696642849,95.0398675744382,95.1387542395913,95.2388577722446,95.3389613048979),
 .UNSPECIFIED.);
#1349=B_SPLINE_CURVE_WITH_KNOTS('',3,(#51150,#51151,#51152,#51153,#51154,
#51155,#51156,#51157,#51158,#51159,#51160,#51161,#51162,#51163,#51164,#51165,
#51166,#51167,#51168,#51169,#51170,#51171,#51172,#51173,#51174,#51175,#51176,
#51177,#51178,#51179,#51180,#51181,#51182,#51183,#51184,#51185,#51186,#51187,
#51188,#51189,#51190,#51191,#51192,#51193,#51194,#51195,#51196,#51197,#51198,
#51199,#51200,#51201,#51202,#51203,#51204,#51205,#51206,#51207,#51208,#51209,
#51210,#51211,#51212,#51213,#51214,#51215,#51216,#51217,#51218,#51219,#51220,
#51221,#51222,#51223,#51224,#51225,#51226,#51227,#51228,#51229,#51230,#51231,
#51232,#51233,#51234,#51235,#51236,#51237,#51238,#51239,#51240,#51241,#51242,
#51243,#51244,#51245,#51246,#51247,#51248,#51249,#51250,#51251,#51252,#51253,
#51254,#51255,#51256,#51257,#51258,#51259,#51260,#51261,#51262,#51263,#51264,
#51265,#51266,#51267,#51268,#51269,#51270,#51271,#51272,#51273,#51274,#51275,
#51276,#51277,#51278,#51279,#51280,#51281,#51282,#51283,#51284,#51285,#51286,
#51287,#51288,#51289,#51290,#51291,#51292,#51293,#51294,#51295,#51296,#51297,
#51298,#51299,#51300,#51301,#51302,#51303,#51304,#51305,#51306,#51307,#51308,
#51309,#51310,#51311,#51312,#51313,#51314,#51315,#51316,#51317,#51318,#51319,
#51320,#51321,#51322,#51323,#51324,#51325,#51326,#51327,#51328,#51329,#51330,
#51331,#51332,#51333,#51334,#51335,#51336,#51337,#51338,#51339),
 .UNSPECIFIED.,.F.,.F.,(4,3,3,3,3,3,3,3,3,3,3,3,3,3,3,3,3,3,3,3,3,3,3,3,
3,3,3,3,3,3,3,3,3,3,3,3,3,3,3,3,3,3,3,3,3,3,3,3,3,3,3,3,3,3,3,3,3,3,3,3,
3,3,3,4),(95.3389613052172,95.4822566433568,95.539153776452,95.6397870702726,
95.7402756494674,95.8406481615783,95.9409573154316,96.0412343831361,96.1415105963123,
96.241886521312,96.3423110867261,96.4429161370912,96.5343532949567,96.6349865887773,
96.7354751679722,96.8358476800831,96.9361568339365,97.0364339016411,97.1367101148173,
97.237086039817,97.3375106052312,97.4381156555964,97.5295528134614,97.6301861072819,
97.7306746864767,97.8310471985875,97.9313563524409,98.0316334201454,98.1319096333215,
98.2322855583211,98.3327101237352,98.4333151741003,98.5247523319661,98.6253856257866,
98.7258742049813,98.8262467170921,98.9265558709454,99.0268329386499,99.1271091518259,
99.2274850768255,99.3279096422396,99.4285146926046,99.5199518504708,99.6205851442916,
99.7210737234867,99.8214462355978,99.9217553894514,100.022032457156,100.122308670332,
100.222684595332,100.323109160747,100.423714211112,100.515151368976,100.615784662796,
100.716273241991,100.816645754102,100.916954907955,101.017231975659,101.117508188835,
101.217884113834,101.318308679248,101.418913729613,101.51035088748,101.622146612397),
 .UNSPECIFIED.);
#1350=B_SPLINE_CURVE_WITH_KNOTS('',3,(#51341,#51342,#51343,#51344,#51345,
#51346,#51347,#51348,#51349,#51350,#51351,#51352,#51353,#51354,#51355,#51356,
#51357,#51358,#51359,#51360,#51361,#51362,#51363,#51364,#51365,#51366,#51367,
#51368,#51369,#51370,#51371,#51372,#51373,#51374,#51375,#51376,#51377,#51378,
#51379,#51380,#51381,#51382,#51383,#51384,#51385,#51386,#51387,#51388,#51389,
#51390,#51391,#51392,#51393,#51394,#51395,#51396,#51397,#51398,#51399,#51400,
#51401,#51402,#51403,#51404,#51405,#51406,#51407,#51408,#51409,#51410,#51411,
#51412,#51413,#51414,#51415,#51416,#51417,#51418,#51419,#51420,#51421,#51422,
#51423,#51424,#51425,#51426,#51427,#51428,#51429,#51430,#51431,#51432,#51433,
#51434,#51435,#51436,#51437,#51438,#51439,#51440,#51441,#51442,#51443,#51444,
#51445,#51446,#51447,#51448,#51449,#51450,#51451,#51452,#51453,#51454,#51455,
#51456,#51457,#51458,#51459,#51460,#51461,#51462,#51463,#51464,#51465,#51466,
#51467,#51468,#51469,#51470,#51471,#51472,#51473,#51474,#51475,#51476,#51477,
#51478,#51479,#51480,#51481,#51482,#51483,#51484,#51485,#51486,#51487,#51488,
#51489,#51490,#51491,#51492,#51493,#51494,#51495,#51496,#51497,#51498,#51499,
#51500,#51501,#51502,#51503,#51504,#51505,#51506,#51507,#51508,#51509,#51510,
#51511,#51512,#51513,#51514,#51515,#51516,#51517,#51518,#51519,#51520,#51521,
#51522,#51523,#51524,#51525,#51526,#51527,#51528,#51529,#51530),
 .UNSPECIFIED.,.F.,.F.,(4,3,3,3,3,3,3,3,3,3,3,3,3,3,3,3,3,3,3,3,3,3,3,3,
3,3,3,3,3,3,3,3,3,3,3,3,3,3,3,3,3,3,3,3,3,3,3,3,3,3,3,3,3,3,3,3,3,3,3,3,
3,3,3,4),(101.622146612616,101.721379451865,101.820473882863,101.919491887866,
102.018466315808,102.11742995792,102.216482812235,102.31557830438,102.414849627253,
102.505550405985,102.606183699806,102.706672279001,102.807044791112,102.907353944965,
103.00763101267,103.107907225847,103.208283150846,103.308707716261,103.409312766626,
103.50074992449,103.60138321831,103.701871797505,103.802244309615,103.902553463469,
104.002830531173,104.103106744349,104.203482669348,104.303907234762,104.404512285127,
104.495949442994,104.596582736814,104.697071316009,104.79744382812,104.897752981973,
104.998030049678,105.098306262854,105.198682187854,105.299106753268,105.399711803633,
105.491148961499,105.59178225532,105.692270834515,105.792643346626,105.892952500479,
105.993229568184,106.09350578136,106.19388170636,106.294306271774,106.394911322139,
106.486348480004,106.586981773825,106.68747035302,106.787842865131,106.888152018984,
106.988429086689,107.088705299865,107.189081224865,107.289505790279,107.390110840645,
107.481547998509,107.591388936057,107.700941320827,107.810012207032,107.905331919234),
 .UNSPECIFIED.);
#1351=B_SPLINE_CURVE_WITH_KNOTS('',3,(#51532,#51533,#51534,#51535,#51536,
#51537,#51538,#51539,#51540,#51541,#51542,#51543,#51544,#51545,#51546,#51547,
#51548,#51549,#51550,#51551,#51552,#51553,#51554,#51555,#51556,#51557,#51558,
#51559,#51560,#51561,#51562,#51563,#51564,#51565,#51566,#51567,#51568,#51569,
#51570,#51571,#51572,#51573,#51574,#51575,#51576,#51577,#51578,#51579,#51580,
#51581,#51582,#51583,#51584,#51585,#51586,#51587,#51588,#51589,#51590,#51591,
#51592,#51593,#51594,#51595,#51596,#51597,#51598,#51599,#51600,#51601,#51602,
#51603,#51604,#51605,#51606,#51607,#51608,#51609,#51610,#51611,#51612,#51613,
#51614,#51615,#51616,#51617,#51618,#51619,#51620,#51621,#51622,#51623,#51624,
#51625,#51626,#51627,#51628,#51629,#51630,#51631,#51632,#51633,#51634,#51635,
#51636,#51637,#51638,#51639,#51640,#51641,#51642,#51643,#51644,#51645,#51646,
#51647,#51648,#51649,#51650,#51651,#51652,#51653,#51654,#51655,#51656,#51657,
#51658,#51659,#51660,#51661,#51662,#51663,#51664,#51665,#51666,#51667,#51668,
#51669,#51670,#51671,#51672,#51673,#51674,#51675,#51676,#51677,#51678,#51679,
#51680,#51681,#51682,#51683,#51684,#51685,#51686,#51687,#51688,#51689,#51690,
#51691,#51692,#51693,#51694,#51695,#51696,#51697,#51698,#51699,#51700,#51701,
#51702,#51703,#51704,#51705,#51706,#51707,#51708,#51709,#51710,#51711,#51712,
#51713,#51714,#51715,#51716,#51717,#51718,#51719,#51720,#51721,#51722,#51723,
#51724),.UNSPECIFIED.,.F.,.F.,(4,3,3,3,3,3,3,3,3,3,3,3,3,3,3,3,3,3,3,3,
3,3,3,3,3,3,3,3,3,3,3,3,3,3,3,3,3,3,3,3,3,3,3,3,3,3,3,3,3,3,3,3,3,3,3,3,
3,3,3,3,3,3,3,3,4),(107.905331919576,108.007663280982,108.110054337197,
108.212614455041,108.31526669938,108.418130027842,108.476747517013,108.577380810834,
108.677869390028,108.778241902139,108.878551055993,108.978828123697,109.079104336873,
109.179480261873,109.279904827287,109.380509877652,109.471947035518,109.572580329339,
109.673068908534,109.773441420645,109.873750574498,109.974027642203,110.074303855379,
110.174679780379,110.275104345793,110.375709396159,110.467146554023,110.567779847843,
110.668268427038,110.768640939148,110.868950093001,110.969227160706,111.069503373882,
111.169879298881,111.270303864295,111.37090891466,111.462346072527,111.562979366347,
111.663467945542,111.763840457653,111.864149611506,111.964426679211,112.064702892387,
112.165078817386,112.265503382801,112.366108433166,112.457545591032,112.558178884853,
112.658667464048,112.759039976159,112.859349130012,112.959626197717,113.059902410893,
113.160278335893,113.260702901308,113.361307951673,113.452745109537,113.552293832374,
113.651710936125,113.751029175624,113.850281183029,113.949525277683,114.048764705495,
114.148072690965,114.188517226756),.UNSPECIFIED.);
#1352=B_SPLINE_CURVE_WITH_KNOTS('',3,(#51726,#51727,#51728,#51729,#51730,
#51731,#51732,#51733,#51734,#51735,#51736,#51737,#51738,#51739,#51740,#51741,
#51742,#51743,#51744,#51745,#51746,#51747,#51748,#51749,#51750,#51751,#51752,
#51753,#51754,#51755,#51756,#51757,#51758,#51759,#51760,#51761,#51762,#51763,
#51764,#51765,#51766,#51767,#51768,#51769,#51770,#51771,#51772,#51773,#51774,
#51775,#51776,#51777,#51778,#51779,#51780,#51781,#51782,#51783,#51784,#51785,
#51786,#51787,#51788,#51789,#51790,#51791,#51792,#51793,#51794,#51795,#51796,
#51797,#51798,#51799,#51800,#51801,#51802,#51803,#51804,#51805,#51806,#51807,
#51808,#51809,#51810,#51811,#51812,#51813,#51814,#51815,#51816,#51817,#51818,
#51819,#51820,#51821,#51822,#51823,#51824,#51825,#51826,#51827,#51828,#51829,
#51830,#51831,#51832,#51833,#51834,#51835,#51836,#51837,#51838,#51839,#51840,
#51841,#51842,#51843,#51844,#51845,#51846,#51847,#51848,#51849,#51850,#51851,
#51852,#51853,#51854,#51855,#51856,#51857,#51858,#51859,#51860,#51861,#51862,
#51863,#51864,#51865,#51866,#51867,#51868,#51869,#51870,#51871,#51872,#51873,
#51874,#51875,#51876,#51877,#51878,#51879,#51880,#51881,#51882,#51883,#51884,
#51885,#51886,#51887,#51888,#51889,#51890,#51891,#51892,#51893,#51894,#51895,
#51896,#51897,#51898,#51899,#51900,#51901,#51902,#51903,#51904,#51905,#51906,
#51907,#51908,#51909,#51910,#51911,#51912,#51913,#51914,#51915),
 .UNSPECIFIED.,.F.,.F.,(4,3,3,3,3,3,3,3,3,3,3,3,3,3,3,3,3,3,3,3,3,3,3,3,
3,3,3,3,3,3,3,3,3,3,3,3,3,3,3,3,3,3,3,3,3,3,3,3,3,3,3,3,3,3,3,3,3,3,3,3,
3,3,3,4),(114.188517227063,114.318230927552,114.447944628041,114.548577921862,
114.649066501058,114.749439013169,114.849748167023,114.950025234728,115.050301447905,
115.150677372905,115.25110193832,115.351706988686,115.443144146546,115.543777440367,
115.644266019562,115.744638531672,115.844947685526,115.94522475323,116.045500966407,
116.145876891406,116.246301456821,116.346906507186,116.438343665051,116.538976958872,
116.639465538066,116.739838050177,116.840147204031,116.940424271735,117.040700484911,
117.141076409911,117.241500975325,117.34210602569,117.433543183556,117.534176477376,
117.634665056571,117.735037568682,117.835346722535,117.935623790239,118.035900003415,
118.136275928415,118.236700493829,118.337305544194,118.42874270206,118.52937599588,
118.629864575075,118.730237087186,118.830546241039,118.930823308744,119.03109952192,
119.13147544692,119.231900012334,119.332505062699,119.423942220565,119.524575514386,
119.625064093581,119.725436605692,119.825745759545,119.92602282725,120.026299040426,
120.126674965426,120.22709953084,120.327704581206,120.41914173907,120.471702533936),
 .UNSPECIFIED.);
#1353=B_SPLINE_CURVE_WITH_KNOTS('',3,(#51917,#51918,#51919,#51920,#51921,
#51922,#51923,#51924,#51925,#51926,#51927,#51928,#51929,#51930,#51931,#51932,
#51933,#51934,#51935,#51936,#51937,#51938,#51939,#51940,#51941,#51942,#51943,
#51944,#51945,#51946,#51947,#51948,#51949,#51950,#51951,#51952,#51953,#51954,
#51955,#51956,#51957,#51958,#51959,#51960,#51961,#51962,#51963,#51964,#51965,
#51966,#51967,#51968,#51969,#51970,#51971,#51972,#51973,#51974,#51975,#51976,
#51977,#51978,#51979,#51980,#51981,#51982,#51983,#51984,#51985,#51986,#51987,
#51988,#51989,#51990,#51991,#51992,#51993,#51994,#51995,#51996,#51997,#51998,
#51999,#52000,#52001,#52002,#52003,#52004,#52005,#52006,#52007,#52008,#52009,
#52010,#52011,#52012,#52013,#52014,#52015,#52016,#52017,#52018,#52019,#52020,
#52021,#52022,#52023,#52024,#52025,#52026,#52027,#52028,#52029,#52030,#52031,
#52032,#52033,#52034,#52035,#52036,#52037,#52038,#52039,#52040,#52041,#52042,
#52043,#52044,#52045,#52046,#52047,#52048,#52049,#52050,#52051,#52052,#52053,
#52054,#52055,#52056,#52057,#52058,#52059,#52060,#52061,#52062,#52063,#52064,
#52065,#52066,#52067,#52068,#52069,#52070,#52071,#52072,#52073,#52074,#52075,
#52076,#52077,#52078,#52079,#52080,#52081,#52082,#52083,#52084,#52085,#52086,
#52087,#52088,#52089,#52090,#52091,#52092,#52093,#52094,#52095,#52096,#52097,
#52098,#52099,#52100,#52101,#52102,#52103,#52104,#52105,#52106,#52107,#52108,
#52109),.UNSPECIFIED.,.F.,.F.,(4,3,3,3,3,3,3,3,3,3,3,3,3,3,3,3,3,3,3,3,
3,3,3,3,3,3,3,3,3,3,3,3,3,3,3,3,3,3,3,3,3,3,3,3,3,3,3,3,3,3,3,3,3,3,3,3,
3,3,3,3,3,3,3,3,4),(120.471702534264,120.571519365994,120.671196490433,
120.77076613455,120.870279000662,120.96976735932,121.069263446661,121.168862437348,
121.268519683046,121.368341435402,121.414341257574,121.514974551395,121.61546313059,
121.715835642701,121.816144796554,121.916421864259,122.016698077435,122.117074002435,
122.217498567849,122.318103618214,122.409540776079,122.5101740699,122.610662649095,
122.711035161206,122.811344315059,122.911621382764,123.01189759594,123.11227352094,
123.212698086354,123.313303136719,123.404740294584,123.505373588405,123.6058621676,
123.70623467971,123.806543833564,123.906820901268,124.007097114444,124.107473039444,
124.207897604858,124.308502655223,124.399939813089,124.500573106909,124.601061686104,
124.701434198214,124.801743352067,124.902020419772,125.002296632948,125.102672557947,
125.203097123361,125.303702173726,125.395139331593,125.495772625413,125.596261204608,
125.696633716719,125.796942870573,125.897219938277,125.997496151453,126.097872076453,
126.198296641867,126.298901692233,126.390338850098,126.504950337584,126.619096027427,
126.732458632805,126.754887840888),.UNSPECIFIED.);
#1354=B_SPLINE_CURVE_WITH_KNOTS('',3,(#52111,#52112,#52113,#52114,#52115,
#52116,#52117,#52118,#52119,#52120,#52121,#52122,#52123,#52124,#52125,#52126,
#52127,#52128,#52129,#52130,#52131,#52132,#52133,#52134,#52135,#52136,#52137,
#52138,#52139,#52140,#52141,#52142,#52143,#52144,#52145,#52146,#52147,#52148,
#52149,#52150,#52151,#52152,#52153,#52154,#52155,#52156,#52157,#52158,#52159,
#52160,#52161,#52162,#52163,#52164,#52165,#52166,#52167,#52168,#52169,#52170,
#52171,#52172,#52173,#52174,#52175,#52176,#52177,#52178,#52179,#52180,#52181,
#52182,#52183,#52184,#52185,#52186,#52187,#52188,#52189,#52190,#52191,#52192,
#52193,#52194,#52195,#52196,#52197,#52198,#52199,#52200,#52201,#52202,#52203,
#52204,#52205,#52206,#52207,#52208,#52209,#52210,#52211,#52212,#52213,#52214,
#52215,#52216,#52217,#52218,#52219,#52220,#52221,#52222,#52223,#52224,#52225,
#52226,#52227,#52228,#52229,#52230,#52231,#52232,#52233,#52234,#52235,#52236,
#52237,#52238,#52239,#52240,#52241,#52242,#52243,#52244,#52245,#52246,#52247,
#52248,#52249,#52250,#52251,#52252,#52253,#52254,#52255,#52256,#52257,#52258,
#52259,#52260,#52261,#52262,#52263,#52264,#52265,#52266,#52267,#52268,#52269,
#52270,#52271,#52272,#52273,#52274,#52275,#52276,#52277,#52278,#52279,#52280,
#52281,#52282,#52283,#52284,#52285,#52286,#52287,#52288,#52289,#52290,#52291,
#52292,#52293,#52294,#52295,#52296,#52297,#52298,#52299,#52300,#52301,#52302,
#52303),.UNSPECIFIED.,.F.,.F.,(4,3,3,3,3,3,3,3,3,3,3,3,3,3,3,3,3,3,3,3,
3,3,3,3,3,3,3,3,3,3,3,3,3,3,3,3,3,3,3,3,3,3,3,3,3,3,3,3,3,3,3,3,3,3,3,3,
3,3,3,3,3,3,3,3,4),(126.754887841115,126.855723392772,126.956565229927,
127.057443412667,127.158455072141,127.259546174342,127.360812752503,127.385538368603,
127.486171662423,127.586660241617,127.687032753728,127.787341907581,127.887618975285,
127.987895188461,128.08827111346,128.188695678874,128.289300729239,128.380737887107,
128.481371180928,128.581859760122,128.682232272233,128.782541426087,128.882818493791,
128.983094706967,129.083470631967,129.183895197381,129.284500247746,129.375937405612,
129.476570699433,129.577059278628,129.677431790739,129.777740944592,129.878018012297,
129.978294225474,130.078670150473,130.179094715888,130.279699766253,130.371136924117,
130.471770217938,130.572258797132,130.672631309243,130.772940463097,130.873217530801,
130.973493743977,131.073869668977,131.174294234391,131.274899284756,131.366336442622,
131.466969736442,131.567458315637,131.667830827747,131.768139981601,131.868417049305,
131.96869326248,132.06906918748,132.169493752893,132.270098803258,132.361535961126,
132.461872922284,132.562070807988,132.662161436375,132.762184969317,132.862166822976,
132.962174894668,133.038073148295),.UNSPECIFIED.);
#1355=B_SPLINE_CURVE_WITH_KNOTS('',3,(#52305,#52306,#52307,#52308,#52309,
#52310,#52311,#52312,#52313,#52314,#52315,#52316,#52317,#52318,#52319,#52320,
#52321,#52322,#52323,#52324,#52325,#52326,#52327,#52328,#52329,#52330,#52331,
#52332,#52333,#52334,#52335,#52336,#52337,#52338,#52339,#52340,#52341,#52342,
#52343,#52344,#52345,#52346,#52347,#52348,#52349,#52350,#52351,#52352,#52353,
#52354,#52355,#52356,#52357,#52358,#52359,#52360,#52361,#52362,#52363,#52364,
#52365,#52366,#52367,#52368,#52369,#52370,#52371,#52372,#52373,#52374,#52375,
#52376,#52377,#52378,#52379,#52380,#52381,#52382,#52383,#52384,#52385,#52386,
#52387,#52388,#52389,#52390,#52391,#52392,#52393,#52394,#52395,#52396,#52397,
#52398,#52399,#52400,#52401,#52402,#52403,#52404,#52405,#52406,#52407,#52408,
#52409,#52410,#52411,#52412,#52413,#52414,#52415,#52416,#52417,#52418,#52419,
#52420,#52421,#52422,#52423,#52424,#52425,#52426,#52427,#52428,#52429,#52430,
#52431,#52432,#52433,#52434,#52435,#52436,#52437,#52438,#52439,#52440,#52441,
#52442,#52443,#52444,#52445,#52446,#52447,#52448,#52449,#52450,#52451,#52452,
#52453,#52454,#52455,#52456,#52457,#52458,#52459,#52460,#52461,#52462,#52463,
#52464,#52465,#52466,#52467,#52468,#52469,#52470,#52471,#52472,#52473,#52474,
#52475,#52476,#52477,#52478,#52479,#52480,#52481,#52482,#52483,#52484,#52485,
#52486,#52487,#52488,#52489,#52490,#52491,#52492,#52493,#52494),
 .UNSPECIFIED.,.F.,.F.,(4,3,3,3,3,3,3,3,3,3,3,3,3,3,3,3,3,3,3,3,3,3,3,3,
3,3,3,3,3,3,3,3,3,3,3,3,3,3,3,3,3,3,3,3,3,3,3,3,3,3,3,3,3,3,3,3,3,3,3,3,
3,3,3,4),(133.03807314869,133.156219331711,133.275714063615,133.356735479631,
133.457368773452,133.557857352647,133.658229864758,133.758539018612,133.858816086317,
133.959092299493,134.059468224493,134.159892789908,134.260497840273,134.351934998136,
134.452568291956,134.553056871151,134.653429383261,134.753738537115,134.854015604819,
134.954291817995,135.054667742994,135.155092308408,135.255697358773,135.34713451664,
135.447767810461,135.548256389655,135.648628901766,135.74893805562,135.849215123324,
135.9494913365,136.0498672615,136.150291826914,136.250896877279,136.342334035145,
136.442967328966,136.543455908161,136.643828420272,136.744137574125,136.84441464183,
136.944690855007,137.045066780006,137.145491345421,137.246096395786,137.33753355365,
137.43816684747,137.538655426665,137.639027938776,137.739337092629,137.839614160334,
137.93989037351,138.040266298509,138.140690863923,138.241295914288,138.332733072154,
138.433247204163,138.533616703136,138.633870529462,138.73406141901,138.834220810923,
138.934380104271,139.034639201367,139.134947940025,139.235434997304,139.321258455253),
 .UNSPECIFIED.);
#1356=B_SPLINE_CURVE_WITH_KNOTS('',3,(#52496,#52497,#52498,#52499,#52500,
#52501,#52502,#52503,#52504,#52505,#52506,#52507,#52508,#52509,#52510,#52511,
#52512,#52513,#52514,#52515,#52516,#52517,#52518,#52519,#52520,#52521,#52522,
#52523,#52524,#52525,#52526,#52527,#52528,#52529,#52530,#52531,#52532,#52533,
#52534,#52535,#52536,#52537,#52538,#52539,#52540,#52541,#52542,#52543,#52544,
#52545,#52546,#52547,#52548,#52549,#52550,#52551,#52552,#52553,#52554,#52555,
#52556,#52557,#52558,#52559,#52560,#52561,#52562,#52563,#52564,#52565,#52566,
#52567,#52568,#52569,#52570,#52571,#52572,#52573,#52574,#52575,#52576,#52577,
#52578,#52579,#52580,#52581,#52582,#52583,#52584,#52585,#52586,#52587,#52588,
#52589,#52590,#52591,#52592,#52593,#52594,#52595,#52596,#52597,#52598,#52599,
#52600,#52601,#52602,#52603,#52604,#52605,#52606,#52607,#52608,#52609,#52610,
#52611,#52612,#52613,#52614,#52615,#52616,#52617,#52618,#52619,#52620,#52621,
#52622,#52623,#52624,#52625,#52626,#52627,#52628,#52629,#52630,#52631,#52632,
#52633,#52634,#52635,#52636,#52637,#52638,#52639,#52640,#52641,#52642,#52643,
#52644,#52645,#52646,#52647,#52648,#52649,#52650,#52651,#52652,#52653,#52654,
#52655,#52656,#52657,#52658,#52659,#52660,#52661,#52662,#52663,#52664,#52665,
#52666,#52667,#52668,#52669,#52670,#52671,#52672,#52673,#52674,#52675,#52676,
#52677,#52678,#52679,#52680,#52681,#52682,#52683,#52684,#52685,#52686,#52687,
#52688),.UNSPECIFIED.,.F.,.F.,(4,3,3,3,3,3,3,3,3,3,3,3,3,3,3,3,3,3,3,3,
3,3,3,3,3,3,3,3,3,3,3,3,3,3,3,3,3,3,3,3,3,3,3,3,3,3,3,3,3,3,3,3,3,3,3,3,
3,3,3,3,3,3,3,3,4),(139.321258455474,139.327932590659,139.428565884479,
139.529054463673,139.629426975784,139.729736129637,139.830013197341,139.930289410516,
140.030665335515,140.131089900929,140.231694951294,140.323132109164,140.423765402986,
140.524253982182,140.624626494294,140.724935648149,140.825212715855,140.925488929032,
141.025864854033,141.126289419449,141.226894469815,141.318331627669,141.418964921488,
141.519453500682,141.619826012792,141.720135166644,141.820412234348,141.920688447523,
142.021064372521,142.121488937934,142.222093988298,142.313531146173,142.414164439991,
142.514653019183,142.615025531291,142.715334685142,142.815611752844,142.915887966017,
143.016263891014,143.116688456426,143.217293506788,143.308730664678,143.409363958508,
143.509852537712,143.610225049831,143.710534203694,143.810811271407,143.911087484593,
144.011463409601,144.111887975024,144.212493025398,144.303930183183,144.404563476994,
144.50505205618,144.605424568282,144.705733722127,144.806010789822,144.90628700299,
145.006662927981,145.107087493387,145.207692543744,145.299129701687,145.420579631092,
145.540533774723,145.604443762298),.UNSPECIFIED.);
#1357=B_SPLINE_CURVE_WITH_KNOTS('',3,(#52690,#52691,#52692,#52693,#52694,
#52695,#52696,#52697,#52698,#52699,#52700,#52701,#52702,#52703,#52704,#52705,
#52706,#52707,#52708,#52709,#52710,#52711,#52712,#52713,#52714,#52715,#52716,
#52717,#52718,#52719,#52720,#52721,#52722,#52723,#52724,#52725,#52726,#52727,
#52728,#52729,#52730,#52731,#52732,#52733,#52734,#52735,#52736,#52737,#52738,
#52739,#52740,#52741,#52742,#52743,#52744,#52745,#52746,#52747,#52748,#52749,
#52750,#52751,#52752,#52753,#52754,#52755,#52756,#52757,#52758,#52759,#52760,
#52761,#52762,#52763,#52764,#52765,#52766,#52767,#52768,#52769,#52770,#52771,
#52772,#52773,#52774,#52775,#52776,#52777,#52778,#52779,#52780,#52781,#52782,
#52783,#52784,#52785,#52786,#52787,#52788,#52789,#52790,#52791,#52792,#52793,
#52794,#52795,#52796,#52797,#52798,#52799,#52800,#52801,#52802,#52803,#52804,
#52805,#52806,#52807,#52808,#52809,#52810,#52811,#52812,#52813,#52814,#52815,
#52816,#52817,#52818,#52819,#52820,#52821,#52822,#52823,#52824,#52825,#52826,
#52827,#52828,#52829,#52830,#52831,#52832,#52833,#52834,#52835,#52836,#52837,
#52838,#52839,#52840,#52841,#52842,#52843,#52844,#52845,#52846,#52847,#52848,
#52849,#52850,#52851,#52852,#52853,#52854,#52855,#52856,#52857,#52858,#52859,
#52860,#52861,#52862,#52863,#52864,#52865,#52866,#52867,#52868,#52869,#52870,
#52871,#52872,#52873,#52874,#52875,#52876,#52877,#52878,#52879),
 .UNSPECIFIED.,.F.,.F.,(4,3,3,3,3,3,3,3,3,3,3,3,3,3,3,3,3,3,3,3,3,3,3,3,
3,3,3,3,3,3,3,3,3,3,3,3,3,3,3,3,3,3,3,3,3,3,3,3,3,3,3,3,3,3,3,3,3,3,3,3,
3,3,3,4),(145.604443762654,145.704257784809,145.804039315887,145.903820193958,
146.003702819992,146.103635283292,146.203751666778,146.294329220192,146.394962514076,
146.495451093335,146.59582360551,146.696132759426,146.796409827195,146.896686040434,
146.997061965496,147.097486530972,147.198091581398,147.289528738697,147.390162032438,
147.490650611553,147.591023123586,147.691332277361,147.791609344988,147.891885558087,
147.992261483012,148.092686048352,148.193291098645,148.284728257202,148.385361550952,
148.485850130075,148.586222642113,148.686531795893,148.786808863523,148.887085076624,
148.987461001549,149.087885566887,149.188490617177,149.279927775706,149.380561069975,
149.481049649619,149.581422162179,149.681731316481,149.782008384634,149.882284598256,
149.982660523697,150.083085089549,150.183690140343,150.275127294211,150.37576058735,
150.476249165865,150.576621677301,150.676930830484,150.777207897522,150.877484110037,
150.977860034389,151.078284599162,151.178889648903,151.270326812716,151.37189564131,
151.473312380576,151.57689155289,151.678083381926,151.78285622588,151.887629069833),
 .UNSPECIFIED.);
#1358=B_SPLINE_CURVE_WITH_KNOTS('',3,(#52881,#52882,#52883,#52884,#52885,
#52886,#52887,#52888,#52889,#52890,#52891,#52892,#52893,#52894,#52895,#52896,
#52897,#52898,#52899,#52900,#52901,#52902,#52903,#52904,#52905,#52906,#52907,
#52908,#52909,#52910,#52911,#52912,#52913,#52914,#52915,#52916,#52917,#52918,
#52919,#52920,#52921,#52922,#52923,#52924,#52925,#52926,#52927,#52928,#52929,
#52930,#52931,#52932,#52933,#52934,#52935,#52936,#52937,#52938,#52939,#52940,
#52941,#52942,#52943,#52944,#52945,#52946,#52947,#52948,#52949,#52950,#52951,
#52952,#52953,#52954,#52955,#52956,#52957,#52958,#52959,#52960,#52961,#52962,
#52963,#52964,#52965,#52966,#52967,#52968,#52969,#52970,#52971,#52972,#52973,
#52974,#52975,#52976,#52977,#52978,#52979,#52980,#52981,#52982,#52983,#52984,
#52985,#52986,#52987,#52988,#52989,#52990,#52991,#52992,#52993,#52994,#52995,
#52996,#52997,#52998,#52999,#53000,#53001,#53002,#53003,#53004,#53005,#53006,
#53007,#53008,#53009,#53010,#53011,#53012,#53013,#53014,#53015,#53016,#53017,
#53018,#53019,#53020,#53021,#53022,#53023,#53024,#53025,#53026,#53027,#53028,
#53029,#53030,#53031,#53032,#53033,#53034,#53035,#53036,#53037,#53038,#53039,
#53040,#53041,#53042,#53043,#53044,#53045,#53046,#53047,#53048,#53049,#53050,
#53051,#53052,#53053,#53054,#53055,#53056,#53057,#53058,#53059,#53060,#53061,
#53062,#53063,#53064,#53065,#53066,#53067,#53068,#53069,#53070,#53071,#53072,
#53073),.UNSPECIFIED.,.F.,.F.,(4,3,3,3,3,3,3,3,3,3,3,3,3,3,3,3,3,3,3,3,
3,3,3,3,3,3,3,3,3,3,3,3,3,3,3,3,3,3,3,3,3,3,3,3,3,3,3,3,3,3,3,3,3,3,3,3,
3,3,3,3,3,3,3,3,4),(151.887629070056,152.000026667646,152.112903200505,
152.226374334767,152.26552633122,152.366159628119,152.466648210403,152.567020725605,
152.667329882549,152.76760695334,152.867883169593,152.968259097634,153.068683666076,
153.169288719408,153.260725849725,153.361359137971,153.461847711597,153.562220218176,
153.662529366523,153.762806428752,153.863082636492,153.963458556155,154.063883116278,
154.16448816149,154.25592536823,154.35655866225,154.457047241589,154.557419753761,
154.657728907625,154.758005975291,154.858282188378,154.958658113213,155.05908267842,
155.159687728511,155.251124886735,155.351758201077,155.452246800884,155.552619333645,
155.652928508164,155.753205596519,155.853481830302,155.953857775697,156.054282361424,
156.154887431724,156.246324405239,156.34695765501,156.447446190172,156.54781865848,
156.64812776869,156.748404792969,156.848680962997,156.949056845581,157.049481368912,
157.150086378246,157.241523923744,157.341206650669,157.444907616414,157.544329788682,
157.643693026811,157.743029769444,157.842372418137,157.94181121822,158.041307175409,
158.140955160636,158.170814376628),.UNSPECIFIED.);
#1359=B_SPLINE_CURVE_WITH_KNOTS('',3,(#53075,#53076,#53077,#53078,#53079,
#53080,#53081,#53082,#53083,#53084,#53085,#53086,#53087,#53088,#53089,#53090,
#53091,#53092,#53093,#53094,#53095,#53096,#53097,#53098,#53099,#53100,#53101,
#53102,#53103,#53104,#53105,#53106,#53107,#53108,#53109,#53110,#53111,#53112,
#53113,#53114,#53115,#53116,#53117,#53118,#53119,#53120,#53121,#53122,#53123,
#53124,#53125,#53126,#53127,#53128,#53129,#53130,#53131,#53132,#53133,#53134,
#53135,#53136,#53137,#53138,#53139,#53140,#53141,#53142,#53143,#53144,#53145,
#53146,#53147,#53148,#53149,#53150,#53151,#53152,#53153,#53154,#53155,#53156,
#53157,#53158,#53159,#53160,#53161,#53162,#53163,#53164,#53165,#53166,#53167,
#53168,#53169,#53170,#53171,#53172,#53173,#53174,#53175,#53176,#53177,#53178,
#53179,#53180,#53181,#53182,#53183,#53184,#53185,#53186,#53187,#53188,#53189,
#53190,#53191,#53192,#53193,#53194,#53195,#53196,#53197,#53198,#53199,#53200,
#53201,#53202,#53203,#53204,#53205,#53206,#53207,#53208,#53209,#53210,#53211,
#53212,#53213,#53214,#53215,#53216,#53217,#53218,#53219,#53220,#53221,#53222,
#53223,#53224,#53225,#53226,#53227,#53228,#53229,#53230,#53231,#53232,#53233,
#53234,#53235,#53236,#53237,#53238,#53239,#53240,#53241,#53242,#53243,#53244,
#53245,#53246,#53247,#53248,#53249,#53250,#53251,#53252,#53253,#53254,#53255,
#53256,#53257,#53258,#53259,#53260,#53261,#53262,#53263,#53264),
 .UNSPECIFIED.,.F.,.F.,(4,3,3,3,3,3,3,3,3,3,3,3,3,3,3,3,3,3,3,3,3,3,3,3,
3,3,3,3,3,3,3,3,3,3,3,3,3,3,3,3,3,3,3,3,3,3,3,3,3,3,3,3,3,3,3,3,3,3,3,3,
3,3,3,4),(158.170814377013,158.236723442249,158.337356868079,158.437845580013,
158.53821822533,158.638527512613,158.738804713784,158.839081060277,158.939457117427,
159.039881814564,159.140486994388,159.231922960753,159.332555916466,159.433044157425,
159.533416332682,159.633725150674,159.734001883964,159.834277764629,159.934653362397,
160.03507760295,160.13568233623,160.227122479258,160.327755990604,160.428244784854,
160.528617507349,160.628926868655,160.729204140619,160.829480554602,160.929856673644,
161.030281429708,161.130886662821,161.222321997763,161.322956102713,161.423445498732,
161.523818832335,161.624128810136,161.724406703087,161.824683741651,161.92506048647,
162.025485869961,162.126091725867,162.217521516267,162.318152281655,162.418638329688,
162.519008318335,162.619314954555,162.719589513872,162.819863231331,162.920236697757,
163.020658821013,163.121261485342,163.212721034772,163.31335661715,163.413847469277,
163.51422222054,163.614533592008,163.714812852928,163.815091232034,163.915469265471,
164.015895911207,164.116502970526,164.207920553277,164.338551892289,164.453999601362),
 .UNSPECIFIED.);
#1360=B_SPLINE_CURVE_WITH_KNOTS('',3,(#53266,#53267,#53268,#53269,#53270,
#53271,#53272,#53273,#53274,#53275),.UNSPECIFIED.,.F.,.F.,(4,1,1,1,1,1,
1,4),(164.453999684193,165.203120071782,166.198319590286,167.193519108791,
168.188718627296,169.1839181458,170.179117664305,170.737184991372),
 .UNSPECIFIED.);
#1361=B_SPLINE_CURVE_WITH_KNOTS('',3,(#53277,#53278,#53279,#53280,#53281,
#53282,#53283,#53284,#53285,#53286,#53287,#53288,#53289,#53290,#53291,#53292),
 .UNSPECIFIED.,.F.,.F.,(4,3,3,3,3,4),(170.737185295228,170.846468267123,
170.955913585094,171.065828907702,171.17431718281,171.179694195601),
 .UNSPECIFIED.);
#1362=B_SPLINE_CURVE_WITH_KNOTS('',3,(#53298,#53299,#53300,#53301,#53302,
#53303,#53304,#53305,#53306,#53307,#53308,#53309,#53310,#53311,#53312,#53313,
#53314,#53315,#53316,#53317,#53318,#53319,#53320,#53321,#53322,#53323,#53324,
#53325,#53326,#53327,#53328,#53329,#53330,#53331,#53332,#53333,#53334,#53335,
#53336,#53337,#53338,#53339,#53340,#53341,#53342,#53343,#53344,#53345,#53346,
#53347,#53348,#53349,#53350,#53351,#53352,#53353,#53354,#53355,#53356,#53357,
#53358,#53359,#53360,#53361,#53362,#53363,#53364,#53365,#53366,#53367,#53368,
#53369,#53370,#53371,#53372,#53373,#53374,#53375,#53376,#53377,#53378,#53379,
#53380,#53381,#53382,#53383,#53384,#53385,#53386,#53387,#53388,#53389,#53390,
#53391,#53392,#53393,#53394,#53395,#53396,#53397,#53398,#53399,#53400,#53401,
#53402,#53403,#53404,#53405,#53406,#53407,#53408,#53409,#53410,#53411,#53412,
#53413,#53414,#53415,#53416,#53417,#53418,#53419,#53420,#53421,#53422,#53423,
#53424,#53425,#53426,#53427,#53428,#53429,#53430,#53431,#53432,#53433,#53434,
#53435,#53436,#53437,#53438,#53439,#53440,#53441,#53442,#53443,#53444,#53445,
#53446,#53447,#53448,#53449,#53450,#53451,#53452,#53453,#53454,#53455,#53456,
#53457,#53458,#53459,#53460,#53461,#53462,#53463,#53464,#53465,#53466,#53467,
#53468,#53469,#53470,#53471,#53472),.UNSPECIFIED.,.F.,.F.,(4,3,3,3,3,3,
3,3,3,3,3,3,3,3,3,3,3,3,3,3,3,3,3,3,3,3,3,3,3,3,3,3,3,3,3,3,3,3,3,3,3,3,
3,3,3,3,3,3,3,3,3,3,3,3,3,3,3,3,4),(-173.164716219819,-173.061774232127,
-172.958895354895,-172.856027311868,-172.753161388755,-172.650272247811,
-172.547334532095,-172.444243715141,-172.341071938644,-172.237700988273,
-172.169516701315,-172.069856695818,-171.970355940224,-171.870851095547,
-171.771557886023,-171.672305896722,-171.57306266092,-171.473376291392,
-171.373994982198,-171.274156082504,-171.17431718281,-171.073555542376,
-170.972938691585,-170.872438670844,-170.772002541256,-170.671599220397,
-170.57119766694,-170.470698748472,-170.370152283834,-170.2694286361,-170.179117664305,
-170.07831586765,-169.977655300651,-169.877106375297,-169.776618199067,
-169.676159756601,-169.575700070683,-169.475138660369,-169.374527217061,
-169.273735113921,-169.1839181458,-169.083409385862,-168.983047108886,-168.882802972129,
-168.782623399859,-168.682476941737,-168.582332189017,-168.482088152488,
-168.381795923466,-168.281322422809,-168.188718627296,-168.089497529044,
-167.990404250906,-167.891405724206,-167.792469004558,-167.693521041499,
-167.594574193245,-167.495518831768,-167.398250967225),.UNSPECIFIED.);
#1363=B_SPLINE_CURVE_WITH_KNOTS('',3,(#53474,#53475,#53476,#53477,#53478,
#53479,#53480,#53481,#53482,#53483,#53484,#53485,#53486,#53487,#53488,#53489,
#53490,#53491,#53492,#53493,#53494,#53495,#53496,#53497,#53498,#53499,#53500,
#53501,#53502,#53503,#53504,#53505,#53506,#53507,#53508,#53509,#53510,#53511,
#53512,#53513,#53514,#53515,#53516,#53517,#53518,#53519,#53520,#53521,#53522,
#53523,#53524,#53525,#53526,#53527,#53528,#53529,#53530,#53531,#53532,#53533,
#53534,#53535,#53536,#53537,#53538,#53539,#53540,#53541,#53542,#53543,#53544,
#53545,#53546,#53547,#53548,#53549,#53550,#53551,#53552,#53553,#53554,#53555,
#53556,#53557,#53558,#53559,#53560,#53561,#53562,#53563,#53564,#53565,#53566,
#53567,#53568,#53569,#53570,#53571,#53572,#53573,#53574,#53575,#53576,#53577,
#53578,#53579,#53580,#53581,#53582,#53583,#53584,#53585,#53586,#53587,#53588,
#53589,#53590,#53591,#53592,#53593,#53594,#53595,#53596,#53597,#53598,#53599,
#53600,#53601,#53602,#53603,#53604,#53605,#53606,#53607,#53608,#53609,#53610,
#53611,#53612,#53613,#53614,#53615,#53616,#53617,#53618,#53619,#53620,#53621,
#53622,#53623,#53624,#53625,#53626,#53627,#53628,#53629,#53630,#53631,#53632,
#53633,#53634,#53635,#53636,#53637,#53638,#53639,#53640,#53641,#53642,#53643,
#53644,#53645,#53646,#53647,#53648,#53649,#53650,#53651,#53652,#53653,#53654,
#53655,#53656,#53657,#53658,#53659,#53660,#53661,#53662,#53663),
 .UNSPECIFIED.,.F.,.F.,(4,3,3,3,3,3,3,3,3,3,3,3,3,3,3,3,3,3,3,3,3,3,3,3,
3,3,3,3,3,3,3,3,3,3,3,3,3,3,3,3,3,3,3,3,3,3,3,3,3,3,3,3,3,3,3,3,3,3,3,3,
3,3,3,4),(-167.398250966954,-167.256843477477,-167.193519108791,-167.092866771413,
-166.992358726914,-166.891966205152,-166.791636719264,-166.691339025476,
-166.591041920208,-166.490644829191,-166.390198914085,-166.289572451256,
-166.198319590286,-166.097703708367,-165.997232803737,-165.896878278283,
-165.796587292888,-165.696328550035,-165.596070792856,-165.495713401586,
-165.395307442073,-165.294720902516,-165.203120071782,-165.102482061844,
-165.001988730649,-164.901611435422,-164.801297481778,-164.701015604418,
-164.600734578522,-164.50035386993,-164.399924529254,-164.299314773851,
-164.207920553277,-164.10728527015,-164.006794651673,-163.906420034439,
-163.806108736309,-163.705829488141,-163.605551061247,-163.505172885449,
-163.404746045344,-163.304138706214,-163.212721034772,-163.112090114221,
-163.011603945902,-162.911233889915,-162.810927218609,-162.710652656398,
-162.610378968209,-162.51000558127,-162.409583565122,-162.308981053238,
-162.217521516268,-162.116887418798,-162.016398028124,-161.916024696634,
-161.815714718978,-161.71543682421,-161.615159781871,-161.514783030236,
-161.414357638253,-161.313751771128,-161.222321997763,-161.115065659774),
 .UNSPECIFIED.);
#1364=B_SPLINE_CURVE_WITH_KNOTS('',3,(#53665,#53666,#53667,#53668,#53669,
#53670,#53671,#53672,#53673,#53674,#53675,#53676,#53677,#53678,#53679,#53680,
#53681,#53682,#53683,#53684,#53685,#53686,#53687,#53688,#53689,#53690,#53691,
#53692,#53693,#53694,#53695,#53696,#53697,#53698,#53699,#53700,#53701,#53702,
#53703,#53704,#53705,#53706,#53707,#53708,#53709,#53710,#53711,#53712,#53713,
#53714,#53715,#53716,#53717,#53718,#53719,#53720,#53721,#53722,#53723,#53724,
#53725,#53726,#53727,#53728,#53729,#53730,#53731,#53732,#53733,#53734,#53735,
#53736,#53737,#53738,#53739,#53740,#53741,#53742,#53743,#53744,#53745,#53746,
#53747,#53748,#53749,#53750,#53751,#53752,#53753,#53754,#53755,#53756,#53757,
#53758,#53759,#53760,#53761,#53762,#53763,#53764,#53765,#53766,#53767,#53768,
#53769,#53770,#53771,#53772,#53773,#53774,#53775,#53776,#53777,#53778,#53779,
#53780,#53781,#53782,#53783,#53784,#53785,#53786,#53787,#53788,#53789,#53790,
#53791,#53792,#53793,#53794,#53795,#53796,#53797,#53798,#53799,#53800,#53801,
#53802,#53803,#53804,#53805,#53806,#53807,#53808,#53809,#53810,#53811,#53812,
#53813,#53814,#53815,#53816,#53817,#53818,#53819,#53820,#53821,#53822,#53823,
#53824,#53825,#53826,#53827,#53828,#53829,#53830,#53831,#53832,#53833,#53834,
#53835,#53836,#53837,#53838,#53839,#53840,#53841,#53842,#53843,#53844,#53845,
#53846,#53847,#53848,#53849,#53850,#53851,#53852,#53853,#53854),
 .UNSPECIFIED.,.F.,.F.,(4,3,3,3,3,3,3,3,3,3,3,3,3,3,3,3,3,3,3,3,3,3,3,3,
3,3,3,3,3,3,3,3,3,3,3,3,3,3,3,3,3,3,3,3,3,3,3,3,3,3,3,3,3,3,3,3,3,3,3,3,
3,3,3,4),(-161.115065659554,-161.015800200422,-160.916674940153,-160.817627264428,
-160.718624347641,-160.619633423009,-160.520554010525,-160.421433091436,
-160.322134850872,-160.227122479258,-160.12648950089,-160.02600124239,-159.925629057356,
-159.825320234315,-159.725043500696,-159.624767624419,-159.524392038399,
-159.423967813645,-159.323363102809,-159.231922960753,-159.131289537792,
-159.030800828007,-158.93042818375,-158.830118896863,-158.729841695426,
-158.629565348006,-158.529189288898,-158.428764589237,-158.328159405962,
-158.236723442249,-158.136090136973,-158.03560154574,-157.935229020767,
-157.834919853554,-157.734642772011,-157.634366544534,-157.533990604604,
-157.43356602389,-157.332960957774,-157.241523923744,-157.14089067075,-157.040402133095,
-156.940029663402,-156.839720552481,-156.739443528165,-156.639167358773,
-156.538791477875,-156.438366956807,-156.337761950686,-156.246324405239,
-156.145691091532,-156.045202492206,-155.94482995969,-155.844520785274,
-155.744243696879,-155.643967462913,-155.543591517113,-155.443166930859,
-155.342561859832,-155.251124886735,-155.140971132557,-155.031115086589,
-154.921757951068,-154.83188035295),.UNSPECIFIED.);
#1365=B_SPLINE_CURVE_WITH_KNOTS('',3,(#53856,#53857,#53858,#53859,#53860,
#53861,#53862,#53863,#53864,#53865,#53866,#53867,#53868,#53869,#53870,#53871,
#53872,#53873,#53874,#53875,#53876,#53877,#53878,#53879,#53880,#53881,#53882,
#53883,#53884,#53885,#53886,#53887,#53888,#53889,#53890,#53891,#53892,#53893,
#53894,#53895,#53896,#53897,#53898,#53899,#53900,#53901,#53902,#53903,#53904,
#53905,#53906,#53907,#53908,#53909,#53910,#53911,#53912,#53913,#53914,#53915,
#53916,#53917,#53918,#53919,#53920,#53921,#53922,#53923,#53924,#53925,#53926,
#53927,#53928,#53929,#53930,#53931,#53932,#53933,#53934,#53935,#53936,#53937,
#53938,#53939,#53940,#53941,#53942,#53943,#53944,#53945,#53946,#53947,#53948,
#53949,#53950,#53951,#53952,#53953,#53954,#53955,#53956,#53957,#53958,#53959,
#53960,#53961,#53962,#53963,#53964,#53965,#53966,#53967,#53968,#53969,#53970,
#53971,#53972,#53973,#53974,#53975,#53976,#53977,#53978,#53979,#53980,#53981,
#53982,#53983,#53984,#53985,#53986,#53987,#53988,#53989,#53990,#53991,#53992,
#53993,#53994,#53995,#53996,#53997,#53998,#53999,#54000,#54001,#54002,#54003,
#54004,#54005,#54006,#54007,#54008,#54009,#54010,#54011,#54012,#54013,#54014,
#54015,#54016,#54017,#54018,#54019,#54020,#54021,#54022,#54023,#54024,#54025,
#54026,#54027,#54028,#54029,#54030,#54031,#54032,#54033,#54034,#54035,#54036,
#54037,#54038,#54039,#54040,#54041,#54042,#54043,#54044,#54045,#54046,#54047,
#54048),.UNSPECIFIED.,.F.,.F.,(4,3,3,3,3,3,3,3,3,3,3,3,3,3,3,3,3,3,3,3,
3,3,3,3,3,3,3,3,3,3,3,3,3,3,3,3,3,3,3,3,3,3,3,3,3,3,3,3,3,3,3,3,3,3,3,3,
3,3,3,3,3,3,3,3,4),(-154.831880352595,-154.729682229563,-154.627429231303,
-154.525011782519,-154.422505655058,-154.319788821663,-154.25592536823,
-154.155292079537,-154.054803505564,-153.954430998793,-153.854121850349,
-153.753844788115,-153.653568580465,-153.553192661038,-153.452768101231,
-153.352163056466,-153.260725849725,-153.160092552944,-153.059603970749,
-152.959231455593,-152.858922298669,-152.758645227872,-152.658369011587,
-152.557993083472,-152.457568514935,-152.356963461469,-152.26552633122,
-152.164893037697,-152.064404458798,-151.964031946975,-151.863722793407,
-151.763445725983,-151.663169513082,-151.562793588349,-151.462369023196,
-151.361763973081,-151.270326812716,-151.169693519517,-151.069204940955,
-150.968832429493,-150.868523276298,-150.768246209259,-150.667969996757,
-150.567594072437,-150.467169507708,-150.366564458028,-150.275127294211,
-150.174493999962,-150.074005420332,-149.97363290778,-149.873323753481,
-149.773046685327,-149.672770471699,-149.572394546247,-149.471969980378,
-149.371364929561,-149.279927775706,-149.180333143564,-149.080870560533,
-148.981507319459,-148.882210835513,-148.782924030068,-148.683642355602,
-148.584295310261,-148.548695045415),.UNSPECIFIED.);
#1366=B_SPLINE_CURVE_WITH_KNOTS('',3,(#54050,#54051,#54052,#54053,#54054,
#54055,#54056,#54057,#54058,#54059,#54060,#54061,#54062,#54063,#54064,#54065,
#54066,#54067,#54068,#54069,#54070,#54071,#54072,#54073,#54074,#54075,#54076,
#54077,#54078,#54079,#54080,#54081,#54082,#54083,#54084,#54085,#54086,#54087,
#54088,#54089,#54090,#54091,#54092,#54093,#54094,#54095,#54096,#54097,#54098,
#54099,#54100,#54101,#54102,#54103,#54104,#54105,#54106,#54107,#54108,#54109,
#54110,#54111,#54112,#54113,#54114,#54115,#54116,#54117,#54118,#54119,#54120,
#54121,#54122,#54123,#54124,#54125,#54126,#54127,#54128,#54129,#54130,#54131,
#54132,#54133,#54134,#54135,#54136,#54137,#54138,#54139,#54140,#54141,#54142,
#54143,#54144,#54145,#54146,#54147,#54148,#54149,#54150,#54151,#54152,#54153,
#54154,#54155,#54156,#54157,#54158,#54159,#54160,#54161,#54162,#54163,#54164,
#54165,#54166,#54167,#54168,#54169,#54170,#54171,#54172,#54173,#54174,#54175,
#54176,#54177,#54178,#54179,#54180,#54181,#54182,#54183,#54184,#54185,#54186,
#54187,#54188,#54189,#54190,#54191,#54192,#54193,#54194,#54195,#54196,#54197,
#54198,#54199,#54200,#54201,#54202,#54203,#54204,#54205,#54206,#54207,#54208,
#54209,#54210,#54211,#54212,#54213,#54214,#54215,#54216,#54217,#54218,#54219,
#54220,#54221,#54222,#54223,#54224,#54225,#54226,#54227,#54228,#54229,#54230,
#54231,#54232,#54233,#54234,#54235,#54236,#54237,#54238,#54239),
 .UNSPECIFIED.,.F.,.F.,(4,3,3,3,3,3,3,3,3,3,3,3,3,3,3,3,3,3,3,3,3,3,3,3,
3,3,3,3,3,3,3,3,3,3,3,3,3,3,3,3,3,3,3,3,3,3,3,3,3,3,3,3,3,3,3,3,3,3,3,3,
3,3,3,4),(-148.548695045061,-148.416711651131,-148.284728257202,-148.184094963453,
-148.083606384331,-147.983233872294,-147.882924718517,-147.782647650889,
-147.682371437791,-147.58199551287,-147.481570947536,-147.38096589725,-147.289528738697,
-147.188895444816,-147.08840686556,-146.988034353387,-146.887725199471,
-146.787448131702,-146.687171918462,-146.586795993399,-146.48637142792,
-146.385766377491,-146.294329220192,-146.193695926386,-146.093207347206,
-145.99283483511,-145.892525681272,-145.792248613582,-145.691972400421,
-145.591596475436,-145.491171910037,-145.390566859687,-145.299129701687,
-145.198496407874,-145.098007828688,-144.997635316585,-144.89732616274,
-144.797049095044,-144.696772881877,-144.596396956886,-144.495972391481,
-144.395367341125,-144.303930183183,-144.203296889354,-144.102808310151,
-144.002435798032,-143.902126644169,-143.801849576456,-143.701573363271,
-143.601197438263,-143.50077287284,-143.400167822466,-143.308730664678,
-143.20809737086,-143.107608791668,-143.007236279559,-142.906927125708,
-142.806650058006,-142.706373844833,-142.605997919835,-142.505573354424,
-142.404968304061,-142.313531146173,-142.265509738235),.UNSPECIFIED.);
#1367=B_SPLINE_CURVE_WITH_KNOTS('',3,(#54241,#54242,#54243,#54244,#54245,
#54246,#54247,#54248,#54249,#54250,#54251,#54252,#54253,#54254,#54255,#54256,
#54257,#54258,#54259,#54260,#54261,#54262,#54263,#54264,#54265,#54266,#54267,
#54268,#54269,#54270,#54271,#54272,#54273,#54274,#54275,#54276,#54277,#54278,
#54279,#54280,#54281,#54282,#54283,#54284,#54285,#54286,#54287,#54288,#54289,
#54290,#54291,#54292,#54293,#54294,#54295,#54296,#54297,#54298,#54299,#54300,
#54301,#54302,#54303,#54304,#54305,#54306,#54307,#54308,#54309,#54310,#54311,
#54312,#54313,#54314,#54315,#54316,#54317,#54318,#54319,#54320,#54321,#54322,
#54323,#54324,#54325,#54326,#54327,#54328,#54329,#54330,#54331,#54332,#54333,
#54334,#54335,#54336,#54337,#54338,#54339,#54340,#54341,#54342,#54343,#54344,
#54345,#54346,#54347,#54348,#54349,#54350,#54351,#54352,#54353,#54354,#54355,
#54356,#54357,#54358,#54359,#54360,#54361,#54362,#54363,#54364,#54365,#54366,
#54367,#54368,#54369,#54370,#54371,#54372,#54373,#54374,#54375,#54376,#54377,
#54378,#54379,#54380,#54381,#54382,#54383,#54384,#54385,#54386,#54387,#54388,
#54389,#54390,#54391,#54392,#54393,#54394,#54395,#54396,#54397,#54398,#54399,
#54400,#54401,#54402,#54403,#54404,#54405,#54406,#54407,#54408,#54409,#54410,
#54411,#54412,#54413,#54414,#54415,#54416,#54417,#54418,#54419,#54420,#54421,
#54422,#54423,#54424,#54425,#54426,#54427,#54428,#54429,#54430,#54431,#54432,
#54433),.UNSPECIFIED.,.F.,.F.,(4,3,3,3,3,3,3,3,3,3,3,3,3,3,3,3,3,3,3,3,
3,3,3,3,3,3,3,3,3,3,3,3,3,3,3,3,3,3,3,3,3,3,3,3,3,3,3,3,3,3,3,3,3,3,3,3,
3,3,3,3,3,3,3,3,4),(-142.265509737928,-142.165633574489,-142.065897851332,
-141.966270709277,-141.866701131734,-141.767156909997,-141.667605870528,
-141.567952330949,-141.468241472944,-141.368364768051,-141.318331627669,
-141.217698333847,-141.117209754651,-141.016837242539,-140.916528088684,
-140.816251020978,-140.715974807801,-140.6155988828,-140.515174317384,-140.414569267018,
-140.323132109164,-140.222498815344,-140.122010236149,-140.021637724038,
-139.921328570185,-139.821051502481,-139.720775289305,-139.620399364306,
-139.519974798892,-139.419369748527,-139.327932590659,-139.227299296839,
-139.126810717644,-139.026438205534,-138.926129051681,-138.825851983977,
-138.725575770801,-138.625199845802,-138.524775280388,-138.424170230023,
-138.332733072155,-138.232099778334,-138.131611199139,-138.031238687028,
-137.930929533175,-137.83065246547,-137.730376252294,-137.630000327294,
-137.52957576188,-137.428970711514,-137.33753355365,-137.236900259829,-137.136411680635,
-137.036039168524,-136.93573001467,-136.835452946965,-136.735176733789,
-136.634800808789,-136.534376243375,-136.433771193009,-136.342334035145,
-136.227285324675,-136.112723200038,-135.998976348791,-135.982324431284),
 .UNSPECIFIED.);
#1368=B_SPLINE_CURVE_WITH_KNOTS('',3,(#54435,#54436,#54437,#54438,#54439,
#54440,#54441,#54442,#54443,#54444,#54445,#54446,#54447,#54448,#54449,#54450,
#54451,#54452,#54453,#54454,#54455,#54456,#54457,#54458,#54459,#54460,#54461,
#54462,#54463,#54464,#54465,#54466,#54467,#54468,#54469,#54470,#54471,#54472,
#54473,#54474,#54475,#54476,#54477,#54478,#54479,#54480,#54481,#54482,#54483,
#54484,#54485,#54486,#54487,#54488,#54489,#54490,#54491,#54492,#54493,#54494,
#54495,#54496,#54497,#54498,#54499,#54500,#54501,#54502,#54503,#54504,#54505,
#54506,#54507,#54508,#54509,#54510,#54511,#54512,#54513,#54514,#54515,#54516,
#54517,#54518,#54519,#54520,#54521,#54522,#54523,#54524,#54525,#54526,#54527,
#54528,#54529,#54530,#54531,#54532,#54533,#54534,#54535,#54536,#54537,#54538,
#54539,#54540,#54541,#54542,#54543,#54544,#54545,#54546,#54547,#54548,#54549,
#54550,#54551,#54552,#54553,#54554,#54555,#54556,#54557,#54558,#54559,#54560,
#54561,#54562,#54563,#54564,#54565,#54566,#54567,#54568,#54569,#54570,#54571,
#54572,#54573,#54574,#54575,#54576,#54577,#54578,#54579,#54580,#54581,#54582,
#54583,#54584,#54585,#54586,#54587,#54588,#54589,#54590,#54591,#54592,#54593,
#54594,#54595,#54596,#54597,#54598,#54599,#54600,#54601,#54602,#54603,#54604,
#54605,#54606,#54607,#54608,#54609,#54610,#54611,#54612,#54613,#54614,#54615,
#54616,#54617,#54618,#54619,#54620,#54621,#54622,#54623,#54624,#54625,#54626,
#54627),.UNSPECIFIED.,.F.,.F.,(4,3,3,3,3,3,3,3,3,3,3,3,3,3,3,3,3,3,3,3,
3,3,3,3,3,3,3,3,3,3,3,3,3,3,3,3,3,3,3,3,3,3,3,3,3,3,3,3,3,3,3,3,3,3,3,3,
3,3,3,3,3,3,3,3,4),(-135.982324431056,-135.881583024083,-135.780838722731,
-135.680061277593,-135.579153091099,-135.478167949569,-135.377006907812,
-135.34713451664,-135.24650122282,-135.146012643626,-135.045640131515,-134.945330977662,
-134.845053909958,-134.744777696782,-134.644401771783,-134.543977206369,
-134.443372156005,-134.351934998136,-134.251301704315,-134.150813125121,
-134.05044061301,-133.950131459156,-133.849854391452,-133.749578178276,
-133.649202253276,-133.548777687862,-133.448172637497,-133.356735479631,
-133.25610218581,-133.155613606615,-133.055241094504,-132.95493194065,-132.854654872945,
-132.754378659769,-132.654002734769,-132.553578169354,-132.452973118989,
-132.361535961126,-132.260902667306,-132.160414088112,-132.060041576001,
-131.959732422148,-131.859455354444,-131.759179141268,-131.658803216269,
-131.558378650855,-131.45777360049,-131.366336442622,-131.265703148802,
-131.165214569607,-131.064842057496,-130.964532903643,-130.864255835938,
-130.763979622762,-130.663603697762,-130.563179132348,-130.462574081983,
-130.371136924117,-130.270722015059,-130.170446946524,-130.07028000736,
-129.970182457444,-129.870127451158,-129.770050097071,-129.699139123876),
 .UNSPECIFIED.);
#1369=B_SPLINE_CURVE_WITH_KNOTS('',3,(#54629,#54630,#54631,#54632,#54633,
#54634,#54635,#54636,#54637,#54638,#54639,#54640,#54641,#54642,#54643,#54644,
#54645,#54646,#54647,#54648,#54649,#54650,#54651,#54652,#54653,#54654,#54655,
#54656,#54657,#54658,#54659,#54660,#54661,#54662,#54663,#54664,#54665,#54666,
#54667,#54668,#54669,#54670,#54671,#54672,#54673,#54674,#54675,#54676,#54677,
#54678,#54679,#54680,#54681,#54682,#54683,#54684,#54685,#54686,#54687,#54688,
#54689,#54690,#54691,#54692,#54693,#54694,#54695,#54696,#54697,#54698,#54699,
#54700,#54701,#54702,#54703,#54704,#54705,#54706,#54707,#54708,#54709,#54710,
#54711,#54712,#54713,#54714,#54715,#54716,#54717,#54718,#54719,#54720,#54721,
#54722,#54723,#54724,#54725,#54726,#54727,#54728,#54729,#54730,#54731,#54732,
#54733,#54734,#54735,#54736,#54737,#54738,#54739,#54740,#54741,#54742,#54743,
#54744,#54745,#54746,#54747,#54748,#54749,#54750,#54751,#54752,#54753,#54754,
#54755,#54756,#54757,#54758,#54759,#54760,#54761,#54762,#54763,#54764,#54765,
#54766,#54767,#54768,#54769,#54770,#54771,#54772,#54773,#54774,#54775,#54776,
#54777,#54778,#54779,#54780,#54781,#54782,#54783,#54784,#54785,#54786,#54787,
#54788,#54789,#54790,#54791,#54792,#54793,#54794,#54795,#54796,#54797,#54798,
#54799,#54800,#54801,#54802,#54803,#54804,#54805,#54806,#54807,#54808,#54809,
#54810,#54811,#54812,#54813,#54814,#54815,#54816,#54817,#54818),
 .UNSPECIFIED.,.F.,.F.,(4,3,3,3,3,3,3,3,3,3,3,3,3,3,3,3,3,3,3,3,3,3,3,3,
3,3,3,3,3,3,3,3,3,3,3,3,3,3,3,3,3,3,3,3,3,3,3,3,3,3,3,3,3,3,3,3,3,3,3,3,
3,3,3,4),(-129.69913912347,-129.581509782298,-129.462588504636,-129.375937405612,
-129.275304111791,-129.174815532596,-129.074443020485,-128.974133866631,
-128.873856798926,-128.77358058575,-128.67320466075,-128.572780095335,-128.47217504497,
-128.380737887107,-128.280104593287,-128.179616014092,-128.079243501981,
-127.978934348128,-127.878657280424,-127.778381067248,-127.678005142249,
-127.577580576835,-127.47697552647,-127.385538368603,-127.284905074783,
-127.184416495588,-127.084043983477,-126.983734829624,-126.883457761919,
-126.783181548743,-126.682805623744,-126.58238105833,-126.481776007964,
-126.390338850098,-126.289705556277,-126.189216977082,-126.088844464971,
-125.988535311117,-125.888258243412,-125.787982030236,-125.687606105236,
-125.587181539821,-125.486576489456,-125.395139331593,-125.294506037773,
-125.194017458578,-125.093644946467,-124.993335792614,-124.89305872491,
-124.792782511734,-124.692406586735,-124.591982021321,-124.491376970956,
-124.399939813089,-124.299503686858,-124.199212133855,-124.099036003752,
-123.998922538952,-123.898840194359,-123.798757464703,-123.698574952104,
-123.598342156662,-123.497932620793,-123.415953817054),.UNSPECIFIED.);
#1370=B_SPLINE_CURVE_WITH_KNOTS('',3,(#54820,#54821,#54822,#54823,#54824,
#54825,#54826,#54827,#54828,#54829,#54830,#54831,#54832,#54833,#54834,#54835,
#54836,#54837,#54838,#54839,#54840,#54841,#54842,#54843,#54844,#54845,#54846,
#54847,#54848,#54849,#54850,#54851,#54852,#54853,#54854,#54855,#54856,#54857,
#54858,#54859,#54860,#54861,#54862,#54863,#54864,#54865,#54866,#54867,#54868,
#54869,#54870,#54871,#54872,#54873,#54874,#54875,#54876,#54877,#54878,#54879,
#54880,#54881,#54882,#54883,#54884,#54885,#54886,#54887,#54888,#54889,#54890,
#54891,#54892,#54893,#54894,#54895,#54896,#54897,#54898,#54899,#54900,#54901,
#54902,#54903,#54904,#54905,#54906,#54907,#54908,#54909,#54910,#54911,#54912,
#54913,#54914,#54915,#54916,#54917,#54918,#54919,#54920,#54921,#54922,#54923,
#54924,#54925,#54926,#54927,#54928,#54929,#54930,#54931,#54932,#54933,#54934,
#54935,#54936,#54937,#54938,#54939,#54940,#54941,#54942,#54943,#54944,#54945,
#54946,#54947,#54948,#54949,#54950,#54951,#54952,#54953,#54954,#54955,#54956,
#54957,#54958,#54959,#54960,#54961,#54962,#54963,#54964,#54965,#54966,#54967,
#54968,#54969,#54970,#54971,#54972,#54973,#54974,#54975,#54976,#54977,#54978,
#54979,#54980,#54981,#54982,#54983,#54984,#54985,#54986,#54987,#54988,#54989,
#54990,#54991,#54992,#54993,#54994,#54995,#54996,#54997,#54998,#54999,#55000,
#55001,#55002,#55003,#55004,#55005,#55006,#55007,#55008,#55009,#55010,#55011,
#55012),.UNSPECIFIED.,.F.,.F.,(4,3,3,3,3,3,3,3,3,3,3,3,3,3,3,3,3,3,3,3,
3,3,3,3,3,3,3,3,3,3,3,3,3,3,3,3,3,3,3,3,3,3,3,3,3,3,3,3,3,3,3,3,3,3,3,3,
3,3,3,3,3,3,3,3,4),(-123.415953816697,-123.404740294584,-123.304107000763,
-123.203618421569,-123.103245909458,-123.002936755605,-122.9026596879,-122.802383474724,
-122.702007549724,-122.60158298431,-122.500977933945,-122.409540776079,
-122.308907482258,-122.208418903063,-122.108046390952,-122.007737237099,
-121.907460169394,-121.807183956218,-121.706808031218,-121.606383465803,
-121.505778415438,-121.414341257574,-121.313707963754,-121.213219384559,
-121.112846872449,-121.012537718596,-120.912260650891,-120.811984437715,
-120.711608512716,-120.611183947302,-120.510578896937,-120.41914173907,
-120.318508445249,-120.218019866055,-120.117647353944,-120.01733820009,
-119.917061132386,-119.81678491921,-119.71640899421,-119.615984428796,-119.515379378431,
-119.423942220565,-119.323308926744,-119.222820347549,-119.122447835438,
-119.022138681584,-118.921861613879,-118.821585400703,-118.721209475703,
-118.620784910289,-118.520179859923,-118.42874270206,-118.32810940824,-118.227620829045,
-118.127248316935,-118.026939163082,-117.926662095377,-117.826385882202,
-117.726009957202,-117.625585391788,-117.524980341423,-117.433543183556,
-117.31144553275,-117.190918574851,-117.132768509857),.UNSPECIFIED.);
#1371=B_SPLINE_CURVE_WITH_KNOTS('',3,(#55014,#55015,#55016,#55017,#55018,
#55019,#55020,#55021,#55022,#55023,#55024,#55025,#55026,#55027,#55028,#55029,
#55030,#55031,#55032,#55033,#55034,#55035,#55036,#55037,#55038,#55039,#55040,
#55041,#55042,#55043,#55044,#55045,#55046,#55047,#55048,#55049,#55050,#55051,
#55052,#55053,#55054,#55055,#55056,#55057,#55058,#55059,#55060,#55061,#55062,
#55063,#55064,#55065,#55066,#55067,#55068,#55069,#55070,#55071,#55072,#55073,
#55074,#55075,#55076,#55077,#55078,#55079,#55080,#55081,#55082,#55083,#55084,
#55085,#55086,#55087,#55088,#55089,#55090,#55091,#55092,#55093,#55094,#55095,
#55096,#55097,#55098,#55099,#55100,#55101,#55102,#55103,#55104,#55105,#55106,
#55107,#55108,#55109,#55110,#55111,#55112,#55113,#55114,#55115,#55116,#55117,
#55118,#55119,#55120,#55121,#55122,#55123,#55124,#55125,#55126,#55127,#55128,
#55129,#55130,#55131,#55132,#55133,#55134,#55135,#55136,#55137,#55138,#55139,
#55140,#55141,#55142,#55143,#55144,#55145,#55146,#55147,#55148,#55149,#55150,
#55151,#55152,#55153,#55154,#55155,#55156,#55157,#55158,#55159,#55160,#55161,
#55162,#55163,#55164,#55165,#55166,#55167,#55168,#55169,#55170,#55171,#55172,
#55173,#55174,#55175,#55176,#55177,#55178,#55179,#55180,#55181,#55182,#55183,
#55184,#55185,#55186,#55187,#55188,#55189,#55190,#55191,#55192,#55193,#55194,
#55195,#55196,#55197,#55198,#55199,#55200,#55201,#55202,#55203),
 .UNSPECIFIED.,.F.,.F.,(4,3,3,3,3,3,3,3,3,3,3,3,3,3,3,3,3,3,3,3,3,3,3,3,
3,3,3,3,3,3,3,3,3,3,3,3,3,3,3,3,3,3,3,3,3,3,3,3,3,3,3,3,3,3,3,3,3,3,3,3,
3,3,3,4),(-117.132768509517,-117.033015063478,-116.933296664845,-116.833581387141,
-116.733766480766,-116.633903776678,-116.533856241353,-116.438343665051,
-116.337710371231,-116.237221792036,-116.136849279925,-116.036540126071,
-115.936263058367,-115.835986845191,-115.735610920191,-115.635186354777,
-115.534581304412,-115.443144146546,-115.342510852725,-115.24202227353,
-115.141649761419,-115.041340607566,-114.941063539861,-114.840787326685,
-114.740411401685,-114.63998683627,-114.539381785905,-114.447944628041,
-114.347311334221,-114.246822755026,-114.146450242915,-114.046141089062,
-113.945864021358,-113.845587808182,-113.745211883183,-113.644787317769,
-113.544182267404,-113.452745109537,-113.352111815717,-113.251623236522,
-113.151250724411,-113.050941570557,-112.950664502853,-112.850388289677,
-112.750012364677,-112.649587799263,-112.548982748898,-112.457545591032,
-112.356912297211,-112.256423718016,-112.156051205905,-112.055742052052,
-111.955464984347,-111.855188771171,-111.754812846171,-111.654388280757,
-111.553783230392,-111.462346072527,-111.360662607761,-111.259132552871,
-111.156745215238,-111.055443771602,-110.95251348697,-110.849583202337),
 .UNSPECIFIED.);
#1372=B_SPLINE_CURVE_WITH_KNOTS('',3,(#55205,#55206,#55207,#55208,#55209,
#55210,#55211,#55212,#55213,#55214),.UNSPECIFIED.,.F.,.F.,(4,1,1,1,1,1,
1,4),(-110.849576038581,-110.467146554023,-109.471947035518,-108.476747517013,
-107.481547998509,-106.486348480004,-105.491148961499,-104.566397895158),
 .UNSPECIFIED.);
#1373=B_SPLINE_CURVE_WITH_KNOTS('',3,(#55216,#55217,#55218,#55219,#55220,
#55221,#55222,#55223,#55224,#55225,#55226),.UNSPECIFIED.,.F.,.F.,(4,1,1,
1,1,1,1,1,4),(-104.566397895158,-104.495949442994,-103.50074992449,-102.505550405985,
-101.51035088748,-100.515151368976,-99.5199518504709,-98.5247523319661,
-98.2832125879783),.UNSPECIFIED.);
#1374=B_SPLINE_CURVE_WITH_KNOTS('',3,(#55228,#55229,#55230,#55231,#55232,
#55233,#55234,#55235,#55236,#55237),.UNSPECIFIED.,.F.,.F.,(4,1,1,1,1,1,
1,4),(-98.2832125879783,-97.5295528134614,-96.5343532949567,-95.539153776452,
-94.5439542579473,-93.5487547394426,-92.5535552209379,-92.0000272807987),
 .UNSPECIFIED.);
#1375=B_SPLINE_CURVE_WITH_KNOTS('',3,(#55239,#55240,#55241,#55242,#55243,
#55244,#55245,#55246,#55247,#55248),.UNSPECIFIED.,.F.,.F.,(4,1,1,1,1,1,
1,4),(-92.0000272807987,-91.5583557024332,-90.5631561839285,-89.5679566654238,
-88.5727571469191,-87.5775576284143,-86.5823581099096,-85.7168419736191),
 .UNSPECIFIED.);
#1376=B_SPLINE_CURVE_WITH_KNOTS('',3,(#55250,#55251,#55252,#55253,#55254,
#55255,#55256,#55257,#55258,#55259,#55260),.UNSPECIFIED.,.F.,.F.,(4,1,1,
1,1,1,1,1,4),(-85.7168419736191,-85.5871585914049,-84.5919590729002,-83.5967595543955,
-82.6015600358908,-81.6063605173861,-80.6111609988814,-79.6159614803767,
-79.4336566664395),.UNSPECIFIED.);
#1377=B_SPLINE_CURVE_WITH_KNOTS('',3,(#55262,#55263,#55264,#55265,#55266,
#55267,#55268,#55269,#55270,#55271),.UNSPECIFIED.,.F.,.F.,(4,1,1,1,1,1,
1,4),(-79.4336566664395,-78.620761961872,-77.6255624433673,-76.6303629248626,
-75.6351634063578,-74.6399638878531,-73.6447643693484,-73.1504713592599),
 .UNSPECIFIED.);
#1378=B_SPLINE_CURVE_WITH_KNOTS('',3,(#55273,#55274,#55275,#55276,#55277,
#55278,#55279,#55280,#55281,#55282),.UNSPECIFIED.,.F.,.F.,(4,1,1,1,1,1,
1,4),(-73.1504713592599,-72.6495648508437,-71.654365332339,-70.6591658138343,
-69.6639662953296,-68.6687667768249,-67.6735672583202,-66.8672860520803),
 .UNSPECIFIED.);
#1379=B_SPLINE_CURVE_WITH_KNOTS('',3,(#55284,#55285,#55286,#55287,#55288,
#55289,#55290,#55291,#55292,#55293,#55294),.UNSPECIFIED.,.F.,.F.,(4,1,1,
1,1,1,1,1,4),(-66.8672860520803,-66.6783677398155,-65.6831682213108,-64.6879687028061,
-63.6927691843014,-62.6975696657967,-61.7023701472919,-60.7071706287872,
-60.5841007449007),.UNSPECIFIED.);
#1380=B_SPLINE_CURVE_WITH_KNOTS('',3,(#55296,#55297,#55298,#55299,#55300,
#55301,#55302,#55303,#55304,#55305),.UNSPECIFIED.,.F.,.F.,(4,1,1,1,1,1,
1,4),(-60.5841007449007,-59.7119711102825,-58.7167715917778,-57.7215720732731,
-56.7263725547684,-55.7311730362637,-54.735973517759,-54.3009201196733),
 .UNSPECIFIED.);
#1381=B_SPLINE_CURVE_WITH_KNOTS('',3,(#55307,#55308,#55309,#55310,#55311,
#55312,#55313,#55314,#55315,#55316,#55317,#55318,#55319,#55320,#55321,#55322,
#55323,#55324,#55325,#55326,#55327,#55328,#55329,#55330,#55331,#55332,#55333,
#55334,#55335,#55336,#55337,#55338,#55339,#55340,#55341,#55342,#55343,#55344,
#55345,#55346,#55347,#55348,#55349,#55350,#55351,#55352,#55353,#55354,#55355,
#55356,#55357,#55358,#55359,#55360,#55361,#55362,#55363,#55364,#55365,#55366,
#55367,#55368,#55369,#55370,#55371,#55372,#55373,#55374,#55375,#55376,#55377,
#55378,#55379,#55380,#55381,#55382,#55383,#55384,#55385,#55386,#55387,#55388,
#55389,#55390,#55391,#55392,#55393,#55394,#55395,#55396,#55397,#55398,#55399,
#55400,#55401,#55402,#55403,#55404,#55405,#55406,#55407,#55408,#55409,#55410,
#55411,#55412,#55413,#55414,#55415,#55416,#55417,#55418,#55419,#55420,#55421,
#55422,#55423,#55424,#55425,#55426,#55427,#55428,#55429,#55430,#55431,#55432,
#55433,#55434,#55435,#55436,#55437,#55438,#55439,#55440,#55441,#55442,#55443,
#55444,#55445,#55446,#55447,#55448,#55449,#55450,#55451,#55452,#55453,#55454,
#55455,#55456,#55457,#55458,#55459,#55460,#55461,#55462,#55463,#55464,#55465,
#55466,#55467,#55468,#55469,#55470,#55471,#55472,#55473,#55474,#55475,#55476,
#55477,#55478,#55479,#55480,#55481,#55482,#55483,#55484,#55485,#55486,#55487,
#55488,#55489,#55490,#55491,#55492,#55493,#55494,#55495,#55496,#55497,#55498,
#55499),.UNSPECIFIED.,.F.,.F.,(4,3,3,3,3,3,3,3,3,3,3,3,3,3,3,3,3,3,3,3,
3,3,3,3,3,3,3,3,3,3,3,3,3,3,3,3,3,3,3,3,3,3,3,3,3,3,3,3,3,3,3,3,3,3,3,3,
3,3,3,3,3,3,3,3,4),(-54.3009154377211,-54.1982387367601,-54.095489715743,
-53.9925596038351,-53.8895284587086,-53.7862850394966,-53.7407739992543,
-53.6401407054337,-53.5396521262388,-53.4392796141279,-53.3389704602745,
-53.2386933925698,-53.1384171793937,-53.0380412543939,-52.9376166889798,
-52.8370116386147,-52.7455744807496,-52.6449411869291,-52.5444526077341,
-52.4440800956232,-52.3437709417699,-52.2434938740655,-52.1432176608895,
-52.0428417358898,-51.9424171704756,-51.8418121201105,-51.7503749622449,
-51.6497416684244,-51.5492530892298,-51.4488805771189,-51.3485714232656,
-51.248294355561,-51.1480181423849,-51.0476422173853,-50.9472176519712,
-50.8466126016061,-50.7551754437401,-50.6545421499194,-50.5540535707246,
-50.4536810586138,-50.3533719047605,-50.2530948370559,-50.1528186238798,
-50.05244269888,-49.9520181334659,-49.8514130831007,-49.7599759252354,-49.6593426314148,
-49.5588540522202,-49.4584815401094,-49.358172386256,-49.2578953185515,
-49.1576191053754,-49.0572431803758,-48.9568186149618,-48.8562135645966,
-48.7647764067307,-48.665331690439,-48.5660176090869,-48.4668013028627,
-48.3676500354695,-48.268502398764,-48.1693583936258,-48.0701377857838,
-48.0177301305415),.UNSPECIFIED.);
#1382=B_SPLINE_CURVE_WITH_KNOTS('',3,(#55501,#55502,#55503,#55504,#55505,
#55506,#55507,#55508,#55509,#55510,#55511,#55512,#55513,#55514,#55515,#55516,
#55517,#55518,#55519,#55520,#55521,#55522,#55523,#55524,#55525,#55526,#55527,
#55528,#55529,#55530,#55531,#55532,#55533,#55534,#55535,#55536,#55537,#55538,
#55539,#55540,#55541,#55542,#55543,#55544,#55545,#55546,#55547,#55548,#55549,
#55550,#55551,#55552,#55553,#55554,#55555,#55556,#55557,#55558,#55559,#55560,
#55561,#55562,#55563,#55564,#55565,#55566,#55567,#55568,#55569,#55570,#55571,
#55572,#55573,#55574,#55575,#55576,#55577,#55578,#55579,#55580,#55581,#55582,
#55583,#55584,#55585,#55586,#55587,#55588,#55589,#55590,#55591,#55592,#55593,
#55594,#55595,#55596,#55597,#55598,#55599,#55600,#55601,#55602,#55603,#55604,
#55605,#55606,#55607,#55608,#55609,#55610,#55611,#55612,#55613,#55614,#55615,
#55616,#55617,#55618,#55619,#55620,#55621,#55622,#55623,#55624,#55625,#55626,
#55627,#55628,#55629,#55630,#55631,#55632,#55633,#55634,#55635,#55636,#55637,
#55638,#55639,#55640,#55641,#55642,#55643,#55644,#55645,#55646,#55647,#55648,
#55649,#55650,#55651,#55652,#55653,#55654,#55655,#55656,#55657,#55658,#55659,
#55660,#55661,#55662,#55663,#55664,#55665,#55666,#55667,#55668,#55669,#55670,
#55671,#55672,#55673,#55674,#55675,#55676,#55677,#55678,#55679,#55680,#55681,
#55682,#55683,#55684,#55685,#55686,#55687,#55688,#55689,#55690),
 .UNSPECIFIED.,.F.,.F.,(4,3,3,3,3,3,3,3,3,3,3,3,3,3,3,3,3,3,3,3,3,3,3,3,
3,3,3,3,3,3,3,3,3,3,3,3,3,3,3,3,3,3,3,3,3,3,3,3,3,3,3,3,3,3,3,3,3,3,3,3,
3,3,3,4),(-48.0177301301753,-47.8875166216952,-47.769576888226,-47.6689435944054,
-47.5684550152104,-47.4680825030995,-47.367773349246,-47.2674962815413,
-47.1672200683651,-47.0668441433653,-46.966419577951,-46.8658145275858,
-46.7743773697213,-46.6737440759008,-46.5732554967061,-46.4728829845953,
-46.372573830742,-46.2722967630375,-46.1720205498615,-46.0716446248619,
-45.9712200594479,-45.8706150090829,-45.7791778512166,-45.678544557396,
-45.5780559782012,-45.4776834660903,-45.3773743122369,-45.2770972445323,
-45.1768210313562,-45.0764451063565,-44.9760205409424,-44.8754154905773,
-44.7839783327119,-44.6833450388914,-44.5828564596966,-44.4824839475857,
-44.3821747937323,-44.2818977260278,-44.1816215128516,-44.081245587852,
-43.9808210224379,-43.8802159720727,-43.7887788142072,-43.6881455203867,
-43.5876569411918,-43.487284429081,-43.3869752752276,-43.286698207523,-43.1864219943469,
-43.0860460693472,-42.985621503933,-42.8850164535679,-42.7935792957025,
-42.6929460018821,-42.5924574226874,-42.4920849105766,-42.3917757567232,
-42.2914986890187,-42.1912224758426,-42.090846550843,-41.9904219854289,
-41.8898169350638,-41.7983797771978,-41.7345448233619),.UNSPECIFIED.);
#1383=B_SPLINE_CURVE_WITH_KNOTS('',3,(#55692,#55693,#55694,#55695,#55696,
#55697,#55698,#55699,#55700,#55701,#55702,#55703,#55704,#55705,#55706,#55707,
#55708,#55709,#55710,#55711,#55712,#55713,#55714,#55715,#55716,#55717,#55718,
#55719,#55720,#55721,#55722,#55723,#55724,#55725,#55726,#55727,#55728,#55729,
#55730,#55731,#55732,#55733,#55734,#55735,#55736,#55737,#55738,#55739,#55740,
#55741,#55742,#55743,#55744,#55745,#55746,#55747,#55748,#55749,#55750,#55751,
#55752,#55753,#55754,#55755,#55756,#55757,#55758,#55759,#55760,#55761,#55762,
#55763,#55764,#55765,#55766,#55767,#55768,#55769,#55770,#55771,#55772,#55773,
#55774,#55775,#55776,#55777,#55778,#55779,#55780,#55781,#55782,#55783,#55784,
#55785,#55786,#55787,#55788,#55789,#55790,#55791,#55792,#55793,#55794,#55795,
#55796,#55797,#55798,#55799,#55800,#55801,#55802,#55803,#55804,#55805,#55806,
#55807,#55808,#55809,#55810,#55811,#55812,#55813,#55814,#55815,#55816,#55817,
#55818,#55819,#55820,#55821,#55822,#55823,#55824,#55825,#55826,#55827,#55828,
#55829,#55830,#55831,#55832,#55833,#55834,#55835,#55836,#55837,#55838,#55839,
#55840,#55841,#55842,#55843,#55844,#55845,#55846,#55847,#55848,#55849,#55850,
#55851,#55852,#55853,#55854,#55855,#55856,#55857,#55858,#55859,#55860,#55861,
#55862,#55863,#55864,#55865,#55866,#55867,#55868,#55869,#55870,#55871,#55872,
#55873,#55874,#55875,#55876,#55877,#55878,#55879,#55880,#55881,#55882,#55883,
#55884),.UNSPECIFIED.,.F.,.F.,(4,3,3,3,3,3,3,3,3,3,3,3,3,3,3,3,3,3,3,3,
3,3,3,3,3,3,3,3,3,3,3,3,3,3,3,3,3,3,3,3,3,3,3,3,3,3,3,3,3,3,3,3,3,3,3,3,
3,3,3,3,3,3,3,3,4),(-41.7345448229899,-41.6348663122446,-41.5309055555507,
-41.4314723515032,-41.3320923789549,-41.2327332315475,-41.1333625337808,
-41.0338869682092,-40.934349449426,-40.8346519333653,-40.8031802586931,
-40.7025469648726,-40.6020583856776,-40.5016858735667,-40.4013767197132,
-40.3010996520086,-40.2008234388324,-40.1004475138327,-40.0000229484186,
-39.8994178980534,-39.8079807401883,-39.7073474463679,-39.6068588671731,
-39.5064863550622,-39.4061772012088,-39.3059001335042,-39.2056239203282,
-39.1052479953285,-39.0048234299144,-38.9042183795492,-38.8127812216836,
-38.7121479278631,-38.6116593486681,-38.5112868365573,-38.4109776827039,
-38.3107006149993,-38.2104244018232,-38.1100484768235,-38.0096239114096,
-37.9090188610445,-37.8175817031789,-37.7169484093583,-37.6164598301635,
-37.5160873180526,-37.4157781641993,-37.3155010964947,-37.2152248833183,
-37.1148489583186,-37.0144243929046,-36.9138193425394,-36.8223821846742,
-36.7217488908536,-36.6212603116586,-36.5208877995478,-36.4205786456944,
-36.3203015779899,-36.2200253648136,-36.1196494398139,-36.0192248743999,
-35.9186198240348,-35.8271826661695,-35.7136072223652,-35.600451639753,
-35.4880062437431,-35.4513595164066),.UNSPECIFIED.);
#1384=B_SPLINE_CURVE_WITH_KNOTS('',3,(#55886,#55887,#55888,#55889,#55890,
#55891,#55892,#55893,#55894,#55895,#55896,#55897,#55898,#55899,#55900,#55901,
#55902,#55903,#55904,#55905,#55906,#55907,#55908,#55909,#55910,#55911,#55912,
#55913,#55914,#55915,#55916,#55917,#55918,#55919,#55920,#55921,#55922,#55923,
#55924,#55925,#55926,#55927,#55928,#55929,#55930,#55931,#55932,#55933,#55934,
#55935,#55936,#55937,#55938,#55939,#55940,#55941,#55942,#55943,#55944,#55945,
#55946,#55947,#55948,#55949,#55950,#55951,#55952,#55953,#55954,#55955,#55956,
#55957,#55958,#55959,#55960,#55961,#55962,#55963,#55964,#55965,#55966,#55967,
#55968,#55969,#55970,#55971,#55972,#55973,#55974,#55975,#55976,#55977,#55978,
#55979,#55980,#55981,#55982,#55983,#55984,#55985,#55986,#55987,#55988,#55989,
#55990,#55991,#55992,#55993,#55994,#55995,#55996,#55997,#55998,#55999,#56000,
#56001,#56002,#56003,#56004,#56005,#56006,#56007,#56008,#56009,#56010,#56011,
#56012,#56013,#56014,#56015,#56016,#56017,#56018,#56019,#56020,#56021,#56022,
#56023,#56024,#56025,#56026,#56027,#56028,#56029,#56030,#56031,#56032,#56033,
#56034,#56035,#56036,#56037,#56038,#56039,#56040,#56041,#56042,#56043,#56044,
#56045,#56046,#56047,#56048,#56049,#56050,#56051,#56052,#56053,#56054,#56055,
#56056,#56057,#56058,#56059,#56060,#56061,#56062,#56063,#56064,#56065,#56066,
#56067,#56068,#56069,#56070,#56071,#56072,#56073,#56074,#56075),
 .UNSPECIFIED.,.F.,.F.,(4,3,3,3,3,3,3,3,3,3,3,3,3,3,3,3,3,3,3,3,3,3,3,3,
3,3,3,3,3,3,3,3,3,3,3,3,3,3,3,3,3,3,3,3,3,3,3,3,3,3,3,3,3,3,3,3,3,3,3,3,
3,3,3,4),(-35.4513595161824,-35.3502780910073,-35.2491815897649,-35.1448819792399,
-35.0435980657394,-34.9377906067021,-34.8319831476648,-34.7313498538444,
-34.6308612746499,-34.5304887625391,-34.4301796086858,-34.3299025409813,
-34.2296263278054,-34.1292504028059,-34.0288258373918,-33.9282207870267,
-33.8367836291601,-33.7361503353399,-33.6356617561455,-33.5352892440351,
-33.4349800901822,-33.3347030224781,-33.2344268093024,-33.1340508843032,
-33.0336263188895,-32.9330212685249,-32.8415841106554,-32.7409508168336,
-32.6404622376377,-32.5400897255256,-32.4397805716711,-32.3395035039652,
-32.239227290788,-32.1388513657872,-32.0384268003719,-31.9378217500056,
-31.8463845921507,-31.745751298331,-31.6452627191372,-31.5448902070272,
-31.4445810531747,-31.3443039854709,-31.2440277722955,-31.1436518472967,
-31.0432272818834,-30.9426222315191,-30.851185073646,-30.750551779828,-30.6500632006356,
-30.5496906885274,-30.4493815346766,-30.3491044669747,-30.2488282538009,
-30.1484523288039,-30.0480277633924,-29.9474227130299,-29.8559855551413,
-29.7558310335539,-29.6558138224566,-29.555901863842,-29.4560514758558,
-29.3562408059202,-29.2563942120037,-29.1681742090028),.UNSPECIFIED.);
#1385=B_SPLINE_CURVE_WITH_KNOTS('',3,(#56077,#56078,#56079,#56080,#56081,
#56082,#56083,#56084,#56085,#56086,#56087,#56088,#56089,#56090,#56091,#56092,
#56093,#56094,#56095,#56096,#56097,#56098,#56099,#56100,#56101,#56102,#56103,
#56104,#56105,#56106,#56107,#56108,#56109,#56110,#56111,#56112,#56113,#56114,
#56115,#56116,#56117,#56118,#56119,#56120,#56121,#56122,#56123,#56124,#56125,
#56126,#56127,#56128,#56129,#56130,#56131,#56132,#56133,#56134,#56135,#56136,
#56137,#56138,#56139,#56140,#56141,#56142,#56143,#56144,#56145,#56146,#56147,
#56148,#56149,#56150,#56151,#56152,#56153,#56154,#56155,#56156,#56157,#56158,
#56159,#56160,#56161,#56162,#56163,#56164,#56165,#56166,#56167,#56168,#56169,
#56170,#56171,#56172,#56173,#56174,#56175,#56176,#56177,#56178,#56179,#56180,
#56181,#56182,#56183,#56184,#56185,#56186,#56187,#56188,#56189,#56190,#56191,
#56192,#56193,#56194,#56195,#56196,#56197,#56198,#56199,#56200,#56201,#56202,
#56203,#56204,#56205,#56206,#56207,#56208,#56209,#56210,#56211,#56212,#56213,
#56214,#56215,#56216,#56217,#56218,#56219,#56220,#56221,#56222,#56223,#56224,
#56225,#56226,#56227,#56228,#56229,#56230,#56231,#56232,#56233,#56234,#56235,
#56236,#56237,#56238,#56239,#56240,#56241,#56242,#56243,#56244,#56245,#56246,
#56247,#56248,#56249,#56250,#56251,#56252,#56253,#56254,#56255,#56256,#56257,
#56258,#56259,#56260,#56261,#56262,#56263,#56264,#56265,#56266,#56267,#56268,
#56269),.UNSPECIFIED.,.F.,.F.,(4,3,3,3,3,3,3,3,3,3,3,3,3,3,3,3,3,3,3,3,
3,3,3,3,3,3,3,3,3,3,3,3,3,3,3,3,3,3,3,3,3,3,3,3,3,3,3,3,3,3,3,3,3,3,3,3,
3,3,3,3,3,3,3,3,4),(-29.1681742086401,-29.048677086425,-28.9276740828448,
-28.8607860366366,-28.7601527428248,-28.6596641636387,-28.5592916515365,
-28.4589824976917,-28.3587054299956,-28.2584292168279,-28.1580532918364,
-28.0576287264303,-27.957023676073,-27.8655865181318,-27.7649532243258,
-27.6644646451456,-27.5640921330496,-27.4637829792112,-27.3635059115216,
-27.2632296983605,-27.1628537733758,-27.0624292079767,-26.9618241576264,
-26.8703869996271,-26.7697537057427,-26.6692651264839,-26.5688926143092,
-26.468583460392,-26.3683063926239,-26.2680301793844,-26.1676542543223,
-26.0672296888461,-25.9666246384202,-25.8751874811224,-25.7745541873821,
-25.6740656082671,-25.5736930962353,-25.4733839424605,-25.3731068748338,
-25.2728306617349,-25.1724547368107,-25.0720301714713,-24.9714251211786,
-24.8799879626177,-24.7793546688679,-24.6788660897448,-24.5784935777071,
-24.4781844239276,-24.3779073562977,-24.2776311431967,-24.1772552182725,
-24.0768306529341,-23.9762256026443,-23.884788444113,-23.7841551498422,
-23.6836665701958,-23.5832940576337,-23.4829849033294,-23.382707835175,
-23.2824316215506,-23.1820556961083,-23.0816311302539,-22.9810260794576,
-22.8895889256083,-22.8849889018232),.UNSPECIFIED.);
#1386=B_SPLINE_CURVE_WITH_KNOTS('',3,(#56271,#56272,#56273,#56274,#56275,
#56276,#56277,#56278,#56279,#56280,#56281,#56282,#56283,#56284,#56285,#56286,
#56287,#56288,#56289,#56290,#56291,#56292,#56293,#56294,#56295,#56296,#56297,
#56298,#56299,#56300,#56301,#56302,#56303,#56304,#56305,#56306,#56307,#56308,
#56309,#56310,#56311,#56312,#56313,#56314,#56315,#56316,#56317,#56318,#56319,
#56320,#56321,#56322,#56323,#56324,#56325,#56326,#56327,#56328,#56329,#56330,
#56331,#56332,#56333,#56334,#56335,#56336,#56337,#56338,#56339,#56340,#56341,
#56342,#56343,#56344,#56345,#56346,#56347,#56348,#56349,#56350,#56351,#56352,
#56353,#56354,#56355,#56356,#56357,#56358,#56359,#56360,#56361,#56362,#56363,
#56364,#56365,#56366,#56367,#56368,#56369,#56370,#56371,#56372,#56373,#56374,
#56375,#56376,#56377,#56378,#56379,#56380,#56381,#56382,#56383,#56384,#56385,
#56386,#56387,#56388,#56389,#56390,#56391,#56392,#56393,#56394,#56395,#56396,
#56397,#56398,#56399,#56400,#56401,#56402,#56403,#56404,#56405,#56406,#56407,
#56408,#56409,#56410,#56411,#56412,#56413,#56414,#56415,#56416,#56417,#56418,
#56419,#56420,#56421,#56422,#56423,#56424,#56425,#56426,#56427,#56428,#56429,
#56430,#56431,#56432,#56433,#56434,#56435,#56436,#56437,#56438,#56439,#56440,
#56441,#56442,#56443,#56444,#56445,#56446,#56447,#56448,#56449,#56450,#56451,
#56452,#56453,#56454,#56455,#56456,#56457,#56458,#56459,#56460),
 .UNSPECIFIED.,.F.,.F.,(4,3,3,3,3,3,3,3,3,3,3,3,3,3,3,3,3,3,3,3,3,3,3,3,
3,3,3,3,3,3,3,3,3,3,3,3,3,3,3,3,3,3,3,3,3,3,3,3,3,3,3,3,3,3,3,3,3,3,3,3,
3,3,3,4),(-22.8849889015675,-22.7844384795331,-22.6840326799569,-22.5837426163004,
-22.4835155834612,-22.383320192787,-22.2831250957898,-22.182830154689,-22.0824858463468,
-21.9819624781745,-21.8943894071036,-21.7937561135299,-21.69326753459,-21.5928950227447,
-21.4925858691631,-21.3923088017363,-21.2920325888435,-21.1916566641336,
-21.0912320990133,-20.9906270489452,-20.8991898885989,-20.7985565916873,
-20.6980680093904,-20.5976954941759,-20.4973863372192,-20.3971092664161,
-20.2968330501503,-20.1964571220964,-20.0960325536427,-19.995427500298,
-19.9039903700942,-19.8033570818677,-19.7028685082599,-19.6024960016997,
-19.5021868533724,-19.4019097911618,-19.3016335834403,-19.2012576637958,
-19.100833103691,-19.0002280584961,-18.9087908515895,-18.808157557575,-18.7076689782416,
-18.6072964660754,-18.5069873122171,-18.4067102445576,-18.3064340314764,
-18.2060581066479,-18.1056335414471,-18.0050284913629,-17.9135913330848,
-17.8129580186678,-17.7124694187854,-17.6120968859483,-17.5117877113545,
-17.4115106229241,-17.3112343890657,-17.2108584435958,-17.1104338577948,
-17.0098287874223,-16.91839181458,-16.798461421715,-16.6798620946292,-16.6018035950335),
 .UNSPECIFIED.);
#1387=B_SPLINE_CURVE_WITH_KNOTS('',3,(#56462,#56463,#56464,#56465,#56466,
#56467,#56468,#56469,#56470,#56471,#56472,#56473,#56474,#56475,#56476,#56477,
#56478,#56479,#56480,#56481,#56482,#56483,#56484,#56485,#56486,#56487,#56488,
#56489,#56490,#56491,#56492,#56493,#56494,#56495,#56496,#56497,#56498,#56499,
#56500,#56501,#56502,#56503,#56504,#56505,#56506,#56507,#56508,#56509,#56510,
#56511,#56512,#56513,#56514,#56515,#56516,#56517,#56518,#56519,#56520,#56521,
#56522,#56523,#56524,#56525,#56526,#56527,#56528,#56529,#56530,#56531,#56532,
#56533,#56534,#56535,#56536,#56537,#56538,#56539,#56540,#56541,#56542,#56543,
#56544,#56545,#56546,#56547,#56548,#56549,#56550,#56551,#56552,#56553,#56554,
#56555,#56556,#56557,#56558,#56559,#56560,#56561,#56562,#56563,#56564,#56565,
#56566,#56567,#56568,#56569,#56570,#56571,#56572,#56573,#56574,#56575,#56576,
#56577,#56578,#56579,#56580,#56581,#56582,#56583,#56584,#56585,#56586,#56587,
#56588,#56589,#56590,#56591,#56592,#56593,#56594,#56595,#56596,#56597,#56598,
#56599,#56600,#56601,#56602,#56603,#56604,#56605,#56606,#56607,#56608,#56609,
#56610,#56611,#56612,#56613,#56614,#56615,#56616,#56617,#56618,#56619,#56620,
#56621,#56622,#56623,#56624,#56625,#56626,#56627,#56628,#56629,#56630,#56631,
#56632,#56633,#56634,#56635,#56636,#56637,#56638,#56639,#56640,#56641,#56642,
#56643,#56644,#56645,#56646,#56647,#56648,#56649,#56650,#56651,#56652,#56653,
#56654),.UNSPECIFIED.,.F.,.F.,(4,3,3,3,3,3,3,3,3,3,3,3,3,3,3,3,3,3,3,3,
3,3,3,3,3,3,3,3,3,3,3,3,3,3,3,3,3,3,3,3,3,3,3,3,3,3,3,3,3,3,3,3,3,3,3,3,
3,3,3,3,3,3,3,3,4),(-16.6018035946436,-16.5018286166216,-16.4018795570295,
-16.3019248208445,-16.2018628992254,-16.1017459451112,-16.0014471696866,
-15.9231922960753,-15.8225589863926,-15.7220703917125,-15.6216978647484,
-15.5213886964323,-15.421111614672,-15.320835387864,-15.2204594499848,-15.1200348720827,
-15.0194298100292,-14.9279927775706,-14.8273593513153,-14.7268706389542,
-14.6264979932084,-14.5261887054969,-14.4259115038978,-14.3256351569767,
-14.2252590994022,-14.1248344018427,-14.0242292216037,-13.9327932590659,
-13.8321603041925,-13.7316720640727,-13.6312998896521,-13.5309910724934,
-13.4307143400328,-13.3304384601937,-13.2300628632367,-13.1296386234898,
-13.0290338909971,-12.9375937405612,-12.8369602289812,-12.7364714345042,
-12.6360987117923,-12.5357893502765,-12.4355120781078,-12.3352356639284,
-12.2348595447007,-12.1344347884583,-12.0338295551795,-11.9423942220565,
-11.8417601148349,-11.7412707165318,-11.6408973806369,-11.5405874005388,
-11.44030950529,-11.3400324644301,-11.2396557173348,-11.1392303315746,-11.0386244734383,
-10.9471947035518,-10.845900037974,-10.7447544119353,-10.6437275255628,
-10.5427944091178,-10.4419147704534,-10.34104881343,-10.318618287464),
 .UNSPECIFIED.);
#1388=B_SPLINE_CURVE_WITH_KNOTS('',3,(#56655,#56656,#56657,#56658,#56659,
#56660,#56661,#56662,#56663,#56664,#56665,#56666,#56667,#56668,#56669,#56670,
#56671,#56672,#56673,#56674,#56675,#56676,#56677,#56678,#56679,#56680,#56681,
#56682,#56683,#56684,#56685,#56686,#56687,#56688,#56689,#56690,#56691,#56692,
#56693,#56694,#56695,#56696,#56697,#56698,#56699,#56700,#56701,#56702,#56703,
#56704,#56705,#56706,#56707,#56708,#56709,#56710,#56711,#56712,#56713,#56714,
#56715,#56716,#56717,#56718,#56719,#56720,#56721,#56722,#56723,#56724,#56725,
#56726,#56727,#56728,#56729,#56730,#56731,#56732,#56733,#56734,#56735,#56736,
#56737,#56738,#56739,#56740,#56741,#56742,#56743,#56744,#56745,#56746,#56747,
#56748,#56749,#56750,#56751,#56752,#56753,#56754,#56755,#56756,#56757,#56758,
#56759,#56760,#56761,#56762,#56763,#56764,#56765,#56766,#56767,#56768,#56769,
#56770,#56771,#56772,#56773,#56774,#56775,#56776,#56777,#56778,#56779,#56780,
#56781,#56782,#56783,#56784,#56785,#56786,#56787,#56788,#56789,#56790,#56791,
#56792,#56793,#56794,#56795,#56796,#56797,#56798,#56799,#56800,#56801,#56802,
#56803,#56804,#56805,#56806,#56807,#56808,#56809,#56810,#56811,#56812,#56813,
#56814,#56815,#56816,#56817,#56818,#56819,#56820,#56821,#56822,#56823,#56824,
#56825,#56826,#56827,#56828,#56829,#56830,#56831,#56832,#56833,#56834,#56835,
#56836,#56837,#56838,#56839,#56840,#56841,#56842,#56843,#56844,#56845,#56846,
#56847),.UNSPECIFIED.,.F.,.F.,(4,3,3,3,3,3,3,3,3,3,3,3,3,3,3,3,3,3,3,3,
3,3,3,3,3,3,3,3,3,3,3,3,3,3,3,3,3,3,3,3,3,3,3,3,3,3,3,3,3,3,3,3,3,3,3,3,
3,3,3,3,3,3,3,3,4),(-10.3186182872368,-10.2052774276635,-10.0913956938805,
-9.97687885509846,-9.95199518504708,-9.85135960040161,-9.75086874603975,
-9.65049399259817,-9.55018261898653,-9.44990335596195,-9.34962497479173,
-9.24924693936844,-9.14882029168565,-9.04821323050691,-8.95679566654237,
-8.85615769082409,-8.75566438639974,-8.65528710663062,-8.55497316155205,
-8.45469128587806,-8.35441025479137,-8.2540295302673,-8.15360016775222,
-8.0529903808043,-7.96159614803767,-7.86098132409402,-7.76051124718896,
-7.66015719974532,-7.55986647932878,-7.45960778877813,-7.35934987137945,
-7.25899198778301,-7.15858535335808,-7.05799783872295,-6.96639662953296,
-6.8657419231591,-6.76523202542015,-6.66483843365732,-6.56450835497409,
-6.46421054479971,-6.36391379921318,-6.26351781155996,-6.16307340882067,
-6.06244913021843,-5.97119711102825,-5.87053955275317,-5.77002638776563,
-5.66962892692334,-5.56929461557409,-5.46899221832587,-5.36869054009127,
-5.26828911882982,-5.16783899958796,-5.06720860033739,-4.97599759252354,
-4.87631117852719,-4.7767689836149,-4.67734052968798,-4.57797267530372,
-4.47863299114264,-4.37928908656279,-4.27984729266011,-4.18035000264988,
-4.08069243412998,-4.03543298063145),.UNSPECIFIED.);
#1389=B_SPLINE_CURVE_WITH_KNOTS('',3,(#56850,#56851,#56852,#56853,#56854,
#56855,#56856,#56857,#56858,#56859,#56860,#56861,#56862,#56863,#56864,#56865,
#56866,#56867,#56868,#56869,#56870,#56871,#56872,#56873,#56874,#56875,#56876,
#56877,#56878,#56879,#56880,#56881,#56882,#56883,#56884,#56885,#56886,#56887,
#56888,#56889),.UNSPECIFIED.,.F.,.F.,(4,3,3,3,3,3,3,3,3,3,3,3,3,4),(177.819192458502,
177.870849877951,177.976746287652,178.087909176253,178.193518105667,178.299063112442,
178.404580569928,178.510106809205,178.615746262861,178.721451484676,178.827334848772,
178.866049396456,179.014820834809,179.070781254618),.UNSPECIFIED.);
#1390=B_SPLINE_CURVE_WITH_KNOTS('',3,(#56891,#56892,#56893,#56894,#56895,
#56896,#56897,#56898,#56899,#56900,#56901,#56902,#56903,#56904,#56905,#56906,
#56907,#56908,#56909,#56910,#56911,#56912,#56913,#56914,#56915,#56916,#56917,
#56918,#56919,#56920,#56921,#56922,#56923,#56924,#56925,#56926,#56927,#56928,
#56929,#56930,#56931,#56932,#56933,#56934,#56935,#56936,#56937,#56938,#56939,
#56940,#56941,#56942,#56943,#56944,#56945,#56946,#56947,#56948,#56949,#56950,
#56951,#56952,#56953,#56954,#56955,#56956,#56957,#56958,#56959,#56960,#56961,
#56962,#56963,#56964,#56965,#56966,#56967,#56968,#56969,#56970,#56971,#56972,
#56973,#56974,#56975,#56976,#56977,#56978,#56979,#56980,#56981,#56982,#56983,
#56984,#56985,#56986,#56987,#56988,#56989,#56990,#56991,#56992,#56993,#56994,
#56995,#56996,#56997,#56998,#56999,#57000,#57001,#57002,#57003,#57004,#57005,
#57006,#57007,#57008),.UNSPECIFIED.,.F.,.F.,(4,3,3,3,3,3,3,3,3,3,3,3,3,
3,3,3,3,3,3,3,3,3,3,3,3,3,3,3,3,3,3,3,3,3,3,3,3,3,3,4),(179.07078125494,
179.174995091213,179.279122198882,179.383200887903,179.487269395697,179.591434908581,
179.695652687092,179.800050733087,179.86124891496,179.966984731998,180.072561027452,
180.178013820682,180.283401178045,180.388759713088,180.49412599568,180.59960664732,
180.705152489819,180.810881328432,180.856448433465,180.962518989792,181.073660110064,
181.179441227978,181.285157249995,181.39084428965,181.496538416766,181.602342168825,
181.708209802484,181.814251277373,181.85164795197,181.957645557193,182.068795796353,
182.174511996658,182.280166179011,182.385794524185,182.491433172546,182.597186535568,
182.703006662787,182.809005320892,182.846847470474,182.852224483266),
 .UNSPECIFIED.);
#1391=B_SPLINE_CURVE_WITH_KNOTS('',3,(#57012,#57013,#57014,#57015,#57016,
#57017,#57018,#57019,#57020,#57021,#57022,#57023,#57024,#57025,#57026,#57027,
#57028,#57029,#57030,#57031,#57032,#57033,#57034,#57035,#57036,#57037,#57038,
#57039,#57040,#57041,#57042,#57043,#57044,#57045,#57046,#57047,#57048,#57049,
#57050,#57051,#57052,#57053,#57054,#57055,#57056,#57057,#57058,#57059,#57060,
#57061,#57062,#57063,#57064,#57065,#57066,#57067,#57068,#57069,#57070,#57071,
#57072,#57073,#57074,#57075,#57076,#57077,#57078,#57079,#57080,#57081,#57082,
#57083,#57084),.UNSPECIFIED.,.F.,.F.,(4,3,3,3,3,3,3,3,3,3,3,3,3,3,3,3,3,
3,3,3,3,3,3,3,4),(179.070781255096,179.185620068578,179.300780012931,179.416435972135,
179.507913446056,179.612695797115,179.717318404753,179.821821446474,179.926261807326,
180.030677319518,180.135105774966,180.239662568643,180.34429093876,180.44912182172,
180.503112964561,180.611895504391,180.722697626725,180.831119906092,180.939439767263,
181.047686885078,181.160343284574,181.268563069598,181.376793276413,181.485096017127,
181.498312483065),.UNSPECIFIED.);
#1392=B_SPLINE_CURVE_WITH_KNOTS('',3,(#57085,#57086,#57087,#57088,#57089,
#57090,#57091,#57092,#57093,#57094,#57095,#57096,#57097,#57098,#57099,#57100,
#57101,#57102,#57103,#57104,#57105,#57106,#57107,#57108,#57109,#57110,#57111,
#57112,#57113,#57114,#57115,#57116,#57117,#57118,#57119,#57120,#57121,#57122,
#57123,#57124,#57125,#57126,#57127,#57128,#57129,#57130,#57131,#57132,#57133,
#57134,#57135,#57136,#57137,#57138),.UNSPECIFIED.,.F.,.F.,(4,2,2,2,2,2,
2,2,2,2,2,2,2,2,2,2,2,2,2,2,2,2,2,2,2,2,4),(-2.43068563765362,-2.42265074372402,
-2.42024534622642,-2.41836210929473,-2.41647245656861,-2.414316274935,-2.41077045154461,
-2.39913112758483,-2.3524461932698,-2.3299497556685,-2.32572060496249,-2.32408420621342,
-2.32294866987872,-2.32192931846328,-2.32025802836276,-2.31602250759433,
-2.27620058838792,-2.24816465604659,-2.23858750987126,-2.23396094982001,
-2.23119225346768,-2.22870741324186,-2.22680052548476,-2.22497300025956,
-2.22243828418116,-2.21585189577543,-2.18872254859161),.UNSPECIFIED.);
#1393=B_SPLINE_CURVE_WITH_KNOTS('',3,(#57142,#57143,#57144,#57145,#57146,
#57147,#57148,#57149,#57150,#57151,#57152,#57153,#57154,#57155,#57156,#57157,
#57158,#57159,#57160,#57161,#57162,#57163,#57164,#57165,#57166,#57167,#57168,
#57169,#57170,#57171,#57172,#57173,#57174,#57175,#57176,#57177,#57178,#57179,
#57180,#57181,#57182,#57183,#57184,#57185,#57186,#57187,#57188,#57189,#57190,
#57191,#57192,#57193,#57194,#57195,#57196,#57197,#57198,#57199,#57200,#57201,
#57202,#57203,#57204,#57205,#57206,#57207,#57208,#57209,#57210,#57211,#57212,
#57213,#57214,#57215,#57216,#57217,#57218,#57219,#57220,#57221,#57222,#57223),
 .UNSPECIFIED.,.F.,.F.,(4,3,3,3,3,3,3,3,3,3,3,3,3,3,3,3,3,3,3,3,3,3,3,3,
3,3,3,4),(-0.423947533719778,-0.398852588470169,-0.377228555616947,-0.372439199709838,
-0.34764842283439,-0.329741977315031,-0.325329288343292,-0.321149784672366,
-0.296981160184881,-0.273087580671514,-0.249893960726593,-0.243157362702744,
-0.239407499053117,-0.235386549537422,-0.212468228537641,-0.204405790338345,
-0.180908491206444,-0.158373335170994,-0.153625676807497,-0.130854845993313,
-0.108177017216731,-0.0856898081540444,-0.0774429266195629,-0.0739031774787725,
-0.0519698695588112,-0.0306589296986993,-0.0096285538345829,0.),
 .UNSPECIFIED.);
#1394=B_SPLINE_CURVE_WITH_KNOTS('',3,(#57224,#57225,#57226,#57227,#57228,
#57229,#57230,#57231,#57232,#57233,#57234,#57235,#57236,#57237,#57238,#57239,
#57240,#57241,#57242,#57243,#57244,#57245,#57246,#57247,#57248,#57249,#57250,
#57251,#57252,#57253,#57254,#57255,#57256,#57257,#57258,#57259,#57260,#57261,
#57262,#57263,#57264,#57265,#57266,#57267,#57268,#57269,#57270,#57271,#57272,
#57273,#57274,#57275,#57276,#57277,#57278,#57279,#57280,#57281,#57282,#57283,
#57284,#57285,#57286,#57287,#57288,#57289,#57290,#57291,#57292,#57293,#57294,
#57295,#57296,#57297,#57298,#57299,#57300,#57301,#57302),.UNSPECIFIED.,
 .F.,.F.,(4,3,3,3,3,3,3,3,3,3,3,3,3,3,3,3,3,3,3,3,3,3,3,3,3,3,4),(-0.430289127733703,
-0.409131203295475,-0.391054495122007,-0.386034754015406,-0.363993110999897,
-0.346793254452062,-0.34223698527339,-0.337890536404446,-0.315048607800531,
-0.292209214405036,-0.269344703384665,-0.26200185233298,-0.25827143431592,
-0.234557662948815,-0.226394258617215,-0.203257661985663,-0.180121065354112,
-0.174814354906448,-0.151194220490317,-0.126840078836855,-0.102485937183392,
-0.0922144100858579,-0.0875882430594912,-0.0625337202221519,-0.0374931773906202,
-0.0129486697203148,0.),.UNSPECIFIED.);
#1395=B_SPLINE_CURVE_WITH_KNOTS('',3,(#58011,#58012,#58013,#58014),
 .UNSPECIFIED.,.F.,.F.,(4,4),(-0.0445064912682737,0.),.UNSPECIFIED.);
#1396=B_SPLINE_CURVE_WITH_KNOTS('',3,(#58015,#58016,#58017,#58018,#58019,
#58020,#58021,#58022,#58023,#58024,#58025,#58026,#58027,#58028,#58029,#58030,
#58031,#58032,#58033,#58034,#58035,#58036,#58037,#58038,#58039,#58040,#58041,
#58042,#58043,#58044,#58045,#58046,#58047,#58048,#58049,#58050,#58051,#58052,
#58053,#58054,#58055,#58056,#58057,#58058,#58059,#58060,#58061,#58062,#58063,
#58064,#58065,#58066,#58067,#58068,#58069,#58070,#58071,#58072,#58073,#58074,
#58075,#58076,#58077,#58078,#58079,#58080,#58081,#58082,#58083,#58084,#58085,
#58086,#58087,#58088,#58089,#58090,#58091,#58092,#58093),.UNSPECIFIED.,
 .F.,.F.,(4,3,3,3,3,3,3,3,3,3,3,3,3,3,3,3,3,3,3,3,3,3,3,3,3,3,4),(-0.430289127733828,
-0.409131192513218,-0.391054556741682,-0.386034835281542,-0.364002044843779,
-0.346793321163048,-0.342237084883542,-0.337890550896376,-0.315216893040039,
-0.292164481757858,-0.275755482800676,-0.262001866763717,-0.25827145905283,
-0.234557688497016,-0.226394258617259,-0.203257656753551,-0.180121054889843,
-0.174814354294875,-0.15112100411559,-0.126993562280297,-0.102598702378716,
-0.0922144183311342,-0.0875882464310277,-0.0626034767801118,-0.0376323704312253,
-0.0129486879091254,0.),.UNSPECIFIED.);
#1397=B_SPLINE_CURVE_WITH_KNOTS('',3,(#58098,#58099,#58100,#58101,#58102,
#58103,#58104,#58105,#58106,#58107,#58108,#58109,#58110,#58111,#58112,#58113,
#58114,#58115,#58116,#58117,#58118,#58119,#58120,#58121,#58122,#58123,#58124,
#58125,#58126,#58127,#58128,#58129,#58130,#58131,#58132,#58133,#58134,#58135,
#58136,#58137,#58138,#58139,#58140,#58141,#58142,#58143,#58144,#58145,#58146,
#58147,#58148,#58149,#58150,#58151,#58152,#58153,#58154,#58155,#58156,#58157,
#58158,#58159,#58160,#58161,#58162,#58163,#58164,#58165,#58166,#58167,#58168,
#58169,#58170,#58171,#58172,#58173,#58174,#58175,#58176,#58177,#58178,#58179),
 .UNSPECIFIED.,.F.,.F.,(4,3,3,3,3,3,3,3,3,3,3,3,3,3,3,3,3,3,3,3,3,3,3,3,
3,3,3,4),(-0.423947483310156,-0.39885253768024,-0.377228574786393,-0.37243923473487,
-0.347648458633374,-0.329742008624217,-0.325329264085242,-0.32114978023783,
-0.297024106120711,-0.273297481373415,-0.256074558614657,-0.24315736654559,
-0.239407516802922,-0.235386554398844,-0.212468243691861,-0.204405790338385,
-0.180908493451503,-0.158373340852528,-0.153625676577744,-0.130854850040819,
-0.108177012449888,-0.0856897908532072,-0.077442917873118,-0.073903169216813,
-0.051969851848939,-0.0306588946937463,-0.00962849885639309,-7.64403705571099E-15),
 .UNSPECIFIED.);
#1398=B_SPLINE_CURVE_WITH_KNOTS('',3,(#58889,#58890,#58891,#58892),
 .UNSPECIFIED.,.F.,.F.,(4,4),(-0.0446329464765972,0.),.UNSPECIFIED.);
#1561=FACE_BOUND('',#3126,.T.);
#1562=FACE_BOUND('',#3240,.T.);
#1777=PLANE('',#14393);
#1778=PLANE('',#14395);
#1779=PLANE('',#14401);
#1780=PLANE('',#14405);
#1781=PLANE('',#14406);
#1782=PLANE('',#14407);
#1783=PLANE('',#14408);
#1784=PLANE('',#14448);
#1785=PLANE('',#14450);
#1786=PLANE('',#14451);
#1787=PLANE('',#14488);
#1788=PLANE('',#14489);
#1789=PLANE('',#14490);
#1790=PLANE('',#14491);
#1791=PLANE('',#14492);
#1792=PLANE('',#14493);
#1793=PLANE('',#14494);
#1794=PLANE('',#14495);
#1795=PLANE('',#14496);
#1796=PLANE('',#14497);
#1797=PLANE('',#14498);
#1798=PLANE('',#14499);
#1799=PLANE('',#14500);
#1800=PLANE('',#14501);
#1801=PLANE('',#14502);
#1802=PLANE('',#14503);
#1803=PLANE('',#14504);
#1804=PLANE('',#14505);
#1805=PLANE('',#14506);
#1806=PLANE('',#14507);
#1807=PLANE('',#14508);
#1808=PLANE('',#14509);
#1809=PLANE('',#14510);
#1810=PLANE('',#14511);
#1811=PLANE('',#14512);
#1812=PLANE('',#14513);
#1813=PLANE('',#14514);
#1814=PLANE('',#14515);
#1815=PLANE('',#14516);
#1816=PLANE('',#14517);
#1817=PLANE('',#14518);
#1818=PLANE('',#14519);
#1819=PLANE('',#14520);
#1820=PLANE('',#14521);
#1821=PLANE('',#14522);
#1822=PLANE('',#14523);
#1823=PLANE('',#14524);
#1824=PLANE('',#14525);
#1825=PLANE('',#14526);
#1826=PLANE('',#14527);
#1827=PLANE('',#14528);
#1828=PLANE('',#14529);
#1829=PLANE('',#14530);
#1830=PLANE('',#14531);
#1831=PLANE('',#14532);
#1832=PLANE('',#14533);
#1833=PLANE('',#14534);
#1834=PLANE('',#14535);
#1835=PLANE('',#14536);
#1836=PLANE('',#14537);
#1837=PLANE('',#14538);
#1838=PLANE('',#14539);
#1839=PLANE('',#14540);
#1840=PLANE('',#14541);
#1841=PLANE('',#14542);
#1842=PLANE('',#14543);
#1843=PLANE('',#14544);
#1844=PLANE('',#14545);
#1845=PLANE('',#14546);
#1846=PLANE('',#14547);
#1847=PLANE('',#14548);
#1848=PLANE('',#14549);
#1849=PLANE('',#14550);
#1850=PLANE('',#14551);
#1851=PLANE('',#14552);
#1852=PLANE('',#14553);
#1853=PLANE('',#14554);
#1854=PLANE('',#14555);
#1855=PLANE('',#14556);
#1856=PLANE('',#14557);
#1857=PLANE('',#14558);
#1858=PLANE('',#14559);
#1859=PLANE('',#14560);
#1860=PLANE('',#14561);
#1861=PLANE('',#14562);
#1862=PLANE('',#14563);
#1863=PLANE('',#14564);
#1864=PLANE('',#14565);
#1865=PLANE('',#14566);
#1866=PLANE('',#14567);
#1867=PLANE('',#14568);
#1868=PLANE('',#14569);
#1869=PLANE('',#14570);
#1870=PLANE('',#14571);
#1871=PLANE('',#14572);
#1872=PLANE('',#14573);
#1873=PLANE('',#14574);
#1874=PLANE('',#14575);
#1875=PLANE('',#14576);
#1876=PLANE('',#14577);
#1877=PLANE('',#14578);
#1878=PLANE('',#14579);
#1879=PLANE('',#14580);
#1880=PLANE('',#14581);
#1881=PLANE('',#14582);
#1882=PLANE('',#14583);
#1883=PLANE('',#14584);
#1884=PLANE('',#14585);
#1885=PLANE('',#14586);
#1886=PLANE('',#14587);
#1887=PLANE('',#14588);
#1888=PLANE('',#14589);
#1889=PLANE('',#14590);
#1890=PLANE('',#14591);
#1891=PLANE('',#14593);
#1892=PLANE('',#14595);
#1893=PLANE('',#14597);
#1894=PLANE('',#14599);
#1895=PLANE('',#14601);
#1896=PLANE('',#14604);
#1897=PLANE('',#14605);
#1898=PLANE('',#14606);
#1899=PLANE('',#14607);
#1900=PLANE('',#14608);
#1901=PLANE('',#14609);
#2366=FACE_OUTER_BOUND('',#3091,.T.);
#2367=FACE_OUTER_BOUND('',#3092,.T.);
#2368=FACE_OUTER_BOUND('',#3093,.T.);
#2369=FACE_OUTER_BOUND('',#3094,.T.);
#2370=FACE_OUTER_BOUND('',#3095,.T.);
#2371=FACE_OUTER_BOUND('',#3096,.T.);
#2372=FACE_OUTER_BOUND('',#3097,.T.);
#2373=FACE_OUTER_BOUND('',#3098,.T.);
#2374=FACE_OUTER_BOUND('',#3099,.T.);
#2375=FACE_OUTER_BOUND('',#3100,.T.);
#2376=FACE_OUTER_BOUND('',#3101,.T.);
#2377=FACE_OUTER_BOUND('',#3102,.T.);
#2378=FACE_OUTER_BOUND('',#3103,.T.);
#2379=FACE_OUTER_BOUND('',#3104,.T.);
#2380=FACE_OUTER_BOUND('',#3105,.T.);
#2381=FACE_OUTER_BOUND('',#3106,.T.);
#2382=FACE_OUTER_BOUND('',#3107,.T.);
#2383=FACE_OUTER_BOUND('',#3108,.T.);
#2384=FACE_OUTER_BOUND('',#3109,.T.);
#2385=FACE_OUTER_BOUND('',#3110,.T.);
#2386=FACE_OUTER_BOUND('',#3111,.T.);
#2387=FACE_OUTER_BOUND('',#3112,.T.);
#2388=FACE_OUTER_BOUND('',#3113,.T.);
#2389=FACE_OUTER_BOUND('',#3114,.T.);
#2390=FACE_OUTER_BOUND('',#3115,.T.);
#2391=FACE_OUTER_BOUND('',#3116,.T.);
#2392=FACE_OUTER_BOUND('',#3117,.T.);
#2393=FACE_OUTER_BOUND('',#3118,.T.);
#2394=FACE_OUTER_BOUND('',#3119,.T.);
#2395=FACE_OUTER_BOUND('',#3120,.T.);
#2396=FACE_OUTER_BOUND('',#3121,.T.);
#2397=FACE_OUTER_BOUND('',#3122,.T.);
#2398=FACE_OUTER_BOUND('',#3123,.T.);
#2399=FACE_OUTER_BOUND('',#3124,.T.);
#2400=FACE_OUTER_BOUND('',#3125,.T.);
#2401=FACE_OUTER_BOUND('',#3127,.T.);
#2402=FACE_OUTER_BOUND('',#3128,.T.);
#2403=FACE_OUTER_BOUND('',#3129,.T.);
#2404=FACE_OUTER_BOUND('',#3130,.T.);
#2405=FACE_OUTER_BOUND('',#3131,.T.);
#2406=FACE_OUTER_BOUND('',#3132,.T.);
#2407=FACE_OUTER_BOUND('',#3133,.T.);
#2408=FACE_OUTER_BOUND('',#3134,.T.);
#2409=FACE_OUTER_BOUND('',#3135,.T.);
#2410=FACE_OUTER_BOUND('',#3136,.T.);
#2411=FACE_OUTER_BOUND('',#3137,.T.);
#2412=FACE_OUTER_BOUND('',#3138,.T.);
#2413=FACE_OUTER_BOUND('',#3139,.T.);
#2414=FACE_OUTER_BOUND('',#3140,.T.);
#2415=FACE_OUTER_BOUND('',#3141,.T.);
#2416=FACE_OUTER_BOUND('',#3142,.T.);
#2417=FACE_OUTER_BOUND('',#3143,.T.);
#2418=FACE_OUTER_BOUND('',#3144,.T.);
#2419=FACE_OUTER_BOUND('',#3145,.T.);
#2420=FACE_OUTER_BOUND('',#3146,.T.);
#2421=FACE_OUTER_BOUND('',#3147,.T.);
#2422=FACE_OUTER_BOUND('',#3148,.T.);
#2423=FACE_OUTER_BOUND('',#3149,.T.);
#2424=FACE_OUTER_BOUND('',#3150,.T.);
#2425=FACE_OUTER_BOUND('',#3151,.T.);
#2426=FACE_OUTER_BOUND('',#3152,.T.);
#2427=FACE_OUTER_BOUND('',#3153,.T.);
#2428=FACE_OUTER_BOUND('',#3154,.T.);
#2429=FACE_OUTER_BOUND('',#3155,.T.);
#2430=FACE_OUTER_BOUND('',#3156,.T.);
#2431=FACE_OUTER_BOUND('',#3157,.T.);
#2432=FACE_OUTER_BOUND('',#3158,.T.);
#2433=FACE_OUTER_BOUND('',#3159,.T.);
#2434=FACE_OUTER_BOUND('',#3160,.T.);
#2435=FACE_OUTER_BOUND('',#3161,.T.);
#2436=FACE_OUTER_BOUND('',#3162,.T.);
#2437=FACE_OUTER_BOUND('',#3163,.T.);
#2438=FACE_OUTER_BOUND('',#3164,.T.);
#2439=FACE_OUTER_BOUND('',#3165,.T.);
#2440=FACE_OUTER_BOUND('',#3166,.T.);
#2441=FACE_OUTER_BOUND('',#3167,.T.);
#2442=FACE_OUTER_BOUND('',#3168,.T.);
#2443=FACE_OUTER_BOUND('',#3169,.T.);
#2444=FACE_OUTER_BOUND('',#3170,.T.);
#2445=FACE_OUTER_BOUND('',#3171,.T.);
#2446=FACE_OUTER_BOUND('',#3172,.T.);
#2447=FACE_OUTER_BOUND('',#3173,.T.);
#2448=FACE_OUTER_BOUND('',#3174,.T.);
#2449=FACE_OUTER_BOUND('',#3175,.T.);
#2450=FACE_OUTER_BOUND('',#3176,.T.);
#2451=FACE_OUTER_BOUND('',#3177,.T.);
#2452=FACE_OUTER_BOUND('',#3178,.T.);
#2453=FACE_OUTER_BOUND('',#3179,.T.);
#2454=FACE_OUTER_BOUND('',#3180,.T.);
#2455=FACE_OUTER_BOUND('',#3181,.T.);
#2456=FACE_OUTER_BOUND('',#3182,.T.);
#2457=FACE_OUTER_BOUND('',#3183,.T.);
#2458=FACE_OUTER_BOUND('',#3184,.T.);
#2459=FACE_OUTER_BOUND('',#3185,.T.);
#2460=FACE_OUTER_BOUND('',#3186,.T.);
#2461=FACE_OUTER_BOUND('',#3187,.T.);
#2462=FACE_OUTER_BOUND('',#3188,.T.);
#2463=FACE_OUTER_BOUND('',#3189,.T.);
#2464=FACE_OUTER_BOUND('',#3190,.T.);
#2465=FACE_OUTER_BOUND('',#3191,.T.);
#2466=FACE_OUTER_BOUND('',#3192,.T.);
#2467=FACE_OUTER_BOUND('',#3193,.T.);
#2468=FACE_OUTER_BOUND('',#3194,.T.);
#2469=FACE_OUTER_BOUND('',#3195,.T.);
#2470=FACE_OUTER_BOUND('',#3196,.T.);
#2471=FACE_OUTER_BOUND('',#3197,.T.);
#2472=FACE_OUTER_BOUND('',#3198,.T.);
#2473=FACE_OUTER_BOUND('',#3199,.T.);
#2474=FACE_OUTER_BOUND('',#3200,.T.);
#2475=FACE_OUTER_BOUND('',#3201,.T.);
#2476=FACE_OUTER_BOUND('',#3202,.T.);
#2477=FACE_OUTER_BOUND('',#3203,.T.);
#2478=FACE_OUTER_BOUND('',#3204,.T.);
#2479=FACE_OUTER_BOUND('',#3205,.T.);
#2480=FACE_OUTER_BOUND('',#3206,.T.);
#2481=FACE_OUTER_BOUND('',#3207,.T.);
#2482=FACE_OUTER_BOUND('',#3208,.T.);
#2483=FACE_OUTER_BOUND('',#3209,.T.);
#2484=FACE_OUTER_BOUND('',#3210,.T.);
#2485=FACE_OUTER_BOUND('',#3211,.T.);
#2486=FACE_OUTER_BOUND('',#3212,.T.);
#2487=FACE_OUTER_BOUND('',#3213,.T.);
#2488=FACE_OUTER_BOUND('',#3214,.T.);
#2489=FACE_OUTER_BOUND('',#3215,.T.);
#2490=FACE_OUTER_BOUND('',#3216,.T.);
#2491=FACE_OUTER_BOUND('',#3217,.T.);
#2492=FACE_OUTER_BOUND('',#3218,.T.);
#2493=FACE_OUTER_BOUND('',#3219,.T.);
#2494=FACE_OUTER_BOUND('',#3220,.T.);
#2495=FACE_OUTER_BOUND('',#3221,.T.);
#2496=FACE_OUTER_BOUND('',#3222,.T.);
#2497=FACE_OUTER_BOUND('',#3223,.T.);
#2498=FACE_OUTER_BOUND('',#3224,.T.);
#2499=FACE_OUTER_BOUND('',#3225,.T.);
#2500=FACE_OUTER_BOUND('',#3226,.T.);
#2501=FACE_OUTER_BOUND('',#3227,.T.);
#2502=FACE_OUTER_BOUND('',#3228,.T.);
#2503=FACE_OUTER_BOUND('',#3229,.T.);
#2504=FACE_OUTER_BOUND('',#3230,.T.);
#2505=FACE_OUTER_BOUND('',#3231,.T.);
#2506=FACE_OUTER_BOUND('',#3232,.T.);
#2507=FACE_OUTER_BOUND('',#3233,.T.);
#2508=FACE_OUTER_BOUND('',#3234,.T.);
#2509=FACE_OUTER_BOUND('',#3235,.T.);
#2510=FACE_OUTER_BOUND('',#3236,.T.);
#2511=FACE_OUTER_BOUND('',#3237,.T.);
#2512=FACE_OUTER_BOUND('',#3238,.T.);
#2513=FACE_OUTER_BOUND('',#3239,.T.);
#2514=FACE_OUTER_BOUND('',#3241,.T.);
#2515=FACE_OUTER_BOUND('',#3242,.T.);
#2516=FACE_OUTER_BOUND('',#3243,.T.);
#2517=FACE_OUTER_BOUND('',#3244,.T.);
#2518=FACE_OUTER_BOUND('',#3245,.T.);
#2519=FACE_OUTER_BOUND('',#3246,.T.);
#2520=FACE_OUTER_BOUND('',#3247,.T.);
#2521=FACE_OUTER_BOUND('',#3248,.T.);
#2522=FACE_OUTER_BOUND('',#3249,.T.);
#2523=FACE_OUTER_BOUND('',#3250,.T.);
#2524=FACE_OUTER_BOUND('',#3251,.T.);
#2525=FACE_OUTER_BOUND('',#3252,.T.);
#2526=FACE_OUTER_BOUND('',#3253,.T.);
#3091=EDGE_LOOP('',(#10847,#10848,#10849,#10850));
#3092=EDGE_LOOP('',(#10851,#10852,#10853,#10854,#10855,#10856));
#3093=EDGE_LOOP('',(#10857,#10858,#10859,#10860,#10861));
#3094=EDGE_LOOP('',(#10862,#10863,#10864,#10865,#10866));
#3095=EDGE_LOOP('',(#10867,#10868,#10869,#10870,#10871));
#3096=EDGE_LOOP('',(#10872,#10873,#10874,#10875,#10876));
#3097=EDGE_LOOP('',(#10877,#10878,#10879,#10880,#10881));
#3098=EDGE_LOOP('',(#10882,#10883,#10884,#10885,#10886));
#3099=EDGE_LOOP('',(#10887,#10888,#10889,#10890,#10891));
#3100=EDGE_LOOP('',(#10892,#10893,#10894,#10895,#10896));
#3101=EDGE_LOOP('',(#10897,#10898,#10899,#10900,#10901));
#3102=EDGE_LOOP('',(#10902,#10903,#10904,#10905,#10906));
#3103=EDGE_LOOP('',(#10907,#10908,#10909,#10910,#10911));
#3104=EDGE_LOOP('',(#10912,#10913,#10914,#10915,#10916));
#3105=EDGE_LOOP('',(#10917,#10918,#10919,#10920,#10921));
#3106=EDGE_LOOP('',(#10922,#10923,#10924,#10925,#10926));
#3107=EDGE_LOOP('',(#10927,#10928,#10929,#10930,#10931));
#3108=EDGE_LOOP('',(#10932,#10933,#10934,#10935,#10936));
#3109=EDGE_LOOP('',(#10937,#10938,#10939,#10940,#10941));
#3110=EDGE_LOOP('',(#10942,#10943,#10944,#10945,#10946));
#3111=EDGE_LOOP('',(#10947,#10948,#10949,#10950,#10951));
#3112=EDGE_LOOP('',(#10952,#10953,#10954,#10955,#10956,#10957));
#3113=EDGE_LOOP('',(#10958,#10959,#10960,#10961));
#3114=EDGE_LOOP('',(#10962,#10963,#10964,#10965,#10966,#10967));
#3115=EDGE_LOOP('',(#10968,#10969,#10970,#10971,#10972));
#3116=EDGE_LOOP('',(#10973,#10974,#10975,#10976,#10977));
#3117=EDGE_LOOP('',(#10978,#10979,#10980,#10981,#10982));
#3118=EDGE_LOOP('',(#10983,#10984,#10985,#10986,#10987,#10988,#10989,#10990,
#10991,#10992,#10993,#10994,#10995,#10996,#10997,#10998,#10999,#11000,#11001,
#11002,#11003,#11004,#11005,#11006,#11007,#11008,#11009,#11010,#11011,#11012,
#11013,#11014,#11015,#11016,#11017,#11018,#11019,#11020,#11021,#11022,#11023,
#11024,#11025,#11026,#11027,#11028,#11029,#11030,#11031,#11032,#11033,#11034,
#11035,#11036,#11037,#11038,#11039,#11040,#11041,#11042));
#3119=EDGE_LOOP('',(#11043,#11044,#11045,#11046,#11047,#11048));
#3120=EDGE_LOOP('',(#11049,#11050,#11051,#11052));
#3121=EDGE_LOOP('',(#11053,#11054,#11055,#11056,#11057,#11058,#11059,#11060,
#11061,#11062,#11063,#11064,#11065,#11066,#11067,#11068,#11069,#11070,#11071,
#11072,#11073,#11074,#11075,#11076,#11077,#11078,#11079,#11080,#11081,#11082,
#11083,#11084,#11085,#11086,#11087,#11088,#11089,#11090,#11091,#11092,#11093,
#11094,#11095,#11096,#11097,#11098,#11099,#11100,#11101,#11102,#11103,#11104,
#11105,#11106,#11107,#11108,#11109,#11110,#11111,#11112,#11113,#11114,#11115,
#11116,#11117,#11118,#11119,#11120,#11121,#11122,#11123,#11124,#11125,#11126,
#11127));
#3122=EDGE_LOOP('',(#11128,#11129,#11130,#11131,#11132));
#3123=EDGE_LOOP('',(#11133,#11134,#11135,#11136,#11137,#11138,#11139,#11140,
#11141,#11142,#11143,#11144,#11145,#11146,#11147,#11148,#11149,#11150,#11151,
#11152,#11153,#11154,#11155,#11156,#11157,#11158,#11159,#11160,#11161,#11162,
#11163,#11164,#11165,#11166,#11167,#11168,#11169,#11170,#11171,#11172,#11173,
#11174,#11175,#11176,#11177,#11178,#11179,#11180,#11181,#11182,#11183,#11184,
#11185,#11186,#11187,#11188,#11189,#11190,#11191,#11192,#11193,#11194,#11195,
#11196,#11197,#11198,#11199,#11200,#11201,#11202,#11203,#11204,#11205,#11206));
#3124=EDGE_LOOP('',(#11207,#11208,#11209,#11210,#11211,#11212,#11213));
#3125=EDGE_LOOP('',(#11214));
#3126=EDGE_LOOP('',(#11215));
#3127=EDGE_LOOP('',(#11216,#11217,#11218,#11219,#11220,#11221,#11222));
#3128=EDGE_LOOP('',(#11223));
#3129=EDGE_LOOP('',(#11224,#11225,#11226,#11227));
#3130=EDGE_LOOP('',(#11228,#11229,#11230,#11231));
#3131=EDGE_LOOP('',(#11232,#11233,#11234));
#3132=EDGE_LOOP('',(#11235,#11236,#11237,#11238,#11239,#11240,#11241,#11242,
#11243,#11244,#11245,#11246,#11247,#11248,#11249,#11250,#11251,#11252,#11253,
#11254,#11255,#11256,#11257,#11258,#11259,#11260,#11261,#11262,#11263,#11264,
#11265,#11266,#11267,#11268,#11269,#11270,#11271,#11272,#11273,#11274,#11275,
#11276,#11277,#11278,#11279,#11280,#11281,#11282,#11283,#11284,#11285,#11286,
#11287,#11288,#11289,#11290,#11291,#11292,#11293,#11294,#11295,#11296,#11297,
#11298,#11299,#11300,#11301,#11302,#11303,#11304,#11305,#11306,#11307,#11308,
#11309,#11310,#11311,#11312,#11313,#11314,#11315,#11316,#11317,#11318,#11319,
#11320,#11321,#11322,#11323,#11324,#11325,#11326,#11327,#11328,#11329,#11330,
#11331,#11332,#11333,#11334,#11335,#11336,#11337,#11338,#11339,#11340,#11341,
#11342,#11343,#11344,#11345));
#3133=EDGE_LOOP('',(#11346,#11347,#11348));
#3134=EDGE_LOOP('',(#11349,#11350,#11351,#11352));
#3135=EDGE_LOOP('',(#11353,#11354,#11355,#11356));
#3136=EDGE_LOOP('',(#11357,#11358,#11359,#11360,#11361,#11362,#11363,#11364,
#11365,#11366,#11367,#11368,#11369,#11370,#11371,#11372,#11373,#11374,#11375,
#11376,#11377,#11378,#11379,#11380,#11381,#11382,#11383,#11384,#11385,#11386,
#11387,#11388,#11389,#11390,#11391,#11392,#11393,#11394,#11395,#11396,#11397,
#11398,#11399,#11400,#11401,#11402,#11403,#11404,#11405,#11406,#11407,#11408,
#11409,#11410,#11411,#11412,#11413,#11414,#11415,#11416,#11417,#11418,#11419,
#11420,#11421,#11422,#11423,#11424,#11425,#11426,#11427,#11428,#11429,#11430,
#11431,#11432,#11433,#11434,#11435,#11436,#11437,#11438,#11439,#11440,#11441,
#11442,#11443,#11444,#11445,#11446,#11447,#11448,#11449,#11450,#11451,#11452,
#11453,#11454,#11455,#11456,#11457,#11458,#11459,#11460,#11461,#11462,#11463,
#11464,#11465,#11466,#11467,#11468,#11469,#11470,#11471,#11472,#11473,#11474,
#11475,#11476,#11477,#11478,#11479,#11480,#11481,#11482,#11483,#11484,#11485,
#11486,#11487,#11488,#11489,#11490,#11491,#11492,#11493,#11494,#11495,#11496,
#11497,#11498,#11499,#11500,#11501,#11502,#11503,#11504));
#3137=EDGE_LOOP('',(#11505,#11506,#11507,#11508));
#3138=EDGE_LOOP('',(#11509,#11510,#11511,#11512));
#3139=EDGE_LOOP('',(#11513,#11514,#11515));
#3140=EDGE_LOOP('',(#11516,#11517,#11518));
#3141=EDGE_LOOP('',(#11519,#11520,#11521,#11522));
#3142=EDGE_LOOP('',(#11523,#11524,#11525,#11526));
#3143=EDGE_LOOP('',(#11527,#11528,#11529,#11530));
#3144=EDGE_LOOP('',(#11531,#11532,#11533,#11534));
#3145=EDGE_LOOP('',(#11535,#11536,#11537));
#3146=EDGE_LOOP('',(#11538,#11539,#11540));
#3147=EDGE_LOOP('',(#11541,#11542,#11543,#11544));
#3148=EDGE_LOOP('',(#11545,#11546,#11547,#11548));
#3149=EDGE_LOOP('',(#11549,#11550,#11551,#11552));
#3150=EDGE_LOOP('',(#11553,#11554,#11555,#11556));
#3151=EDGE_LOOP('',(#11557,#11558,#11559));
#3152=EDGE_LOOP('',(#11560,#11561,#11562));
#3153=EDGE_LOOP('',(#11563,#11564,#11565,#11566));
#3154=EDGE_LOOP('',(#11567,#11568,#11569,#11570));
#3155=EDGE_LOOP('',(#11571,#11572,#11573,#11574));
#3156=EDGE_LOOP('',(#11575,#11576,#11577,#11578));
#3157=EDGE_LOOP('',(#11579,#11580,#11581));
#3158=EDGE_LOOP('',(#11582,#11583,#11584));
#3159=EDGE_LOOP('',(#11585,#11586,#11587,#11588));
#3160=EDGE_LOOP('',(#11589,#11590,#11591,#11592));
#3161=EDGE_LOOP('',(#11593,#11594,#11595,#11596));
#3162=EDGE_LOOP('',(#11597,#11598,#11599,#11600));
#3163=EDGE_LOOP('',(#11601,#11602,#11603));
#3164=EDGE_LOOP('',(#11604,#11605,#11606));
#3165=EDGE_LOOP('',(#11607,#11608,#11609,#11610));
#3166=EDGE_LOOP('',(#11611,#11612,#11613,#11614));
#3167=EDGE_LOOP('',(#11615,#11616,#11617,#11618));
#3168=EDGE_LOOP('',(#11619,#11620,#11621,#11622));
#3169=EDGE_LOOP('',(#11623,#11624,#11625));
#3170=EDGE_LOOP('',(#11626,#11627,#11628));
#3171=EDGE_LOOP('',(#11629,#11630,#11631,#11632));
#3172=EDGE_LOOP('',(#11633,#11634,#11635,#11636));
#3173=EDGE_LOOP('',(#11637,#11638,#11639,#11640));
#3174=EDGE_LOOP('',(#11641,#11642,#11643,#11644));
#3175=EDGE_LOOP('',(#11645,#11646,#11647));
#3176=EDGE_LOOP('',(#11648,#11649,#11650));
#3177=EDGE_LOOP('',(#11651,#11652,#11653,#11654));
#3178=EDGE_LOOP('',(#11655,#11656,#11657,#11658));
#3179=EDGE_LOOP('',(#11659,#11660,#11661,#11662));
#3180=EDGE_LOOP('',(#11663,#11664,#11665,#11666));
#3181=EDGE_LOOP('',(#11667,#11668,#11669));
#3182=EDGE_LOOP('',(#11670,#11671,#11672,#11673));
#3183=EDGE_LOOP('',(#11674,#11675,#11676,#11677));
#3184=EDGE_LOOP('',(#11678,#11679,#11680,#11681));
#3185=EDGE_LOOP('',(#11682,#11683,#11684,#11685));
#3186=EDGE_LOOP('',(#11686,#11687,#11688,#11689));
#3187=EDGE_LOOP('',(#11690,#11691,#11692));
#3188=EDGE_LOOP('',(#11693,#11694,#11695));
#3189=EDGE_LOOP('',(#11696,#11697,#11698,#11699));
#3190=EDGE_LOOP('',(#11700,#11701,#11702,#11703));
#3191=EDGE_LOOP('',(#11704,#11705,#11706,#11707));
#3192=EDGE_LOOP('',(#11708,#11709,#11710,#11711));
#3193=EDGE_LOOP('',(#11712,#11713,#11714));
#3194=EDGE_LOOP('',(#11715,#11716,#11717));
#3195=EDGE_LOOP('',(#11718,#11719,#11720,#11721));
#3196=EDGE_LOOP('',(#11722,#11723,#11724,#11725));
#3197=EDGE_LOOP('',(#11726,#11727,#11728,#11729));
#3198=EDGE_LOOP('',(#11730,#11731,#11732,#11733));
#3199=EDGE_LOOP('',(#11734,#11735,#11736));
#3200=EDGE_LOOP('',(#11737,#11738,#11739));
#3201=EDGE_LOOP('',(#11740,#11741,#11742,#11743));
#3202=EDGE_LOOP('',(#11744,#11745,#11746,#11747));
#3203=EDGE_LOOP('',(#11748,#11749,#11750,#11751));
#3204=EDGE_LOOP('',(#11752,#11753,#11754,#11755));
#3205=EDGE_LOOP('',(#11756,#11757,#11758));
#3206=EDGE_LOOP('',(#11759,#11760,#11761));
#3207=EDGE_LOOP('',(#11762,#11763,#11764,#11765));
#3208=EDGE_LOOP('',(#11766,#11767,#11768,#11769));
#3209=EDGE_LOOP('',(#11770,#11771,#11772,#11773));
#3210=EDGE_LOOP('',(#11774,#11775,#11776,#11777));
#3211=EDGE_LOOP('',(#11778,#11779,#11780));
#3212=EDGE_LOOP('',(#11781,#11782,#11783));
#3213=EDGE_LOOP('',(#11784,#11785,#11786,#11787));
#3214=EDGE_LOOP('',(#11788,#11789,#11790,#11791));
#3215=EDGE_LOOP('',(#11792,#11793,#11794,#11795));
#3216=EDGE_LOOP('',(#11796,#11797,#11798,#11799));
#3217=EDGE_LOOP('',(#11800,#11801,#11802));
#3218=EDGE_LOOP('',(#11803,#11804,#11805));
#3219=EDGE_LOOP('',(#11806,#11807,#11808,#11809));
#3220=EDGE_LOOP('',(#11810,#11811,#11812,#11813));
#3221=EDGE_LOOP('',(#11814,#11815,#11816,#11817));
#3222=EDGE_LOOP('',(#11818,#11819,#11820,#11821));
#3223=EDGE_LOOP('',(#11822,#11823,#11824));
#3224=EDGE_LOOP('',(#11825,#11826,#11827));
#3225=EDGE_LOOP('',(#11828,#11829,#11830,#11831));
#3226=EDGE_LOOP('',(#11832,#11833,#11834,#11835));
#3227=EDGE_LOOP('',(#11836,#11837,#11838,#11839));
#3228=EDGE_LOOP('',(#11840,#11841,#11842,#11843));
#3229=EDGE_LOOP('',(#11844,#11845,#11846));
#3230=EDGE_LOOP('',(#11847,#11848,#11849));
#3231=EDGE_LOOP('',(#11850,#11851,#11852,#11853));
#3232=EDGE_LOOP('',(#11854,#11855,#11856,#11857));
#3233=EDGE_LOOP('',(#11858,#11859,#11860,#11861));
#3234=EDGE_LOOP('',(#11862,#11863,#11864,#11865));
#3235=EDGE_LOOP('',(#11866,#11867,#11868));
#3236=EDGE_LOOP('',(#11869,#11870,#11871));
#3237=EDGE_LOOP('',(#11872,#11873,#11874,#11875));
#3238=EDGE_LOOP('',(#11876,#11877,#11878,#11879));
#3239=EDGE_LOOP('',(#11880));
#3240=EDGE_LOOP('',(#11881,#11882,#11883,#11884,#11885,#11886));
#3241=EDGE_LOOP('',(#11887,#11888));
#3242=EDGE_LOOP('',(#11889,#11890));
#3243=EDGE_LOOP('',(#11891,#11892));
#3244=EDGE_LOOP('',(#11893,#11894));
#3245=EDGE_LOOP('',(#11895,#11896));
#3246=EDGE_LOOP('',(#11897,#11898));
#3247=EDGE_LOOP('',(#11899,#11900,#11901,#11902,#11903,#11904,#11905,#11906));
#3248=EDGE_LOOP('',(#11907,#11908,#11909,#11910));
#3249=EDGE_LOOP('',(#11911,#11912,#11913,#11914));
#3250=EDGE_LOOP('',(#11915,#11916,#11917,#11918));
#3251=EDGE_LOOP('',(#11919,#11920,#11921,#11922));
#3252=EDGE_LOOP('',(#11923,#11924,#11925,#11926));
#3253=EDGE_LOOP('',(#11927,#11928,#11929,#11930));
#3654=CIRCLE('',#14360,1.92913);
#3655=CIRCLE('',#14388,2.36347);
#3656=CIRCLE('',#14389,2.36347);
#3657=CIRCLE('',#14390,2.36347);
#3658=CIRCLE('',#14392,1.92913);
#3659=CIRCLE('',#14394,2.36347);
#3660=CIRCLE('',#14396,2.36347);
#3661=CIRCLE('',#14397,2.36347);
#3662=CIRCLE('',#14399,2.56347);
#3663=CIRCLE('',#14400,0.2);
#3664=CIRCLE('',#14402,3.9624);
#3665=CIRCLE('',#14404,1.96347);
#3666=CIRCLE('',#14409,3.9624);
#3667=CIRCLE('',#14411,3.9624);
#3668=CIRCLE('',#14412,3.9624);
#3669=CIRCLE('',#14413,3.9624);
#3670=CIRCLE('',#14414,3.9624);
#3671=CIRCLE('',#14415,3.9624);
#3672=CIRCLE('',#14416,3.9624);
#3673=CIRCLE('',#14417,3.9624);
#3674=CIRCLE('',#14418,3.9624);
#3675=CIRCLE('',#14419,3.9624);
#3676=CIRCLE('',#14420,3.9624);
#3677=CIRCLE('',#14421,3.9624);
#3678=CIRCLE('',#14422,3.9624);
#3679=CIRCLE('',#14423,3.9624);
#3680=CIRCLE('',#14424,3.9624);
#3681=CIRCLE('',#14425,3.9624);
#3682=CIRCLE('',#14426,3.9624);
#3683=CIRCLE('',#14427,3.9624);
#3684=CIRCLE('',#14428,3.9624);
#3685=CIRCLE('',#14429,3.9624);
#3686=CIRCLE('',#14430,3.9624);
#3687=CIRCLE('',#14431,3.9624);
#3688=CIRCLE('',#14432,3.9624);
#3689=CIRCLE('',#14433,3.9624);
#3690=CIRCLE('',#14434,3.9624);
#3691=CIRCLE('',#14435,3.9624);
#3692=CIRCLE('',#14436,3.9624);
#3693=CIRCLE('',#14437,3.9624);
#3694=CIRCLE('',#14438,3.9624);
#3695=CIRCLE('',#14439,3.9624);
#3696=CIRCLE('',#14440,3.9624);
#3697=CIRCLE('',#14441,3.9624);
#3698=CIRCLE('',#14442,3.9624);
#3699=CIRCLE('',#14443,3.9624);
#3700=CIRCLE('',#14444,3.9624);
#3701=CIRCLE('',#14445,3.9624);
#3702=CIRCLE('',#14446,3.9624);
#3703=CIRCLE('',#14447,3.5624);
#3704=CIRCLE('',#14449,3.9624);
#3705=CIRCLE('',#14453,3.9624);
#3706=CIRCLE('',#14454,3.9624);
#3707=CIRCLE('',#14455,3.9624);
#3708=CIRCLE('',#14456,3.9624);
#3709=CIRCLE('',#14457,3.9624);
#3710=CIRCLE('',#14458,3.9624);
#3711=CIRCLE('',#14459,3.9624);
#3712=CIRCLE('',#14460,3.9624);
#3713=CIRCLE('',#14461,3.9624);
#3714=CIRCLE('',#14462,3.9624);
#3715=CIRCLE('',#14463,3.9624);
#3716=CIRCLE('',#14464,3.9624);
#3717=CIRCLE('',#14465,3.9624);
#3718=CIRCLE('',#14466,3.9624);
#3719=CIRCLE('',#14467,3.9624);
#3720=CIRCLE('',#14468,3.9624);
#3721=CIRCLE('',#14469,3.9624);
#3722=CIRCLE('',#14470,3.9624);
#3723=CIRCLE('',#14471,3.9624);
#3724=CIRCLE('',#14472,3.9624);
#3725=CIRCLE('',#14473,3.9624);
#3726=CIRCLE('',#14474,3.9624);
#3727=CIRCLE('',#14475,3.9624);
#3728=CIRCLE('',#14476,3.9624);
#3729=CIRCLE('',#14477,3.9624);
#3730=CIRCLE('',#14478,3.9624);
#3731=CIRCLE('',#14479,3.9624);
#3732=CIRCLE('',#14480,3.9624);
#3733=CIRCLE('',#14481,3.9624);
#3734=CIRCLE('',#14482,3.9624);
#3735=CIRCLE('',#14483,3.9624);
#3736=CIRCLE('',#14484,3.9624);
#3737=CIRCLE('',#14485,3.9624);
#3738=CIRCLE('',#14486,3.9624);
#3739=CIRCLE('',#14487,3.9624);
#3740=CIRCLE('',#14592,2.29135888084633);
#3741=CIRCLE('',#14594,2.29135888084633);
#3742=CIRCLE('',#14596,2.29135888084633);
#3743=CIRCLE('',#14598,2.29135888084633);
#3744=CIRCLE('',#14600,2.29135888084633);
#3745=CIRCLE('',#14602,2.29135888084633);
#4304=LINE('',#37378,#5215);
#4305=LINE('',#37600,#5216);
#4306=LINE('',#38015,#5217);
#4307=LINE('',#38451,#5218);
#4308=LINE('',#38912,#5219);
#4309=LINE('',#39451,#5220);
#4310=LINE('',#39914,#5221);
#4311=LINE('',#40417,#5222);
#4312=LINE('',#40894,#5223);
#4313=LINE('',#41353,#5224);
#4314=LINE('',#41796,#5225);
#4315=LINE('',#42255,#5226);
#4316=LINE('',#42724,#5227);
#4317=LINE('',#43181,#5228);
#4318=LINE('',#43630,#5229);
#4319=LINE('',#44093,#5230);
#4320=LINE('',#44530,#5231);
#4321=LINE('',#45011,#5232);
#4322=LINE('',#45502,#5233);
#4323=LINE('',#45947,#5234);
#4324=LINE('',#46416,#5235);
#4325=LINE('',#46842,#5236);
#4326=LINE('',#47342,#5237);
#4327=LINE('',#47794,#5238);
#4328=LINE('',#48245,#5239);
#4329=LINE('',#48697,#5240);
#4330=LINE('',#49204,#5241);
#4331=LINE('',#58902,#5242);
#4332=LINE('',#58908,#5243);
#4333=LINE('',#58910,#5244);
#4334=LINE('',#58912,#5245);
#4335=LINE('',#58922,#5246);
#4336=LINE('',#58923,#5247);
#4337=LINE('',#59279,#5248);
#4338=LINE('',#59286,#5249);
#4339=LINE('',#59287,#5250);
#4340=LINE('',#59289,#5251);
#4341=LINE('',#59290,#5252);
#4342=LINE('',#59292,#5253);
#4343=LINE('',#59297,#5254);
#4344=LINE('',#59300,#5255);
#4345=LINE('',#59302,#5256);
#4346=LINE('',#59305,#5257);
#4347=LINE('',#59307,#5258);
#4348=LINE('',#59310,#5259);
#4349=LINE('',#59312,#5260);
#4350=LINE('',#59315,#5261);
#4351=LINE('',#59317,#5262);
#4352=LINE('',#59320,#5263);
#4353=LINE('',#59322,#5264);
#4354=LINE('',#59325,#5265);
#4355=LINE('',#59327,#5266);
#4356=LINE('',#59330,#5267);
#4357=LINE('',#59332,#5268);
#4358=LINE('',#59335,#5269);
#4359=LINE('',#59337,#5270);
#4360=LINE('',#59340,#5271);
#4361=LINE('',#59342,#5272);
#4362=LINE('',#59345,#5273);
#4363=LINE('',#59347,#5274);
#4364=LINE('',#59350,#5275);
#4365=LINE('',#59352,#5276);
#4366=LINE('',#59355,#5277);
#4367=LINE('',#59357,#5278);
#4368=LINE('',#59360,#5279);
#4369=LINE('',#59362,#5280);
#4370=LINE('',#59365,#5281);
#4371=LINE('',#59367,#5282);
#4372=LINE('',#59370,#5283);
#4373=LINE('',#59372,#5284);
#4374=LINE('',#59375,#5285);
#4375=LINE('',#59377,#5286);
#4376=LINE('',#59380,#5287);
#4377=LINE('',#59382,#5288);
#4378=LINE('',#59385,#5289);
#4379=LINE('',#59387,#5290);
#4380=LINE('',#59390,#5291);
#4381=LINE('',#59392,#5292);
#4382=LINE('',#59395,#5293);
#4383=LINE('',#59397,#5294);
#4384=LINE('',#59400,#5295);
#4385=LINE('',#59402,#5296);
#4386=LINE('',#59405,#5297);
#4387=LINE('',#59407,#5298);
#4388=LINE('',#59410,#5299);
#4389=LINE('',#59412,#5300);
#4390=LINE('',#59415,#5301);
#4391=LINE('',#59417,#5302);
#4392=LINE('',#59420,#5303);
#4393=LINE('',#59422,#5304);
#4394=LINE('',#59425,#5305);
#4395=LINE('',#59427,#5306);
#4396=LINE('',#59430,#5307);
#4397=LINE('',#59432,#5308);
#4398=LINE('',#59435,#5309);
#4399=LINE('',#59437,#5310);
#4400=LINE('',#59440,#5311);
#4401=LINE('',#59442,#5312);
#4402=LINE('',#59445,#5313);
#4403=LINE('',#59447,#5314);
#4404=LINE('',#59450,#5315);
#4405=LINE('',#59452,#5316);
#4406=LINE('',#59455,#5317);
#4407=LINE('',#59457,#5318);
#4408=LINE('',#59460,#5319);
#4409=LINE('',#59462,#5320);
#4410=LINE('',#59465,#5321);
#4411=LINE('',#59466,#5322);
#4412=LINE('',#59469,#5323);
#4413=LINE('',#59470,#5324);
#4414=LINE('',#59472,#5325);
#4415=LINE('',#59476,#5326);
#4416=LINE('',#59477,#5327);
#4417=LINE('',#59479,#5328);
#4418=LINE('',#59483,#5329);
#4419=LINE('',#59484,#5330);
#4420=LINE('',#59486,#5331);
#4421=LINE('',#59490,#5332);
#4422=LINE('',#59491,#5333);
#4423=LINE('',#59493,#5334);
#4424=LINE('',#59497,#5335);
#4425=LINE('',#59498,#5336);
#4426=LINE('',#59500,#5337);
#4427=LINE('',#59504,#5338);
#4428=LINE('',#59505,#5339);
#4429=LINE('',#59507,#5340);
#4430=LINE('',#59511,#5341);
#4431=LINE('',#59512,#5342);
#4432=LINE('',#59514,#5343);
#4433=LINE('',#59518,#5344);
#4434=LINE('',#59519,#5345);
#4435=LINE('',#59521,#5346);
#4436=LINE('',#59525,#5347);
#4437=LINE('',#59526,#5348);
#4438=LINE('',#59528,#5349);
#4439=LINE('',#59532,#5350);
#4440=LINE('',#59533,#5351);
#4441=LINE('',#59535,#5352);
#4442=LINE('',#59539,#5353);
#4443=LINE('',#59540,#5354);
#4444=LINE('',#59542,#5355);
#4445=LINE('',#59546,#5356);
#4446=LINE('',#59547,#5357);
#4447=LINE('',#59549,#5358);
#4448=LINE('',#59553,#5359);
#4449=LINE('',#59554,#5360);
#4450=LINE('',#59556,#5361);
#4451=LINE('',#59560,#5362);
#4452=LINE('',#59561,#5363);
#4453=LINE('',#59563,#5364);
#4454=LINE('',#59567,#5365);
#4455=LINE('',#59568,#5366);
#4456=LINE('',#59570,#5367);
#4457=LINE('',#59574,#5368);
#4458=LINE('',#59575,#5369);
#4459=LINE('',#59577,#5370);
#4460=LINE('',#59581,#5371);
#4461=LINE('',#59582,#5372);
#4462=LINE('',#59584,#5373);
#4463=LINE('',#59588,#5374);
#4464=LINE('',#59589,#5375);
#4465=LINE('',#59591,#5376);
#4466=LINE('',#59595,#5377);
#4467=LINE('',#59596,#5378);
#4468=LINE('',#59598,#5379);
#4469=LINE('',#59602,#5380);
#4470=LINE('',#59603,#5381);
#4471=LINE('',#59605,#5382);
#4472=LINE('',#59609,#5383);
#4473=LINE('',#59610,#5384);
#4474=LINE('',#59612,#5385);
#4475=LINE('',#59616,#5386);
#4476=LINE('',#59617,#5387);
#4477=LINE('',#59619,#5388);
#4478=LINE('',#59623,#5389);
#4479=LINE('',#59624,#5390);
#4480=LINE('',#59626,#5391);
#4481=LINE('',#59630,#5392);
#4482=LINE('',#59631,#5393);
#4483=LINE('',#59633,#5394);
#4484=LINE('',#59637,#5395);
#4485=LINE('',#59638,#5396);
#4486=LINE('',#59640,#5397);
#4487=LINE('',#59644,#5398);
#4488=LINE('',#59645,#5399);
#4489=LINE('',#59647,#5400);
#4490=LINE('',#59651,#5401);
#4491=LINE('',#59652,#5402);
#4492=LINE('',#59654,#5403);
#4493=LINE('',#59658,#5404);
#4494=LINE('',#59659,#5405);
#4495=LINE('',#59661,#5406);
#4496=LINE('',#59665,#5407);
#4497=LINE('',#59666,#5408);
#4498=LINE('',#59668,#5409);
#4499=LINE('',#59672,#5410);
#4500=LINE('',#59673,#5411);
#4501=LINE('',#59675,#5412);
#4502=LINE('',#59679,#5413);
#4503=LINE('',#59680,#5414);
#4504=LINE('',#59682,#5415);
#4505=LINE('',#59686,#5416);
#4506=LINE('',#59687,#5417);
#4507=LINE('',#59689,#5418);
#4508=LINE('',#59693,#5419);
#4509=LINE('',#59694,#5420);
#4510=LINE('',#59696,#5421);
#4511=LINE('',#59700,#5422);
#4512=LINE('',#59701,#5423);
#4513=LINE('',#59703,#5424);
#4514=LINE('',#59708,#5425);
#4515=LINE('',#59710,#5426);
#4516=LINE('',#59712,#5427);
#4517=LINE('',#59714,#5428);
#4518=LINE('',#59716,#5429);
#4519=LINE('',#59717,#5430);
#4520=LINE('',#59721,#5431);
#4521=LINE('',#59725,#5432);
#4522=LINE('',#59729,#5433);
#4523=LINE('',#59733,#5434);
#4524=LINE('',#59737,#5435);
#4525=LINE('',#59740,#5436);
#4526=LINE('',#59744,#5437);
#4527=LINE('',#59746,#5438);
#4528=LINE('',#59747,#5439);
#4529=LINE('',#59749,#5440);
#4530=LINE('',#59751,#5441);
#4531=LINE('',#59753,#5442);
#4532=LINE('',#59755,#5443);
#5215=VECTOR('',#16717,1.92913);
#5216=VECTOR('',#16722,1.92913);
#5217=VECTOR('',#16725,1.92913);
#5218=VECTOR('',#16728,1.92913);
#5219=VECTOR('',#16731,1.92913);
#5220=VECTOR('',#16734,1.92913);
#5221=VECTOR('',#16737,1.92913);
#5222=VECTOR('',#16740,1.92913);
#5223=VECTOR('',#16743,1.92913);
#5224=VECTOR('',#16746,1.92913);
#5225=VECTOR('',#16749,1.92913);
#5226=VECTOR('',#16752,1.92913);
#5227=VECTOR('',#16755,1.92913);
#5228=VECTOR('',#16758,1.92913);
#5229=VECTOR('',#16761,1.92913);
#5230=VECTOR('',#16764,1.92913);
#5231=VECTOR('',#16767,1.92913);
#5232=VECTOR('',#16770,1.92913);
#5233=VECTOR('',#16773,1.92913);
#5234=VECTOR('',#16776,1.92913);
#5235=VECTOR('',#16779,1.92913);
#5236=VECTOR('',#16782,1.92913);
#5237=VECTOR('',#16785,1.92913);
#5238=VECTOR('',#16788,1.92913);
#5239=VECTOR('',#16791,1.92913);
#5240=VECTOR('',#16794,1.92913);
#5241=VECTOR('',#16797,1.92913);
#5242=VECTOR('',#16832,2.16347);
#5243=VECTOR('',#16839,10.);
#5244=VECTOR('',#16840,10.);
#5245=VECTOR('',#16841,10.);
#5246=VECTOR('',#16844,10.);
#5247=VECTOR('',#16845,10.);
#5248=VECTOR('',#16924,3.7624);
#5249=VECTOR('',#16931,10.);
#5250=VECTOR('',#16932,10.);
#5251=VECTOR('',#16935,10.);
#5252=VECTOR('',#16936,10.);
#5253=VECTOR('',#16939,10.);
#5254=VECTOR('',#16944,3.9624);
#5255=VECTOR('',#16947,10.);
#5256=VECTOR('',#16948,10.);
#5257=VECTOR('',#16951,10.);
#5258=VECTOR('',#16952,10.);
#5259=VECTOR('',#16955,10.);
#5260=VECTOR('',#16956,10.);
#5261=VECTOR('',#16959,10.);
#5262=VECTOR('',#16960,10.);
#5263=VECTOR('',#16963,10.);
#5264=VECTOR('',#16964,10.);
#5265=VECTOR('',#16967,10.);
#5266=VECTOR('',#16968,10.);
#5267=VECTOR('',#16971,10.);
#5268=VECTOR('',#16972,10.);
#5269=VECTOR('',#16975,10.);
#5270=VECTOR('',#16976,10.);
#5271=VECTOR('',#16979,10.);
#5272=VECTOR('',#16980,10.);
#5273=VECTOR('',#16983,10.);
#5274=VECTOR('',#16984,10.);
#5275=VECTOR('',#16987,10.);
#5276=VECTOR('',#16988,10.);
#5277=VECTOR('',#16991,10.);
#5278=VECTOR('',#16992,10.);
#5279=VECTOR('',#16995,10.);
#5280=VECTOR('',#16996,10.);
#5281=VECTOR('',#16999,10.);
#5282=VECTOR('',#17000,10.);
#5283=VECTOR('',#17003,10.);
#5284=VECTOR('',#17004,10.);
#5285=VECTOR('',#17007,10.);
#5286=VECTOR('',#17008,10.);
#5287=VECTOR('',#17011,10.);
#5288=VECTOR('',#17012,10.);
#5289=VECTOR('',#17015,10.);
#5290=VECTOR('',#17016,10.);
#5291=VECTOR('',#17019,10.);
#5292=VECTOR('',#17020,10.);
#5293=VECTOR('',#17023,10.);
#5294=VECTOR('',#17024,10.);
#5295=VECTOR('',#17027,10.);
#5296=VECTOR('',#17028,10.);
#5297=VECTOR('',#17031,10.);
#5298=VECTOR('',#17032,10.);
#5299=VECTOR('',#17035,10.);
#5300=VECTOR('',#17036,10.);
#5301=VECTOR('',#17039,10.);
#5302=VECTOR('',#17040,10.);
#5303=VECTOR('',#17043,10.);
#5304=VECTOR('',#17044,10.);
#5305=VECTOR('',#17047,10.);
#5306=VECTOR('',#17048,10.);
#5307=VECTOR('',#17051,10.);
#5308=VECTOR('',#17052,10.);
#5309=VECTOR('',#17055,10.);
#5310=VECTOR('',#17056,10.);
#5311=VECTOR('',#17059,10.);
#5312=VECTOR('',#17060,10.);
#5313=VECTOR('',#17063,10.);
#5314=VECTOR('',#17064,10.);
#5315=VECTOR('',#17067,10.);
#5316=VECTOR('',#17068,10.);
#5317=VECTOR('',#17071,10.);
#5318=VECTOR('',#17072,10.);
#5319=VECTOR('',#17075,10.);
#5320=VECTOR('',#17076,10.);
#5321=VECTOR('',#17079,10.);
#5322=VECTOR('',#17080,10.);
#5323=VECTOR('',#17083,10.);
#5324=VECTOR('',#17084,10.);
#5325=VECTOR('',#17087,10.);
#5326=VECTOR('',#17092,10.);
#5327=VECTOR('',#17093,10.);
#5328=VECTOR('',#17096,10.);
#5329=VECTOR('',#17101,10.);
#5330=VECTOR('',#17102,10.);
#5331=VECTOR('',#17105,10.);
#5332=VECTOR('',#17110,10.);
#5333=VECTOR('',#17111,10.);
#5334=VECTOR('',#17114,10.);
#5335=VECTOR('',#17119,10.);
#5336=VECTOR('',#17120,10.);
#5337=VECTOR('',#17123,10.);
#5338=VECTOR('',#17128,10.);
#5339=VECTOR('',#17129,10.);
#5340=VECTOR('',#17132,10.);
#5341=VECTOR('',#17137,10.);
#5342=VECTOR('',#17138,10.);
#5343=VECTOR('',#17141,10.);
#5344=VECTOR('',#17146,10.);
#5345=VECTOR('',#17147,10.);
#5346=VECTOR('',#17150,10.);
#5347=VECTOR('',#17155,10.);
#5348=VECTOR('',#17156,10.);
#5349=VECTOR('',#17159,10.);
#5350=VECTOR('',#17164,10.);
#5351=VECTOR('',#17165,10.);
#5352=VECTOR('',#17168,10.);
#5353=VECTOR('',#17173,10.);
#5354=VECTOR('',#17174,10.);
#5355=VECTOR('',#17177,10.);
#5356=VECTOR('',#17182,10.);
#5357=VECTOR('',#17183,10.);
#5358=VECTOR('',#17186,10.);
#5359=VECTOR('',#17191,10.);
#5360=VECTOR('',#17192,10.);
#5361=VECTOR('',#17195,10.);
#5362=VECTOR('',#17200,10.);
#5363=VECTOR('',#17201,10.);
#5364=VECTOR('',#17204,10.);
#5365=VECTOR('',#17209,10.);
#5366=VECTOR('',#17210,10.);
#5367=VECTOR('',#17213,10.);
#5368=VECTOR('',#17218,10.);
#5369=VECTOR('',#17219,10.);
#5370=VECTOR('',#17222,10.);
#5371=VECTOR('',#17227,10.);
#5372=VECTOR('',#17228,10.);
#5373=VECTOR('',#17231,10.);
#5374=VECTOR('',#17236,10.);
#5375=VECTOR('',#17237,10.);
#5376=VECTOR('',#17240,10.);
#5377=VECTOR('',#17245,10.);
#5378=VECTOR('',#17246,10.);
#5379=VECTOR('',#17249,10.);
#5380=VECTOR('',#17254,10.);
#5381=VECTOR('',#17255,10.);
#5382=VECTOR('',#17258,10.);
#5383=VECTOR('',#17263,10.);
#5384=VECTOR('',#17264,10.);
#5385=VECTOR('',#17267,10.);
#5386=VECTOR('',#17272,10.);
#5387=VECTOR('',#17273,10.);
#5388=VECTOR('',#17276,10.);
#5389=VECTOR('',#17281,10.);
#5390=VECTOR('',#17282,10.);
#5391=VECTOR('',#17285,10.);
#5392=VECTOR('',#17290,10.);
#5393=VECTOR('',#17291,10.);
#5394=VECTOR('',#17294,10.);
#5395=VECTOR('',#17299,10.);
#5396=VECTOR('',#17300,10.);
#5397=VECTOR('',#17303,10.);
#5398=VECTOR('',#17308,10.);
#5399=VECTOR('',#17309,10.);
#5400=VECTOR('',#17312,10.);
#5401=VECTOR('',#17317,10.);
#5402=VECTOR('',#17318,10.);
#5403=VECTOR('',#17321,10.);
#5404=VECTOR('',#17326,10.);
#5405=VECTOR('',#17327,10.);
#5406=VECTOR('',#17330,10.);
#5407=VECTOR('',#17335,10.);
#5408=VECTOR('',#17336,10.);
#5409=VECTOR('',#17339,10.);
#5410=VECTOR('',#17344,10.);
#5411=VECTOR('',#17345,10.);
#5412=VECTOR('',#17348,10.);
#5413=VECTOR('',#17353,10.);
#5414=VECTOR('',#17354,10.);
#5415=VECTOR('',#17357,10.);
#5416=VECTOR('',#17362,10.);
#5417=VECTOR('',#17363,10.);
#5418=VECTOR('',#17366,10.);
#5419=VECTOR('',#17371,10.);
#5420=VECTOR('',#17372,10.);
#5421=VECTOR('',#17375,10.);
#5422=VECTOR('',#17380,10.);
#5423=VECTOR('',#17381,10.);
#5424=VECTOR('',#17384,10.);
#5425=VECTOR('',#17389,10.);
#5426=VECTOR('',#17390,10.);
#5427=VECTOR('',#17391,10.);
#5428=VECTOR('',#17392,10.);
#5429=VECTOR('',#17393,10.);
#5430=VECTOR('',#17394,9.99999999999999);
#5431=VECTOR('',#17397,10.);
#5432=VECTOR('',#17402,10.);
#5433=VECTOR('',#17407,10.);
#5434=VECTOR('',#17412,10.);
#5435=VECTOR('',#17417,10.);
#5436=VECTOR('',#17422,9.99999999999999);
#5437=VECTOR('',#17427,1.14567944042316);
#5438=VECTOR('',#17430,10.);
#5439=VECTOR('',#17431,10.);
#5440=VECTOR('',#17434,10.);
#5441=VECTOR('',#17437,10.);
#5442=VECTOR('',#17440,10.);
#5443=VECTOR('',#17443,10.);
#6311=VERTEX_POINT('',#37376);
#6312=VERTEX_POINT('',#37377);
#6313=VERTEX_POINT('',#37379);
#6314=VERTEX_POINT('',#37510);
#6315=VERTEX_POINT('',#37598);
#6316=VERTEX_POINT('',#37599);
#6317=VERTEX_POINT('',#37601);
#6318=VERTEX_POINT('',#37793);
#6319=VERTEX_POINT('',#38013);
#6320=VERTEX_POINT('',#38014);
#6321=VERTEX_POINT('',#38016);
#6322=VERTEX_POINT('',#38449);
#6323=VERTEX_POINT('',#38450);
#6324=VERTEX_POINT('',#38680);
#6325=VERTEX_POINT('',#38910);
#6326=VERTEX_POINT('',#38911);
#6327=VERTEX_POINT('',#38913);
#6328=VERTEX_POINT('',#39449);
#6329=VERTEX_POINT('',#39450);
#6330=VERTEX_POINT('',#39686);
#6331=VERTEX_POINT('',#39912);
#6332=VERTEX_POINT('',#39913);
#6333=VERTEX_POINT('',#39915);
#6334=VERTEX_POINT('',#40415);
#6335=VERTEX_POINT('',#40416);
#6336=VERTEX_POINT('',#40634);
#6337=VERTEX_POINT('',#40892);
#6338=VERTEX_POINT('',#40893);
#6339=VERTEX_POINT('',#40895);
#6340=VERTEX_POINT('',#41351);
#6341=VERTEX_POINT('',#41352);
#6342=VERTEX_POINT('',#41562);
#6343=VERTEX_POINT('',#41794);
#6344=VERTEX_POINT('',#41795);
#6345=VERTEX_POINT('',#41797);
#6346=VERTEX_POINT('',#42253);
#6347=VERTEX_POINT('',#42254);
#6348=VERTEX_POINT('',#42484);
#6349=VERTEX_POINT('',#42722);
#6350=VERTEX_POINT('',#42723);
#6351=VERTEX_POINT('',#42725);
#6352=VERTEX_POINT('',#43179);
#6353=VERTEX_POINT('',#43180);
#6354=VERTEX_POINT('',#43408);
#6355=VERTEX_POINT('',#43628);
#6356=VERTEX_POINT('',#43629);
#6357=VERTEX_POINT('',#43631);
#6358=VERTEX_POINT('',#44091);
#6359=VERTEX_POINT('',#44092);
#6360=VERTEX_POINT('',#44306);
#6361=VERTEX_POINT('',#44528);
#6362=VERTEX_POINT('',#44529);
#6363=VERTEX_POINT('',#44531);
#6364=VERTEX_POINT('',#45009);
#6365=VERTEX_POINT('',#45010);
#6366=VERTEX_POINT('',#45228);
#6367=VERTEX_POINT('',#45500);
#6368=VERTEX_POINT('',#45501);
#6369=VERTEX_POINT('',#45503);
#6370=VERTEX_POINT('',#45945);
#6371=VERTEX_POINT('',#45946);
#6372=VERTEX_POINT('',#46178);
#6373=VERTEX_POINT('',#46414);
#6374=VERTEX_POINT('',#46415);
#6375=VERTEX_POINT('',#46417);
#6376=VERTEX_POINT('',#46840);
#6377=VERTEX_POINT('',#46841);
#6378=VERTEX_POINT('',#46843);
#6379=VERTEX_POINT('',#47066);
#6380=VERTEX_POINT('',#47340);
#6381=VERTEX_POINT('',#47341);
#6382=VERTEX_POINT('',#47792);
#6383=VERTEX_POINT('',#47793);
#6384=VERTEX_POINT('',#47795);
#6385=VERTEX_POINT('',#48024);
#6386=VERTEX_POINT('',#48243);
#6387=VERTEX_POINT('',#48244);
#6388=VERTEX_POINT('',#48476);
#6389=VERTEX_POINT('',#48695);
#6390=VERTEX_POINT('',#48696);
#6391=VERTEX_POINT('',#48698);
#6392=VERTEX_POINT('',#49202);
#6393=VERTEX_POINT('',#49203);
#6394=VERTEX_POINT('',#49431);
#6395=VERTEX_POINT('',#49636);
#6396=VERTEX_POINT('',#49637);
#6397=VERTEX_POINT('',#49705);
#6398=VERTEX_POINT('',#49707);
#6399=VERTEX_POINT('',#49713);
#6400=VERTEX_POINT('',#49904);
#6401=VERTEX_POINT('',#50098);
#6402=VERTEX_POINT('',#50292);
#6403=VERTEX_POINT('',#50483);
#6404=VERTEX_POINT('',#50494);
#6405=VERTEX_POINT('',#50505);
#6406=VERTEX_POINT('',#50517);
#6407=VERTEX_POINT('',#50528);
#6408=VERTEX_POINT('',#50539);
#6409=VERTEX_POINT('',#50551);
#6410=VERTEX_POINT('',#50562);
#6411=VERTEX_POINT('',#50573);
#6412=VERTEX_POINT('',#50764);
#6413=VERTEX_POINT('',#50958);
#6414=VERTEX_POINT('',#51149);
#6415=VERTEX_POINT('',#51340);
#6416=VERTEX_POINT('',#51531);
#6417=VERTEX_POINT('',#51725);
#6418=VERTEX_POINT('',#51916);
#6419=VERTEX_POINT('',#52110);
#6420=VERTEX_POINT('',#52304);
#6421=VERTEX_POINT('',#52495);
#6422=VERTEX_POINT('',#52689);
#6423=VERTEX_POINT('',#52880);
#6424=VERTEX_POINT('',#53074);
#6425=VERTEX_POINT('',#53265);
#6426=VERTEX_POINT('',#53276);
#6427=VERTEX_POINT('',#53293);
#6428=VERTEX_POINT('',#53295);
#6429=VERTEX_POINT('',#53297);
#6430=VERTEX_POINT('',#53473);
#6431=VERTEX_POINT('',#53664);
#6432=VERTEX_POINT('',#53855);
#6433=VERTEX_POINT('',#54049);
#6434=VERTEX_POINT('',#54240);
#6435=VERTEX_POINT('',#54434);
#6436=VERTEX_POINT('',#54628);
#6437=VERTEX_POINT('',#54819);
#6438=VERTEX_POINT('',#55013);
#6439=VERTEX_POINT('',#55204);
#6440=VERTEX_POINT('',#55215);
#6441=VERTEX_POINT('',#55227);
#6442=VERTEX_POINT('',#55238);
#6443=VERTEX_POINT('',#55249);
#6444=VERTEX_POINT('',#55261);
#6445=VERTEX_POINT('',#55272);
#6446=VERTEX_POINT('',#55283);
#6447=VERTEX_POINT('',#55295);
#6448=VERTEX_POINT('',#55306);
#6449=VERTEX_POINT('',#55500);
#6450=VERTEX_POINT('',#55691);
#6451=VERTEX_POINT('',#55885);
#6452=VERTEX_POINT('',#56076);
#6453=VERTEX_POINT('',#56270);
#6454=VERTEX_POINT('',#56461);
#6455=VERTEX_POINT('',#56849);
#6456=VERTEX_POINT('',#56890);
#6457=VERTEX_POINT('',#57009);
#6458=VERTEX_POINT('',#57011);
#6459=VERTEX_POINT('',#57140);
#6460=VERTEX_POINT('',#58095);
#6461=VERTEX_POINT('',#58096);
#6462=VERTEX_POINT('',#58894);
#6463=VERTEX_POINT('',#58898);
#6464=VERTEX_POINT('',#58901);
#6465=VERTEX_POINT('',#58906);
#6466=VERTEX_POINT('',#58907);
#6467=VERTEX_POINT('',#58909);
#6468=VERTEX_POINT('',#58911);
#6469=VERTEX_POINT('',#58917);
#6470=VERTEX_POINT('',#58921);
#6471=VERTEX_POINT('',#58927);
#6472=VERTEX_POINT('',#58928);
#6473=VERTEX_POINT('',#58932);
#6474=VERTEX_POINT('',#58934);
#6475=VERTEX_POINT('',#58938);
#6476=VERTEX_POINT('',#58942);
#6477=VERTEX_POINT('',#58944);
#6478=VERTEX_POINT('',#58948);
#6479=VERTEX_POINT('',#58952);
#6480=VERTEX_POINT('',#58954);
#6481=VERTEX_POINT('',#58958);
#6482=VERTEX_POINT('',#58962);
#6483=VERTEX_POINT('',#58964);
#6484=VERTEX_POINT('',#58968);
#6485=VERTEX_POINT('',#58972);
#6486=VERTEX_POINT('',#58974);
#6487=VERTEX_POINT('',#58978);
#6488=VERTEX_POINT('',#58982);
#6489=VERTEX_POINT('',#58984);
#6490=VERTEX_POINT('',#58988);
#6491=VERTEX_POINT('',#58992);
#6492=VERTEX_POINT('',#58994);
#6493=VERTEX_POINT('',#58998);
#6494=VERTEX_POINT('',#59002);
#6495=VERTEX_POINT('',#59004);
#6496=VERTEX_POINT('',#59008);
#6497=VERTEX_POINT('',#59012);
#6498=VERTEX_POINT('',#59014);
#6499=VERTEX_POINT('',#59018);
#6500=VERTEX_POINT('',#59022);
#6501=VERTEX_POINT('',#59024);
#6502=VERTEX_POINT('',#59028);
#6503=VERTEX_POINT('',#59032);
#6504=VERTEX_POINT('',#59034);
#6505=VERTEX_POINT('',#59038);
#6506=VERTEX_POINT('',#59042);
#6507=VERTEX_POINT('',#59044);
#6508=VERTEX_POINT('',#59048);
#6509=VERTEX_POINT('',#59052);
#6510=VERTEX_POINT('',#59054);
#6511=VERTEX_POINT('',#59058);
#6512=VERTEX_POINT('',#59062);
#6513=VERTEX_POINT('',#59064);
#6514=VERTEX_POINT('',#59068);
#6515=VERTEX_POINT('',#59072);
#6516=VERTEX_POINT('',#59074);
#6517=VERTEX_POINT('',#59078);
#6518=VERTEX_POINT('',#59082);
#6519=VERTEX_POINT('',#59084);
#6520=VERTEX_POINT('',#59088);
#6521=VERTEX_POINT('',#59092);
#6522=VERTEX_POINT('',#59094);
#6523=VERTEX_POINT('',#59098);
#6524=VERTEX_POINT('',#59102);
#6525=VERTEX_POINT('',#59104);
#6526=VERTEX_POINT('',#59108);
#6527=VERTEX_POINT('',#59113);
#6528=VERTEX_POINT('',#59115);
#6529=VERTEX_POINT('',#59119);
#6530=VERTEX_POINT('',#59123);
#6531=VERTEX_POINT('',#59125);
#6532=VERTEX_POINT('',#59129);
#6533=VERTEX_POINT('',#59133);
#6534=VERTEX_POINT('',#59135);
#6535=VERTEX_POINT('',#59139);
#6536=VERTEX_POINT('',#59143);
#6537=VERTEX_POINT('',#59145);
#6538=VERTEX_POINT('',#59149);
#6539=VERTEX_POINT('',#59153);
#6540=VERTEX_POINT('',#59155);
#6541=VERTEX_POINT('',#59159);
#6542=VERTEX_POINT('',#59163);
#6543=VERTEX_POINT('',#59165);
#6544=VERTEX_POINT('',#59169);
#6545=VERTEX_POINT('',#59173);
#6546=VERTEX_POINT('',#59175);
#6547=VERTEX_POINT('',#59179);
#6548=VERTEX_POINT('',#59183);
#6549=VERTEX_POINT('',#59185);
#6550=VERTEX_POINT('',#59189);
#6551=VERTEX_POINT('',#59193);
#6552=VERTEX_POINT('',#59195);
#6553=VERTEX_POINT('',#59199);
#6554=VERTEX_POINT('',#59203);
#6555=VERTEX_POINT('',#59205);
#6556=VERTEX_POINT('',#59209);
#6557=VERTEX_POINT('',#59213);
#6558=VERTEX_POINT('',#59215);
#6559=VERTEX_POINT('',#59219);
#6560=VERTEX_POINT('',#59223);
#6561=VERTEX_POINT('',#59225);
#6562=VERTEX_POINT('',#59229);
#6563=VERTEX_POINT('',#59233);
#6564=VERTEX_POINT('',#59235);
#6565=VERTEX_POINT('',#59239);
#6566=VERTEX_POINT('',#59243);
#6567=VERTEX_POINT('',#59245);
#6568=VERTEX_POINT('',#59249);
#6569=VERTEX_POINT('',#59253);
#6570=VERTEX_POINT('',#59255);
#6571=VERTEX_POINT('',#59259);
#6572=VERTEX_POINT('',#59263);
#6573=VERTEX_POINT('',#59265);
#6574=VERTEX_POINT('',#59269);
#6575=VERTEX_POINT('',#59273);
#6576=VERTEX_POINT('',#59278);
#6577=VERTEX_POINT('',#59282);
#6578=VERTEX_POINT('',#59283);
#6579=VERTEX_POINT('',#59285);
#6580=VERTEX_POINT('',#59294);
#6581=VERTEX_POINT('',#59295);
#6582=VERTEX_POINT('',#59298);
#6583=VERTEX_POINT('',#59301);
#6584=VERTEX_POINT('',#59303);
#6585=VERTEX_POINT('',#59306);
#6586=VERTEX_POINT('',#59308);
#6587=VERTEX_POINT('',#59311);
#6588=VERTEX_POINT('',#59313);
#6589=VERTEX_POINT('',#59316);
#6590=VERTEX_POINT('',#59318);
#6591=VERTEX_POINT('',#59321);
#6592=VERTEX_POINT('',#59323);
#6593=VERTEX_POINT('',#59326);
#6594=VERTEX_POINT('',#59328);
#6595=VERTEX_POINT('',#59331);
#6596=VERTEX_POINT('',#59333);
#6597=VERTEX_POINT('',#59336);
#6598=VERTEX_POINT('',#59338);
#6599=VERTEX_POINT('',#59341);
#6600=VERTEX_POINT('',#59343);
#6601=VERTEX_POINT('',#59346);
#6602=VERTEX_POINT('',#59348);
#6603=VERTEX_POINT('',#59351);
#6604=VERTEX_POINT('',#59353);
#6605=VERTEX_POINT('',#59356);
#6606=VERTEX_POINT('',#59358);
#6607=VERTEX_POINT('',#59361);
#6608=VERTEX_POINT('',#59363);
#6609=VERTEX_POINT('',#59366);
#6610=VERTEX_POINT('',#59368);
#6611=VERTEX_POINT('',#59371);
#6612=VERTEX_POINT('',#59373);
#6613=VERTEX_POINT('',#59376);
#6614=VERTEX_POINT('',#59378);
#6615=VERTEX_POINT('',#59381);
#6616=VERTEX_POINT('',#59383);
#6617=VERTEX_POINT('',#59386);
#6618=VERTEX_POINT('',#59388);
#6619=VERTEX_POINT('',#59391);
#6620=VERTEX_POINT('',#59393);
#6621=VERTEX_POINT('',#59396);
#6622=VERTEX_POINT('',#59398);
#6623=VERTEX_POINT('',#59401);
#6624=VERTEX_POINT('',#59403);
#6625=VERTEX_POINT('',#59406);
#6626=VERTEX_POINT('',#59408);
#6627=VERTEX_POINT('',#59411);
#6628=VERTEX_POINT('',#59413);
#6629=VERTEX_POINT('',#59416);
#6630=VERTEX_POINT('',#59418);
#6631=VERTEX_POINT('',#59421);
#6632=VERTEX_POINT('',#59423);
#6633=VERTEX_POINT('',#59426);
#6634=VERTEX_POINT('',#59428);
#6635=VERTEX_POINT('',#59431);
#6636=VERTEX_POINT('',#59433);
#6637=VERTEX_POINT('',#59436);
#6638=VERTEX_POINT('',#59438);
#6639=VERTEX_POINT('',#59441);
#6640=VERTEX_POINT('',#59443);
#6641=VERTEX_POINT('',#59446);
#6642=VERTEX_POINT('',#59448);
#6643=VERTEX_POINT('',#59451);
#6644=VERTEX_POINT('',#59453);
#6645=VERTEX_POINT('',#59456);
#6646=VERTEX_POINT('',#59458);
#6647=VERTEX_POINT('',#59461);
#6648=VERTEX_POINT('',#59463);
#6649=VERTEX_POINT('',#59468);
#6650=VERTEX_POINT('',#59475);
#6651=VERTEX_POINT('',#59482);
#6652=VERTEX_POINT('',#59489);
#6653=VERTEX_POINT('',#59496);
#6654=VERTEX_POINT('',#59503);
#6655=VERTEX_POINT('',#59510);
#6656=VERTEX_POINT('',#59517);
#6657=VERTEX_POINT('',#59524);
#6658=VERTEX_POINT('',#59531);
#6659=VERTEX_POINT('',#59538);
#6660=VERTEX_POINT('',#59545);
#6661=VERTEX_POINT('',#59552);
#6662=VERTEX_POINT('',#59559);
#6663=VERTEX_POINT('',#59566);
#6664=VERTEX_POINT('',#59573);
#6665=VERTEX_POINT('',#59580);
#6666=VERTEX_POINT('',#59587);
#6667=VERTEX_POINT('',#59594);
#6668=VERTEX_POINT('',#59601);
#6669=VERTEX_POINT('',#59608);
#6670=VERTEX_POINT('',#59615);
#6671=VERTEX_POINT('',#59622);
#6672=VERTEX_POINT('',#59629);
#6673=VERTEX_POINT('',#59636);
#6674=VERTEX_POINT('',#59643);
#6675=VERTEX_POINT('',#59650);
#6676=VERTEX_POINT('',#59657);
#6677=VERTEX_POINT('',#59664);
#6678=VERTEX_POINT('',#59671);
#6679=VERTEX_POINT('',#59678);
#6680=VERTEX_POINT('',#59685);
#6681=VERTEX_POINT('',#59692);
#6682=VERTEX_POINT('',#59699);
#6683=VERTEX_POINT('',#59706);
#6684=VERTEX_POINT('',#59707);
#6685=VERTEX_POINT('',#59709);
#6686=VERTEX_POINT('',#59711);
#6687=VERTEX_POINT('',#59713);
#6688=VERTEX_POINT('',#59715);
#6689=VERTEX_POINT('',#59719);
#6690=VERTEX_POINT('',#59720);
#6691=VERTEX_POINT('',#59724);
#6692=VERTEX_POINT('',#59728);
#6693=VERTEX_POINT('',#59732);
#6694=VERTEX_POINT('',#59736);
#6695=VERTEX_POINT('',#59743);
#7958=EDGE_CURVE('',#6311,#6312,#4304,.T.);
#7959=EDGE_CURVE('',#6313,#6311,#1250,.T.);
#7960=EDGE_CURVE('',#6314,#6313,#3654,.T.);
#7961=EDGE_CURVE('',#6314,#6312,#1251,.T.);
#7962=EDGE_CURVE('',#6315,#6316,#4305,.T.);
#7963=EDGE_CURVE('',#6317,#6315,#1252,.T.);
#7964=EDGE_CURVE('',#6311,#6317,#1253,.T.);
#7965=EDGE_CURVE('',#6312,#6318,#1254,.T.);
#7966=EDGE_CURVE('',#6318,#6316,#1255,.T.);
#7967=EDGE_CURVE('',#6319,#6320,#4306,.T.);
#7968=EDGE_CURVE('',#6321,#6319,#1256,.F.);
#7969=EDGE_CURVE('',#6315,#6321,#1257,.T.);
#7970=EDGE_CURVE('',#6316,#6320,#1258,.T.);
#7971=EDGE_CURVE('',#6322,#6323,#4307,.T.);
#7972=EDGE_CURVE('',#6319,#6322,#1259,.F.);
#7973=EDGE_CURVE('',#6320,#6324,#1260,.T.);
#7974=EDGE_CURVE('',#6324,#6323,#1261,.T.);
#7975=EDGE_CURVE('',#6325,#6326,#4308,.T.);
#7976=EDGE_CURVE('',#6327,#6325,#1262,.F.);
#7977=EDGE_CURVE('',#6322,#6327,#1263,.F.);
#7978=EDGE_CURVE('',#6323,#6326,#1264,.T.);
#7979=EDGE_CURVE('',#6328,#6329,#4309,.T.);
#7980=EDGE_CURVE('',#6325,#6328,#1265,.F.);
#7981=EDGE_CURVE('',#6326,#6330,#1266,.T.);
#7982=EDGE_CURVE('',#6330,#6329,#1267,.T.);
#7983=EDGE_CURVE('',#6331,#6332,#4310,.T.);
#7984=EDGE_CURVE('',#6333,#6331,#1268,.F.);
#7985=EDGE_CURVE('',#6328,#6333,#1269,.F.);
#7986=EDGE_CURVE('',#6329,#6332,#1270,.T.);
#7987=EDGE_CURVE('',#6334,#6335,#4311,.T.);
#7988=EDGE_CURVE('',#6331,#6334,#1271,.F.);
#7989=EDGE_CURVE('',#6332,#6336,#1272,.T.);
#7990=EDGE_CURVE('',#6336,#6335,#1273,.T.);
#7991=EDGE_CURVE('',#6337,#6338,#4312,.T.);
#7992=EDGE_CURVE('',#6339,#6337,#1274,.F.);
#7993=EDGE_CURVE('',#6334,#6339,#1275,.F.);
#7994=EDGE_CURVE('',#6335,#6338,#1276,.T.);
#7995=EDGE_CURVE('',#6340,#6341,#4313,.T.);
#7996=EDGE_CURVE('',#6337,#6340,#1277,.F.);
#7997=EDGE_CURVE('',#6338,#6342,#1278,.T.);
#7998=EDGE_CURVE('',#6342,#6341,#1279,.T.);
#7999=EDGE_CURVE('',#6343,#6344,#4314,.T.);
#8000=EDGE_CURVE('',#6345,#6343,#1280,.F.);
#8001=EDGE_CURVE('',#6340,#6345,#1281,.F.);
#8002=EDGE_CURVE('',#6341,#6344,#1282,.T.);
#8003=EDGE_CURVE('',#6346,#6347,#4315,.T.);
#8004=EDGE_CURVE('',#6343,#6346,#1283,.F.);
#8005=EDGE_CURVE('',#6344,#6348,#1284,.T.);
#8006=EDGE_CURVE('',#6348,#6347,#1285,.T.);
#8007=EDGE_CURVE('',#6349,#6350,#4316,.T.);
#8008=EDGE_CURVE('',#6351,#6349,#1286,.F.);
#8009=EDGE_CURVE('',#6346,#6351,#1287,.F.);
#8010=EDGE_CURVE('',#6347,#6350,#1288,.T.);
#8011=EDGE_CURVE('',#6352,#6353,#4317,.T.);
#8012=EDGE_CURVE('',#6349,#6352,#1289,.F.);
#8013=EDGE_CURVE('',#6350,#6354,#1290,.T.);
#8014=EDGE_CURVE('',#6354,#6353,#1291,.T.);
#8015=EDGE_CURVE('',#6355,#6356,#4318,.T.);
#8016=EDGE_CURVE('',#6357,#6355,#1292,.F.);
#8017=EDGE_CURVE('',#6352,#6357,#1293,.F.);
#8018=EDGE_CURVE('',#6353,#6356,#1294,.T.);
#8019=EDGE_CURVE('',#6358,#6359,#4319,.T.);
#8020=EDGE_CURVE('',#6355,#6358,#1295,.F.);
#8021=EDGE_CURVE('',#6356,#6360,#1296,.T.);
#8022=EDGE_CURVE('',#6360,#6359,#1297,.T.);
#8023=EDGE_CURVE('',#6361,#6362,#4320,.T.);
#8024=EDGE_CURVE('',#6363,#6361,#1298,.F.);
#8025=EDGE_CURVE('',#6358,#6363,#1299,.F.);
#8026=EDGE_CURVE('',#6359,#6362,#1300,.T.);
#8027=EDGE_CURVE('',#6364,#6365,#4321,.T.);
#8028=EDGE_CURVE('',#6361,#6364,#1301,.F.);
#8029=EDGE_CURVE('',#6362,#6366,#1302,.T.);
#8030=EDGE_CURVE('',#6366,#6365,#1303,.T.);
#8031=EDGE_CURVE('',#6367,#6368,#4322,.T.);
#8032=EDGE_CURVE('',#6369,#6367,#1304,.F.);
#8033=EDGE_CURVE('',#6364,#6369,#1305,.F.);
#8034=EDGE_CURVE('',#6365,#6368,#1306,.T.);
#8035=EDGE_CURVE('',#6370,#6371,#4323,.T.);
#8036=EDGE_CURVE('',#6367,#6370,#1307,.F.);
#8037=EDGE_CURVE('',#6368,#6372,#1308,.T.);
#8038=EDGE_CURVE('',#6372,#6371,#1309,.T.);
#8039=EDGE_CURVE('',#6373,#6374,#4324,.T.);
#8040=EDGE_CURVE('',#6375,#6373,#1310,.T.);
#8041=EDGE_CURVE('',#6370,#6375,#1311,.F.);
#8042=EDGE_CURVE('',#6371,#6374,#1312,.T.);
#8043=EDGE_CURVE('',#6376,#6377,#4325,.T.);
#8044=EDGE_CURVE('',#6378,#6376,#1313,.F.);
#8045=EDGE_CURVE('',#6373,#6378,#1314,.T.);
#8046=EDGE_CURVE('',#6374,#6379,#1315,.T.);
#8047=EDGE_CURVE('',#6379,#6377,#1316,.T.);
#8048=EDGE_CURVE('',#6380,#6381,#4326,.T.);
#8049=EDGE_CURVE('',#6376,#6380,#1317,.F.);
#8050=EDGE_CURVE('',#6377,#6381,#1318,.T.);
#8051=EDGE_CURVE('',#6382,#6383,#4327,.T.);
#8052=EDGE_CURVE('',#6384,#6382,#1319,.F.);
#8053=EDGE_CURVE('',#6380,#6384,#1320,.F.);
#8054=EDGE_CURVE('',#6381,#6385,#1321,.T.);
#8055=EDGE_CURVE('',#6385,#6383,#1322,.T.);
#8056=EDGE_CURVE('',#6386,#6387,#4328,.T.);
#8057=EDGE_CURVE('',#6382,#6386,#1323,.F.);
#8058=EDGE_CURVE('',#6383,#6388,#1324,.T.);
#8059=EDGE_CURVE('',#6388,#6387,#1325,.T.);
#8060=EDGE_CURVE('',#6389,#6390,#4329,.T.);
#8061=EDGE_CURVE('',#6391,#6389,#1326,.F.);
#8062=EDGE_CURVE('',#6386,#6391,#1327,.F.);
#8063=EDGE_CURVE('',#6387,#6390,#1328,.T.);
#8064=EDGE_CURVE('',#6392,#6393,#4330,.T.);
#8065=EDGE_CURVE('',#6389,#6392,#1329,.F.);
#8066=EDGE_CURVE('',#6390,#6394,#1330,.T.);
#8067=EDGE_CURVE('',#6394,#6393,#1331,.T.);
#8068=EDGE_CURVE('',#6395,#6396,#1332,.T.);
#8069=EDGE_CURVE('',#6397,#6396,#3655,.T.);
#8070=EDGE_CURVE('',#6397,#6398,#1333,.T.);
#8071=EDGE_CURVE('',#6398,#6399,#1334,.T.);
#8072=EDGE_CURVE('',#6399,#6400,#1335,.T.);
#8073=EDGE_CURVE('',#6400,#6401,#1336,.T.);
#8074=EDGE_CURVE('',#6401,#6402,#1337,.T.);
#8075=EDGE_CURVE('',#6402,#6403,#1338,.T.);
#8076=EDGE_CURVE('',#6403,#6404,#1339,.T.);
#8077=EDGE_CURVE('',#6404,#6405,#1340,.T.);
#8078=EDGE_CURVE('',#6405,#6406,#1341,.T.);
#8079=EDGE_CURVE('',#6406,#6407,#1342,.T.);
#8080=EDGE_CURVE('',#6407,#6408,#1343,.T.);
#8081=EDGE_CURVE('',#6408,#6409,#1344,.T.);
#8082=EDGE_CURVE('',#6409,#6410,#1345,.T.);
#8083=EDGE_CURVE('',#6410,#6411,#1346,.T.);
#8084=EDGE_CURVE('',#6411,#6412,#1347,.T.);
#8085=EDGE_CURVE('',#6412,#6413,#1348,.T.);
#8086=EDGE_CURVE('',#6413,#6414,#1349,.T.);
#8087=EDGE_CURVE('',#6414,#6415,#1350,.T.);
#8088=EDGE_CURVE('',#6415,#6416,#1351,.T.);
#8089=EDGE_CURVE('',#6416,#6417,#1352,.T.);
#8090=EDGE_CURVE('',#6417,#6418,#1353,.T.);
#8091=EDGE_CURVE('',#6418,#6419,#1354,.T.);
#8092=EDGE_CURVE('',#6419,#6420,#1355,.T.);
#8093=EDGE_CURVE('',#6420,#6421,#1356,.T.);
#8094=EDGE_CURVE('',#6421,#6422,#1357,.T.);
#8095=EDGE_CURVE('',#6422,#6423,#1358,.T.);
#8096=EDGE_CURVE('',#6423,#6424,#1359,.T.);
#8097=EDGE_CURVE('',#6424,#6425,#1360,.T.);
#8098=EDGE_CURVE('',#6425,#6426,#1361,.T.);
#8099=EDGE_CURVE('',#6427,#6426,#3656,.T.);
#8100=EDGE_CURVE('',#6428,#6427,#3657,.T.);
#8101=EDGE_CURVE('',#6428,#6429,#1362,.T.);
#8102=EDGE_CURVE('',#6429,#6430,#1363,.T.);
#8103=EDGE_CURVE('',#6430,#6431,#1364,.T.);
#8104=EDGE_CURVE('',#6431,#6432,#1365,.T.);
#8105=EDGE_CURVE('',#6432,#6433,#1366,.T.);
#8106=EDGE_CURVE('',#6433,#6434,#1367,.T.);
#8107=EDGE_CURVE('',#6434,#6435,#1368,.T.);
#8108=EDGE_CURVE('',#6435,#6436,#1369,.T.);
#8109=EDGE_CURVE('',#6436,#6437,#1370,.T.);
#8110=EDGE_CURVE('',#6437,#6438,#1371,.T.);
#8111=EDGE_CURVE('',#6438,#6439,#1372,.T.);
#8112=EDGE_CURVE('',#6439,#6440,#1373,.T.);
#8113=EDGE_CURVE('',#6440,#6441,#1374,.T.);
#8114=EDGE_CURVE('',#6441,#6442,#1375,.T.);
#8115=EDGE_CURVE('',#6442,#6443,#1376,.T.);
#8116=EDGE_CURVE('',#6443,#6444,#1377,.T.);
#8117=EDGE_CURVE('',#6444,#6445,#1378,.T.);
#8118=EDGE_CURVE('',#6445,#6446,#1379,.T.);
#8119=EDGE_CURVE('',#6446,#6447,#1380,.T.);
#8120=EDGE_CURVE('',#6447,#6448,#1381,.T.);
#8121=EDGE_CURVE('',#6448,#6449,#1382,.T.);
#8122=EDGE_CURVE('',#6449,#6450,#1383,.T.);
#8123=EDGE_CURVE('',#6450,#6451,#1384,.T.);
#8124=EDGE_CURVE('',#6451,#6452,#1385,.T.);
#8125=EDGE_CURVE('',#6452,#6453,#1386,.T.);
#8126=EDGE_CURVE('',#6453,#6454,#1387,.T.);
#8127=EDGE_CURVE('',#6454,#6395,#1388,.T.);
#8128=EDGE_CURVE('',#6393,#6455,#1389,.T.);
#8129=EDGE_CURVE('',#6455,#6456,#1390,.T.);
#8130=EDGE_CURVE('',#6457,#6456,#3658,.T.);
#8131=EDGE_CURVE('',#6458,#6457,#1391,.T.);
#8132=EDGE_CURVE('',#6392,#6458,#1392,.F.);
#8133=EDGE_CURVE('',#6459,#6428,#3659,.T.);
#8134=EDGE_CURVE('',#6459,#6457,#1393,.T.);
#8135=EDGE_CURVE('',#6456,#6428,#1394,.T.);
#8136=EDGE_CURVE('',#6426,#6459,#1395,.T.);
#8137=EDGE_CURVE('',#6313,#6397,#1396,.T.);
#8138=EDGE_CURVE('',#6460,#6461,#3660,.T.);
#8139=EDGE_CURVE('',#6460,#6314,#1397,.T.);
#8140=EDGE_CURVE('',#6461,#6397,#3661,.T.);
#8141=EDGE_CURVE('',#6396,#6460,#1398,.T.);
#8142=EDGE_CURVE('',#6462,#6462,#3662,.T.);
#8143=EDGE_CURVE('',#6462,#6461,#3663,.T.);
#8144=EDGE_CURVE('',#6463,#6463,#3664,.T.);
#8145=EDGE_CURVE('',#6427,#6464,#4331,.T.);
#8146=EDGE_CURVE('',#6464,#6464,#3665,.T.);
#8147=EDGE_CURVE('',#6465,#6466,#4332,.T.);
#8148=EDGE_CURVE('',#6465,#6467,#4333,.T.);
#8149=EDGE_CURVE('',#6468,#6467,#4334,.T.);
#8150=EDGE_CURVE('',#6466,#6468,#859,.T.);
#8151=EDGE_CURVE('',#6468,#6469,#860,.T.);
#8152=EDGE_CURVE('',#6467,#6470,#4335,.T.);
#8153=EDGE_CURVE('',#6469,#6470,#4336,.T.);
#8154=EDGE_CURVE('',#6470,#6465,#3666,.T.);
#8155=EDGE_CURVE('',#6471,#6472,#861,.T.);
#8156=EDGE_CURVE('',#6472,#6473,#3667,.T.);
#8157=EDGE_CURVE('',#6473,#6474,#862,.T.);
#8158=EDGE_CURVE('',#6474,#6475,#863,.T.);
#8159=EDGE_CURVE('',#6475,#6476,#3668,.T.);
#8160=EDGE_CURVE('',#6476,#6477,#864,.T.);
#8161=EDGE_CURVE('',#6477,#6478,#865,.T.);
#8162=EDGE_CURVE('',#6478,#6479,#3669,.T.);
#8163=EDGE_CURVE('',#6479,#6480,#866,.T.);
#8164=EDGE_CURVE('',#6480,#6481,#867,.T.);
#8165=EDGE_CURVE('',#6481,#6482,#3670,.T.);
#8166=EDGE_CURVE('',#6482,#6483,#868,.T.);
#8167=EDGE_CURVE('',#6483,#6484,#869,.T.);
#8168=EDGE_CURVE('',#6484,#6485,#3671,.T.);
#8169=EDGE_CURVE('',#6485,#6486,#870,.T.);
#8170=EDGE_CURVE('',#6486,#6487,#871,.T.);
#8171=EDGE_CURVE('',#6487,#6488,#3672,.T.);
#8172=EDGE_CURVE('',#6488,#6489,#872,.T.);
#8173=EDGE_CURVE('',#6489,#6490,#873,.T.);
#8174=EDGE_CURVE('',#6490,#6491,#3673,.T.);
#8175=EDGE_CURVE('',#6491,#6492,#874,.T.);
#8176=EDGE_CURVE('',#6492,#6493,#875,.T.);
#8177=EDGE_CURVE('',#6493,#6494,#3674,.T.);
#8178=EDGE_CURVE('',#6494,#6495,#876,.T.);
#8179=EDGE_CURVE('',#6495,#6496,#877,.T.);
#8180=EDGE_CURVE('',#6496,#6497,#3675,.T.);
#8181=EDGE_CURVE('',#6497,#6498,#878,.T.);
#8182=EDGE_CURVE('',#6498,#6499,#879,.T.);
#8183=EDGE_CURVE('',#6499,#6500,#3676,.T.);
#8184=EDGE_CURVE('',#6500,#6501,#880,.T.);
#8185=EDGE_CURVE('',#6501,#6502,#881,.T.);
#8186=EDGE_CURVE('',#6502,#6503,#3677,.T.);
#8187=EDGE_CURVE('',#6503,#6504,#882,.T.);
#8188=EDGE_CURVE('',#6504,#6505,#883,.T.);
#8189=EDGE_CURVE('',#6505,#6506,#3678,.T.);
#8190=EDGE_CURVE('',#6506,#6507,#884,.T.);
#8191=EDGE_CURVE('',#6507,#6508,#885,.T.);
#8192=EDGE_CURVE('',#6508,#6509,#3679,.T.);
#8193=EDGE_CURVE('',#6509,#6510,#886,.T.);
#8194=EDGE_CURVE('',#6510,#6511,#887,.T.);
#8195=EDGE_CURVE('',#6511,#6512,#3680,.T.);
#8196=EDGE_CURVE('',#6512,#6513,#888,.T.);
#8197=EDGE_CURVE('',#6513,#6514,#889,.T.);
#8198=EDGE_CURVE('',#6514,#6515,#3681,.T.);
#8199=EDGE_CURVE('',#6515,#6516,#890,.T.);
#8200=EDGE_CURVE('',#6516,#6517,#891,.T.);
#8201=EDGE_CURVE('',#6517,#6518,#3682,.T.);
#8202=EDGE_CURVE('',#6518,#6519,#892,.T.);
#8203=EDGE_CURVE('',#6519,#6520,#893,.T.);
#8204=EDGE_CURVE('',#6520,#6521,#3683,.T.);
#8205=EDGE_CURVE('',#6521,#6522,#894,.T.);
#8206=EDGE_CURVE('',#6522,#6523,#895,.T.);
#8207=EDGE_CURVE('',#6523,#6524,#3684,.T.);
#8208=EDGE_CURVE('',#6524,#6525,#896,.T.);
#8209=EDGE_CURVE('',#6525,#6526,#897,.T.);
#8210=EDGE_CURVE('',#6526,#6466,#3685,.T.);
#8211=EDGE_CURVE('',#6469,#6527,#3686,.T.);
#8212=EDGE_CURVE('',#6527,#6528,#898,.T.);
#8213=EDGE_CURVE('',#6528,#6529,#899,.T.);
#8214=EDGE_CURVE('',#6529,#6530,#3687,.T.);
#8215=EDGE_CURVE('',#6530,#6531,#900,.T.);
#8216=EDGE_CURVE('',#6531,#6532,#901,.T.);
#8217=EDGE_CURVE('',#6532,#6533,#3688,.T.);
#8218=EDGE_CURVE('',#6533,#6534,#902,.T.);
#8219=EDGE_CURVE('',#6534,#6535,#903,.T.);
#8220=EDGE_CURVE('',#6535,#6536,#3689,.T.);
#8221=EDGE_CURVE('',#6536,#6537,#904,.T.);
#8222=EDGE_CURVE('',#6537,#6538,#905,.T.);
#8223=EDGE_CURVE('',#6538,#6539,#3690,.T.);
#8224=EDGE_CURVE('',#6539,#6540,#906,.T.);
#8225=EDGE_CURVE('',#6540,#6541,#907,.T.);
#8226=EDGE_CURVE('',#6541,#6542,#3691,.T.);
#8227=EDGE_CURVE('',#6542,#6543,#908,.T.);
#8228=EDGE_CURVE('',#6543,#6544,#909,.T.);
#8229=EDGE_CURVE('',#6544,#6545,#3692,.T.);
#8230=EDGE_CURVE('',#6545,#6546,#910,.T.);
#8231=EDGE_CURVE('',#6546,#6547,#911,.T.);
#8232=EDGE_CURVE('',#6547,#6548,#3693,.T.);
#8233=EDGE_CURVE('',#6548,#6549,#912,.T.);
#8234=EDGE_CURVE('',#6549,#6550,#913,.T.);
#8235=EDGE_CURVE('',#6550,#6551,#3694,.T.);
#8236=EDGE_CURVE('',#6551,#6552,#914,.T.);
#8237=EDGE_CURVE('',#6552,#6553,#915,.T.);
#8238=EDGE_CURVE('',#6553,#6554,#3695,.T.);
#8239=EDGE_CURVE('',#6554,#6555,#916,.T.);
#8240=EDGE_CURVE('',#6555,#6556,#917,.T.);
#8241=EDGE_CURVE('',#6556,#6557,#3696,.T.);
#8242=EDGE_CURVE('',#6557,#6558,#918,.T.);
#8243=EDGE_CURVE('',#6558,#6559,#919,.T.);
#8244=EDGE_CURVE('',#6559,#6560,#3697,.T.);
#8245=EDGE_CURVE('',#6560,#6561,#920,.T.);
#8246=EDGE_CURVE('',#6561,#6562,#921,.T.);
#8247=EDGE_CURVE('',#6562,#6563,#3698,.T.);
#8248=EDGE_CURVE('',#6563,#6564,#922,.T.);
#8249=EDGE_CURVE('',#6564,#6565,#923,.T.);
#8250=EDGE_CURVE('',#6565,#6566,#3699,.T.);
#8251=EDGE_CURVE('',#6566,#6567,#924,.T.);
#8252=EDGE_CURVE('',#6567,#6568,#925,.T.);
#8253=EDGE_CURVE('',#6568,#6569,#3700,.T.);
#8254=EDGE_CURVE('',#6569,#6570,#926,.T.);
#8255=EDGE_CURVE('',#6570,#6571,#927,.T.);
#8256=EDGE_CURVE('',#6571,#6572,#3701,.T.);
#8257=EDGE_CURVE('',#6572,#6573,#928,.T.);
#8258=EDGE_CURVE('',#6573,#6574,#929,.T.);
#8259=EDGE_CURVE('',#6574,#6575,#3702,.T.);
#8260=EDGE_CURVE('',#6575,#6471,#930,.T.);
#8261=EDGE_CURVE('',#6471,#6576,#4337,.T.);
#8262=EDGE_CURVE('',#6576,#6576,#3703,.T.);
#8263=EDGE_CURVE('',#6577,#6578,#3704,.T.);
#8264=EDGE_CURVE('',#6579,#6577,#4338,.T.);
#8265=EDGE_CURVE('',#6578,#6579,#4339,.T.);
#8266=EDGE_CURVE('',#6578,#6527,#4340,.T.);
#8267=EDGE_CURVE('',#6528,#6579,#4341,.T.);
#8268=EDGE_CURVE('',#6529,#6577,#4342,.T.);
#8269=EDGE_CURVE('',#6580,#6581,#3705,.T.);
#8270=EDGE_CURVE('',#6581,#6463,#4343,.T.);
#8271=EDGE_CURVE('',#6581,#6582,#3706,.T.);
#8272=EDGE_CURVE('',#6582,#6575,#4344,.T.);
#8273=EDGE_CURVE('',#6574,#6583,#4345,.T.);
#8274=EDGE_CURVE('',#6583,#6584,#3707,.T.);
#8275=EDGE_CURVE('',#6584,#6572,#4346,.T.);
#8276=EDGE_CURVE('',#6571,#6585,#4347,.T.);
#8277=EDGE_CURVE('',#6585,#6586,#3708,.T.);
#8278=EDGE_CURVE('',#6586,#6569,#4348,.T.);
#8279=EDGE_CURVE('',#6568,#6587,#4349,.T.);
#8280=EDGE_CURVE('',#6587,#6588,#3709,.T.);
#8281=EDGE_CURVE('',#6588,#6566,#4350,.T.);
#8282=EDGE_CURVE('',#6565,#6589,#4351,.T.);
#8283=EDGE_CURVE('',#6589,#6590,#3710,.T.);
#8284=EDGE_CURVE('',#6590,#6563,#4352,.T.);
#8285=EDGE_CURVE('',#6562,#6591,#4353,.T.);
#8286=EDGE_CURVE('',#6591,#6592,#3711,.T.);
#8287=EDGE_CURVE('',#6592,#6560,#4354,.T.);
#8288=EDGE_CURVE('',#6559,#6593,#4355,.T.);
#8289=EDGE_CURVE('',#6593,#6594,#3712,.T.);
#8290=EDGE_CURVE('',#6594,#6557,#4356,.T.);
#8291=EDGE_CURVE('',#6556,#6595,#4357,.T.);
#8292=EDGE_CURVE('',#6595,#6596,#3713,.T.);
#8293=EDGE_CURVE('',#6596,#6554,#4358,.T.);
#8294=EDGE_CURVE('',#6553,#6597,#4359,.T.);
#8295=EDGE_CURVE('',#6597,#6598,#3714,.T.);
#8296=EDGE_CURVE('',#6598,#6551,#4360,.T.);
#8297=EDGE_CURVE('',#6550,#6599,#4361,.T.);
#8298=EDGE_CURVE('',#6599,#6600,#3715,.T.);
#8299=EDGE_CURVE('',#6600,#6548,#4362,.T.);
#8300=EDGE_CURVE('',#6547,#6601,#4363,.T.);
#8301=EDGE_CURVE('',#6601,#6602,#3716,.T.);
#8302=EDGE_CURVE('',#6602,#6545,#4364,.T.);
#8303=EDGE_CURVE('',#6544,#6603,#4365,.T.);
#8304=EDGE_CURVE('',#6603,#6604,#3717,.T.);
#8305=EDGE_CURVE('',#6604,#6542,#4366,.T.);
#8306=EDGE_CURVE('',#6541,#6605,#4367,.T.);
#8307=EDGE_CURVE('',#6605,#6606,#3718,.T.);
#8308=EDGE_CURVE('',#6606,#6539,#4368,.T.);
#8309=EDGE_CURVE('',#6538,#6607,#4369,.T.);
#8310=EDGE_CURVE('',#6607,#6608,#3719,.T.);
#8311=EDGE_CURVE('',#6608,#6536,#4370,.T.);
#8312=EDGE_CURVE('',#6535,#6609,#4371,.T.);
#8313=EDGE_CURVE('',#6609,#6610,#3720,.T.);
#8314=EDGE_CURVE('',#6610,#6533,#4372,.T.);
#8315=EDGE_CURVE('',#6532,#6611,#4373,.T.);
#8316=EDGE_CURVE('',#6611,#6612,#3721,.T.);
#8317=EDGE_CURVE('',#6612,#6530,#4374,.T.);
#8318=EDGE_CURVE('',#6526,#6613,#4375,.T.);
#8319=EDGE_CURVE('',#6613,#6614,#3722,.T.);
#8320=EDGE_CURVE('',#6614,#6524,#4376,.T.);
#8321=EDGE_CURVE('',#6523,#6615,#4377,.T.);
#8322=EDGE_CURVE('',#6615,#6616,#3723,.T.);
#8323=EDGE_CURVE('',#6616,#6521,#4378,.T.);
#8324=EDGE_CURVE('',#6520,#6617,#4379,.T.);
#8325=EDGE_CURVE('',#6617,#6618,#3724,.T.);
#8326=EDGE_CURVE('',#6618,#6518,#4380,.T.);
#8327=EDGE_CURVE('',#6517,#6619,#4381,.T.);
#8328=EDGE_CURVE('',#6619,#6620,#3725,.T.);
#8329=EDGE_CURVE('',#6620,#6515,#4382,.T.);
#8330=EDGE_CURVE('',#6514,#6621,#4383,.T.);
#8331=EDGE_CURVE('',#6621,#6622,#3726,.T.);
#8332=EDGE_CURVE('',#6622,#6512,#4384,.T.);
#8333=EDGE_CURVE('',#6511,#6623,#4385,.T.);
#8334=EDGE_CURVE('',#6623,#6624,#3727,.T.);
#8335=EDGE_CURVE('',#6624,#6509,#4386,.T.);
#8336=EDGE_CURVE('',#6508,#6625,#4387,.T.);
#8337=EDGE_CURVE('',#6625,#6626,#3728,.T.);
#8338=EDGE_CURVE('',#6626,#6506,#4388,.T.);
#8339=EDGE_CURVE('',#6505,#6627,#4389,.T.);
#8340=EDGE_CURVE('',#6627,#6628,#3729,.T.);
#8341=EDGE_CURVE('',#6628,#6503,#4390,.T.);
#8342=EDGE_CURVE('',#6502,#6629,#4391,.T.);
#8343=EDGE_CURVE('',#6629,#6630,#3730,.T.);
#8344=EDGE_CURVE('',#6630,#6500,#4392,.T.);
#8345=EDGE_CURVE('',#6499,#6631,#4393,.T.);
#8346=EDGE_CURVE('',#6631,#6632,#3731,.T.);
#8347=EDGE_CURVE('',#6632,#6497,#4394,.T.);
#8348=EDGE_CURVE('',#6496,#6633,#4395,.T.);
#8349=EDGE_CURVE('',#6633,#6634,#3732,.T.);
#8350=EDGE_CURVE('',#6634,#6494,#4396,.T.);
#8351=EDGE_CURVE('',#6493,#6635,#4397,.T.);
#8352=EDGE_CURVE('',#6635,#6636,#3733,.T.);
#8353=EDGE_CURVE('',#6636,#6491,#4398,.T.);
#8354=EDGE_CURVE('',#6490,#6637,#4399,.T.);
#8355=EDGE_CURVE('',#6637,#6638,#3734,.T.);
#8356=EDGE_CURVE('',#6638,#6488,#4400,.T.);
#8357=EDGE_CURVE('',#6487,#6639,#4401,.T.);
#8358=EDGE_CURVE('',#6639,#6640,#3735,.T.);
#8359=EDGE_CURVE('',#6640,#6485,#4402,.T.);
#8360=EDGE_CURVE('',#6484,#6641,#4403,.T.);
#8361=EDGE_CURVE('',#6641,#6642,#3736,.T.);
#8362=EDGE_CURVE('',#6642,#6482,#4404,.T.);
#8363=EDGE_CURVE('',#6481,#6643,#4405,.T.);
#8364=EDGE_CURVE('',#6643,#6644,#3737,.T.);
#8365=EDGE_CURVE('',#6644,#6479,#4406,.T.);
#8366=EDGE_CURVE('',#6478,#6645,#4407,.T.);
#8367=EDGE_CURVE('',#6645,#6646,#3738,.T.);
#8368=EDGE_CURVE('',#6646,#6476,#4408,.T.);
#8369=EDGE_CURVE('',#6475,#6647,#4409,.T.);
#8370=EDGE_CURVE('',#6647,#6648,#3739,.T.);
#8371=EDGE_CURVE('',#6648,#6473,#4410,.T.);
#8372=EDGE_CURVE('',#6472,#6580,#4411,.T.);
#8373=EDGE_CURVE('',#6612,#6649,#4412,.T.);
#8374=EDGE_CURVE('',#6531,#6649,#4413,.T.);
#8375=EDGE_CURVE('',#6649,#6611,#4414,.T.);
#8376=EDGE_CURVE('',#6650,#6609,#4415,.T.);
#8377=EDGE_CURVE('',#6610,#6650,#4416,.T.);
#8378=EDGE_CURVE('',#6534,#6650,#4417,.T.);
#8379=EDGE_CURVE('',#6608,#6651,#4418,.T.);
#8380=EDGE_CURVE('',#6537,#6651,#4419,.T.);
#8381=EDGE_CURVE('',#6651,#6607,#4420,.T.);
#8382=EDGE_CURVE('',#6652,#6605,#4421,.T.);
#8383=EDGE_CURVE('',#6606,#6652,#4422,.T.);
#8384=EDGE_CURVE('',#6540,#6652,#4423,.T.);
#8385=EDGE_CURVE('',#6604,#6653,#4424,.T.);
#8386=EDGE_CURVE('',#6543,#6653,#4425,.T.);
#8387=EDGE_CURVE('',#6653,#6603,#4426,.T.);
#8388=EDGE_CURVE('',#6654,#6601,#4427,.T.);
#8389=EDGE_CURVE('',#6602,#6654,#4428,.T.);
#8390=EDGE_CURVE('',#6546,#6654,#4429,.T.);
#8391=EDGE_CURVE('',#6600,#6655,#4430,.T.);
#8392=EDGE_CURVE('',#6549,#6655,#4431,.T.);
#8393=EDGE_CURVE('',#6655,#6599,#4432,.T.);
#8394=EDGE_CURVE('',#6656,#6597,#4433,.T.);
#8395=EDGE_CURVE('',#6598,#6656,#4434,.T.);
#8396=EDGE_CURVE('',#6552,#6656,#4435,.T.);
#8397=EDGE_CURVE('',#6596,#6657,#4436,.T.);
#8398=EDGE_CURVE('',#6555,#6657,#4437,.T.);
#8399=EDGE_CURVE('',#6657,#6595,#4438,.T.);
#8400=EDGE_CURVE('',#6658,#6593,#4439,.T.);
#8401=EDGE_CURVE('',#6594,#6658,#4440,.T.);
#8402=EDGE_CURVE('',#6558,#6658,#4441,.T.);
#8403=EDGE_CURVE('',#6592,#6659,#4442,.T.);
#8404=EDGE_CURVE('',#6561,#6659,#4443,.T.);
#8405=EDGE_CURVE('',#6659,#6591,#4444,.T.);
#8406=EDGE_CURVE('',#6660,#6589,#4445,.T.);
#8407=EDGE_CURVE('',#6590,#6660,#4446,.T.);
#8408=EDGE_CURVE('',#6564,#6660,#4447,.T.);
#8409=EDGE_CURVE('',#6588,#6661,#4448,.T.);
#8410=EDGE_CURVE('',#6567,#6661,#4449,.T.);
#8411=EDGE_CURVE('',#6661,#6587,#4450,.T.);
#8412=EDGE_CURVE('',#6662,#6585,#4451,.T.);
#8413=EDGE_CURVE('',#6586,#6662,#4452,.T.);
#8414=EDGE_CURVE('',#6570,#6662,#4453,.T.);
#8415=EDGE_CURVE('',#6584,#6663,#4454,.T.);
#8416=EDGE_CURVE('',#6573,#6663,#4455,.T.);
#8417=EDGE_CURVE('',#6663,#6583,#4456,.T.);
#8418=EDGE_CURVE('',#6664,#6580,#4457,.T.);
#8419=EDGE_CURVE('',#6582,#6664,#4458,.T.);
#8420=EDGE_CURVE('',#6471,#6664,#4459,.T.);
#8421=EDGE_CURVE('',#6648,#6665,#4460,.T.);
#8422=EDGE_CURVE('',#6474,#6665,#4461,.T.);
#8423=EDGE_CURVE('',#6665,#6647,#4462,.T.);
#8424=EDGE_CURVE('',#6666,#6645,#4463,.T.);
#8425=EDGE_CURVE('',#6646,#6666,#4464,.T.);
#8426=EDGE_CURVE('',#6477,#6666,#4465,.T.);
#8427=EDGE_CURVE('',#6644,#6667,#4466,.T.);
#8428=EDGE_CURVE('',#6480,#6667,#4467,.T.);
#8429=EDGE_CURVE('',#6667,#6643,#4468,.T.);
#8430=EDGE_CURVE('',#6668,#6641,#4469,.T.);
#8431=EDGE_CURVE('',#6642,#6668,#4470,.T.);
#8432=EDGE_CURVE('',#6483,#6668,#4471,.T.);
#8433=EDGE_CURVE('',#6640,#6669,#4472,.T.);
#8434=EDGE_CURVE('',#6486,#6669,#4473,.T.);
#8435=EDGE_CURVE('',#6669,#6639,#4474,.T.);
#8436=EDGE_CURVE('',#6670,#6637,#4475,.T.);
#8437=EDGE_CURVE('',#6638,#6670,#4476,.T.);
#8438=EDGE_CURVE('',#6489,#6670,#4477,.T.);
#8439=EDGE_CURVE('',#6636,#6671,#4478,.T.);
#8440=EDGE_CURVE('',#6492,#6671,#4479,.T.);
#8441=EDGE_CURVE('',#6671,#6635,#4480,.T.);
#8442=EDGE_CURVE('',#6672,#6633,#4481,.T.);
#8443=EDGE_CURVE('',#6634,#6672,#4482,.T.);
#8444=EDGE_CURVE('',#6495,#6672,#4483,.T.);
#8445=EDGE_CURVE('',#6632,#6673,#4484,.T.);
#8446=EDGE_CURVE('',#6498,#6673,#4485,.T.);
#8447=EDGE_CURVE('',#6673,#6631,#4486,.T.);
#8448=EDGE_CURVE('',#6674,#6629,#4487,.T.);
#8449=EDGE_CURVE('',#6630,#6674,#4488,.T.);
#8450=EDGE_CURVE('',#6501,#6674,#4489,.T.);
#8451=EDGE_CURVE('',#6628,#6675,#4490,.T.);
#8452=EDGE_CURVE('',#6504,#6675,#4491,.T.);
#8453=EDGE_CURVE('',#6675,#6627,#4492,.T.);
#8454=EDGE_CURVE('',#6676,#6625,#4493,.T.);
#8455=EDGE_CURVE('',#6626,#6676,#4494,.T.);
#8456=EDGE_CURVE('',#6507,#6676,#4495,.T.);
#8457=EDGE_CURVE('',#6624,#6677,#4496,.T.);
#8458=EDGE_CURVE('',#6510,#6677,#4497,.T.);
#8459=EDGE_CURVE('',#6677,#6623,#4498,.T.);
#8460=EDGE_CURVE('',#6678,#6621,#4499,.T.);
#8461=EDGE_CURVE('',#6622,#6678,#4500,.T.);
#8462=EDGE_CURVE('',#6513,#6678,#4501,.T.);
#8463=EDGE_CURVE('',#6620,#6679,#4502,.T.);
#8464=EDGE_CURVE('',#6516,#6679,#4503,.T.);
#8465=EDGE_CURVE('',#6679,#6619,#4504,.T.);
#8466=EDGE_CURVE('',#6680,#6617,#4505,.T.);
#8467=EDGE_CURVE('',#6618,#6680,#4506,.T.);
#8468=EDGE_CURVE('',#6519,#6680,#4507,.T.);
#8469=EDGE_CURVE('',#6616,#6681,#4508,.T.);
#8470=EDGE_CURVE('',#6522,#6681,#4509,.T.);
#8471=EDGE_CURVE('',#6681,#6615,#4510,.T.);
#8472=EDGE_CURVE('',#6682,#6613,#4511,.T.);
#8473=EDGE_CURVE('',#6614,#6682,#4512,.T.);
#8474=EDGE_CURVE('',#6525,#6682,#4513,.T.);
#8475=EDGE_CURVE('',#6683,#6684,#4514,.T.);
#8476=EDGE_CURVE('',#6684,#6685,#4515,.T.);
#8477=EDGE_CURVE('',#6685,#6686,#4516,.T.);
#8478=EDGE_CURVE('',#6686,#6687,#4517,.T.);
#8479=EDGE_CURVE('',#6687,#6688,#4518,.T.);
#8480=EDGE_CURVE('',#6688,#6683,#4519,.T.);
#8481=EDGE_CURVE('',#6689,#6690,#4520,.T.);
#8482=EDGE_CURVE('',#6690,#6689,#3740,.T.);
#8483=EDGE_CURVE('',#6690,#6691,#4521,.T.);
#8484=EDGE_CURVE('',#6691,#6690,#3741,.T.);
#8485=EDGE_CURVE('',#6691,#6692,#4522,.T.);
#8486=EDGE_CURVE('',#6692,#6691,#3742,.T.);
#8487=EDGE_CURVE('',#6692,#6693,#4523,.T.);
#8488=EDGE_CURVE('',#6693,#6692,#3743,.T.);
#8489=EDGE_CURVE('',#6693,#6694,#4524,.T.);
#8490=EDGE_CURVE('',#6694,#6693,#3744,.T.);
#8491=EDGE_CURVE('',#6694,#6689,#4525,.T.);
#8492=EDGE_CURVE('',#6689,#6694,#3745,.T.);
#8493=EDGE_CURVE('',#6695,#6692,#4526,.T.);
#8494=EDGE_CURVE('',#6683,#6689,#4527,.T.);
#8495=EDGE_CURVE('',#6684,#6690,#4528,.T.);
#8496=EDGE_CURVE('',#6688,#6694,#4529,.T.);
#8497=EDGE_CURVE('',#6687,#6693,#4530,.T.);
#8498=EDGE_CURVE('',#6686,#6692,#4531,.T.);
#8499=EDGE_CURVE('',#6685,#6691,#4532,.T.);
#10847=ORIENTED_EDGE('',*,*,#7958,.F.);
#10848=ORIENTED_EDGE('',*,*,#7959,.F.);
#10849=ORIENTED_EDGE('',*,*,#7960,.F.);
#10850=ORIENTED_EDGE('',*,*,#7961,.T.);
#10851=ORIENTED_EDGE('',*,*,#7962,.F.);
#10852=ORIENTED_EDGE('',*,*,#7963,.F.);
#10853=ORIENTED_EDGE('',*,*,#7964,.F.);
#10854=ORIENTED_EDGE('',*,*,#7958,.T.);
#10855=ORIENTED_EDGE('',*,*,#7965,.T.);
#10856=ORIENTED_EDGE('',*,*,#7966,.T.);
#10857=ORIENTED_EDGE('',*,*,#7967,.F.);
#10858=ORIENTED_EDGE('',*,*,#7968,.F.);
#10859=ORIENTED_EDGE('',*,*,#7969,.F.);
#10860=ORIENTED_EDGE('',*,*,#7962,.T.);
#10861=ORIENTED_EDGE('',*,*,#7970,.T.);
#10862=ORIENTED_EDGE('',*,*,#7971,.F.);
#10863=ORIENTED_EDGE('',*,*,#7972,.F.);
#10864=ORIENTED_EDGE('',*,*,#7967,.T.);
#10865=ORIENTED_EDGE('',*,*,#7973,.T.);
#10866=ORIENTED_EDGE('',*,*,#7974,.T.);
#10867=ORIENTED_EDGE('',*,*,#7975,.F.);
#10868=ORIENTED_EDGE('',*,*,#7976,.F.);
#10869=ORIENTED_EDGE('',*,*,#7977,.F.);
#10870=ORIENTED_EDGE('',*,*,#7971,.T.);
#10871=ORIENTED_EDGE('',*,*,#7978,.T.);
#10872=ORIENTED_EDGE('',*,*,#7979,.F.);
#10873=ORIENTED_EDGE('',*,*,#7980,.F.);
#10874=ORIENTED_EDGE('',*,*,#7975,.T.);
#10875=ORIENTED_EDGE('',*,*,#7981,.T.);
#10876=ORIENTED_EDGE('',*,*,#7982,.T.);
#10877=ORIENTED_EDGE('',*,*,#7983,.F.);
#10878=ORIENTED_EDGE('',*,*,#7984,.F.);
#10879=ORIENTED_EDGE('',*,*,#7985,.F.);
#10880=ORIENTED_EDGE('',*,*,#7979,.T.);
#10881=ORIENTED_EDGE('',*,*,#7986,.T.);
#10882=ORIENTED_EDGE('',*,*,#7987,.F.);
#10883=ORIENTED_EDGE('',*,*,#7988,.F.);
#10884=ORIENTED_EDGE('',*,*,#7983,.T.);
#10885=ORIENTED_EDGE('',*,*,#7989,.T.);
#10886=ORIENTED_EDGE('',*,*,#7990,.T.);
#10887=ORIENTED_EDGE('',*,*,#7991,.F.);
#10888=ORIENTED_EDGE('',*,*,#7992,.F.);
#10889=ORIENTED_EDGE('',*,*,#7993,.F.);
#10890=ORIENTED_EDGE('',*,*,#7987,.T.);
#10891=ORIENTED_EDGE('',*,*,#7994,.T.);
#10892=ORIENTED_EDGE('',*,*,#7995,.F.);
#10893=ORIENTED_EDGE('',*,*,#7996,.F.);
#10894=ORIENTED_EDGE('',*,*,#7991,.T.);
#10895=ORIENTED_EDGE('',*,*,#7997,.T.);
#10896=ORIENTED_EDGE('',*,*,#7998,.T.);
#10897=ORIENTED_EDGE('',*,*,#7999,.F.);
#10898=ORIENTED_EDGE('',*,*,#8000,.F.);
#10899=ORIENTED_EDGE('',*,*,#8001,.F.);
#10900=ORIENTED_EDGE('',*,*,#7995,.T.);
#10901=ORIENTED_EDGE('',*,*,#8002,.T.);
#10902=ORIENTED_EDGE('',*,*,#8003,.F.);
#10903=ORIENTED_EDGE('',*,*,#8004,.F.);
#10904=ORIENTED_EDGE('',*,*,#7999,.T.);
#10905=ORIENTED_EDGE('',*,*,#8005,.T.);
#10906=ORIENTED_EDGE('',*,*,#8006,.T.);
#10907=ORIENTED_EDGE('',*,*,#8007,.F.);
#10908=ORIENTED_EDGE('',*,*,#8008,.F.);
#10909=ORIENTED_EDGE('',*,*,#8009,.F.);
#10910=ORIENTED_EDGE('',*,*,#8003,.T.);
#10911=ORIENTED_EDGE('',*,*,#8010,.T.);
#10912=ORIENTED_EDGE('',*,*,#8011,.F.);
#10913=ORIENTED_EDGE('',*,*,#8012,.F.);
#10914=ORIENTED_EDGE('',*,*,#8007,.T.);
#10915=ORIENTED_EDGE('',*,*,#8013,.T.);
#10916=ORIENTED_EDGE('',*,*,#8014,.T.);
#10917=ORIENTED_EDGE('',*,*,#8015,.F.);
#10918=ORIENTED_EDGE('',*,*,#8016,.F.);
#10919=ORIENTED_EDGE('',*,*,#8017,.F.);
#10920=ORIENTED_EDGE('',*,*,#8011,.T.);
#10921=ORIENTED_EDGE('',*,*,#8018,.T.);
#10922=ORIENTED_EDGE('',*,*,#8019,.F.);
#10923=ORIENTED_EDGE('',*,*,#8020,.F.);
#10924=ORIENTED_EDGE('',*,*,#8015,.T.);
#10925=ORIENTED_EDGE('',*,*,#8021,.T.);
#10926=ORIENTED_EDGE('',*,*,#8022,.T.);
#10927=ORIENTED_EDGE('',*,*,#8023,.F.);
#10928=ORIENTED_EDGE('',*,*,#8024,.F.);
#10929=ORIENTED_EDGE('',*,*,#8025,.F.);
#10930=ORIENTED_EDGE('',*,*,#8019,.T.);
#10931=ORIENTED_EDGE('',*,*,#8026,.T.);
#10932=ORIENTED_EDGE('',*,*,#8027,.F.);
#10933=ORIENTED_EDGE('',*,*,#8028,.F.);
#10934=ORIENTED_EDGE('',*,*,#8023,.T.);
#10935=ORIENTED_EDGE('',*,*,#8029,.T.);
#10936=ORIENTED_EDGE('',*,*,#8030,.T.);
#10937=ORIENTED_EDGE('',*,*,#8031,.F.);
#10938=ORIENTED_EDGE('',*,*,#8032,.F.);
#10939=ORIENTED_EDGE('',*,*,#8033,.F.);
#10940=ORIENTED_EDGE('',*,*,#8027,.T.);
#10941=ORIENTED_EDGE('',*,*,#8034,.T.);
#10942=ORIENTED_EDGE('',*,*,#8035,.F.);
#10943=ORIENTED_EDGE('',*,*,#8036,.F.);
#10944=ORIENTED_EDGE('',*,*,#8031,.T.);
#10945=ORIENTED_EDGE('',*,*,#8037,.T.);
#10946=ORIENTED_EDGE('',*,*,#8038,.T.);
#10947=ORIENTED_EDGE('',*,*,#8039,.F.);
#10948=ORIENTED_EDGE('',*,*,#8040,.F.);
#10949=ORIENTED_EDGE('',*,*,#8041,.F.);
#10950=ORIENTED_EDGE('',*,*,#8035,.T.);
#10951=ORIENTED_EDGE('',*,*,#8042,.T.);
#10952=ORIENTED_EDGE('',*,*,#8043,.F.);
#10953=ORIENTED_EDGE('',*,*,#8044,.F.);
#10954=ORIENTED_EDGE('',*,*,#8045,.F.);
#10955=ORIENTED_EDGE('',*,*,#8039,.T.);
#10956=ORIENTED_EDGE('',*,*,#8046,.T.);
#10957=ORIENTED_EDGE('',*,*,#8047,.T.);
#10958=ORIENTED_EDGE('',*,*,#8048,.F.);
#10959=ORIENTED_EDGE('',*,*,#8049,.F.);
#10960=ORIENTED_EDGE('',*,*,#8043,.T.);
#10961=ORIENTED_EDGE('',*,*,#8050,.T.);
#10962=ORIENTED_EDGE('',*,*,#8051,.F.);
#10963=ORIENTED_EDGE('',*,*,#8052,.F.);
#10964=ORIENTED_EDGE('',*,*,#8053,.F.);
#10965=ORIENTED_EDGE('',*,*,#8048,.T.);
#10966=ORIENTED_EDGE('',*,*,#8054,.T.);
#10967=ORIENTED_EDGE('',*,*,#8055,.T.);
#10968=ORIENTED_EDGE('',*,*,#8056,.F.);
#10969=ORIENTED_EDGE('',*,*,#8057,.F.);
#10970=ORIENTED_EDGE('',*,*,#8051,.T.);
#10971=ORIENTED_EDGE('',*,*,#8058,.T.);
#10972=ORIENTED_EDGE('',*,*,#8059,.T.);
#10973=ORIENTED_EDGE('',*,*,#8060,.F.);
#10974=ORIENTED_EDGE('',*,*,#8061,.F.);
#10975=ORIENTED_EDGE('',*,*,#8062,.F.);
#10976=ORIENTED_EDGE('',*,*,#8056,.T.);
#10977=ORIENTED_EDGE('',*,*,#8063,.T.);
#10978=ORIENTED_EDGE('',*,*,#8064,.F.);
#10979=ORIENTED_EDGE('',*,*,#8065,.F.);
#10980=ORIENTED_EDGE('',*,*,#8060,.T.);
#10981=ORIENTED_EDGE('',*,*,#8066,.T.);
#10982=ORIENTED_EDGE('',*,*,#8067,.T.);
#10983=ORIENTED_EDGE('',*,*,#8068,.T.);
#10984=ORIENTED_EDGE('',*,*,#8069,.F.);
#10985=ORIENTED_EDGE('',*,*,#8070,.T.);
#10986=ORIENTED_EDGE('',*,*,#8071,.T.);
#10987=ORIENTED_EDGE('',*,*,#8072,.T.);
#10988=ORIENTED_EDGE('',*,*,#8073,.T.);
#10989=ORIENTED_EDGE('',*,*,#8074,.T.);
#10990=ORIENTED_EDGE('',*,*,#8075,.T.);
#10991=ORIENTED_EDGE('',*,*,#8076,.T.);
#10992=ORIENTED_EDGE('',*,*,#8077,.T.);
#10993=ORIENTED_EDGE('',*,*,#8078,.T.);
#10994=ORIENTED_EDGE('',*,*,#8079,.T.);
#10995=ORIENTED_EDGE('',*,*,#8080,.T.);
#10996=ORIENTED_EDGE('',*,*,#8081,.T.);
#10997=ORIENTED_EDGE('',*,*,#8082,.T.);
#10998=ORIENTED_EDGE('',*,*,#8083,.T.);
#10999=ORIENTED_EDGE('',*,*,#8084,.T.);
#11000=ORIENTED_EDGE('',*,*,#8085,.T.);
#11001=ORIENTED_EDGE('',*,*,#8086,.T.);
#11002=ORIENTED_EDGE('',*,*,#8087,.T.);
#11003=ORIENTED_EDGE('',*,*,#8088,.T.);
#11004=ORIENTED_EDGE('',*,*,#8089,.T.);
#11005=ORIENTED_EDGE('',*,*,#8090,.T.);
#11006=ORIENTED_EDGE('',*,*,#8091,.T.);
#11007=ORIENTED_EDGE('',*,*,#8092,.T.);
#11008=ORIENTED_EDGE('',*,*,#8093,.T.);
#11009=ORIENTED_EDGE('',*,*,#8094,.T.);
#11010=ORIENTED_EDGE('',*,*,#8095,.T.);
#11011=ORIENTED_EDGE('',*,*,#8096,.T.);
#11012=ORIENTED_EDGE('',*,*,#8097,.T.);
#11013=ORIENTED_EDGE('',*,*,#8098,.T.);
#11014=ORIENTED_EDGE('',*,*,#8099,.F.);
#11015=ORIENTED_EDGE('',*,*,#8100,.F.);
#11016=ORIENTED_EDGE('',*,*,#8101,.T.);
#11017=ORIENTED_EDGE('',*,*,#8102,.T.);
#11018=ORIENTED_EDGE('',*,*,#8103,.T.);
#11019=ORIENTED_EDGE('',*,*,#8104,.T.);
#11020=ORIENTED_EDGE('',*,*,#8105,.T.);
#11021=ORIENTED_EDGE('',*,*,#8106,.T.);
#11022=ORIENTED_EDGE('',*,*,#8107,.T.);
#11023=ORIENTED_EDGE('',*,*,#8108,.T.);
#11024=ORIENTED_EDGE('',*,*,#8109,.T.);
#11025=ORIENTED_EDGE('',*,*,#8110,.T.);
#11026=ORIENTED_EDGE('',*,*,#8111,.T.);
#11027=ORIENTED_EDGE('',*,*,#8112,.T.);
#11028=ORIENTED_EDGE('',*,*,#8113,.T.);
#11029=ORIENTED_EDGE('',*,*,#8114,.T.);
#11030=ORIENTED_EDGE('',*,*,#8115,.T.);
#11031=ORIENTED_EDGE('',*,*,#8116,.T.);
#11032=ORIENTED_EDGE('',*,*,#8117,.T.);
#11033=ORIENTED_EDGE('',*,*,#8118,.T.);
#11034=ORIENTED_EDGE('',*,*,#8119,.T.);
#11035=ORIENTED_EDGE('',*,*,#8120,.T.);
#11036=ORIENTED_EDGE('',*,*,#8121,.T.);
#11037=ORIENTED_EDGE('',*,*,#8122,.T.);
#11038=ORIENTED_EDGE('',*,*,#8123,.T.);
#11039=ORIENTED_EDGE('',*,*,#8124,.T.);
#11040=ORIENTED_EDGE('',*,*,#8125,.T.);
#11041=ORIENTED_EDGE('',*,*,#8126,.T.);
#11042=ORIENTED_EDGE('',*,*,#8127,.T.);
#11043=ORIENTED_EDGE('',*,*,#8064,.T.);
#11044=ORIENTED_EDGE('',*,*,#8128,.T.);
#11045=ORIENTED_EDGE('',*,*,#8129,.T.);
#11046=ORIENTED_EDGE('',*,*,#8130,.F.);
#11047=ORIENTED_EDGE('',*,*,#8131,.F.);
#11048=ORIENTED_EDGE('',*,*,#8132,.F.);
#11049=ORIENTED_EDGE('',*,*,#8133,.F.);
#11050=ORIENTED_EDGE('',*,*,#8134,.T.);
#11051=ORIENTED_EDGE('',*,*,#8130,.T.);
#11052=ORIENTED_EDGE('',*,*,#8135,.T.);
#11053=ORIENTED_EDGE('',*,*,#8134,.F.);
#11054=ORIENTED_EDGE('',*,*,#8136,.F.);
#11055=ORIENTED_EDGE('',*,*,#8098,.F.);
#11056=ORIENTED_EDGE('',*,*,#8097,.F.);
#11057=ORIENTED_EDGE('',*,*,#8096,.F.);
#11058=ORIENTED_EDGE('',*,*,#8095,.F.);
#11059=ORIENTED_EDGE('',*,*,#8094,.F.);
#11060=ORIENTED_EDGE('',*,*,#8093,.F.);
#11061=ORIENTED_EDGE('',*,*,#8092,.F.);
#11062=ORIENTED_EDGE('',*,*,#8091,.F.);
#11063=ORIENTED_EDGE('',*,*,#8090,.F.);
#11064=ORIENTED_EDGE('',*,*,#8089,.F.);
#11065=ORIENTED_EDGE('',*,*,#8088,.F.);
#11066=ORIENTED_EDGE('',*,*,#8087,.F.);
#11067=ORIENTED_EDGE('',*,*,#8086,.F.);
#11068=ORIENTED_EDGE('',*,*,#8085,.F.);
#11069=ORIENTED_EDGE('',*,*,#8084,.F.);
#11070=ORIENTED_EDGE('',*,*,#8083,.F.);
#11071=ORIENTED_EDGE('',*,*,#8082,.F.);
#11072=ORIENTED_EDGE('',*,*,#8081,.F.);
#11073=ORIENTED_EDGE('',*,*,#8080,.F.);
#11074=ORIENTED_EDGE('',*,*,#8079,.F.);
#11075=ORIENTED_EDGE('',*,*,#8078,.F.);
#11076=ORIENTED_EDGE('',*,*,#8077,.F.);
#11077=ORIENTED_EDGE('',*,*,#8076,.F.);
#11078=ORIENTED_EDGE('',*,*,#8075,.F.);
#11079=ORIENTED_EDGE('',*,*,#8074,.F.);
#11080=ORIENTED_EDGE('',*,*,#8073,.F.);
#11081=ORIENTED_EDGE('',*,*,#8072,.F.);
#11082=ORIENTED_EDGE('',*,*,#8071,.F.);
#11083=ORIENTED_EDGE('',*,*,#8070,.F.);
#11084=ORIENTED_EDGE('',*,*,#8137,.F.);
#11085=ORIENTED_EDGE('',*,*,#7959,.T.);
#11086=ORIENTED_EDGE('',*,*,#7964,.T.);
#11087=ORIENTED_EDGE('',*,*,#7963,.T.);
#11088=ORIENTED_EDGE('',*,*,#7969,.T.);
#11089=ORIENTED_EDGE('',*,*,#7968,.T.);
#11090=ORIENTED_EDGE('',*,*,#7972,.T.);
#11091=ORIENTED_EDGE('',*,*,#7977,.T.);
#11092=ORIENTED_EDGE('',*,*,#7976,.T.);
#11093=ORIENTED_EDGE('',*,*,#7980,.T.);
#11094=ORIENTED_EDGE('',*,*,#7985,.T.);
#11095=ORIENTED_EDGE('',*,*,#7984,.T.);
#11096=ORIENTED_EDGE('',*,*,#7988,.T.);
#11097=ORIENTED_EDGE('',*,*,#7993,.T.);
#11098=ORIENTED_EDGE('',*,*,#7992,.T.);
#11099=ORIENTED_EDGE('',*,*,#7996,.T.);
#11100=ORIENTED_EDGE('',*,*,#8001,.T.);
#11101=ORIENTED_EDGE('',*,*,#8000,.T.);
#11102=ORIENTED_EDGE('',*,*,#8004,.T.);
#11103=ORIENTED_EDGE('',*,*,#8009,.T.);
#11104=ORIENTED_EDGE('',*,*,#8008,.T.);
#11105=ORIENTED_EDGE('',*,*,#8012,.T.);
#11106=ORIENTED_EDGE('',*,*,#8017,.T.);
#11107=ORIENTED_EDGE('',*,*,#8016,.T.);
#11108=ORIENTED_EDGE('',*,*,#8020,.T.);
#11109=ORIENTED_EDGE('',*,*,#8025,.T.);
#11110=ORIENTED_EDGE('',*,*,#8024,.T.);
#11111=ORIENTED_EDGE('',*,*,#8028,.T.);
#11112=ORIENTED_EDGE('',*,*,#8033,.T.);
#11113=ORIENTED_EDGE('',*,*,#8032,.T.);
#11114=ORIENTED_EDGE('',*,*,#8036,.T.);
#11115=ORIENTED_EDGE('',*,*,#8041,.T.);
#11116=ORIENTED_EDGE('',*,*,#8040,.T.);
#11117=ORIENTED_EDGE('',*,*,#8045,.T.);
#11118=ORIENTED_EDGE('',*,*,#8044,.T.);
#11119=ORIENTED_EDGE('',*,*,#8049,.T.);
#11120=ORIENTED_EDGE('',*,*,#8053,.T.);
#11121=ORIENTED_EDGE('',*,*,#8052,.T.);
#11122=ORIENTED_EDGE('',*,*,#8057,.T.);
#11123=ORIENTED_EDGE('',*,*,#8062,.T.);
#11124=ORIENTED_EDGE('',*,*,#8061,.T.);
#11125=ORIENTED_EDGE('',*,*,#8065,.T.);
#11126=ORIENTED_EDGE('',*,*,#8132,.T.);
#11127=ORIENTED_EDGE('',*,*,#8131,.T.);
#11128=ORIENTED_EDGE('',*,*,#8138,.F.);
#11129=ORIENTED_EDGE('',*,*,#8139,.T.);
#11130=ORIENTED_EDGE('',*,*,#7960,.T.);
#11131=ORIENTED_EDGE('',*,*,#8137,.T.);
#11132=ORIENTED_EDGE('',*,*,#8140,.F.);
#11133=ORIENTED_EDGE('',*,*,#8135,.F.);
#11134=ORIENTED_EDGE('',*,*,#8129,.F.);
#11135=ORIENTED_EDGE('',*,*,#8128,.F.);
#11136=ORIENTED_EDGE('',*,*,#8067,.F.);
#11137=ORIENTED_EDGE('',*,*,#8066,.F.);
#11138=ORIENTED_EDGE('',*,*,#8063,.F.);
#11139=ORIENTED_EDGE('',*,*,#8059,.F.);
#11140=ORIENTED_EDGE('',*,*,#8058,.F.);
#11141=ORIENTED_EDGE('',*,*,#8055,.F.);
#11142=ORIENTED_EDGE('',*,*,#8054,.F.);
#11143=ORIENTED_EDGE('',*,*,#8050,.F.);
#11144=ORIENTED_EDGE('',*,*,#8047,.F.);
#11145=ORIENTED_EDGE('',*,*,#8046,.F.);
#11146=ORIENTED_EDGE('',*,*,#8042,.F.);
#11147=ORIENTED_EDGE('',*,*,#8038,.F.);
#11148=ORIENTED_EDGE('',*,*,#8037,.F.);
#11149=ORIENTED_EDGE('',*,*,#8034,.F.);
#11150=ORIENTED_EDGE('',*,*,#8030,.F.);
#11151=ORIENTED_EDGE('',*,*,#8029,.F.);
#11152=ORIENTED_EDGE('',*,*,#8026,.F.);
#11153=ORIENTED_EDGE('',*,*,#8022,.F.);
#11154=ORIENTED_EDGE('',*,*,#8021,.F.);
#11155=ORIENTED_EDGE('',*,*,#8018,.F.);
#11156=ORIENTED_EDGE('',*,*,#8014,.F.);
#11157=ORIENTED_EDGE('',*,*,#8013,.F.);
#11158=ORIENTED_EDGE('',*,*,#8010,.F.);
#11159=ORIENTED_EDGE('',*,*,#8006,.F.);
#11160=ORIENTED_EDGE('',*,*,#8005,.F.);
#11161=ORIENTED_EDGE('',*,*,#8002,.F.);
#11162=ORIENTED_EDGE('',*,*,#7998,.F.);
#11163=ORIENTED_EDGE('',*,*,#7997,.F.);
#11164=ORIENTED_EDGE('',*,*,#7994,.F.);
#11165=ORIENTED_EDGE('',*,*,#7990,.F.);
#11166=ORIENTED_EDGE('',*,*,#7989,.F.);
#11167=ORIENTED_EDGE('',*,*,#7986,.F.);
#11168=ORIENTED_EDGE('',*,*,#7982,.F.);
#11169=ORIENTED_EDGE('',*,*,#7981,.F.);
#11170=ORIENTED_EDGE('',*,*,#7978,.F.);
#11171=ORIENTED_EDGE('',*,*,#7974,.F.);
#11172=ORIENTED_EDGE('',*,*,#7973,.F.);
#11173=ORIENTED_EDGE('',*,*,#7970,.F.);
#11174=ORIENTED_EDGE('',*,*,#7966,.F.);
#11175=ORIENTED_EDGE('',*,*,#7965,.F.);
#11176=ORIENTED_EDGE('',*,*,#7961,.F.);
#11177=ORIENTED_EDGE('',*,*,#8139,.F.);
#11178=ORIENTED_EDGE('',*,*,#8141,.F.);
#11179=ORIENTED_EDGE('',*,*,#8068,.F.);
#11180=ORIENTED_EDGE('',*,*,#8127,.F.);
#11181=ORIENTED_EDGE('',*,*,#8126,.F.);
#11182=ORIENTED_EDGE('',*,*,#8125,.F.);
#11183=ORIENTED_EDGE('',*,*,#8124,.F.);
#11184=ORIENTED_EDGE('',*,*,#8123,.F.);
#11185=ORIENTED_EDGE('',*,*,#8122,.F.);
#11186=ORIENTED_EDGE('',*,*,#8121,.F.);
#11187=ORIENTED_EDGE('',*,*,#8120,.F.);
#11188=ORIENTED_EDGE('',*,*,#8119,.F.);
#11189=ORIENTED_EDGE('',*,*,#8118,.F.);
#11190=ORIENTED_EDGE('',*,*,#8117,.F.);
#11191=ORIENTED_EDGE('',*,*,#8116,.F.);
#11192=ORIENTED_EDGE('',*,*,#8115,.F.);
#11193=ORIENTED_EDGE('',*,*,#8114,.F.);
#11194=ORIENTED_EDGE('',*,*,#8113,.F.);
#11195=ORIENTED_EDGE('',*,*,#8112,.F.);
#11196=ORIENTED_EDGE('',*,*,#8111,.F.);
#11197=ORIENTED_EDGE('',*,*,#8110,.F.);
#11198=ORIENTED_EDGE('',*,*,#8109,.F.);
#11199=ORIENTED_EDGE('',*,*,#8108,.F.);
#11200=ORIENTED_EDGE('',*,*,#8107,.F.);
#11201=ORIENTED_EDGE('',*,*,#8106,.F.);
#11202=ORIENTED_EDGE('',*,*,#8105,.F.);
#11203=ORIENTED_EDGE('',*,*,#8104,.F.);
#11204=ORIENTED_EDGE('',*,*,#8103,.F.);
#11205=ORIENTED_EDGE('',*,*,#8102,.F.);
#11206=ORIENTED_EDGE('',*,*,#8101,.F.);
#11207=ORIENTED_EDGE('',*,*,#8142,.T.);
#11208=ORIENTED_EDGE('',*,*,#8143,.T.);
#11209=ORIENTED_EDGE('',*,*,#8140,.T.);
#11210=ORIENTED_EDGE('',*,*,#8069,.T.);
#11211=ORIENTED_EDGE('',*,*,#8141,.T.);
#11212=ORIENTED_EDGE('',*,*,#8138,.T.);
#11213=ORIENTED_EDGE('',*,*,#8143,.F.);
#11214=ORIENTED_EDGE('',*,*,#8144,.T.);
#11215=ORIENTED_EDGE('',*,*,#8142,.F.);
#11216=ORIENTED_EDGE('',*,*,#8100,.T.);
#11217=ORIENTED_EDGE('',*,*,#8145,.T.);
#11218=ORIENTED_EDGE('',*,*,#8146,.T.);
#11219=ORIENTED_EDGE('',*,*,#8145,.F.);
#11220=ORIENTED_EDGE('',*,*,#8099,.T.);
#11221=ORIENTED_EDGE('',*,*,#8136,.T.);
#11222=ORIENTED_EDGE('',*,*,#8133,.T.);
#11223=ORIENTED_EDGE('',*,*,#8146,.F.);
#11224=ORIENTED_EDGE('',*,*,#8147,.F.);
#11225=ORIENTED_EDGE('',*,*,#8148,.T.);
#11226=ORIENTED_EDGE('',*,*,#8149,.F.);
#11227=ORIENTED_EDGE('',*,*,#8150,.F.);
#11228=ORIENTED_EDGE('',*,*,#8151,.F.);
#11229=ORIENTED_EDGE('',*,*,#8149,.T.);
#11230=ORIENTED_EDGE('',*,*,#8152,.T.);
#11231=ORIENTED_EDGE('',*,*,#8153,.F.);
#11232=ORIENTED_EDGE('',*,*,#8154,.F.);
#11233=ORIENTED_EDGE('',*,*,#8152,.F.);
#11234=ORIENTED_EDGE('',*,*,#8148,.F.);
#11235=ORIENTED_EDGE('',*,*,#8155,.T.);
#11236=ORIENTED_EDGE('',*,*,#8156,.T.);
#11237=ORIENTED_EDGE('',*,*,#8157,.T.);
#11238=ORIENTED_EDGE('',*,*,#8158,.T.);
#11239=ORIENTED_EDGE('',*,*,#8159,.T.);
#11240=ORIENTED_EDGE('',*,*,#8160,.T.);
#11241=ORIENTED_EDGE('',*,*,#8161,.T.);
#11242=ORIENTED_EDGE('',*,*,#8162,.T.);
#11243=ORIENTED_EDGE('',*,*,#8163,.T.);
#11244=ORIENTED_EDGE('',*,*,#8164,.T.);
#11245=ORIENTED_EDGE('',*,*,#8165,.T.);
#11246=ORIENTED_EDGE('',*,*,#8166,.T.);
#11247=ORIENTED_EDGE('',*,*,#8167,.T.);
#11248=ORIENTED_EDGE('',*,*,#8168,.T.);
#11249=ORIENTED_EDGE('',*,*,#8169,.T.);
#11250=ORIENTED_EDGE('',*,*,#8170,.T.);
#11251=ORIENTED_EDGE('',*,*,#8171,.T.);
#11252=ORIENTED_EDGE('',*,*,#8172,.T.);
#11253=ORIENTED_EDGE('',*,*,#8173,.T.);
#11254=ORIENTED_EDGE('',*,*,#8174,.T.);
#11255=ORIENTED_EDGE('',*,*,#8175,.T.);
#11256=ORIENTED_EDGE('',*,*,#8176,.T.);
#11257=ORIENTED_EDGE('',*,*,#8177,.T.);
#11258=ORIENTED_EDGE('',*,*,#8178,.T.);
#11259=ORIENTED_EDGE('',*,*,#8179,.T.);
#11260=ORIENTED_EDGE('',*,*,#8180,.T.);
#11261=ORIENTED_EDGE('',*,*,#8181,.T.);
#11262=ORIENTED_EDGE('',*,*,#8182,.T.);
#11263=ORIENTED_EDGE('',*,*,#8183,.T.);
#11264=ORIENTED_EDGE('',*,*,#8184,.T.);
#11265=ORIENTED_EDGE('',*,*,#8185,.T.);
#11266=ORIENTED_EDGE('',*,*,#8186,.T.);
#11267=ORIENTED_EDGE('',*,*,#8187,.T.);
#11268=ORIENTED_EDGE('',*,*,#8188,.T.);
#11269=ORIENTED_EDGE('',*,*,#8189,.T.);
#11270=ORIENTED_EDGE('',*,*,#8190,.T.);
#11271=ORIENTED_EDGE('',*,*,#8191,.T.);
#11272=ORIENTED_EDGE('',*,*,#8192,.T.);
#11273=ORIENTED_EDGE('',*,*,#8193,.T.);
#11274=ORIENTED_EDGE('',*,*,#8194,.T.);
#11275=ORIENTED_EDGE('',*,*,#8195,.T.);
#11276=ORIENTED_EDGE('',*,*,#8196,.T.);
#11277=ORIENTED_EDGE('',*,*,#8197,.T.);
#11278=ORIENTED_EDGE('',*,*,#8198,.T.);
#11279=ORIENTED_EDGE('',*,*,#8199,.T.);
#11280=ORIENTED_EDGE('',*,*,#8200,.T.);
#11281=ORIENTED_EDGE('',*,*,#8201,.T.);
#11282=ORIENTED_EDGE('',*,*,#8202,.T.);
#11283=ORIENTED_EDGE('',*,*,#8203,.T.);
#11284=ORIENTED_EDGE('',*,*,#8204,.T.);
#11285=ORIENTED_EDGE('',*,*,#8205,.T.);
#11286=ORIENTED_EDGE('',*,*,#8206,.T.);
#11287=ORIENTED_EDGE('',*,*,#8207,.T.);
#11288=ORIENTED_EDGE('',*,*,#8208,.T.);
#11289=ORIENTED_EDGE('',*,*,#8209,.T.);
#11290=ORIENTED_EDGE('',*,*,#8210,.T.);
#11291=ORIENTED_EDGE('',*,*,#8150,.T.);
#11292=ORIENTED_EDGE('',*,*,#8151,.T.);
#11293=ORIENTED_EDGE('',*,*,#8211,.T.);
#11294=ORIENTED_EDGE('',*,*,#8212,.T.);
#11295=ORIENTED_EDGE('',*,*,#8213,.T.);
#11296=ORIENTED_EDGE('',*,*,#8214,.T.);
#11297=ORIENTED_EDGE('',*,*,#8215,.T.);
#11298=ORIENTED_EDGE('',*,*,#8216,.T.);
#11299=ORIENTED_EDGE('',*,*,#8217,.T.);
#11300=ORIENTED_EDGE('',*,*,#8218,.T.);
#11301=ORIENTED_EDGE('',*,*,#8219,.T.);
#11302=ORIENTED_EDGE('',*,*,#8220,.T.);
#11303=ORIENTED_EDGE('',*,*,#8221,.T.);
#11304=ORIENTED_EDGE('',*,*,#8222,.T.);
#11305=ORIENTED_EDGE('',*,*,#8223,.T.);
#11306=ORIENTED_EDGE('',*,*,#8224,.T.);
#11307=ORIENTED_EDGE('',*,*,#8225,.T.);
#11308=ORIENTED_EDGE('',*,*,#8226,.T.);
#11309=ORIENTED_EDGE('',*,*,#8227,.T.);
#11310=ORIENTED_EDGE('',*,*,#8228,.T.);
#11311=ORIENTED_EDGE('',*,*,#8229,.T.);
#11312=ORIENTED_EDGE('',*,*,#8230,.T.);
#11313=ORIENTED_EDGE('',*,*,#8231,.T.);
#11314=ORIENTED_EDGE('',*,*,#8232,.T.);
#11315=ORIENTED_EDGE('',*,*,#8233,.T.);
#11316=ORIENTED_EDGE('',*,*,#8234,.T.);
#11317=ORIENTED_EDGE('',*,*,#8235,.T.);
#11318=ORIENTED_EDGE('',*,*,#8236,.T.);
#11319=ORIENTED_EDGE('',*,*,#8237,.T.);
#11320=ORIENTED_EDGE('',*,*,#8238,.T.);
#11321=ORIENTED_EDGE('',*,*,#8239,.T.);
#11322=ORIENTED_EDGE('',*,*,#8240,.T.);
#11323=ORIENTED_EDGE('',*,*,#8241,.T.);
#11324=ORIENTED_EDGE('',*,*,#8242,.T.);
#11325=ORIENTED_EDGE('',*,*,#8243,.T.);
#11326=ORIENTED_EDGE('',*,*,#8244,.T.);
#11327=ORIENTED_EDGE('',*,*,#8245,.T.);
#11328=ORIENTED_EDGE('',*,*,#8246,.T.);
#11329=ORIENTED_EDGE('',*,*,#8247,.T.);
#11330=ORIENTED_EDGE('',*,*,#8248,.T.);
#11331=ORIENTED_EDGE('',*,*,#8249,.T.);
#11332=ORIENTED_EDGE('',*,*,#8250,.T.);
#11333=ORIENTED_EDGE('',*,*,#8251,.T.);
#11334=ORIENTED_EDGE('',*,*,#8252,.T.);
#11335=ORIENTED_EDGE('',*,*,#8253,.T.);
#11336=ORIENTED_EDGE('',*,*,#8254,.T.);
#11337=ORIENTED_EDGE('',*,*,#8255,.T.);
#11338=ORIENTED_EDGE('',*,*,#8256,.T.);
#11339=ORIENTED_EDGE('',*,*,#8257,.T.);
#11340=ORIENTED_EDGE('',*,*,#8258,.T.);
#11341=ORIENTED_EDGE('',*,*,#8259,.T.);
#11342=ORIENTED_EDGE('',*,*,#8260,.T.);
#11343=ORIENTED_EDGE('',*,*,#8261,.T.);
#11344=ORIENTED_EDGE('',*,*,#8262,.T.);
#11345=ORIENTED_EDGE('',*,*,#8261,.F.);
#11346=ORIENTED_EDGE('',*,*,#8263,.F.);
#11347=ORIENTED_EDGE('',*,*,#8264,.F.);
#11348=ORIENTED_EDGE('',*,*,#8265,.F.);
#11349=ORIENTED_EDGE('',*,*,#8266,.F.);
#11350=ORIENTED_EDGE('',*,*,#8265,.T.);
#11351=ORIENTED_EDGE('',*,*,#8267,.F.);
#11352=ORIENTED_EDGE('',*,*,#8212,.F.);
#11353=ORIENTED_EDGE('',*,*,#8268,.F.);
#11354=ORIENTED_EDGE('',*,*,#8213,.F.);
#11355=ORIENTED_EDGE('',*,*,#8267,.T.);
#11356=ORIENTED_EDGE('',*,*,#8264,.T.);
#11357=ORIENTED_EDGE('',*,*,#8269,.T.);
#11358=ORIENTED_EDGE('',*,*,#8270,.T.);
#11359=ORIENTED_EDGE('',*,*,#8144,.F.);
#11360=ORIENTED_EDGE('',*,*,#8270,.F.);
#11361=ORIENTED_EDGE('',*,*,#8271,.T.);
#11362=ORIENTED_EDGE('',*,*,#8272,.T.);
#11363=ORIENTED_EDGE('',*,*,#8259,.F.);
#11364=ORIENTED_EDGE('',*,*,#8273,.T.);
#11365=ORIENTED_EDGE('',*,*,#8274,.T.);
#11366=ORIENTED_EDGE('',*,*,#8275,.T.);
#11367=ORIENTED_EDGE('',*,*,#8256,.F.);
#11368=ORIENTED_EDGE('',*,*,#8276,.T.);
#11369=ORIENTED_EDGE('',*,*,#8277,.T.);
#11370=ORIENTED_EDGE('',*,*,#8278,.T.);
#11371=ORIENTED_EDGE('',*,*,#8253,.F.);
#11372=ORIENTED_EDGE('',*,*,#8279,.T.);
#11373=ORIENTED_EDGE('',*,*,#8280,.T.);
#11374=ORIENTED_EDGE('',*,*,#8281,.T.);
#11375=ORIENTED_EDGE('',*,*,#8250,.F.);
#11376=ORIENTED_EDGE('',*,*,#8282,.T.);
#11377=ORIENTED_EDGE('',*,*,#8283,.T.);
#11378=ORIENTED_EDGE('',*,*,#8284,.T.);
#11379=ORIENTED_EDGE('',*,*,#8247,.F.);
#11380=ORIENTED_EDGE('',*,*,#8285,.T.);
#11381=ORIENTED_EDGE('',*,*,#8286,.T.);
#11382=ORIENTED_EDGE('',*,*,#8287,.T.);
#11383=ORIENTED_EDGE('',*,*,#8244,.F.);
#11384=ORIENTED_EDGE('',*,*,#8288,.T.);
#11385=ORIENTED_EDGE('',*,*,#8289,.T.);
#11386=ORIENTED_EDGE('',*,*,#8290,.T.);
#11387=ORIENTED_EDGE('',*,*,#8241,.F.);
#11388=ORIENTED_EDGE('',*,*,#8291,.T.);
#11389=ORIENTED_EDGE('',*,*,#8292,.T.);
#11390=ORIENTED_EDGE('',*,*,#8293,.T.);
#11391=ORIENTED_EDGE('',*,*,#8238,.F.);
#11392=ORIENTED_EDGE('',*,*,#8294,.T.);
#11393=ORIENTED_EDGE('',*,*,#8295,.T.);
#11394=ORIENTED_EDGE('',*,*,#8296,.T.);
#11395=ORIENTED_EDGE('',*,*,#8235,.F.);
#11396=ORIENTED_EDGE('',*,*,#8297,.T.);
#11397=ORIENTED_EDGE('',*,*,#8298,.T.);
#11398=ORIENTED_EDGE('',*,*,#8299,.T.);
#11399=ORIENTED_EDGE('',*,*,#8232,.F.);
#11400=ORIENTED_EDGE('',*,*,#8300,.T.);
#11401=ORIENTED_EDGE('',*,*,#8301,.T.);
#11402=ORIENTED_EDGE('',*,*,#8302,.T.);
#11403=ORIENTED_EDGE('',*,*,#8229,.F.);
#11404=ORIENTED_EDGE('',*,*,#8303,.T.);
#11405=ORIENTED_EDGE('',*,*,#8304,.T.);
#11406=ORIENTED_EDGE('',*,*,#8305,.T.);
#11407=ORIENTED_EDGE('',*,*,#8226,.F.);
#11408=ORIENTED_EDGE('',*,*,#8306,.T.);
#11409=ORIENTED_EDGE('',*,*,#8307,.T.);
#11410=ORIENTED_EDGE('',*,*,#8308,.T.);
#11411=ORIENTED_EDGE('',*,*,#8223,.F.);
#11412=ORIENTED_EDGE('',*,*,#8309,.T.);
#11413=ORIENTED_EDGE('',*,*,#8310,.T.);
#11414=ORIENTED_EDGE('',*,*,#8311,.T.);
#11415=ORIENTED_EDGE('',*,*,#8220,.F.);
#11416=ORIENTED_EDGE('',*,*,#8312,.T.);
#11417=ORIENTED_EDGE('',*,*,#8313,.T.);
#11418=ORIENTED_EDGE('',*,*,#8314,.T.);
#11419=ORIENTED_EDGE('',*,*,#8217,.F.);
#11420=ORIENTED_EDGE('',*,*,#8315,.T.);
#11421=ORIENTED_EDGE('',*,*,#8316,.T.);
#11422=ORIENTED_EDGE('',*,*,#8317,.T.);
#11423=ORIENTED_EDGE('',*,*,#8214,.F.);
#11424=ORIENTED_EDGE('',*,*,#8268,.T.);
#11425=ORIENTED_EDGE('',*,*,#8263,.T.);
#11426=ORIENTED_EDGE('',*,*,#8266,.T.);
#11427=ORIENTED_EDGE('',*,*,#8211,.F.);
#11428=ORIENTED_EDGE('',*,*,#8153,.T.);
#11429=ORIENTED_EDGE('',*,*,#8154,.T.);
#11430=ORIENTED_EDGE('',*,*,#8147,.T.);
#11431=ORIENTED_EDGE('',*,*,#8210,.F.);
#11432=ORIENTED_EDGE('',*,*,#8318,.T.);
#11433=ORIENTED_EDGE('',*,*,#8319,.T.);
#11434=ORIENTED_EDGE('',*,*,#8320,.T.);
#11435=ORIENTED_EDGE('',*,*,#8207,.F.);
#11436=ORIENTED_EDGE('',*,*,#8321,.T.);
#11437=ORIENTED_EDGE('',*,*,#8322,.T.);
#11438=ORIENTED_EDGE('',*,*,#8323,.T.);
#11439=ORIENTED_EDGE('',*,*,#8204,.F.);
#11440=ORIENTED_EDGE('',*,*,#8324,.T.);
#11441=ORIENTED_EDGE('',*,*,#8325,.T.);
#11442=ORIENTED_EDGE('',*,*,#8326,.T.);
#11443=ORIENTED_EDGE('',*,*,#8201,.F.);
#11444=ORIENTED_EDGE('',*,*,#8327,.T.);
#11445=ORIENTED_EDGE('',*,*,#8328,.T.);
#11446=ORIENTED_EDGE('',*,*,#8329,.T.);
#11447=ORIENTED_EDGE('',*,*,#8198,.F.);
#11448=ORIENTED_EDGE('',*,*,#8330,.T.);
#11449=ORIENTED_EDGE('',*,*,#8331,.T.);
#11450=ORIENTED_EDGE('',*,*,#8332,.T.);
#11451=ORIENTED_EDGE('',*,*,#8195,.F.);
#11452=ORIENTED_EDGE('',*,*,#8333,.T.);
#11453=ORIENTED_EDGE('',*,*,#8334,.T.);
#11454=ORIENTED_EDGE('',*,*,#8335,.T.);
#11455=ORIENTED_EDGE('',*,*,#8192,.F.);
#11456=ORIENTED_EDGE('',*,*,#8336,.T.);
#11457=ORIENTED_EDGE('',*,*,#8337,.T.);
#11458=ORIENTED_EDGE('',*,*,#8338,.T.);
#11459=ORIENTED_EDGE('',*,*,#8189,.F.);
#11460=ORIENTED_EDGE('',*,*,#8339,.T.);
#11461=ORIENTED_EDGE('',*,*,#8340,.T.);
#11462=ORIENTED_EDGE('',*,*,#8341,.T.);
#11463=ORIENTED_EDGE('',*,*,#8186,.F.);
#11464=ORIENTED_EDGE('',*,*,#8342,.T.);
#11465=ORIENTED_EDGE('',*,*,#8343,.T.);
#11466=ORIENTED_EDGE('',*,*,#8344,.T.);
#11467=ORIENTED_EDGE('',*,*,#8183,.F.);
#11468=ORIENTED_EDGE('',*,*,#8345,.T.);
#11469=ORIENTED_EDGE('',*,*,#8346,.T.);
#11470=ORIENTED_EDGE('',*,*,#8347,.T.);
#11471=ORIENTED_EDGE('',*,*,#8180,.F.);
#11472=ORIENTED_EDGE('',*,*,#8348,.T.);
#11473=ORIENTED_EDGE('',*,*,#8349,.T.);
#11474=ORIENTED_EDGE('',*,*,#8350,.T.);
#11475=ORIENTED_EDGE('',*,*,#8177,.F.);
#11476=ORIENTED_EDGE('',*,*,#8351,.T.);
#11477=ORIENTED_EDGE('',*,*,#8352,.T.);
#11478=ORIENTED_EDGE('',*,*,#8353,.T.);
#11479=ORIENTED_EDGE('',*,*,#8174,.F.);
#11480=ORIENTED_EDGE('',*,*,#8354,.T.);
#11481=ORIENTED_EDGE('',*,*,#8355,.T.);
#11482=ORIENTED_EDGE('',*,*,#8356,.T.);
#11483=ORIENTED_EDGE('',*,*,#8171,.F.);
#11484=ORIENTED_EDGE('',*,*,#8357,.T.);
#11485=ORIENTED_EDGE('',*,*,#8358,.T.);
#11486=ORIENTED_EDGE('',*,*,#8359,.T.);
#11487=ORIENTED_EDGE('',*,*,#8168,.F.);
#11488=ORIENTED_EDGE('',*,*,#8360,.T.);
#11489=ORIENTED_EDGE('',*,*,#8361,.T.);
#11490=ORIENTED_EDGE('',*,*,#8362,.T.);
#11491=ORIENTED_EDGE('',*,*,#8165,.F.);
#11492=ORIENTED_EDGE('',*,*,#8363,.T.);
#11493=ORIENTED_EDGE('',*,*,#8364,.T.);
#11494=ORIENTED_EDGE('',*,*,#8365,.T.);
#11495=ORIENTED_EDGE('',*,*,#8162,.F.);
#11496=ORIENTED_EDGE('',*,*,#8366,.T.);
#11497=ORIENTED_EDGE('',*,*,#8367,.T.);
#11498=ORIENTED_EDGE('',*,*,#8368,.T.);
#11499=ORIENTED_EDGE('',*,*,#8159,.F.);
#11500=ORIENTED_EDGE('',*,*,#8369,.T.);
#11501=ORIENTED_EDGE('',*,*,#8370,.T.);
#11502=ORIENTED_EDGE('',*,*,#8371,.T.);
#11503=ORIENTED_EDGE('',*,*,#8156,.F.);
#11504=ORIENTED_EDGE('',*,*,#8372,.T.);
#11505=ORIENTED_EDGE('',*,*,#8317,.F.);
#11506=ORIENTED_EDGE('',*,*,#8373,.T.);
#11507=ORIENTED_EDGE('',*,*,#8374,.F.);
#11508=ORIENTED_EDGE('',*,*,#8215,.F.);
#11509=ORIENTED_EDGE('',*,*,#8216,.F.);
#11510=ORIENTED_EDGE('',*,*,#8374,.T.);
#11511=ORIENTED_EDGE('',*,*,#8375,.T.);
#11512=ORIENTED_EDGE('',*,*,#8315,.F.);
#11513=ORIENTED_EDGE('',*,*,#8316,.F.);
#11514=ORIENTED_EDGE('',*,*,#8375,.F.);
#11515=ORIENTED_EDGE('',*,*,#8373,.F.);
#11516=ORIENTED_EDGE('',*,*,#8313,.F.);
#11517=ORIENTED_EDGE('',*,*,#8376,.F.);
#11518=ORIENTED_EDGE('',*,*,#8377,.F.);
#11519=ORIENTED_EDGE('',*,*,#8314,.F.);
#11520=ORIENTED_EDGE('',*,*,#8377,.T.);
#11521=ORIENTED_EDGE('',*,*,#8378,.F.);
#11522=ORIENTED_EDGE('',*,*,#8218,.F.);
#11523=ORIENTED_EDGE('',*,*,#8312,.F.);
#11524=ORIENTED_EDGE('',*,*,#8219,.F.);
#11525=ORIENTED_EDGE('',*,*,#8378,.T.);
#11526=ORIENTED_EDGE('',*,*,#8376,.T.);
#11527=ORIENTED_EDGE('',*,*,#8311,.F.);
#11528=ORIENTED_EDGE('',*,*,#8379,.T.);
#11529=ORIENTED_EDGE('',*,*,#8380,.F.);
#11530=ORIENTED_EDGE('',*,*,#8221,.F.);
#11531=ORIENTED_EDGE('',*,*,#8222,.F.);
#11532=ORIENTED_EDGE('',*,*,#8380,.T.);
#11533=ORIENTED_EDGE('',*,*,#8381,.T.);
#11534=ORIENTED_EDGE('',*,*,#8309,.F.);
#11535=ORIENTED_EDGE('',*,*,#8310,.F.);
#11536=ORIENTED_EDGE('',*,*,#8381,.F.);
#11537=ORIENTED_EDGE('',*,*,#8379,.F.);
#11538=ORIENTED_EDGE('',*,*,#8307,.F.);
#11539=ORIENTED_EDGE('',*,*,#8382,.F.);
#11540=ORIENTED_EDGE('',*,*,#8383,.F.);
#11541=ORIENTED_EDGE('',*,*,#8308,.F.);
#11542=ORIENTED_EDGE('',*,*,#8383,.T.);
#11543=ORIENTED_EDGE('',*,*,#8384,.F.);
#11544=ORIENTED_EDGE('',*,*,#8224,.F.);
#11545=ORIENTED_EDGE('',*,*,#8306,.F.);
#11546=ORIENTED_EDGE('',*,*,#8225,.F.);
#11547=ORIENTED_EDGE('',*,*,#8384,.T.);
#11548=ORIENTED_EDGE('',*,*,#8382,.T.);
#11549=ORIENTED_EDGE('',*,*,#8305,.F.);
#11550=ORIENTED_EDGE('',*,*,#8385,.T.);
#11551=ORIENTED_EDGE('',*,*,#8386,.F.);
#11552=ORIENTED_EDGE('',*,*,#8227,.F.);
#11553=ORIENTED_EDGE('',*,*,#8228,.F.);
#11554=ORIENTED_EDGE('',*,*,#8386,.T.);
#11555=ORIENTED_EDGE('',*,*,#8387,.T.);
#11556=ORIENTED_EDGE('',*,*,#8303,.F.);
#11557=ORIENTED_EDGE('',*,*,#8304,.F.);
#11558=ORIENTED_EDGE('',*,*,#8387,.F.);
#11559=ORIENTED_EDGE('',*,*,#8385,.F.);
#11560=ORIENTED_EDGE('',*,*,#8301,.F.);
#11561=ORIENTED_EDGE('',*,*,#8388,.F.);
#11562=ORIENTED_EDGE('',*,*,#8389,.F.);
#11563=ORIENTED_EDGE('',*,*,#8302,.F.);
#11564=ORIENTED_EDGE('',*,*,#8389,.T.);
#11565=ORIENTED_EDGE('',*,*,#8390,.F.);
#11566=ORIENTED_EDGE('',*,*,#8230,.F.);
#11567=ORIENTED_EDGE('',*,*,#8300,.F.);
#11568=ORIENTED_EDGE('',*,*,#8231,.F.);
#11569=ORIENTED_EDGE('',*,*,#8390,.T.);
#11570=ORIENTED_EDGE('',*,*,#8388,.T.);
#11571=ORIENTED_EDGE('',*,*,#8299,.F.);
#11572=ORIENTED_EDGE('',*,*,#8391,.T.);
#11573=ORIENTED_EDGE('',*,*,#8392,.F.);
#11574=ORIENTED_EDGE('',*,*,#8233,.F.);
#11575=ORIENTED_EDGE('',*,*,#8234,.F.);
#11576=ORIENTED_EDGE('',*,*,#8392,.T.);
#11577=ORIENTED_EDGE('',*,*,#8393,.T.);
#11578=ORIENTED_EDGE('',*,*,#8297,.F.);
#11579=ORIENTED_EDGE('',*,*,#8298,.F.);
#11580=ORIENTED_EDGE('',*,*,#8393,.F.);
#11581=ORIENTED_EDGE('',*,*,#8391,.F.);
#11582=ORIENTED_EDGE('',*,*,#8295,.F.);
#11583=ORIENTED_EDGE('',*,*,#8394,.F.);
#11584=ORIENTED_EDGE('',*,*,#8395,.F.);
#11585=ORIENTED_EDGE('',*,*,#8296,.F.);
#11586=ORIENTED_EDGE('',*,*,#8395,.T.);
#11587=ORIENTED_EDGE('',*,*,#8396,.F.);
#11588=ORIENTED_EDGE('',*,*,#8236,.F.);
#11589=ORIENTED_EDGE('',*,*,#8294,.F.);
#11590=ORIENTED_EDGE('',*,*,#8237,.F.);
#11591=ORIENTED_EDGE('',*,*,#8396,.T.);
#11592=ORIENTED_EDGE('',*,*,#8394,.T.);
#11593=ORIENTED_EDGE('',*,*,#8293,.F.);
#11594=ORIENTED_EDGE('',*,*,#8397,.T.);
#11595=ORIENTED_EDGE('',*,*,#8398,.F.);
#11596=ORIENTED_EDGE('',*,*,#8239,.F.);
#11597=ORIENTED_EDGE('',*,*,#8240,.F.);
#11598=ORIENTED_EDGE('',*,*,#8398,.T.);
#11599=ORIENTED_EDGE('',*,*,#8399,.T.);
#11600=ORIENTED_EDGE('',*,*,#8291,.F.);
#11601=ORIENTED_EDGE('',*,*,#8292,.F.);
#11602=ORIENTED_EDGE('',*,*,#8399,.F.);
#11603=ORIENTED_EDGE('',*,*,#8397,.F.);
#11604=ORIENTED_EDGE('',*,*,#8289,.F.);
#11605=ORIENTED_EDGE('',*,*,#8400,.F.);
#11606=ORIENTED_EDGE('',*,*,#8401,.F.);
#11607=ORIENTED_EDGE('',*,*,#8290,.F.);
#11608=ORIENTED_EDGE('',*,*,#8401,.T.);
#11609=ORIENTED_EDGE('',*,*,#8402,.F.);
#11610=ORIENTED_EDGE('',*,*,#8242,.F.);
#11611=ORIENTED_EDGE('',*,*,#8288,.F.);
#11612=ORIENTED_EDGE('',*,*,#8243,.F.);
#11613=ORIENTED_EDGE('',*,*,#8402,.T.);
#11614=ORIENTED_EDGE('',*,*,#8400,.T.);
#11615=ORIENTED_EDGE('',*,*,#8287,.F.);
#11616=ORIENTED_EDGE('',*,*,#8403,.T.);
#11617=ORIENTED_EDGE('',*,*,#8404,.F.);
#11618=ORIENTED_EDGE('',*,*,#8245,.F.);
#11619=ORIENTED_EDGE('',*,*,#8246,.F.);
#11620=ORIENTED_EDGE('',*,*,#8404,.T.);
#11621=ORIENTED_EDGE('',*,*,#8405,.T.);
#11622=ORIENTED_EDGE('',*,*,#8285,.F.);
#11623=ORIENTED_EDGE('',*,*,#8286,.F.);
#11624=ORIENTED_EDGE('',*,*,#8405,.F.);
#11625=ORIENTED_EDGE('',*,*,#8403,.F.);
#11626=ORIENTED_EDGE('',*,*,#8283,.F.);
#11627=ORIENTED_EDGE('',*,*,#8406,.F.);
#11628=ORIENTED_EDGE('',*,*,#8407,.F.);
#11629=ORIENTED_EDGE('',*,*,#8284,.F.);
#11630=ORIENTED_EDGE('',*,*,#8407,.T.);
#11631=ORIENTED_EDGE('',*,*,#8408,.F.);
#11632=ORIENTED_EDGE('',*,*,#8248,.F.);
#11633=ORIENTED_EDGE('',*,*,#8282,.F.);
#11634=ORIENTED_EDGE('',*,*,#8249,.F.);
#11635=ORIENTED_EDGE('',*,*,#8408,.T.);
#11636=ORIENTED_EDGE('',*,*,#8406,.T.);
#11637=ORIENTED_EDGE('',*,*,#8281,.F.);
#11638=ORIENTED_EDGE('',*,*,#8409,.T.);
#11639=ORIENTED_EDGE('',*,*,#8410,.F.);
#11640=ORIENTED_EDGE('',*,*,#8251,.F.);
#11641=ORIENTED_EDGE('',*,*,#8252,.F.);
#11642=ORIENTED_EDGE('',*,*,#8410,.T.);
#11643=ORIENTED_EDGE('',*,*,#8411,.T.);
#11644=ORIENTED_EDGE('',*,*,#8279,.F.);
#11645=ORIENTED_EDGE('',*,*,#8280,.F.);
#11646=ORIENTED_EDGE('',*,*,#8411,.F.);
#11647=ORIENTED_EDGE('',*,*,#8409,.F.);
#11648=ORIENTED_EDGE('',*,*,#8277,.F.);
#11649=ORIENTED_EDGE('',*,*,#8412,.F.);
#11650=ORIENTED_EDGE('',*,*,#8413,.F.);
#11651=ORIENTED_EDGE('',*,*,#8278,.F.);
#11652=ORIENTED_EDGE('',*,*,#8413,.T.);
#11653=ORIENTED_EDGE('',*,*,#8414,.F.);
#11654=ORIENTED_EDGE('',*,*,#8254,.F.);
#11655=ORIENTED_EDGE('',*,*,#8276,.F.);
#11656=ORIENTED_EDGE('',*,*,#8255,.F.);
#11657=ORIENTED_EDGE('',*,*,#8414,.T.);
#11658=ORIENTED_EDGE('',*,*,#8412,.T.);
#11659=ORIENTED_EDGE('',*,*,#8275,.F.);
#11660=ORIENTED_EDGE('',*,*,#8415,.T.);
#11661=ORIENTED_EDGE('',*,*,#8416,.F.);
#11662=ORIENTED_EDGE('',*,*,#8257,.F.);
#11663=ORIENTED_EDGE('',*,*,#8258,.F.);
#11664=ORIENTED_EDGE('',*,*,#8416,.T.);
#11665=ORIENTED_EDGE('',*,*,#8417,.T.);
#11666=ORIENTED_EDGE('',*,*,#8273,.F.);
#11667=ORIENTED_EDGE('',*,*,#8274,.F.);
#11668=ORIENTED_EDGE('',*,*,#8417,.F.);
#11669=ORIENTED_EDGE('',*,*,#8415,.F.);
#11670=ORIENTED_EDGE('',*,*,#8269,.F.);
#11671=ORIENTED_EDGE('',*,*,#8418,.F.);
#11672=ORIENTED_EDGE('',*,*,#8419,.F.);
#11673=ORIENTED_EDGE('',*,*,#8271,.F.);
#11674=ORIENTED_EDGE('',*,*,#8272,.F.);
#11675=ORIENTED_EDGE('',*,*,#8419,.T.);
#11676=ORIENTED_EDGE('',*,*,#8420,.F.);
#11677=ORIENTED_EDGE('',*,*,#8260,.F.);
#11678=ORIENTED_EDGE('',*,*,#8372,.F.);
#11679=ORIENTED_EDGE('',*,*,#8155,.F.);
#11680=ORIENTED_EDGE('',*,*,#8420,.T.);
#11681=ORIENTED_EDGE('',*,*,#8418,.T.);
#11682=ORIENTED_EDGE('',*,*,#8371,.F.);
#11683=ORIENTED_EDGE('',*,*,#8421,.T.);
#11684=ORIENTED_EDGE('',*,*,#8422,.F.);
#11685=ORIENTED_EDGE('',*,*,#8157,.F.);
#11686=ORIENTED_EDGE('',*,*,#8158,.F.);
#11687=ORIENTED_EDGE('',*,*,#8422,.T.);
#11688=ORIENTED_EDGE('',*,*,#8423,.T.);
#11689=ORIENTED_EDGE('',*,*,#8369,.F.);
#11690=ORIENTED_EDGE('',*,*,#8370,.F.);
#11691=ORIENTED_EDGE('',*,*,#8423,.F.);
#11692=ORIENTED_EDGE('',*,*,#8421,.F.);
#11693=ORIENTED_EDGE('',*,*,#8367,.F.);
#11694=ORIENTED_EDGE('',*,*,#8424,.F.);
#11695=ORIENTED_EDGE('',*,*,#8425,.F.);
#11696=ORIENTED_EDGE('',*,*,#8368,.F.);
#11697=ORIENTED_EDGE('',*,*,#8425,.T.);
#11698=ORIENTED_EDGE('',*,*,#8426,.F.);
#11699=ORIENTED_EDGE('',*,*,#8160,.F.);
#11700=ORIENTED_EDGE('',*,*,#8366,.F.);
#11701=ORIENTED_EDGE('',*,*,#8161,.F.);
#11702=ORIENTED_EDGE('',*,*,#8426,.T.);
#11703=ORIENTED_EDGE('',*,*,#8424,.T.);
#11704=ORIENTED_EDGE('',*,*,#8365,.F.);
#11705=ORIENTED_EDGE('',*,*,#8427,.T.);
#11706=ORIENTED_EDGE('',*,*,#8428,.F.);
#11707=ORIENTED_EDGE('',*,*,#8163,.F.);
#11708=ORIENTED_EDGE('',*,*,#8164,.F.);
#11709=ORIENTED_EDGE('',*,*,#8428,.T.);
#11710=ORIENTED_EDGE('',*,*,#8429,.T.);
#11711=ORIENTED_EDGE('',*,*,#8363,.F.);
#11712=ORIENTED_EDGE('',*,*,#8364,.F.);
#11713=ORIENTED_EDGE('',*,*,#8429,.F.);
#11714=ORIENTED_EDGE('',*,*,#8427,.F.);
#11715=ORIENTED_EDGE('',*,*,#8361,.F.);
#11716=ORIENTED_EDGE('',*,*,#8430,.F.);
#11717=ORIENTED_EDGE('',*,*,#8431,.F.);
#11718=ORIENTED_EDGE('',*,*,#8362,.F.);
#11719=ORIENTED_EDGE('',*,*,#8431,.T.);
#11720=ORIENTED_EDGE('',*,*,#8432,.F.);
#11721=ORIENTED_EDGE('',*,*,#8166,.F.);
#11722=ORIENTED_EDGE('',*,*,#8360,.F.);
#11723=ORIENTED_EDGE('',*,*,#8167,.F.);
#11724=ORIENTED_EDGE('',*,*,#8432,.T.);
#11725=ORIENTED_EDGE('',*,*,#8430,.T.);
#11726=ORIENTED_EDGE('',*,*,#8359,.F.);
#11727=ORIENTED_EDGE('',*,*,#8433,.T.);
#11728=ORIENTED_EDGE('',*,*,#8434,.F.);
#11729=ORIENTED_EDGE('',*,*,#8169,.F.);
#11730=ORIENTED_EDGE('',*,*,#8170,.F.);
#11731=ORIENTED_EDGE('',*,*,#8434,.T.);
#11732=ORIENTED_EDGE('',*,*,#8435,.T.);
#11733=ORIENTED_EDGE('',*,*,#8357,.F.);
#11734=ORIENTED_EDGE('',*,*,#8358,.F.);
#11735=ORIENTED_EDGE('',*,*,#8435,.F.);
#11736=ORIENTED_EDGE('',*,*,#8433,.F.);
#11737=ORIENTED_EDGE('',*,*,#8355,.F.);
#11738=ORIENTED_EDGE('',*,*,#8436,.F.);
#11739=ORIENTED_EDGE('',*,*,#8437,.F.);
#11740=ORIENTED_EDGE('',*,*,#8356,.F.);
#11741=ORIENTED_EDGE('',*,*,#8437,.T.);
#11742=ORIENTED_EDGE('',*,*,#8438,.F.);
#11743=ORIENTED_EDGE('',*,*,#8172,.F.);
#11744=ORIENTED_EDGE('',*,*,#8354,.F.);
#11745=ORIENTED_EDGE('',*,*,#8173,.F.);
#11746=ORIENTED_EDGE('',*,*,#8438,.T.);
#11747=ORIENTED_EDGE('',*,*,#8436,.T.);
#11748=ORIENTED_EDGE('',*,*,#8353,.F.);
#11749=ORIENTED_EDGE('',*,*,#8439,.T.);
#11750=ORIENTED_EDGE('',*,*,#8440,.F.);
#11751=ORIENTED_EDGE('',*,*,#8175,.F.);
#11752=ORIENTED_EDGE('',*,*,#8176,.F.);
#11753=ORIENTED_EDGE('',*,*,#8440,.T.);
#11754=ORIENTED_EDGE('',*,*,#8441,.T.);
#11755=ORIENTED_EDGE('',*,*,#8351,.F.);
#11756=ORIENTED_EDGE('',*,*,#8352,.F.);
#11757=ORIENTED_EDGE('',*,*,#8441,.F.);
#11758=ORIENTED_EDGE('',*,*,#8439,.F.);
#11759=ORIENTED_EDGE('',*,*,#8349,.F.);
#11760=ORIENTED_EDGE('',*,*,#8442,.F.);
#11761=ORIENTED_EDGE('',*,*,#8443,.F.);
#11762=ORIENTED_EDGE('',*,*,#8350,.F.);
#11763=ORIENTED_EDGE('',*,*,#8443,.T.);
#11764=ORIENTED_EDGE('',*,*,#8444,.F.);
#11765=ORIENTED_EDGE('',*,*,#8178,.F.);
#11766=ORIENTED_EDGE('',*,*,#8348,.F.);
#11767=ORIENTED_EDGE('',*,*,#8179,.F.);
#11768=ORIENTED_EDGE('',*,*,#8444,.T.);
#11769=ORIENTED_EDGE('',*,*,#8442,.T.);
#11770=ORIENTED_EDGE('',*,*,#8347,.F.);
#11771=ORIENTED_EDGE('',*,*,#8445,.T.);
#11772=ORIENTED_EDGE('',*,*,#8446,.F.);
#11773=ORIENTED_EDGE('',*,*,#8181,.F.);
#11774=ORIENTED_EDGE('',*,*,#8182,.F.);
#11775=ORIENTED_EDGE('',*,*,#8446,.T.);
#11776=ORIENTED_EDGE('',*,*,#8447,.T.);
#11777=ORIENTED_EDGE('',*,*,#8345,.F.);
#11778=ORIENTED_EDGE('',*,*,#8346,.F.);
#11779=ORIENTED_EDGE('',*,*,#8447,.F.);
#11780=ORIENTED_EDGE('',*,*,#8445,.F.);
#11781=ORIENTED_EDGE('',*,*,#8343,.F.);
#11782=ORIENTED_EDGE('',*,*,#8448,.F.);
#11783=ORIENTED_EDGE('',*,*,#8449,.F.);
#11784=ORIENTED_EDGE('',*,*,#8344,.F.);
#11785=ORIENTED_EDGE('',*,*,#8449,.T.);
#11786=ORIENTED_EDGE('',*,*,#8450,.F.);
#11787=ORIENTED_EDGE('',*,*,#8184,.F.);
#11788=ORIENTED_EDGE('',*,*,#8342,.F.);
#11789=ORIENTED_EDGE('',*,*,#8185,.F.);
#11790=ORIENTED_EDGE('',*,*,#8450,.T.);
#11791=ORIENTED_EDGE('',*,*,#8448,.T.);
#11792=ORIENTED_EDGE('',*,*,#8341,.F.);
#11793=ORIENTED_EDGE('',*,*,#8451,.T.);
#11794=ORIENTED_EDGE('',*,*,#8452,.F.);
#11795=ORIENTED_EDGE('',*,*,#8187,.F.);
#11796=ORIENTED_EDGE('',*,*,#8188,.F.);
#11797=ORIENTED_EDGE('',*,*,#8452,.T.);
#11798=ORIENTED_EDGE('',*,*,#8453,.T.);
#11799=ORIENTED_EDGE('',*,*,#8339,.F.);
#11800=ORIENTED_EDGE('',*,*,#8340,.F.);
#11801=ORIENTED_EDGE('',*,*,#8453,.F.);
#11802=ORIENTED_EDGE('',*,*,#8451,.F.);
#11803=ORIENTED_EDGE('',*,*,#8337,.F.);
#11804=ORIENTED_EDGE('',*,*,#8454,.F.);
#11805=ORIENTED_EDGE('',*,*,#8455,.F.);
#11806=ORIENTED_EDGE('',*,*,#8338,.F.);
#11807=ORIENTED_EDGE('',*,*,#8455,.T.);
#11808=ORIENTED_EDGE('',*,*,#8456,.F.);
#11809=ORIENTED_EDGE('',*,*,#8190,.F.);
#11810=ORIENTED_EDGE('',*,*,#8336,.F.);
#11811=ORIENTED_EDGE('',*,*,#8191,.F.);
#11812=ORIENTED_EDGE('',*,*,#8456,.T.);
#11813=ORIENTED_EDGE('',*,*,#8454,.T.);
#11814=ORIENTED_EDGE('',*,*,#8335,.F.);
#11815=ORIENTED_EDGE('',*,*,#8457,.T.);
#11816=ORIENTED_EDGE('',*,*,#8458,.F.);
#11817=ORIENTED_EDGE('',*,*,#8193,.F.);
#11818=ORIENTED_EDGE('',*,*,#8194,.F.);
#11819=ORIENTED_EDGE('',*,*,#8458,.T.);
#11820=ORIENTED_EDGE('',*,*,#8459,.T.);
#11821=ORIENTED_EDGE('',*,*,#8333,.F.);
#11822=ORIENTED_EDGE('',*,*,#8334,.F.);
#11823=ORIENTED_EDGE('',*,*,#8459,.F.);
#11824=ORIENTED_EDGE('',*,*,#8457,.F.);
#11825=ORIENTED_EDGE('',*,*,#8331,.F.);
#11826=ORIENTED_EDGE('',*,*,#8460,.F.);
#11827=ORIENTED_EDGE('',*,*,#8461,.F.);
#11828=ORIENTED_EDGE('',*,*,#8332,.F.);
#11829=ORIENTED_EDGE('',*,*,#8461,.T.);
#11830=ORIENTED_EDGE('',*,*,#8462,.F.);
#11831=ORIENTED_EDGE('',*,*,#8196,.F.);
#11832=ORIENTED_EDGE('',*,*,#8330,.F.);
#11833=ORIENTED_EDGE('',*,*,#8197,.F.);
#11834=ORIENTED_EDGE('',*,*,#8462,.T.);
#11835=ORIENTED_EDGE('',*,*,#8460,.T.);
#11836=ORIENTED_EDGE('',*,*,#8329,.F.);
#11837=ORIENTED_EDGE('',*,*,#8463,.T.);
#11838=ORIENTED_EDGE('',*,*,#8464,.F.);
#11839=ORIENTED_EDGE('',*,*,#8199,.F.);
#11840=ORIENTED_EDGE('',*,*,#8200,.F.);
#11841=ORIENTED_EDGE('',*,*,#8464,.T.);
#11842=ORIENTED_EDGE('',*,*,#8465,.T.);
#11843=ORIENTED_EDGE('',*,*,#8327,.F.);
#11844=ORIENTED_EDGE('',*,*,#8328,.F.);
#11845=ORIENTED_EDGE('',*,*,#8465,.F.);
#11846=ORIENTED_EDGE('',*,*,#8463,.F.);
#11847=ORIENTED_EDGE('',*,*,#8325,.F.);
#11848=ORIENTED_EDGE('',*,*,#8466,.F.);
#11849=ORIENTED_EDGE('',*,*,#8467,.F.);
#11850=ORIENTED_EDGE('',*,*,#8326,.F.);
#11851=ORIENTED_EDGE('',*,*,#8467,.T.);
#11852=ORIENTED_EDGE('',*,*,#8468,.F.);
#11853=ORIENTED_EDGE('',*,*,#8202,.F.);
#11854=ORIENTED_EDGE('',*,*,#8324,.F.);
#11855=ORIENTED_EDGE('',*,*,#8203,.F.);
#11856=ORIENTED_EDGE('',*,*,#8468,.T.);
#11857=ORIENTED_EDGE('',*,*,#8466,.T.);
#11858=ORIENTED_EDGE('',*,*,#8323,.F.);
#11859=ORIENTED_EDGE('',*,*,#8469,.T.);
#11860=ORIENTED_EDGE('',*,*,#8470,.F.);
#11861=ORIENTED_EDGE('',*,*,#8205,.F.);
#11862=ORIENTED_EDGE('',*,*,#8206,.F.);
#11863=ORIENTED_EDGE('',*,*,#8470,.T.);
#11864=ORIENTED_EDGE('',*,*,#8471,.T.);
#11865=ORIENTED_EDGE('',*,*,#8321,.F.);
#11866=ORIENTED_EDGE('',*,*,#8322,.F.);
#11867=ORIENTED_EDGE('',*,*,#8471,.F.);
#11868=ORIENTED_EDGE('',*,*,#8469,.F.);
#11869=ORIENTED_EDGE('',*,*,#8319,.F.);
#11870=ORIENTED_EDGE('',*,*,#8472,.F.);
#11871=ORIENTED_EDGE('',*,*,#8473,.F.);
#11872=ORIENTED_EDGE('',*,*,#8320,.F.);
#11873=ORIENTED_EDGE('',*,*,#8473,.T.);
#11874=ORIENTED_EDGE('',*,*,#8474,.F.);
#11875=ORIENTED_EDGE('',*,*,#8208,.F.);
#11876=ORIENTED_EDGE('',*,*,#8318,.F.);
#11877=ORIENTED_EDGE('',*,*,#8209,.F.);
#11878=ORIENTED_EDGE('',*,*,#8474,.T.);
#11879=ORIENTED_EDGE('',*,*,#8472,.T.);
#11880=ORIENTED_EDGE('',*,*,#8262,.F.);
#11881=ORIENTED_EDGE('',*,*,#8475,.T.);
#11882=ORIENTED_EDGE('',*,*,#8476,.T.);
#11883=ORIENTED_EDGE('',*,*,#8477,.T.);
#11884=ORIENTED_EDGE('',*,*,#8478,.T.);
#11885=ORIENTED_EDGE('',*,*,#8479,.T.);
#11886=ORIENTED_EDGE('',*,*,#8480,.T.);
#11887=ORIENTED_EDGE('',*,*,#8481,.F.);
#11888=ORIENTED_EDGE('',*,*,#8482,.F.);
#11889=ORIENTED_EDGE('',*,*,#8483,.F.);
#11890=ORIENTED_EDGE('',*,*,#8484,.F.);
#11891=ORIENTED_EDGE('',*,*,#8485,.F.);
#11892=ORIENTED_EDGE('',*,*,#8486,.F.);
#11893=ORIENTED_EDGE('',*,*,#8487,.F.);
#11894=ORIENTED_EDGE('',*,*,#8488,.F.);
#11895=ORIENTED_EDGE('',*,*,#8489,.F.);
#11896=ORIENTED_EDGE('',*,*,#8490,.F.);
#11897=ORIENTED_EDGE('',*,*,#8491,.F.);
#11898=ORIENTED_EDGE('',*,*,#8492,.F.);
#11899=ORIENTED_EDGE('',*,*,#8493,.T.);
#11900=ORIENTED_EDGE('',*,*,#8486,.T.);
#11901=ORIENTED_EDGE('',*,*,#8484,.T.);
#11902=ORIENTED_EDGE('',*,*,#8482,.T.);
#11903=ORIENTED_EDGE('',*,*,#8492,.T.);
#11904=ORIENTED_EDGE('',*,*,#8490,.T.);
#11905=ORIENTED_EDGE('',*,*,#8488,.T.);
#11906=ORIENTED_EDGE('',*,*,#8493,.F.);
#11907=ORIENTED_EDGE('',*,*,#8475,.F.);
#11908=ORIENTED_EDGE('',*,*,#8494,.T.);
#11909=ORIENTED_EDGE('',*,*,#8481,.T.);
#11910=ORIENTED_EDGE('',*,*,#8495,.F.);
#11911=ORIENTED_EDGE('',*,*,#8480,.F.);
#11912=ORIENTED_EDGE('',*,*,#8496,.T.);
#11913=ORIENTED_EDGE('',*,*,#8491,.T.);
#11914=ORIENTED_EDGE('',*,*,#8494,.F.);
#11915=ORIENTED_EDGE('',*,*,#8479,.F.);
#11916=ORIENTED_EDGE('',*,*,#8497,.T.);
#11917=ORIENTED_EDGE('',*,*,#8489,.T.);
#11918=ORIENTED_EDGE('',*,*,#8496,.F.);
#11919=ORIENTED_EDGE('',*,*,#8478,.F.);
#11920=ORIENTED_EDGE('',*,*,#8498,.T.);
#11921=ORIENTED_EDGE('',*,*,#8487,.T.);
#11922=ORIENTED_EDGE('',*,*,#8497,.F.);
#11923=ORIENTED_EDGE('',*,*,#8477,.F.);
#11924=ORIENTED_EDGE('',*,*,#8499,.T.);
#11925=ORIENTED_EDGE('',*,*,#8485,.T.);
#11926=ORIENTED_EDGE('',*,*,#8498,.F.);
#11927=ORIENTED_EDGE('',*,*,#8476,.F.);
#11928=ORIENTED_EDGE('',*,*,#8495,.T.);
#11929=ORIENTED_EDGE('',*,*,#8483,.T.);
#11930=ORIENTED_EDGE('',*,*,#8499,.F.);
#12940=CYLINDRICAL_SURFACE('',#14359,1.92913);
#12941=CYLINDRICAL_SURFACE('',#14361,1.92913);
#12942=CYLINDRICAL_SURFACE('',#14362,1.92913);
#12943=CYLINDRICAL_SURFACE('',#14363,1.92913);
#12944=CYLINDRICAL_SURFACE('',#14364,1.92913);
#12945=CYLINDRICAL_SURFACE('',#14365,1.92913);
#12946=CYLINDRICAL_SURFACE('',#14366,1.92913);
#12947=CYLINDRICAL_SURFACE('',#14367,1.92913);
#12948=CYLINDRICAL_SURFACE('',#14368,1.92913);
#12949=CYLINDRICAL_SURFACE('',#14369,1.92913);
#12950=CYLINDRICAL_SURFACE('',#14370,1.92913);
#12951=CYLINDRICAL_SURFACE('',#14371,1.92913);
#12952=CYLINDRICAL_SURFACE('',#14372,1.92913);
#12953=CYLINDRICAL_SURFACE('',#14373,1.92913);
#12954=CYLINDRICAL_SURFACE('',#14374,1.92913);
#12955=CYLINDRICAL_SURFACE('',#14375,1.92913);
#12956=CYLINDRICAL_SURFACE('',#14376,1.92913);
#12957=CYLINDRICAL_SURFACE('',#14377,1.92913);
#12958=CYLINDRICAL_SURFACE('',#14378,1.92913);
#12959=CYLINDRICAL_SURFACE('',#14379,1.92913);
#12960=CYLINDRICAL_SURFACE('',#14380,1.92913);
#12961=CYLINDRICAL_SURFACE('',#14381,1.92913);
#12962=CYLINDRICAL_SURFACE('',#14382,1.92913);
#12963=CYLINDRICAL_SURFACE('',#14383,1.92913);
#12964=CYLINDRICAL_SURFACE('',#14384,1.92913);
#12965=CYLINDRICAL_SURFACE('',#14385,1.92913);
#12966=CYLINDRICAL_SURFACE('',#14386,1.92913);
#12967=CYLINDRICAL_SURFACE('',#14387,2.36347);
#12968=CYLINDRICAL_SURFACE('',#14391,1.92913);
#12969=CYLINDRICAL_SURFACE('',#14452,3.9624);
#13326=ADVANCED_FACE('',(#2366),#12940,.T.);
#13327=ADVANCED_FACE('',(#2367),#12941,.T.);
#13328=ADVANCED_FACE('',(#2368),#12942,.T.);
#13329=ADVANCED_FACE('',(#2369),#12943,.T.);
#13330=ADVANCED_FACE('',(#2370),#12944,.T.);
#13331=ADVANCED_FACE('',(#2371),#12945,.T.);
#13332=ADVANCED_FACE('',(#2372),#12946,.T.);
#13333=ADVANCED_FACE('',(#2373),#12947,.T.);
#13334=ADVANCED_FACE('',(#2374),#12948,.T.);
#13335=ADVANCED_FACE('',(#2375),#12949,.T.);
#13336=ADVANCED_FACE('',(#2376),#12950,.T.);
#13337=ADVANCED_FACE('',(#2377),#12951,.T.);
#13338=ADVANCED_FACE('',(#2378),#12952,.T.);
#13339=ADVANCED_FACE('',(#2379),#12953,.T.);
#13340=ADVANCED_FACE('',(#2380),#12954,.T.);
#13341=ADVANCED_FACE('',(#2381),#12955,.T.);
#13342=ADVANCED_FACE('',(#2382),#12956,.T.);
#13343=ADVANCED_FACE('',(#2383),#12957,.T.);
#13344=ADVANCED_FACE('',(#2384),#12958,.T.);
#13345=ADVANCED_FACE('',(#2385),#12959,.T.);
#13346=ADVANCED_FACE('',(#2386),#12960,.T.);
#13347=ADVANCED_FACE('',(#2387),#12961,.T.);
#13348=ADVANCED_FACE('',(#2388),#12962,.T.);
#13349=ADVANCED_FACE('',(#2389),#12963,.T.);
#13350=ADVANCED_FACE('',(#2390),#12964,.T.);
#13351=ADVANCED_FACE('',(#2391),#12965,.T.);
#13352=ADVANCED_FACE('',(#2392),#12966,.T.);
#13353=ADVANCED_FACE('',(#2393),#12967,.T.);
#13354=ADVANCED_FACE('',(#2394),#12968,.T.);
#13355=ADVANCED_FACE('',(#2395),#1777,.F.);
#13356=ADVANCED_FACE('',(#2396),#1008,.F.);
#13357=ADVANCED_FACE('',(#2397),#1778,.T.);
#13358=ADVANCED_FACE('',(#2398),#1009,.F.);
#13359=ADVANCED_FACE('',(#2399),#1004,.F.);
#13360=ADVANCED_FACE('',(#2400,#1561),#1779,.T.);
#13361=ADVANCED_FACE('',(#2401),#1097,.T.);
#13362=ADVANCED_FACE('',(#2402),#1780,.T.);
#13363=ADVANCED_FACE('',(#2403),#1781,.F.);
#13364=ADVANCED_FACE('',(#2404),#1782,.F.);
#13365=ADVANCED_FACE('',(#2405),#1783,.F.);
#13366=ADVANCED_FACE('',(#2406),#1098,.T.);
#13367=ADVANCED_FACE('',(#2407),#1784,.F.);
#13368=ADVANCED_FACE('',(#2408),#1785,.F.);
#13369=ADVANCED_FACE('',(#2409),#1786,.F.);
#13370=ADVANCED_FACE('',(#2410),#12969,.T.);
#13371=ADVANCED_FACE('',(#2411),#1787,.F.);
#13372=ADVANCED_FACE('',(#2412),#1788,.F.);
#13373=ADVANCED_FACE('',(#2413),#1789,.F.);
#13374=ADVANCED_FACE('',(#2414),#1790,.F.);
#13375=ADVANCED_FACE('',(#2415),#1791,.F.);
#13376=ADVANCED_FACE('',(#2416),#1792,.F.);
#13377=ADVANCED_FACE('',(#2417),#1793,.F.);
#13378=ADVANCED_FACE('',(#2418),#1794,.F.);
#13379=ADVANCED_FACE('',(#2419),#1795,.F.);
#13380=ADVANCED_FACE('',(#2420),#1796,.F.);
#13381=ADVANCED_FACE('',(#2421),#1797,.F.);
#13382=ADVANCED_FACE('',(#2422),#1798,.F.);
#13383=ADVANCED_FACE('',(#2423),#1799,.F.);
#13384=ADVANCED_FACE('',(#2424),#1800,.F.);
#13385=ADVANCED_FACE('',(#2425),#1801,.F.);
#13386=ADVANCED_FACE('',(#2426),#1802,.F.);
#13387=ADVANCED_FACE('',(#2427),#1803,.F.);
#13388=ADVANCED_FACE('',(#2428),#1804,.F.);
#13389=ADVANCED_FACE('',(#2429),#1805,.F.);
#13390=ADVANCED_FACE('',(#2430),#1806,.F.);
#13391=ADVANCED_FACE('',(#2431),#1807,.F.);
#13392=ADVANCED_FACE('',(#2432),#1808,.F.);
#13393=ADVANCED_FACE('',(#2433),#1809,.F.);
#13394=ADVANCED_FACE('',(#2434),#1810,.F.);
#13395=ADVANCED_FACE('',(#2435),#1811,.F.);
#13396=ADVANCED_FACE('',(#2436),#1812,.F.);
#13397=ADVANCED_FACE('',(#2437),#1813,.F.);
#13398=ADVANCED_FACE('',(#2438),#1814,.F.);
#13399=ADVANCED_FACE('',(#2439),#1815,.F.);
#13400=ADVANCED_FACE('',(#2440),#1816,.F.);
#13401=ADVANCED_FACE('',(#2441),#1817,.F.);
#13402=ADVANCED_FACE('',(#2442),#1818,.F.);
#13403=ADVANCED_FACE('',(#2443),#1819,.F.);
#13404=ADVANCED_FACE('',(#2444),#1820,.F.);
#13405=ADVANCED_FACE('',(#2445),#1821,.F.);
#13406=ADVANCED_FACE('',(#2446),#1822,.F.);
#13407=ADVANCED_FACE('',(#2447),#1823,.F.);
#13408=ADVANCED_FACE('',(#2448),#1824,.F.);
#13409=ADVANCED_FACE('',(#2449),#1825,.F.);
#13410=ADVANCED_FACE('',(#2450),#1826,.F.);
#13411=ADVANCED_FACE('',(#2451),#1827,.F.);
#13412=ADVANCED_FACE('',(#2452),#1828,.F.);
#13413=ADVANCED_FACE('',(#2453),#1829,.F.);
#13414=ADVANCED_FACE('',(#2454),#1830,.F.);
#13415=ADVANCED_FACE('',(#2455),#1831,.F.);
#13416=ADVANCED_FACE('',(#2456),#1832,.F.);
#13417=ADVANCED_FACE('',(#2457),#1833,.F.);
#13418=ADVANCED_FACE('',(#2458),#1834,.F.);
#13419=ADVANCED_FACE('',(#2459),#1835,.F.);
#13420=ADVANCED_FACE('',(#2460),#1836,.F.);
#13421=ADVANCED_FACE('',(#2461),#1837,.F.);
#13422=ADVANCED_FACE('',(#2462),#1838,.F.);
#13423=ADVANCED_FACE('',(#2463),#1839,.F.);
#13424=ADVANCED_FACE('',(#2464),#1840,.F.);
#13425=ADVANCED_FACE('',(#2465),#1841,.F.);
#13426=ADVANCED_FACE('',(#2466),#1842,.F.);
#13427=ADVANCED_FACE('',(#2467),#1843,.F.);
#13428=ADVANCED_FACE('',(#2468),#1844,.F.);
#13429=ADVANCED_FACE('',(#2469),#1845,.F.);
#13430=ADVANCED_FACE('',(#2470),#1846,.F.);
#13431=ADVANCED_FACE('',(#2471),#1847,.F.);
#13432=ADVANCED_FACE('',(#2472),#1848,.F.);
#13433=ADVANCED_FACE('',(#2473),#1849,.F.);
#13434=ADVANCED_FACE('',(#2474),#1850,.F.);
#13435=ADVANCED_FACE('',(#2475),#1851,.F.);
#13436=ADVANCED_FACE('',(#2476),#1852,.F.);
#13437=ADVANCED_FACE('',(#2477),#1853,.F.);
#13438=ADVANCED_FACE('',(#2478),#1854,.F.);
#13439=ADVANCED_FACE('',(#2479),#1855,.F.);
#13440=ADVANCED_FACE('',(#2480),#1856,.F.);
#13441=ADVANCED_FACE('',(#2481),#1857,.F.);
#13442=ADVANCED_FACE('',(#2482),#1858,.F.);
#13443=ADVANCED_FACE('',(#2483),#1859,.F.);
#13444=ADVANCED_FACE('',(#2484),#1860,.F.);
#13445=ADVANCED_FACE('',(#2485),#1861,.F.);
#13446=ADVANCED_FACE('',(#2486),#1862,.F.);
#13447=ADVANCED_FACE('',(#2487),#1863,.F.);
#13448=ADVANCED_FACE('',(#2488),#1864,.F.);
#13449=ADVANCED_FACE('',(#2489),#1865,.F.);
#13450=ADVANCED_FACE('',(#2490),#1866,.F.);
#13451=ADVANCED_FACE('',(#2491),#1867,.F.);
#13452=ADVANCED_FACE('',(#2492),#1868,.F.);
#13453=ADVANCED_FACE('',(#2493),#1869,.F.);
#13454=ADVANCED_FACE('',(#2494),#1870,.F.);
#13455=ADVANCED_FACE('',(#2495),#1871,.F.);
#13456=ADVANCED_FACE('',(#2496),#1872,.F.);
#13457=ADVANCED_FACE('',(#2497),#1873,.F.);
#13458=ADVANCED_FACE('',(#2498),#1874,.F.);
#13459=ADVANCED_FACE('',(#2499),#1875,.F.);
#13460=ADVANCED_FACE('',(#2500),#1876,.F.);
#13461=ADVANCED_FACE('',(#2501),#1877,.F.);
#13462=ADVANCED_FACE('',(#2502),#1878,.F.);
#13463=ADVANCED_FACE('',(#2503),#1879,.F.);
#13464=ADVANCED_FACE('',(#2504),#1880,.F.);
#13465=ADVANCED_FACE('',(#2505),#1881,.F.);
#13466=ADVANCED_FACE('',(#2506),#1882,.F.);
#13467=ADVANCED_FACE('',(#2507),#1883,.F.);
#13468=ADVANCED_FACE('',(#2508),#1884,.F.);
#13469=ADVANCED_FACE('',(#2509),#1885,.F.);
#13470=ADVANCED_FACE('',(#2510),#1886,.F.);
#13471=ADVANCED_FACE('',(#2511),#1887,.F.);
#13472=ADVANCED_FACE('',(#2512),#1888,.F.);
#13473=ADVANCED_FACE('',(#2513,#1562),#1889,.F.);
#13474=ADVANCED_FACE('',(#2514),#1890,.F.);
#13475=ADVANCED_FACE('',(#2515),#1891,.F.);
#13476=ADVANCED_FACE('',(#2516),#1892,.F.);
#13477=ADVANCED_FACE('',(#2517),#1893,.F.);
#13478=ADVANCED_FACE('',(#2518),#1894,.F.);
#13479=ADVANCED_FACE('',(#2519),#1895,.F.);
#13480=ADVANCED_FACE('',(#2520),#1099,.F.);
#13481=ADVANCED_FACE('',(#2521),#1896,.F.);
#13482=ADVANCED_FACE('',(#2522),#1897,.F.);
#13483=ADVANCED_FACE('',(#2523),#1898,.F.);
#13484=ADVANCED_FACE('',(#2524),#1899,.F.);
#13485=ADVANCED_FACE('',(#2525),#1900,.F.);
#13486=ADVANCED_FACE('',(#2526),#1901,.F.);
#13643=CLOSED_SHELL('',(#13326,#13327,#13328,#13329,#13330,#13331,#13332,
#13333,#13334,#13335,#13336,#13337,#13338,#13339,#13340,#13341,#13342,#13343,
#13344,#13345,#13346,#13347,#13348,#13349,#13350,#13351,#13352,#13353,#13354,
#13355,#13356,#13357,#13358,#13359,#13360,#13361,#13362,#13363,#13364,#13365,
#13366,#13367,#13368,#13369,#13370,#13371,#13372,#13373,#13374,#13375,#13376,
#13377,#13378,#13379,#13380,#13381,#13382,#13383,#13384,#13385,#13386,#13387,
#13388,#13389,#13390,#13391,#13392,#13393,#13394,#13395,#13396,#13397,#13398,
#13399,#13400,#13401,#13402,#13403,#13404,#13405,#13406,#13407,#13408,#13409,
#13410,#13411,#13412,#13413,#13414,#13415,#13416,#13417,#13418,#13419,#13420,
#13421,#13422,#13423,#13424,#13425,#13426,#13427,#13428,#13429,#13430,#13431,
#13432,#13433,#13434,#13435,#13436,#13437,#13438,#13439,#13440,#13441,#13442,
#13443,#13444,#13445,#13446,#13447,#13448,#13449,#13450,#13451,#13452,#13453,
#13454,#13455,#13456,#13457,#13458,#13459,#13460,#13461,#13462,#13463,#13464,
#13465,#13466,#13467,#13468,#13469,#13470,#13471,#13472,#13473,#13474,#13475,
#13476,#13477,#13478,#13479,#13480,#13481,#13482,#13483,#13484,#13485,#13486));
#14358=AXIS2_PLACEMENT_3D('',#37374,#16713,#16714);
#14359=AXIS2_PLACEMENT_3D('',#37375,#16715,#16716);
#14360=AXIS2_PLACEMENT_3D('',#37511,#16718,#16719);
#14361=AXIS2_PLACEMENT_3D('',#37597,#16720,#16721);
#14362=AXIS2_PLACEMENT_3D('',#38012,#16723,#16724);
#14363=AXIS2_PLACEMENT_3D('',#38448,#16726,#16727);
#14364=AXIS2_PLACEMENT_3D('',#38909,#16729,#16730);
#14365=AXIS2_PLACEMENT_3D('',#39448,#16732,#16733);
#14366=AXIS2_PLACEMENT_3D('',#39911,#16735,#16736);
#14367=AXIS2_PLACEMENT_3D('',#40414,#16738,#16739);
#14368=AXIS2_PLACEMENT_3D('',#40891,#16741,#16742);
#14369=AXIS2_PLACEMENT_3D('',#41350,#16744,#16745);
#14370=AXIS2_PLACEMENT_3D('',#41793,#16747,#16748);
#14371=AXIS2_PLACEMENT_3D('',#42252,#16750,#16751);
#14372=AXIS2_PLACEMENT_3D('',#42721,#16753,#16754);
#14373=AXIS2_PLACEMENT_3D('',#43178,#16756,#16757);
#14374=AXIS2_PLACEMENT_3D('',#43627,#16759,#16760);
#14375=AXIS2_PLACEMENT_3D('',#44090,#16762,#16763);
#14376=AXIS2_PLACEMENT_3D('',#44527,#16765,#16766);
#14377=AXIS2_PLACEMENT_3D('',#45008,#16768,#16769);
#14378=AXIS2_PLACEMENT_3D('',#45499,#16771,#16772);
#14379=AXIS2_PLACEMENT_3D('',#45944,#16774,#16775);
#14380=AXIS2_PLACEMENT_3D('',#46413,#16777,#16778);
#14381=AXIS2_PLACEMENT_3D('',#46839,#16780,#16781);
#14382=AXIS2_PLACEMENT_3D('',#47339,#16783,#16784);
#14383=AXIS2_PLACEMENT_3D('',#47791,#16786,#16787);
#14384=AXIS2_PLACEMENT_3D('',#48242,#16789,#16790);
#14385=AXIS2_PLACEMENT_3D('',#48694,#16792,#16793);
#14386=AXIS2_PLACEMENT_3D('',#49201,#16795,#16796);
#14387=AXIS2_PLACEMENT_3D('',#49635,#16798,#16799);
#14388=AXIS2_PLACEMENT_3D('',#49706,#16800,#16801);
#14389=AXIS2_PLACEMENT_3D('',#53294,#16802,#16803);
#14390=AXIS2_PLACEMENT_3D('',#53296,#16804,#16805);
#14391=AXIS2_PLACEMENT_3D('',#56848,#16806,#16807);
#14392=AXIS2_PLACEMENT_3D('',#57010,#16808,#16809);
#14393=AXIS2_PLACEMENT_3D('',#57139,#16810,#16811);
#14394=AXIS2_PLACEMENT_3D('',#57141,#16812,#16813);
#14395=AXIS2_PLACEMENT_3D('',#58094,#16814,#16815);
#14396=AXIS2_PLACEMENT_3D('',#58097,#16816,#16817);
#14397=AXIS2_PLACEMENT_3D('',#58180,#16818,#16819);
#14398=AXIS2_PLACEMENT_3D('',#58893,#16820,#16821);
#14399=AXIS2_PLACEMENT_3D('',#58895,#16822,#16823);
#14400=AXIS2_PLACEMENT_3D('',#58896,#16824,#16825);
#14401=AXIS2_PLACEMENT_3D('',#58897,#16826,#16827);
#14402=AXIS2_PLACEMENT_3D('',#58899,#16828,#16829);
#14403=AXIS2_PLACEMENT_3D('',#58900,#16830,#16831);
#14404=AXIS2_PLACEMENT_3D('',#58903,#16833,#16834);
#14405=AXIS2_PLACEMENT_3D('',#58904,#16835,#16836);
#14406=AXIS2_PLACEMENT_3D('',#58905,#16837,#16838);
#14407=AXIS2_PLACEMENT_3D('',#58916,#16842,#16843);
#14408=AXIS2_PLACEMENT_3D('',#58924,#16846,#16847);
#14409=AXIS2_PLACEMENT_3D('',#58925,#16848,#16849);
#14410=AXIS2_PLACEMENT_3D('',#58926,#16850,#16851);
#14411=AXIS2_PLACEMENT_3D('',#58933,#16852,#16853);
#14412=AXIS2_PLACEMENT_3D('',#58943,#16854,#16855);
#14413=AXIS2_PLACEMENT_3D('',#58953,#16856,#16857);
#14414=AXIS2_PLACEMENT_3D('',#58963,#16858,#16859);
#14415=AXIS2_PLACEMENT_3D('',#58973,#16860,#16861);
#14416=AXIS2_PLACEMENT_3D('',#58983,#16862,#16863);
#14417=AXIS2_PLACEMENT_3D('',#58993,#16864,#16865);
#14418=AXIS2_PLACEMENT_3D('',#59003,#16866,#16867);
#14419=AXIS2_PLACEMENT_3D('',#59013,#16868,#16869);
#14420=AXIS2_PLACEMENT_3D('',#59023,#16870,#16871);
#14421=AXIS2_PLACEMENT_3D('',#59033,#16872,#16873);
#14422=AXIS2_PLACEMENT_3D('',#59043,#16874,#16875);
#14423=AXIS2_PLACEMENT_3D('',#59053,#16876,#16877);
#14424=AXIS2_PLACEMENT_3D('',#59063,#16878,#16879);
#14425=AXIS2_PLACEMENT_3D('',#59073,#16880,#16881);
#14426=AXIS2_PLACEMENT_3D('',#59083,#16882,#16883);
#14427=AXIS2_PLACEMENT_3D('',#59093,#16884,#16885);
#14428=AXIS2_PLACEMENT_3D('',#59103,#16886,#16887);
#14429=AXIS2_PLACEMENT_3D('',#59112,#16888,#16889);
#14430=AXIS2_PLACEMENT_3D('',#59114,#16890,#16891);
#14431=AXIS2_PLACEMENT_3D('',#59124,#16892,#16893);
#14432=AXIS2_PLACEMENT_3D('',#59134,#16894,#16895);
#14433=AXIS2_PLACEMENT_3D('',#59144,#16896,#16897);
#14434=AXIS2_PLACEMENT_3D('',#59154,#16898,#16899);
#14435=AXIS2_PLACEMENT_3D('',#59164,#16900,#16901);
#14436=AXIS2_PLACEMENT_3D('',#59174,#16902,#16903);
#14437=AXIS2_PLACEMENT_3D('',#59184,#16904,#16905);
#14438=AXIS2_PLACEMENT_3D('',#59194,#16906,#16907);
#14439=AXIS2_PLACEMENT_3D('',#59204,#16908,#16909);
#14440=AXIS2_PLACEMENT_3D('',#59214,#16910,#16911);
#14441=AXIS2_PLACEMENT_3D('',#59224,#16912,#16913);
#14442=AXIS2_PLACEMENT_3D('',#59234,#16914,#16915);
#14443=AXIS2_PLACEMENT_3D('',#59244,#16916,#16917);
#14444=AXIS2_PLACEMENT_3D('',#59254,#16918,#16919);
#14445=AXIS2_PLACEMENT_3D('',#59264,#16920,#16921);
#14446=AXIS2_PLACEMENT_3D('',#59274,#16922,#16923);
#14447=AXIS2_PLACEMENT_3D('',#59280,#16925,#16926);
#14448=AXIS2_PLACEMENT_3D('',#59281,#16927,#16928);
#14449=AXIS2_PLACEMENT_3D('',#59284,#16929,#16930);
#14450=AXIS2_PLACEMENT_3D('',#59288,#16933,#16934);
#14451=AXIS2_PLACEMENT_3D('',#59291,#16937,#16938);
#14452=AXIS2_PLACEMENT_3D('',#59293,#16940,#16941);
#14453=AXIS2_PLACEMENT_3D('',#59296,#16942,#16943);
#14454=AXIS2_PLACEMENT_3D('',#59299,#16945,#16946);
#14455=AXIS2_PLACEMENT_3D('',#59304,#16949,#16950);
#14456=AXIS2_PLACEMENT_3D('',#59309,#16953,#16954);
#14457=AXIS2_PLACEMENT_3D('',#59314,#16957,#16958);
#14458=AXIS2_PLACEMENT_3D('',#59319,#16961,#16962);
#14459=AXIS2_PLACEMENT_3D('',#59324,#16965,#16966);
#14460=AXIS2_PLACEMENT_3D('',#59329,#16969,#16970);
#14461=AXIS2_PLACEMENT_3D('',#59334,#16973,#16974);
#14462=AXIS2_PLACEMENT_3D('',#59339,#16977,#16978);
#14463=AXIS2_PLACEMENT_3D('',#59344,#16981,#16982);
#14464=AXIS2_PLACEMENT_3D('',#59349,#16985,#16986);
#14465=AXIS2_PLACEMENT_3D('',#59354,#16989,#16990);
#14466=AXIS2_PLACEMENT_3D('',#59359,#16993,#16994);
#14467=AXIS2_PLACEMENT_3D('',#59364,#16997,#16998);
#14468=AXIS2_PLACEMENT_3D('',#59369,#17001,#17002);
#14469=AXIS2_PLACEMENT_3D('',#59374,#17005,#17006);
#14470=AXIS2_PLACEMENT_3D('',#59379,#17009,#17010);
#14471=AXIS2_PLACEMENT_3D('',#59384,#17013,#17014);
#14472=AXIS2_PLACEMENT_3D('',#59389,#17017,#17018);
#14473=AXIS2_PLACEMENT_3D('',#59394,#17021,#17022);
#14474=AXIS2_PLACEMENT_3D('',#59399,#17025,#17026);
#14475=AXIS2_PLACEMENT_3D('',#59404,#17029,#17030);
#14476=AXIS2_PLACEMENT_3D('',#59409,#17033,#17034);
#14477=AXIS2_PLACEMENT_3D('',#59414,#17037,#17038);
#14478=AXIS2_PLACEMENT_3D('',#59419,#17041,#17042);
#14479=AXIS2_PLACEMENT_3D('',#59424,#17045,#17046);
#14480=AXIS2_PLACEMENT_3D('',#59429,#17049,#17050);
#14481=AXIS2_PLACEMENT_3D('',#59434,#17053,#17054);
#14482=AXIS2_PLACEMENT_3D('',#59439,#17057,#17058);
#14483=AXIS2_PLACEMENT_3D('',#59444,#17061,#17062);
#14484=AXIS2_PLACEMENT_3D('',#59449,#17065,#17066);
#14485=AXIS2_PLACEMENT_3D('',#59454,#17069,#17070);
#14486=AXIS2_PLACEMENT_3D('',#59459,#17073,#17074);
#14487=AXIS2_PLACEMENT_3D('',#59464,#17077,#17078);
#14488=AXIS2_PLACEMENT_3D('',#59467,#17081,#17082);
#14489=AXIS2_PLACEMENT_3D('',#59471,#17085,#17086);
#14490=AXIS2_PLACEMENT_3D('',#59473,#17088,#17089);
#14491=AXIS2_PLACEMENT_3D('',#59474,#17090,#17091);
#14492=AXIS2_PLACEMENT_3D('',#59478,#17094,#17095);
#14493=AXIS2_PLACEMENT_3D('',#59480,#17097,#17098);
#14494=AXIS2_PLACEMENT_3D('',#59481,#17099,#17100);
#14495=AXIS2_PLACEMENT_3D('',#59485,#17103,#17104);
#14496=AXIS2_PLACEMENT_3D('',#59487,#17106,#17107);
#14497=AXIS2_PLACEMENT_3D('',#59488,#17108,#17109);
#14498=AXIS2_PLACEMENT_3D('',#59492,#17112,#17113);
#14499=AXIS2_PLACEMENT_3D('',#59494,#17115,#17116);
#14500=AXIS2_PLACEMENT_3D('',#59495,#17117,#17118);
#14501=AXIS2_PLACEMENT_3D('',#59499,#17121,#17122);
#14502=AXIS2_PLACEMENT_3D('',#59501,#17124,#17125);
#14503=AXIS2_PLACEMENT_3D('',#59502,#17126,#17127);
#14504=AXIS2_PLACEMENT_3D('',#59506,#17130,#17131);
#14505=AXIS2_PLACEMENT_3D('',#59508,#17133,#17134);
#14506=AXIS2_PLACEMENT_3D('',#59509,#17135,#17136);
#14507=AXIS2_PLACEMENT_3D('',#59513,#17139,#17140);
#14508=AXIS2_PLACEMENT_3D('',#59515,#17142,#17143);
#14509=AXIS2_PLACEMENT_3D('',#59516,#17144,#17145);
#14510=AXIS2_PLACEMENT_3D('',#59520,#17148,#17149);
#14511=AXIS2_PLACEMENT_3D('',#59522,#17151,#17152);
#14512=AXIS2_PLACEMENT_3D('',#59523,#17153,#17154);
#14513=AXIS2_PLACEMENT_3D('',#59527,#17157,#17158);
#14514=AXIS2_PLACEMENT_3D('',#59529,#17160,#17161);
#14515=AXIS2_PLACEMENT_3D('',#59530,#17162,#17163);
#14516=AXIS2_PLACEMENT_3D('',#59534,#17166,#17167);
#14517=AXIS2_PLACEMENT_3D('',#59536,#17169,#17170);
#14518=AXIS2_PLACEMENT_3D('',#59537,#17171,#17172);
#14519=AXIS2_PLACEMENT_3D('',#59541,#17175,#17176);
#14520=AXIS2_PLACEMENT_3D('',#59543,#17178,#17179);
#14521=AXIS2_PLACEMENT_3D('',#59544,#17180,#17181);
#14522=AXIS2_PLACEMENT_3D('',#59548,#17184,#17185);
#14523=AXIS2_PLACEMENT_3D('',#59550,#17187,#17188);
#14524=AXIS2_PLACEMENT_3D('',#59551,#17189,#17190);
#14525=AXIS2_PLACEMENT_3D('',#59555,#17193,#17194);
#14526=AXIS2_PLACEMENT_3D('',#59557,#17196,#17197);
#14527=AXIS2_PLACEMENT_3D('',#59558,#17198,#17199);
#14528=AXIS2_PLACEMENT_3D('',#59562,#17202,#17203);
#14529=AXIS2_PLACEMENT_3D('',#59564,#17205,#17206);
#14530=AXIS2_PLACEMENT_3D('',#59565,#17207,#17208);
#14531=AXIS2_PLACEMENT_3D('',#59569,#17211,#17212);
#14532=AXIS2_PLACEMENT_3D('',#59571,#17214,#17215);
#14533=AXIS2_PLACEMENT_3D('',#59572,#17216,#17217);
#14534=AXIS2_PLACEMENT_3D('',#59576,#17220,#17221);
#14535=AXIS2_PLACEMENT_3D('',#59578,#17223,#17224);
#14536=AXIS2_PLACEMENT_3D('',#59579,#17225,#17226);
#14537=AXIS2_PLACEMENT_3D('',#59583,#17229,#17230);
#14538=AXIS2_PLACEMENT_3D('',#59585,#17232,#17233);
#14539=AXIS2_PLACEMENT_3D('',#59586,#17234,#17235);
#14540=AXIS2_PLACEMENT_3D('',#59590,#17238,#17239);
#14541=AXIS2_PLACEMENT_3D('',#59592,#17241,#17242);
#14542=AXIS2_PLACEMENT_3D('',#59593,#17243,#17244);
#14543=AXIS2_PLACEMENT_3D('',#59597,#17247,#17248);
#14544=AXIS2_PLACEMENT_3D('',#59599,#17250,#17251);
#14545=AXIS2_PLACEMENT_3D('',#59600,#17252,#17253);
#14546=AXIS2_PLACEMENT_3D('',#59604,#17256,#17257);
#14547=AXIS2_PLACEMENT_3D('',#59606,#17259,#17260);
#14548=AXIS2_PLACEMENT_3D('',#59607,#17261,#17262);
#14549=AXIS2_PLACEMENT_3D('',#59611,#17265,#17266);
#14550=AXIS2_PLACEMENT_3D('',#59613,#17268,#17269);
#14551=AXIS2_PLACEMENT_3D('',#59614,#17270,#17271);
#14552=AXIS2_PLACEMENT_3D('',#59618,#17274,#17275);
#14553=AXIS2_PLACEMENT_3D('',#59620,#17277,#17278);
#14554=AXIS2_PLACEMENT_3D('',#59621,#17279,#17280);
#14555=AXIS2_PLACEMENT_3D('',#59625,#17283,#17284);
#14556=AXIS2_PLACEMENT_3D('',#59627,#17286,#17287);
#14557=AXIS2_PLACEMENT_3D('',#59628,#17288,#17289);
#14558=AXIS2_PLACEMENT_3D('',#59632,#17292,#17293);
#14559=AXIS2_PLACEMENT_3D('',#59634,#17295,#17296);
#14560=AXIS2_PLACEMENT_3D('',#59635,#17297,#17298);
#14561=AXIS2_PLACEMENT_3D('',#59639,#17301,#17302);
#14562=AXIS2_PLACEMENT_3D('',#59641,#17304,#17305);
#14563=AXIS2_PLACEMENT_3D('',#59642,#17306,#17307);
#14564=AXIS2_PLACEMENT_3D('',#59646,#17310,#17311);
#14565=AXIS2_PLACEMENT_3D('',#59648,#17313,#17314);
#14566=AXIS2_PLACEMENT_3D('',#59649,#17315,#17316);
#14567=AXIS2_PLACEMENT_3D('',#59653,#17319,#17320);
#14568=AXIS2_PLACEMENT_3D('',#59655,#17322,#17323);
#14569=AXIS2_PLACEMENT_3D('',#59656,#17324,#17325);
#14570=AXIS2_PLACEMENT_3D('',#59660,#17328,#17329);
#14571=AXIS2_PLACEMENT_3D('',#59662,#17331,#17332);
#14572=AXIS2_PLACEMENT_3D('',#59663,#17333,#17334);
#14573=AXIS2_PLACEMENT_3D('',#59667,#17337,#17338);
#14574=AXIS2_PLACEMENT_3D('',#59669,#17340,#17341);
#14575=AXIS2_PLACEMENT_3D('',#59670,#17342,#17343);
#14576=AXIS2_PLACEMENT_3D('',#59674,#17346,#17347);
#14577=AXIS2_PLACEMENT_3D('',#59676,#17349,#17350);
#14578=AXIS2_PLACEMENT_3D('',#59677,#17351,#17352);
#14579=AXIS2_PLACEMENT_3D('',#59681,#17355,#17356);
#14580=AXIS2_PLACEMENT_3D('',#59683,#17358,#17359);
#14581=AXIS2_PLACEMENT_3D('',#59684,#17360,#17361);
#14582=AXIS2_PLACEMENT_3D('',#59688,#17364,#17365);
#14583=AXIS2_PLACEMENT_3D('',#59690,#17367,#17368);
#14584=AXIS2_PLACEMENT_3D('',#59691,#17369,#17370);
#14585=AXIS2_PLACEMENT_3D('',#59695,#17373,#17374);
#14586=AXIS2_PLACEMENT_3D('',#59697,#17376,#17377);
#14587=AXIS2_PLACEMENT_3D('',#59698,#17378,#17379);
#14588=AXIS2_PLACEMENT_3D('',#59702,#17382,#17383);
#14589=AXIS2_PLACEMENT_3D('',#59704,#17385,#17386);
#14590=AXIS2_PLACEMENT_3D('',#59705,#17387,#17388);
#14591=AXIS2_PLACEMENT_3D('',#59718,#17395,#17396);
#14592=AXIS2_PLACEMENT_3D('',#59722,#17398,#17399);
#14593=AXIS2_PLACEMENT_3D('',#59723,#17400,#17401);
#14594=AXIS2_PLACEMENT_3D('',#59726,#17403,#17404);
#14595=AXIS2_PLACEMENT_3D('',#59727,#17405,#17406);
#14596=AXIS2_PLACEMENT_3D('',#59730,#17408,#17409);
#14597=AXIS2_PLACEMENT_3D('',#59731,#17410,#17411);
#14598=AXIS2_PLACEMENT_3D('',#59734,#17413,#17414);
#14599=AXIS2_PLACEMENT_3D('',#59735,#17415,#17416);
#14600=AXIS2_PLACEMENT_3D('',#59738,#17418,#17419);
#14601=AXIS2_PLACEMENT_3D('',#59739,#17420,#17421);
#14602=AXIS2_PLACEMENT_3D('',#59741,#17423,#17424);
#14603=AXIS2_PLACEMENT_3D('',#59742,#17425,#17426);
#14604=AXIS2_PLACEMENT_3D('',#59745,#17428,#17429);
#14605=AXIS2_PLACEMENT_3D('',#59748,#17432,#17433);
#14606=AXIS2_PLACEMENT_3D('',#59750,#17435,#17436);
#14607=AXIS2_PLACEMENT_3D('',#59752,#17438,#17439);
#14608=AXIS2_PLACEMENT_3D('',#59754,#17441,#17442);
#14609=AXIS2_PLACEMENT_3D('',#59756,#17444,#17445);
#16713=DIRECTION('axis',(0.,0.,1.));
#16714=DIRECTION('refdir',(1.,0.,0.));
#16715=DIRECTION('center_axis',(0.,1.,0.));
#16716=DIRECTION('ref_axis',(0.314077325660087,0.,0.949397405466335));
#16717=DIRECTION('',(0.,-1.,0.));
#16718=DIRECTION('center_axis',(0.,-1.,0.));
#16719=DIRECTION('ref_axis',(1.,0.,9.89867765446222E-14));
#16720=DIRECTION('center_axis',(0.,1.,0.));
#16721=DIRECTION('ref_axis',(0.314077325660087,0.,0.949397405466335));
#16722=DIRECTION('',(0.,-1.,0.));
#16723=DIRECTION('center_axis',(0.,1.,0.));
#16724=DIRECTION('ref_axis',(0.314077325660087,0.,0.949397405466335));
#16725=DIRECTION('',(0.,-1.,0.));
#16726=DIRECTION('center_axis',(0.,1.,0.));
#16727=DIRECTION('ref_axis',(0.314077325660087,0.,0.949397405466335));
#16728=DIRECTION('',(0.,-1.,0.));
#16729=DIRECTION('center_axis',(0.,1.,0.));
#16730=DIRECTION('ref_axis',(0.314077325660087,0.,0.949397405466335));
#16731=DIRECTION('',(0.,-1.,0.));
#16732=DIRECTION('center_axis',(0.,1.,0.));
#16733=DIRECTION('ref_axis',(0.314077325660087,0.,0.949397405466335));
#16734=DIRECTION('',(0.,-1.,0.));
#16735=DIRECTION('center_axis',(0.,1.,0.));
#16736=DIRECTION('ref_axis',(0.314077325660087,0.,0.949397405466335));
#16737=DIRECTION('',(0.,-1.,0.));
#16738=DIRECTION('center_axis',(0.,1.,0.));
#16739=DIRECTION('ref_axis',(0.314077325660087,0.,0.949397405466335));
#16740=DIRECTION('',(0.,-1.,0.));
#16741=DIRECTION('center_axis',(0.,1.,0.));
#16742=DIRECTION('ref_axis',(0.314077325660087,0.,0.949397405466335));
#16743=DIRECTION('',(0.,-1.,0.));
#16744=DIRECTION('center_axis',(0.,1.,0.));
#16745=DIRECTION('ref_axis',(0.314077325660087,0.,0.949397405466335));
#16746=DIRECTION('',(0.,-1.,0.));
#16747=DIRECTION('center_axis',(0.,1.,0.));
#16748=DIRECTION('ref_axis',(0.314077325660087,0.,0.949397405466335));
#16749=DIRECTION('',(0.,-1.,0.));
#16750=DIRECTION('center_axis',(0.,1.,0.));
#16751=DIRECTION('ref_axis',(0.314077325660087,0.,0.949397405466335));
#16752=DIRECTION('',(0.,-1.,0.));
#16753=DIRECTION('center_axis',(0.,1.,0.));
#16754=DIRECTION('ref_axis',(0.314077325660087,0.,0.949397405466335));
#16755=DIRECTION('',(0.,-1.,0.));
#16756=DIRECTION('center_axis',(0.,1.,0.));
#16757=DIRECTION('ref_axis',(0.314077325660087,0.,0.949397405466335));
#16758=DIRECTION('',(0.,-1.,0.));
#16759=DIRECTION('center_axis',(0.,1.,0.));
#16760=DIRECTION('ref_axis',(0.314077325660087,0.,0.949397405466335));
#16761=DIRECTION('',(0.,-1.,0.));
#16762=DIRECTION('center_axis',(0.,1.,0.));
#16763=DIRECTION('ref_axis',(0.314077325660087,0.,0.949397405466335));
#16764=DIRECTION('',(0.,-1.,0.));
#16765=DIRECTION('center_axis',(0.,1.,0.));
#16766=DIRECTION('ref_axis',(0.314077325660087,0.,0.949397405466335));
#16767=DIRECTION('',(0.,-1.,0.));
#16768=DIRECTION('center_axis',(0.,1.,0.));
#16769=DIRECTION('ref_axis',(0.314077325660087,0.,0.949397405466335));
#16770=DIRECTION('',(0.,-1.,0.));
#16771=DIRECTION('center_axis',(0.,1.,0.));
#16772=DIRECTION('ref_axis',(0.314077325660087,0.,0.949397405466335));
#16773=DIRECTION('',(0.,-1.,0.));
#16774=DIRECTION('center_axis',(0.,1.,0.));
#16775=DIRECTION('ref_axis',(0.314077325660087,0.,0.949397405466335));
#16776=DIRECTION('',(0.,-1.,0.));
#16777=DIRECTION('center_axis',(0.,1.,0.));
#16778=DIRECTION('ref_axis',(0.314077325660087,0.,0.949397405466335));
#16779=DIRECTION('',(0.,-1.,0.));
#16780=DIRECTION('center_axis',(0.,1.,0.));
#16781=DIRECTION('ref_axis',(0.314077325660087,0.,0.949397405466335));
#16782=DIRECTION('',(0.,-1.,0.));
#16783=DIRECTION('center_axis',(0.,1.,0.));
#16784=DIRECTION('ref_axis',(0.314077325660087,0.,0.949397405466335));
#16785=DIRECTION('',(0.,-1.,0.));
#16786=DIRECTION('center_axis',(0.,1.,0.));
#16787=DIRECTION('ref_axis',(0.314077325660087,0.,0.949397405466335));
#16788=DIRECTION('',(0.,-1.,0.));
#16789=DIRECTION('center_axis',(0.,1.,0.));
#16790=DIRECTION('ref_axis',(0.314077325660087,0.,0.949397405466335));
#16791=DIRECTION('',(0.,-1.,0.));
#16792=DIRECTION('center_axis',(0.,1.,0.));
#16793=DIRECTION('ref_axis',(0.314077325660087,0.,0.949397405466335));
#16794=DIRECTION('',(0.,-1.,0.));
#16795=DIRECTION('center_axis',(0.,1.,0.));
#16796=DIRECTION('ref_axis',(0.314077325660087,0.,0.949397405466335));
#16797=DIRECTION('',(0.,-1.,0.));
#16798=DIRECTION('center_axis',(0.,1.,0.));
#16799=DIRECTION('ref_axis',(1.,0.,0.));
#16800=DIRECTION('center_axis',(0.,-1.,0.));
#16801=DIRECTION('ref_axis',(1.,0.,0.));
#16802=DIRECTION('center_axis',(0.,1.,0.));
#16803=DIRECTION('ref_axis',(1.,0.,0.));
#16804=DIRECTION('center_axis',(0.,1.,0.));
#16805=DIRECTION('ref_axis',(1.,0.,0.));
#16806=DIRECTION('center_axis',(0.,1.,0.));
#16807=DIRECTION('ref_axis',(0.314077325660087,0.,0.949397405466335));
#16808=DIRECTION('center_axis',(0.,1.,0.));
#16809=DIRECTION('ref_axis',(1.,0.,9.89867765446222E-14));
#16810=DIRECTION('center_axis',(0.,1.,0.));
#16811=DIRECTION('ref_axis',(0.,0.,1.));
#16812=DIRECTION('center_axis',(0.,1.,0.));
#16813=DIRECTION('ref_axis',(1.,0.,0.));
#16814=DIRECTION('center_axis',(0.,1.,0.));
#16815=DIRECTION('ref_axis',(0.,0.,1.));
#16816=DIRECTION('center_axis',(0.,-1.,0.));
#16817=DIRECTION('ref_axis',(1.,0.,0.));
#16818=DIRECTION('center_axis',(0.,-1.,0.));
#16819=DIRECTION('ref_axis',(1.,0.,0.));
#16820=DIRECTION('center_axis',(0.,-1.,0.));
#16821=DIRECTION('ref_axis',(0.,0.,-1.));
#16822=DIRECTION('center_axis',(0.,1.,0.));
#16823=DIRECTION('ref_axis',(1.,0.,0.));
#16824=DIRECTION('center_axis',(1.,0.,0.));
#16825=DIRECTION('ref_axis',(0.,0.,1.));
#16826=DIRECTION('center_axis',(0.,1.,0.));
#16827=DIRECTION('ref_axis',(1.,0.,0.));
#16828=DIRECTION('center_axis',(0.,1.,0.));
#16829=DIRECTION('ref_axis',(1.,0.,0.));
#16830=DIRECTION('center_axis',(0.,-1.,0.));
#16831=DIRECTION('ref_axis',(1.,0.,0.));
#16832=DIRECTION('',(0.707106781186547,0.707106781186548,8.65956056235493E-17));
#16833=DIRECTION('center_axis',(0.,-1.,0.));
#16834=DIRECTION('ref_axis',(1.,0.,0.));
#16835=DIRECTION('center_axis',(0.,1.,0.));
#16836=DIRECTION('ref_axis',(1.,0.,0.));
#16837=DIRECTION('center_axis',(-0.241286600017026,0.,-0.970453902383943));
#16838=DIRECTION('ref_axis',(-0.970453902383943,0.,0.241286600017026));
#16839=DIRECTION('',(0.,-1.,0.));
#16840=DIRECTION('',(-0.970453902383943,0.,0.241286600017026));
#16841=DIRECTION('',(0.,1.,0.));
#16842=DIRECTION('center_axis',(-0.558650020314825,0.,0.829403493362697));
#16843=DIRECTION('ref_axis',(0.829403493362697,0.,0.558650020314825));
#16844=DIRECTION('',(0.829403493362697,0.,0.558650020314825));
#16845=DIRECTION('',(0.,1.,0.));
#16846=DIRECTION('center_axis',(0.,1.,0.));
#16847=DIRECTION('ref_axis',(-0.17364817766693,0.,0.984807753012208));
#16848=DIRECTION('center_axis',(0.,1.,0.));
#16849=DIRECTION('ref_axis',(1.,0.,0.));
#16850=DIRECTION('center_axis',(0.,1.,0.));
#16851=DIRECTION('ref_axis',(1.,0.,0.));
#16852=DIRECTION('center_axis',(0.,-1.,0.));
#16853=DIRECTION('ref_axis',(1.,0.,0.));
#16854=DIRECTION('center_axis',(0.,-1.,0.));
#16855=DIRECTION('ref_axis',(1.,0.,0.));
#16856=DIRECTION('center_axis',(0.,-1.,0.));
#16857=DIRECTION('ref_axis',(1.,0.,0.));
#16858=DIRECTION('center_axis',(0.,-1.,0.));
#16859=DIRECTION('ref_axis',(1.,0.,0.));
#16860=DIRECTION('center_axis',(0.,-1.,0.));
#16861=DIRECTION('ref_axis',(1.,0.,0.));
#16862=DIRECTION('center_axis',(0.,-1.,0.));
#16863=DIRECTION('ref_axis',(1.,0.,0.));
#16864=DIRECTION('center_axis',(0.,-1.,0.));
#16865=DIRECTION('ref_axis',(1.,0.,0.));
#16866=DIRECTION('center_axis',(0.,-1.,0.));
#16867=DIRECTION('ref_axis',(1.,0.,0.));
#16868=DIRECTION('center_axis',(0.,-1.,0.));
#16869=DIRECTION('ref_axis',(1.,0.,0.));
#16870=DIRECTION('center_axis',(0.,-1.,0.));
#16871=DIRECTION('ref_axis',(1.,0.,0.));
#16872=DIRECTION('center_axis',(0.,-1.,0.));
#16873=DIRECTION('ref_axis',(1.,0.,0.));
#16874=DIRECTION('center_axis',(0.,-1.,0.));
#16875=DIRECTION('ref_axis',(1.,0.,0.));
#16876=DIRECTION('center_axis',(0.,-1.,0.));
#16877=DIRECTION('ref_axis',(1.,0.,0.));
#16878=DIRECTION('center_axis',(0.,-1.,0.));
#16879=DIRECTION('ref_axis',(1.,0.,0.));
#16880=DIRECTION('center_axis',(0.,-1.,0.));
#16881=DIRECTION('ref_axis',(1.,0.,0.));
#16882=DIRECTION('center_axis',(0.,-1.,0.));
#16883=DIRECTION('ref_axis',(1.,0.,0.));
#16884=DIRECTION('center_axis',(0.,-1.,0.));
#16885=DIRECTION('ref_axis',(1.,0.,0.));
#16886=DIRECTION('center_axis',(0.,-1.,0.));
#16887=DIRECTION('ref_axis',(1.,0.,0.));
#16888=DIRECTION('center_axis',(0.,-1.,0.));
#16889=DIRECTION('ref_axis',(1.,0.,0.));
#16890=DIRECTION('center_axis',(0.,-1.,0.));
#16891=DIRECTION('ref_axis',(1.,0.,0.));
#16892=DIRECTION('center_axis',(0.,-1.,0.));
#16893=DIRECTION('ref_axis',(1.,0.,0.));
#16894=DIRECTION('center_axis',(0.,-1.,0.));
#16895=DIRECTION('ref_axis',(1.,0.,0.));
#16896=DIRECTION('center_axis',(0.,-1.,0.));
#16897=DIRECTION('ref_axis',(1.,0.,0.));
#16898=DIRECTION('center_axis',(0.,-1.,0.));
#16899=DIRECTION('ref_axis',(1.,0.,0.));
#16900=DIRECTION('center_axis',(0.,-1.,0.));
#16901=DIRECTION('ref_axis',(1.,0.,0.));
#16902=DIRECTION('center_axis',(0.,-1.,0.));
#16903=DIRECTION('ref_axis',(1.,0.,0.));
#16904=DIRECTION('center_axis',(0.,-1.,0.));
#16905=DIRECTION('ref_axis',(1.,0.,0.));
#16906=DIRECTION('center_axis',(0.,-1.,0.));
#16907=DIRECTION('ref_axis',(1.,0.,0.));
#16908=DIRECTION('center_axis',(0.,-1.,0.));
#16909=DIRECTION('ref_axis',(1.,0.,0.));
#16910=DIRECTION('center_axis',(0.,-1.,0.));
#16911=DIRECTION('ref_axis',(1.,0.,0.));
#16912=DIRECTION('center_axis',(0.,-1.,0.));
#16913=DIRECTION('ref_axis',(1.,0.,0.));
#16914=DIRECTION('center_axis',(0.,-1.,0.));
#16915=DIRECTION('ref_axis',(1.,0.,0.));
#16916=DIRECTION('center_axis',(0.,-1.,0.));
#16917=DIRECTION('ref_axis',(1.,0.,0.));
#16918=DIRECTION('center_axis',(0.,-1.,0.));
#16919=DIRECTION('ref_axis',(1.,0.,0.));
#16920=DIRECTION('center_axis',(0.,-1.,0.));
#16921=DIRECTION('ref_axis',(1.,0.,0.));
#16922=DIRECTION('center_axis',(0.,-1.,0.));
#16923=DIRECTION('ref_axis',(1.,0.,0.));
#16924=DIRECTION('',(0.707106781186547,-0.707106781186548,-8.65956056235493E-17));
#16925=DIRECTION('center_axis',(0.,1.,0.));
#16926=DIRECTION('ref_axis',(1.,0.,0.));
#16927=DIRECTION('center_axis',(0.,1.,0.));
#16928=DIRECTION('ref_axis',(-0.342020143325669,0.,0.939692620785908));
#16929=DIRECTION('center_axis',(0.,1.,0.));
#16930=DIRECTION('ref_axis',(1.,0.,0.));
#16931=DIRECTION('',(0.71979443265773,0.,0.694187276399486));
#16932=DIRECTION('',(-0.997609505397066,0.,0.0691033627359896));
#16933=DIRECTION('center_axis',(-0.0691033627359896,0.,-0.997609505397066));
#16934=DIRECTION('ref_axis',(-0.997609505397066,0.,0.0691033627359896));
#16935=DIRECTION('',(0.,-1.,0.));
#16936=DIRECTION('',(0.,1.,0.));
#16937=DIRECTION('center_axis',(-0.694187276399486,0.,0.71979443265773));
#16938=DIRECTION('ref_axis',(0.71979443265773,0.,0.694187276399486));
#16939=DIRECTION('',(0.,1.,0.));
#16940=DIRECTION('center_axis',(0.,-1.,0.));
#16941=DIRECTION('ref_axis',(1.,0.,0.));
#16942=DIRECTION('center_axis',(0.,1.,0.));
#16943=DIRECTION('ref_axis',(1.,0.,0.));
#16944=DIRECTION('',(0.,1.,0.));
#16945=DIRECTION('center_axis',(0.,1.,0.));
#16946=DIRECTION('ref_axis',(1.,0.,0.));
#16947=DIRECTION('',(0.,-1.,0.));
#16948=DIRECTION('',(0.,1.,0.));
#16949=DIRECTION('center_axis',(0.,1.,0.));
#16950=DIRECTION('ref_axis',(1.,0.,0.));
#16951=DIRECTION('',(0.,-1.,0.));
#16952=DIRECTION('',(0.,1.,0.));
#16953=DIRECTION('center_axis',(0.,1.,0.));
#16954=DIRECTION('ref_axis',(1.,0.,0.));
#16955=DIRECTION('',(0.,-1.,0.));
#16956=DIRECTION('',(0.,1.,0.));
#16957=DIRECTION('center_axis',(0.,1.,0.));
#16958=DIRECTION('ref_axis',(1.,0.,0.));
#16959=DIRECTION('',(0.,-1.,0.));
#16960=DIRECTION('',(0.,1.,0.));
#16961=DIRECTION('center_axis',(0.,1.,0.));
#16962=DIRECTION('ref_axis',(1.,0.,0.));
#16963=DIRECTION('',(0.,-1.,0.));
#16964=DIRECTION('',(0.,1.,0.));
#16965=DIRECTION('center_axis',(0.,1.,0.));
#16966=DIRECTION('ref_axis',(1.,0.,0.));
#16967=DIRECTION('',(0.,-1.,0.));
#16968=DIRECTION('',(0.,1.,0.));
#16969=DIRECTION('center_axis',(0.,1.,0.));
#16970=DIRECTION('ref_axis',(1.,0.,0.));
#16971=DIRECTION('',(0.,-1.,0.));
#16972=DIRECTION('',(0.,1.,0.));
#16973=DIRECTION('center_axis',(0.,1.,0.));
#16974=DIRECTION('ref_axis',(1.,0.,0.));
#16975=DIRECTION('',(0.,-1.,0.));
#16976=DIRECTION('',(0.,1.,0.));
#16977=DIRECTION('center_axis',(0.,1.,0.));
#16978=DIRECTION('ref_axis',(1.,0.,0.));
#16979=DIRECTION('',(0.,-1.,0.));
#16980=DIRECTION('',(0.,1.,0.));
#16981=DIRECTION('center_axis',(0.,1.,0.));
#16982=DIRECTION('ref_axis',(1.,0.,0.));
#16983=DIRECTION('',(0.,-1.,0.));
#16984=DIRECTION('',(0.,1.,0.));
#16985=DIRECTION('center_axis',(0.,1.,0.));
#16986=DIRECTION('ref_axis',(1.,0.,0.));
#16987=DIRECTION('',(0.,-1.,0.));
#16988=DIRECTION('',(0.,1.,0.));
#16989=DIRECTION('center_axis',(0.,1.,0.));
#16990=DIRECTION('ref_axis',(1.,0.,0.));
#16991=DIRECTION('',(0.,-1.,0.));
#16992=DIRECTION('',(0.,1.,0.));
#16993=DIRECTION('center_axis',(0.,1.,0.));
#16994=DIRECTION('ref_axis',(1.,0.,0.));
#16995=DIRECTION('',(0.,-1.,0.));
#16996=DIRECTION('',(0.,1.,0.));
#16997=DIRECTION('center_axis',(0.,1.,0.));
#16998=DIRECTION('ref_axis',(1.,0.,0.));
#16999=DIRECTION('',(0.,-1.,0.));
#17000=DIRECTION('',(0.,1.,0.));
#17001=DIRECTION('center_axis',(0.,1.,0.));
#17002=DIRECTION('ref_axis',(1.,0.,0.));
#17003=DIRECTION('',(0.,-1.,0.));
#17004=DIRECTION('',(0.,1.,0.));
#17005=DIRECTION('center_axis',(0.,1.,0.));
#17006=DIRECTION('ref_axis',(1.,0.,0.));
#17007=DIRECTION('',(0.,-1.,0.));
#17008=DIRECTION('',(0.,1.,0.));
#17009=DIRECTION('center_axis',(0.,1.,0.));
#17010=DIRECTION('ref_axis',(1.,0.,0.));
#17011=DIRECTION('',(0.,-1.,0.));
#17012=DIRECTION('',(0.,1.,0.));
#17013=DIRECTION('center_axis',(0.,1.,0.));
#17014=DIRECTION('ref_axis',(1.,0.,0.));
#17015=DIRECTION('',(0.,-1.,0.));
#17016=DIRECTION('',(0.,1.,0.));
#17017=DIRECTION('center_axis',(0.,1.,0.));
#17018=DIRECTION('ref_axis',(1.,0.,0.));
#17019=DIRECTION('',(0.,-1.,0.));
#17020=DIRECTION('',(0.,1.,0.));
#17021=DIRECTION('center_axis',(0.,1.,0.));
#17022=DIRECTION('ref_axis',(1.,0.,0.));
#17023=DIRECTION('',(0.,-1.,0.));
#17024=DIRECTION('',(0.,1.,0.));
#17025=DIRECTION('center_axis',(0.,1.,0.));
#17026=DIRECTION('ref_axis',(1.,0.,0.));
#17027=DIRECTION('',(0.,-1.,0.));
#17028=DIRECTION('',(0.,1.,0.));
#17029=DIRECTION('center_axis',(0.,1.,0.));
#17030=DIRECTION('ref_axis',(1.,0.,0.));
#17031=DIRECTION('',(0.,-1.,0.));
#17032=DIRECTION('',(0.,1.,0.));
#17033=DIRECTION('center_axis',(0.,1.,0.));
#17034=DIRECTION('ref_axis',(1.,0.,0.));
#17035=DIRECTION('',(0.,-1.,0.));
#17036=DIRECTION('',(0.,1.,0.));
#17037=DIRECTION('center_axis',(0.,1.,0.));
#17038=DIRECTION('ref_axis',(1.,0.,0.));
#17039=DIRECTION('',(0.,-1.,0.));
#17040=DIRECTION('',(0.,1.,0.));
#17041=DIRECTION('center_axis',(0.,1.,0.));
#17042=DIRECTION('ref_axis',(1.,0.,0.));
#17043=DIRECTION('',(0.,-1.,0.));
#17044=DIRECTION('',(0.,1.,0.));
#17045=DIRECTION('center_axis',(0.,1.,0.));
#17046=DIRECTION('ref_axis',(1.,0.,0.));
#17047=DIRECTION('',(0.,-1.,0.));
#17048=DIRECTION('',(0.,1.,0.));
#17049=DIRECTION('center_axis',(0.,1.,0.));
#17050=DIRECTION('ref_axis',(1.,0.,0.));
#17051=DIRECTION('',(0.,-1.,0.));
#17052=DIRECTION('',(0.,1.,0.));
#17053=DIRECTION('center_axis',(0.,1.,0.));
#17054=DIRECTION('ref_axis',(1.,0.,0.));
#17055=DIRECTION('',(0.,-1.,0.));
#17056=DIRECTION('',(0.,1.,0.));
#17057=DIRECTION('center_axis',(0.,1.,0.));
#17058=DIRECTION('ref_axis',(1.,0.,0.));
#17059=DIRECTION('',(0.,-1.,0.));
#17060=DIRECTION('',(0.,1.,0.));
#17061=DIRECTION('center_axis',(0.,1.,0.));
#17062=DIRECTION('ref_axis',(1.,0.,0.));
#17063=DIRECTION('',(0.,-1.,0.));
#17064=DIRECTION('',(0.,1.,0.));
#17065=DIRECTION('center_axis',(0.,1.,0.));
#17066=DIRECTION('ref_axis',(1.,0.,0.));
#17067=DIRECTION('',(0.,-1.,0.));
#17068=DIRECTION('',(0.,1.,0.));
#17069=DIRECTION('center_axis',(0.,1.,0.));
#17070=DIRECTION('ref_axis',(1.,0.,0.));
#17071=DIRECTION('',(0.,-1.,0.));
#17072=DIRECTION('',(0.,1.,0.));
#17073=DIRECTION('center_axis',(0.,1.,0.));
#17074=DIRECTION('ref_axis',(1.,0.,0.));
#17075=DIRECTION('',(0.,-1.,0.));
#17076=DIRECTION('',(0.,1.,0.));
#17077=DIRECTION('center_axis',(0.,1.,0.));
#17078=DIRECTION('ref_axis',(1.,0.,0.));
#17079=DIRECTION('',(0.,-1.,0.));
#17080=DIRECTION('',(0.,1.,0.));
#17081=DIRECTION('center_axis',(0.10517954525379,0.,-0.994453248403466));
#17082=DIRECTION('ref_axis',(-0.994453248403466,0.,-0.10517954525379));
#17083=DIRECTION('',(-0.994453248403466,0.,-0.10517954525379));
#17084=DIRECTION('',(0.,1.,0.));
#17085=DIRECTION('center_axis',(-0.808632003366459,0.,0.588314782350016));
#17086=DIRECTION('ref_axis',(0.588314782350016,0.,0.808632003366459));
#17087=DIRECTION('',(0.588314782350016,0.,0.808632003366459));
#17088=DIRECTION('center_axis',(0.,1.,0.));
#17089=DIRECTION('ref_axis',(-0.5,0.,0.866025403784438));
#17090=DIRECTION('center_axis',(0.,1.,0.));
#17091=DIRECTION('ref_axis',(-0.64278760968654,0.,0.766044443118978));
#17092=DIRECTION('',(0.438959485082241,0.,0.89850685609868));
#17093=DIRECTION('',(-0.961081032674752,0.,-0.276266625984452));
#17094=DIRECTION('center_axis',(0.276266625984452,0.,-0.961081032674752));
#17095=DIRECTION('ref_axis',(-0.961081032674752,0.,-0.276266625984452));
#17096=DIRECTION('',(0.,1.,0.));
#17097=DIRECTION('center_axis',(-0.89850685609868,0.,0.438959485082241));
#17098=DIRECTION('ref_axis',(0.438959485082241,0.,0.89850685609868));
#17099=DIRECTION('center_axis',(0.438959485082234,0.,-0.898506856098683));
#17100=DIRECTION('ref_axis',(-0.898506856098683,0.,-0.438959485082234));
#17101=DIRECTION('',(-0.898506856098683,0.,-0.438959485082234));
#17102=DIRECTION('',(0.,1.,0.));
#17103=DIRECTION('center_axis',(-0.961081032674749,0.,0.27626662598446));
#17104=DIRECTION('ref_axis',(0.27626662598446,0.,0.961081032674749));
#17105=DIRECTION('',(0.27626662598446,0.,0.961081032674749));
#17106=DIRECTION('center_axis',(0.,1.,0.));
#17107=DIRECTION('ref_axis',(-0.766044443118978,0.,0.642787609686539));
#17108=DIRECTION('center_axis',(0.,1.,0.));
#17109=DIRECTION('ref_axis',(-0.866025403784439,0.,0.5));
#17110=DIRECTION('',(0.105179545253798,0.,0.994453248403465));
#17111=DIRECTION('',(-0.808632003366464,0.,-0.58831478235001));
#17112=DIRECTION('center_axis',(0.58831478235001,0.,-0.808632003366464));
#17113=DIRECTION('ref_axis',(-0.808632003366464,0.,-0.58831478235001));
#17114=DIRECTION('',(0.,1.,0.));
#17115=DIRECTION('center_axis',(-0.994453248403465,0.,0.105179545253798));
#17116=DIRECTION('ref_axis',(0.105179545253798,0.,0.994453248403465));
#17117=DIRECTION('center_axis',(0.719794432657726,0.,-0.694187276399491));
#17118=DIRECTION('ref_axis',(-0.694187276399491,0.,-0.719794432657726));
#17119=DIRECTION('',(-0.694187276399491,0.,-0.719794432657726));
#17120=DIRECTION('',(0.,1.,0.));
#17121=DIRECTION('center_axis',(-0.997609505397066,0.,-0.0691033627359827));
#17122=DIRECTION('ref_axis',(-0.0691033627359827,0.,0.997609505397066));
#17123=DIRECTION('',(-0.0691033627359827,0.,0.997609505397066));
#17124=DIRECTION('center_axis',(0.,1.,0.));
#17125=DIRECTION('ref_axis',(-0.939692620785909,0.,0.342020143325668));
#17126=DIRECTION('center_axis',(0.,1.,0.));
#17127=DIRECTION('ref_axis',(-0.984807753012208,0.,0.17364817766693));
#17128=DIRECTION('',(-0.241286600017019,0.,0.970453902383945));
#17129=DIRECTION('',(-0.558650020314831,0.,-0.829403493362693));
#17130=DIRECTION('center_axis',(0.829403493362693,0.,-0.558650020314831));
#17131=DIRECTION('ref_axis',(-0.558650020314831,0.,-0.829403493362693));
#17132=DIRECTION('',(0.,1.,0.));
#17133=DIRECTION('center_axis',(-0.970453902383945,0.,-0.241286600017019));
#17134=DIRECTION('ref_axis',(-0.241286600017019,0.,0.970453902383945));
#17135=DIRECTION('center_axis',(0.913811548620253,0.,-0.406138466053456));
#17136=DIRECTION('ref_axis',(-0.406138466053456,0.,-0.913811548620253));
#17137=DIRECTION('',(-0.406138466053456,0.,-0.913811548620253));
#17138=DIRECTION('',(0.,1.,0.));
#17139=DIRECTION('center_axis',(-0.913811548620257,0.,-0.406138466053449));
#17140=DIRECTION('ref_axis',(-0.406138466053449,0.,0.913811548620257));
#17141=DIRECTION('',(-0.406138466053449,0.,0.913811548620257));
#17142=DIRECTION('center_axis',(0.,1.,0.));
#17143=DIRECTION('ref_axis',(-1.,0.,-1.83697019872103E-16));
#17144=DIRECTION('center_axis',(0.,1.,0.));
#17145=DIRECTION('ref_axis',(-0.984807753012208,0.,-0.17364817766693));
#17146=DIRECTION('',(-0.558650020314825,0.,0.829403493362697));
#17147=DIRECTION('',(-0.241286600017026,0.,-0.970453902383943));
#17148=DIRECTION('center_axis',(0.970453902383943,0.,-0.241286600017026));
#17149=DIRECTION('ref_axis',(-0.241286600017026,0.,-0.970453902383943));
#17150=DIRECTION('',(0.,1.,0.));
#17151=DIRECTION('center_axis',(-0.829403493362697,0.,-0.558650020314825));
#17152=DIRECTION('ref_axis',(-0.558650020314825,0.,0.829403493362697));
#17153=DIRECTION('center_axis',(0.997609505397066,0.,-0.0691033627359897));
#17154=DIRECTION('ref_axis',(-0.0691033627359897,0.,-0.997609505397066));
#17155=DIRECTION('',(-0.0691033627359897,0.,-0.997609505397066));
#17156=DIRECTION('',(0.,1.,0.));
#17157=DIRECTION('center_axis',(-0.719794432657731,0.,-0.694187276399486));
#17158=DIRECTION('ref_axis',(-0.694187276399486,0.,0.719794432657731));
#17159=DIRECTION('',(-0.694187276399485,0.,0.719794432657731));
#17160=DIRECTION('center_axis',(0.,1.,0.));
#17161=DIRECTION('ref_axis',(-0.939692620785908,0.,-0.342020143325669));
#17162=DIRECTION('center_axis',(0.,1.,0.));
#17163=DIRECTION('ref_axis',(-0.866025403784438,0.,-0.5));
#17164=DIRECTION('',(-0.808632003366459,0.,0.588314782350016));
#17165=DIRECTION('',(0.10517954525379,0.,-0.994453248403466));
#17166=DIRECTION('center_axis',(0.994453248403466,0.,0.10517954525379));
#17167=DIRECTION('ref_axis',(0.10517954525379,0.,-0.994453248403466));
#17168=DIRECTION('',(0.,1.,0.));
#17169=DIRECTION('center_axis',(-0.588314782350016,0.,-0.808632003366459));
#17170=DIRECTION('ref_axis',(-0.808632003366459,0.,0.588314782350016));
#17171=DIRECTION('center_axis',(0.961081032674752,0.,0.276266625984452));
#17172=DIRECTION('ref_axis',(0.276266625984452,0.,-0.961081032674752));
#17173=DIRECTION('',(0.276266625984452,0.,-0.961081032674752));
#17174=DIRECTION('',(0.,1.,0.));
#17175=DIRECTION('center_axis',(-0.438959485082242,0.,-0.89850685609868));
#17176=DIRECTION('ref_axis',(-0.89850685609868,0.,0.438959485082242));
#17177=DIRECTION('',(-0.89850685609868,0.,0.438959485082241));
#17178=DIRECTION('center_axis',(0.,1.,0.));
#17179=DIRECTION('ref_axis',(-0.766044443118978,0.,-0.642787609686539));
#17180=DIRECTION('center_axis',(0.,1.,0.));
#17181=DIRECTION('ref_axis',(-0.642787609686539,0.,-0.766044443118978));
#17182=DIRECTION('',(-0.961081032674749,0.,0.27626662598446));
#17183=DIRECTION('',(0.438959485082234,0.,-0.898506856098683));
#17184=DIRECTION('center_axis',(0.898506856098683,0.,0.438959485082234));
#17185=DIRECTION('ref_axis',(0.438959485082234,0.,-0.898506856098683));
#17186=DIRECTION('',(0.,1.,0.));
#17187=DIRECTION('center_axis',(-0.27626662598446,0.,-0.961081032674749));
#17188=DIRECTION('ref_axis',(-0.961081032674749,0.,0.27626662598446));
#17189=DIRECTION('center_axis',(0.808632003366463,0.,0.58831478235001));
#17190=DIRECTION('ref_axis',(0.58831478235001,0.,-0.808632003366463));
#17191=DIRECTION('',(0.58831478235001,0.,-0.808632003366463));
#17192=DIRECTION('',(0.,1.,0.));
#17193=DIRECTION('center_axis',(-0.105179545253798,0.,-0.994453248403465));
#17194=DIRECTION('ref_axis',(-0.994453248403465,0.,0.105179545253798));
#17195=DIRECTION('',(-0.994453248403465,0.,0.105179545253798));
#17196=DIRECTION('center_axis',(0.,1.,0.));
#17197=DIRECTION('ref_axis',(-0.5,0.,-0.866025403784439));
#17198=DIRECTION('center_axis',(0.,1.,0.));
#17199=DIRECTION('ref_axis',(-0.342020143325669,0.,-0.939692620785908));
#17200=DIRECTION('',(-0.997609505397066,0.,-0.0691033627359822));
#17201=DIRECTION('',(0.719794432657725,0.,-0.694187276399491));
#17202=DIRECTION('center_axis',(0.694187276399491,0.,0.719794432657725));
#17203=DIRECTION('ref_axis',(0.719794432657725,0.,-0.694187276399491));
#17204=DIRECTION('',(0.,1.,0.));
#17205=DIRECTION('center_axis',(0.0691033627359822,0.,-0.997609505397066));
#17206=DIRECTION('ref_axis',(-0.997609505397066,0.,-0.0691033627359822));
#17207=DIRECTION('center_axis',(0.558650020314831,0.,0.829403493362693));
#17208=DIRECTION('ref_axis',(0.829403493362693,0.,-0.558650020314831));
#17209=DIRECTION('',(0.829403493362693,0.,-0.558650020314831));
#17210=DIRECTION('',(0.,1.,0.));
#17211=DIRECTION('center_axis',(0.241286600017019,0.,-0.970453902383945));
#17212=DIRECTION('ref_axis',(-0.970453902383945,0.,-0.241286600017019));
#17213=DIRECTION('',(-0.970453902383945,0.,-0.241286600017019));
#17214=DIRECTION('center_axis',(0.,1.,0.));
#17215=DIRECTION('ref_axis',(-0.17364817766693,0.,-0.984807753012208));
#17216=DIRECTION('center_axis',(0.,1.,0.));
#17217=DIRECTION('ref_axis',(1.22464679914735E-16,0.,-1.));
#17218=DIRECTION('',(-0.913811548620257,0.,-0.406138466053448));
#17219=DIRECTION('',(0.913811548620253,0.,-0.406138466053456));
#17220=DIRECTION('center_axis',(0.406138466053456,0.,0.913811548620253));
#17221=DIRECTION('ref_axis',(0.913811548620253,0.,-0.406138466053456));
#17222=DIRECTION('',(0.,1.,0.));
#17223=DIRECTION('center_axis',(0.406138466053449,0.,-0.913811548620257));
#17224=DIRECTION('ref_axis',(-0.913811548620257,0.,-0.406138466053449));
#17225=DIRECTION('center_axis',(0.241286600017026,0.,0.970453902383943));
#17226=DIRECTION('ref_axis',(0.970453902383943,0.,-0.241286600017026));
#17227=DIRECTION('',(0.970453902383943,0.,-0.241286600017026));
#17228=DIRECTION('',(0.,1.,0.));
#17229=DIRECTION('center_axis',(0.558650020314825,0.,-0.829403493362697));
#17230=DIRECTION('ref_axis',(-0.829403493362697,0.,-0.558650020314825));
#17231=DIRECTION('',(-0.829403493362697,0.,-0.558650020314825));
#17232=DIRECTION('center_axis',(0.,1.,0.));
#17233=DIRECTION('ref_axis',(0.173648177666931,0.,-0.984807753012208));
#17234=DIRECTION('center_axis',(0.,1.,0.));
#17235=DIRECTION('ref_axis',(0.342020143325669,0.,-0.939692620785908));
#17236=DIRECTION('',(-0.719794432657731,0.,-0.694187276399485));
#17237=DIRECTION('',(0.997609505397066,0.,-0.0691033627359902));
#17238=DIRECTION('center_axis',(0.0691033627359902,0.,0.997609505397066));
#17239=DIRECTION('ref_axis',(0.997609505397066,0.,-0.0691033627359902));
#17240=DIRECTION('',(0.,1.,0.));
#17241=DIRECTION('center_axis',(0.694187276399485,0.,-0.719794432657731));
#17242=DIRECTION('ref_axis',(-0.719794432657731,0.,-0.694187276399485));
#17243=DIRECTION('center_axis',(-0.10517954525379,0.,0.994453248403466));
#17244=DIRECTION('ref_axis',(0.994453248403466,0.,0.10517954525379));
#17245=DIRECTION('',(0.994453248403466,0.,0.10517954525379));
#17246=DIRECTION('',(0.,1.,0.));
#17247=DIRECTION('center_axis',(0.808632003366459,0.,-0.588314782350017));
#17248=DIRECTION('ref_axis',(-0.588314782350017,0.,-0.808632003366459));
#17249=DIRECTION('',(-0.588314782350017,0.,-0.808632003366458));
#17250=DIRECTION('center_axis',(0.,1.,0.));
#17251=DIRECTION('ref_axis',(0.5,0.,-0.866025403784439));
#17252=DIRECTION('center_axis',(0.,1.,0.));
#17253=DIRECTION('ref_axis',(0.642787609686539,0.,-0.766044443118978));
#17254=DIRECTION('',(-0.438959485082241,0.,-0.89850685609868));
#17255=DIRECTION('',(0.961081032674752,0.,0.276266625984452));
#17256=DIRECTION('center_axis',(-0.276266625984452,0.,0.961081032674752));
#17257=DIRECTION('ref_axis',(0.961081032674752,0.,0.276266625984452));
#17258=DIRECTION('',(0.,1.,0.));
#17259=DIRECTION('center_axis',(0.89850685609868,0.,-0.438959485082242));
#17260=DIRECTION('ref_axis',(-0.438959485082242,0.,-0.89850685609868));
#17261=DIRECTION('center_axis',(-0.438959485082234,0.,0.898506856098683));
#17262=DIRECTION('ref_axis',(0.898506856098683,0.,0.438959485082234));
#17263=DIRECTION('',(0.898506856098683,0.,0.438959485082234));
#17264=DIRECTION('',(0.,1.,0.));
#17265=DIRECTION('center_axis',(0.961081032674749,0.,-0.27626662598446));
#17266=DIRECTION('ref_axis',(-0.27626662598446,0.,-0.961081032674749));
#17267=DIRECTION('',(-0.27626662598446,0.,-0.961081032674749));
#17268=DIRECTION('center_axis',(0.,1.,0.));
#17269=DIRECTION('ref_axis',(0.766044443118978,0.,-0.642787609686539));
#17270=DIRECTION('center_axis',(0.,1.,0.));
#17271=DIRECTION('ref_axis',(0.866025403784439,0.,-0.5));
#17272=DIRECTION('',(-0.105179545253798,0.,-0.994453248403465));
#17273=DIRECTION('',(0.808632003366463,0.,0.58831478235001));
#17274=DIRECTION('center_axis',(-0.58831478235001,0.,0.808632003366463));
#17275=DIRECTION('ref_axis',(0.808632003366463,0.,0.58831478235001));
#17276=DIRECTION('',(0.,1.,0.));
#17277=DIRECTION('center_axis',(0.994453248403465,0.,-0.105179545253798));
#17278=DIRECTION('ref_axis',(-0.105179545253798,0.,-0.994453248403465));
#17279=DIRECTION('center_axis',(-0.719794432657725,0.,0.694187276399491));
#17280=DIRECTION('ref_axis',(0.694187276399491,0.,0.719794432657725));
#17281=DIRECTION('',(0.694187276399491,0.,0.719794432657725));
#17282=DIRECTION('',(0.,1.,0.));
#17283=DIRECTION('center_axis',(0.997609505397066,0.,0.0691033627359822));
#17284=DIRECTION('ref_axis',(0.0691033627359822,0.,-0.997609505397066));
#17285=DIRECTION('',(0.0691033627359822,0.,-0.997609505397066));
#17286=DIRECTION('center_axis',(0.,1.,0.));
#17287=DIRECTION('ref_axis',(0.939692620785908,0.,-0.342020143325669));
#17288=DIRECTION('center_axis',(0.,1.,0.));
#17289=DIRECTION('ref_axis',(0.984807753012208,0.,-0.17364817766693));
#17290=DIRECTION('',(0.241286600017018,0.,-0.970453902383945));
#17291=DIRECTION('',(0.558650020314831,0.,0.829403493362693));
#17292=DIRECTION('center_axis',(-0.829403493362693,0.,0.558650020314831));
#17293=DIRECTION('ref_axis',(0.558650020314831,0.,0.829403493362693));
#17294=DIRECTION('',(0.,1.,0.));
#17295=DIRECTION('center_axis',(0.970453902383945,0.,0.241286600017018));
#17296=DIRECTION('ref_axis',(0.241286600017018,0.,-0.970453902383945));
#17297=DIRECTION('center_axis',(-0.913811548620253,0.,0.406138466053456));
#17298=DIRECTION('ref_axis',(0.406138466053456,0.,0.913811548620253));
#17299=DIRECTION('',(0.406138466053456,0.,0.913811548620253));
#17300=DIRECTION('',(0.,1.,0.));
#17301=DIRECTION('center_axis',(0.913811548620257,0.,0.406138466053448));
#17302=DIRECTION('ref_axis',(0.406138466053448,0.,-0.913811548620257));
#17303=DIRECTION('',(0.406138466053448,0.,-0.913811548620257));
#17304=DIRECTION('center_axis',(0.,1.,0.));
#17305=DIRECTION('ref_axis',(1.,0.,6.12323399573677E-17));
#17306=DIRECTION('center_axis',(0.,1.,0.));
#17307=DIRECTION('ref_axis',(0.984807753012208,0.,0.17364817766693));
#17308=DIRECTION('',(0.558650020314825,0.,-0.829403493362697));
#17309=DIRECTION('',(0.241286600017026,0.,0.970453902383943));
#17310=DIRECTION('center_axis',(-0.970453902383943,0.,0.241286600017026));
#17311=DIRECTION('ref_axis',(0.241286600017026,0.,0.970453902383943));
#17312=DIRECTION('',(0.,1.,0.));
#17313=DIRECTION('center_axis',(0.829403493362697,0.,0.558650020314825));
#17314=DIRECTION('ref_axis',(0.558650020314825,0.,-0.829403493362697));
#17315=DIRECTION('center_axis',(-0.997609505397066,0.,0.0691033627359903));
#17316=DIRECTION('ref_axis',(0.0691033627359903,0.,0.997609505397066));
#17317=DIRECTION('',(0.0691033627359903,0.,0.997609505397066));
#17318=DIRECTION('',(0.,1.,0.));
#17319=DIRECTION('center_axis',(0.719794432657731,0.,0.694187276399485));
#17320=DIRECTION('ref_axis',(0.694187276399485,0.,-0.719794432657731));
#17321=DIRECTION('',(0.694187276399485,0.,-0.719794432657731));
#17322=DIRECTION('center_axis',(0.,1.,0.));
#17323=DIRECTION('ref_axis',(0.939692620785908,0.,0.342020143325669));
#17324=DIRECTION('center_axis',(0.,1.,0.));
#17325=DIRECTION('ref_axis',(0.866025403784439,0.,0.5));
#17326=DIRECTION('',(0.808632003366459,0.,-0.588314782350017));
#17327=DIRECTION('',(-0.10517954525379,0.,0.994453248403466));
#17328=DIRECTION('center_axis',(-0.994453248403466,0.,-0.10517954525379));
#17329=DIRECTION('ref_axis',(-0.10517954525379,0.,0.994453248403466));
#17330=DIRECTION('',(0.,1.,0.));
#17331=DIRECTION('center_axis',(0.588314782350017,0.,0.808632003366459));
#17332=DIRECTION('ref_axis',(0.808632003366459,0.,-0.588314782350017));
#17333=DIRECTION('center_axis',(-0.961081032674752,0.,-0.276266625984452));
#17334=DIRECTION('ref_axis',(-0.276266625984452,0.,0.961081032674752));
#17335=DIRECTION('',(-0.276266625984452,0.,0.961081032674752));
#17336=DIRECTION('',(0.,1.,0.));
#17337=DIRECTION('center_axis',(0.438959485082242,0.,0.89850685609868));
#17338=DIRECTION('ref_axis',(0.89850685609868,0.,-0.438959485082242));
#17339=DIRECTION('',(0.89850685609868,0.,-0.438959485082242));
#17340=DIRECTION('center_axis',(0.,1.,0.));
#17341=DIRECTION('ref_axis',(0.766044443118978,0.,0.642787609686539));
#17342=DIRECTION('center_axis',(0.,1.,0.));
#17343=DIRECTION('ref_axis',(0.642787609686539,0.,0.766044443118978));
#17344=DIRECTION('',(0.961081032674749,0.,-0.27626662598446));
#17345=DIRECTION('',(-0.438959485082234,0.,0.898506856098683));
#17346=DIRECTION('center_axis',(-0.898506856098683,0.,-0.438959485082234));
#17347=DIRECTION('ref_axis',(-0.438959485082234,0.,0.898506856098683));
#17348=DIRECTION('',(0.,1.,0.));
#17349=DIRECTION('center_axis',(0.27626662598446,0.,0.961081032674749));
#17350=DIRECTION('ref_axis',(0.961081032674749,0.,-0.27626662598446));
#17351=DIRECTION('center_axis',(-0.808632003366463,0.,-0.58831478235001));
#17352=DIRECTION('ref_axis',(-0.58831478235001,0.,0.808632003366463));
#17353=DIRECTION('',(-0.58831478235001,0.,0.808632003366463));
#17354=DIRECTION('',(0.,1.,0.));
#17355=DIRECTION('center_axis',(0.105179545253798,0.,0.994453248403465));
#17356=DIRECTION('ref_axis',(0.994453248403465,0.,-0.105179545253798));
#17357=DIRECTION('',(0.994453248403465,0.,-0.105179545253798));
#17358=DIRECTION('center_axis',(0.,1.,0.));
#17359=DIRECTION('ref_axis',(0.5,0.,0.866025403784439));
#17360=DIRECTION('center_axis',(0.,1.,0.));
#17361=DIRECTION('ref_axis',(0.342020143325669,0.,0.939692620785908));
#17362=DIRECTION('',(0.997609505397066,0.,0.0691033627359822));
#17363=DIRECTION('',(-0.719794432657725,0.,0.694187276399491));
#17364=DIRECTION('center_axis',(-0.694187276399491,0.,-0.719794432657725));
#17365=DIRECTION('ref_axis',(-0.719794432657725,0.,0.694187276399491));
#17366=DIRECTION('',(0.,1.,0.));
#17367=DIRECTION('center_axis',(-0.0691033627359822,0.,0.997609505397066));
#17368=DIRECTION('ref_axis',(0.997609505397066,0.,0.0691033627359822));
#17369=DIRECTION('center_axis',(-0.558650020314831,0.,-0.829403493362693));
#17370=DIRECTION('ref_axis',(-0.829403493362693,0.,0.558650020314831));
#17371=DIRECTION('',(-0.829403493362693,0.,0.558650020314831));
#17372=DIRECTION('',(0.,1.,0.));
#17373=DIRECTION('center_axis',(-0.241286600017018,0.,0.970453902383945));
#17374=DIRECTION('ref_axis',(0.970453902383945,0.,0.241286600017018));
#17375=DIRECTION('',(0.970453902383945,0.,0.241286600017018));
#17376=DIRECTION('center_axis',(0.,1.,0.));
#17377=DIRECTION('ref_axis',(0.17364817766693,0.,0.984807753012208));
#17378=DIRECTION('center_axis',(0.,1.,0.));
#17379=DIRECTION('ref_axis',(0.,0.,1.));
#17380=DIRECTION('',(0.913811548620257,0.,0.406138466053448));
#17381=DIRECTION('',(-0.913811548620253,0.,0.406138466053456));
#17382=DIRECTION('center_axis',(-0.406138466053456,0.,-0.913811548620253));
#17383=DIRECTION('ref_axis',(-0.913811548620253,0.,0.406138466053456));
#17384=DIRECTION('',(0.,1.,0.));
#17385=DIRECTION('center_axis',(-0.406138466053448,0.,0.913811548620257));
#17386=DIRECTION('ref_axis',(0.913811548620257,0.,0.406138466053448));
#17387=DIRECTION('center_axis',(0.,1.,0.));
#17388=DIRECTION('ref_axis',(1.,0.,0.));
#17389=DIRECTION('',(-0.5,0.,-0.866025403784439));
#17390=DIRECTION('',(-1.,0.,0.));
#17391=DIRECTION('',(-0.499999999999999,0.,0.866025403784439));
#17392=DIRECTION('',(0.500000000000001,0.,0.866025403784438));
#17393=DIRECTION('',(1.,0.,0.));
#17394=DIRECTION('',(0.5,0.,-0.866025403784438));
#17395=DIRECTION('center_axis',(0.,-1.,0.));
#17396=DIRECTION('ref_axis',(0.,0.,-1.));
#17397=DIRECTION('',(-0.5,0.,-0.866025403784439));
#17398=DIRECTION('center_axis',(0.,-1.,0.));
#17399=DIRECTION('ref_axis',(1.,0.,0.));
#17400=DIRECTION('center_axis',(0.,-1.,0.));
#17401=DIRECTION('ref_axis',(0.,0.,-1.));
#17402=DIRECTION('',(-1.,0.,0.));
#17403=DIRECTION('center_axis',(0.,-1.,0.));
#17404=DIRECTION('ref_axis',(1.,0.,0.));
#17405=DIRECTION('center_axis',(0.,-1.,0.));
#17406=DIRECTION('ref_axis',(0.,0.,-1.));
#17407=DIRECTION('',(-0.499999999999999,0.,0.866025403784439));
#17408=DIRECTION('center_axis',(0.,-1.,0.));
#17409=DIRECTION('ref_axis',(1.,0.,0.));
#17410=DIRECTION('center_axis',(0.,-1.,0.));
#17411=DIRECTION('ref_axis',(0.,0.,-1.));
#17412=DIRECTION('',(0.500000000000001,0.,0.866025403784438));
#17413=DIRECTION('center_axis',(0.,-1.,0.));
#17414=DIRECTION('ref_axis',(1.,0.,0.));
#17415=DIRECTION('center_axis',(0.,-1.,0.));
#17416=DIRECTION('ref_axis',(0.,0.,-1.));
#17417=DIRECTION('',(1.,0.,0.));
#17418=DIRECTION('center_axis',(0.,-1.,0.));
#17419=DIRECTION('ref_axis',(1.,0.,0.));
#17420=DIRECTION('center_axis',(0.,-1.,0.));
#17421=DIRECTION('ref_axis',(0.,0.,-1.));
#17422=DIRECTION('',(0.5,0.,-0.866025403784438));
#17423=DIRECTION('center_axis',(0.,-1.,0.));
#17424=DIRECTION('ref_axis',(1.,0.,0.));
#17425=DIRECTION('center_axis',(0.,-1.,0.));
#17426=DIRECTION('ref_axis',(1.,0.,0.));
#17427=DIRECTION('',(-0.85716730070211,-0.515038074910058,-1.04972719113862E-16));
#17428=DIRECTION('center_axis',(0.866025403784439,0.,-0.5));
#17429=DIRECTION('ref_axis',(-0.5,0.,-0.866025403784439));
#17430=DIRECTION('',(0.,1.,0.));
#17431=DIRECTION('',(0.,1.,0.));
#17432=DIRECTION('center_axis',(0.866025403784438,0.,0.5));
#17433=DIRECTION('ref_axis',(0.5,0.,-0.866025403784438));
#17434=DIRECTION('',(0.,1.,0.));
#17435=DIRECTION('center_axis',(0.,0.,1.));
#17436=DIRECTION('ref_axis',(1.,0.,0.));
#17437=DIRECTION('',(0.,1.,0.));
#17438=DIRECTION('center_axis',(-0.866025403784438,0.,0.500000000000001));
#17439=DIRECTION('ref_axis',(0.500000000000001,0.,0.866025403784438));
#17440=DIRECTION('',(0.,1.,0.));
#17441=DIRECTION('center_axis',(-0.866025403784439,0.,-0.499999999999999));
#17442=DIRECTION('ref_axis',(-0.499999999999999,0.,0.866025403784439));
#17443=DIRECTION('',(0.,1.,0.));
#17444=DIRECTION('center_axis',(0.,0.,-1.));
#17445=DIRECTION('ref_axis',(-1.,0.,0.));
#37374=CARTESIAN_POINT('',(0.,0.,0.));
#37375=CARTESIAN_POINT('Origin',(20.,-1.3495818343519,38.1));
#37376=CARTESIAN_POINT('',(19.3941040087494,0.647822633508007,36.2684889831927));
#37377=CARTESIAN_POINT('',(19.3941040087494,0.476638002189708,36.2684889831927));
#37378=CARTESIAN_POINT('',(19.3941040087494,-1.3495818343519,36.2684889831927));
#37379=CARTESIAN_POINT('',(18.7916762743506,0.125,39.6038272277535));
#37380=CARTESIAN_POINT('Ctrl Pts',(18.7916762743506,0.125,39.6038272277535));
#37381=CARTESIAN_POINT('Ctrl Pts',(18.7943552369861,0.125226424639445,39.6059797716448));
#37382=CARTESIAN_POINT('Ctrl Pts',(18.7970399207417,0.125452849278891,39.6081251322344));
#37383=CARTESIAN_POINT('Ctrl Pts',(18.7997303009197,0.125679273918337,39.6102632904132));
#37384=CARTESIAN_POINT('Ctrl Pts',(18.8527715398381,0.130143268819914,39.652417391807));
#37385=CARTESIAN_POINT('Ctrl Pts',(18.9081395171264,0.134607263721491,39.6918559953245));
#37386=CARTESIAN_POINT('Ctrl Pts',(18.9655252616266,0.139071258623068,39.7283134134949));
#37387=CARTESIAN_POINT('Ctrl Pts',(19.0256935947433,0.143751709048666,39.766538622563));
#37388=CARTESIAN_POINT('Ctrl Pts',(19.0880799935966,0.148432159474263,39.801485767529));
#37389=CARTESIAN_POINT('Ctrl Pts',(19.1522887348155,0.153112609899861,39.8328958906349));
#37390=CARTESIAN_POINT('Ctrl Pts',(19.2133616772821,0.15756447851049,39.8627720197242));
#37391=CARTESIAN_POINT('Ctrl Pts',(19.2760826304735,0.16201634712112,39.8894482656142));
#37392=CARTESIAN_POINT('Ctrl Pts',(19.3400830864951,0.166468215731749,39.912747148438));
#37393=CARTESIAN_POINT('Ctrl Pts',(19.4040445432911,0.170917371558144,39.9360318338882));
#37394=CARTESIAN_POINT('Ctrl Pts',(19.4692834950642,0.175366527384539,39.9559430713765));
#37395=CARTESIAN_POINT('Ctrl Pts',(19.5354114062265,0.179815683210935,39.9723514615145));
#37396=CARTESIAN_POINT('Ctrl Pts',(19.6015216446514,0.184263649996855,39.9887554664971));
#37397=CARTESIAN_POINT('Ctrl Pts',(19.6685198937496,0.188711616782775,40.0016583645436));
#37398=CARTESIAN_POINT('Ctrl Pts',(19.7360041588761,0.193159583568696,40.0109810969157));
#37399=CARTESIAN_POINT('Ctrl Pts',(19.803493474664,0.197607883249622,40.0203045270204));
#37400=CARTESIAN_POINT('Ctrl Pts',(19.8714683913022,0.202056182930547,40.0260471949188));
#37401=CARTESIAN_POINT('Ctrl Pts',(19.9395202713372,0.206504482611473,40.0281817236249));
#37402=CARTESIAN_POINT('Ctrl Pts',(20.0076437637078,0.210957463325894,40.0303184985375));
#37403=CARTESIAN_POINT('Ctrl Pts',(20.0758438888056,0.215410444040316,40.0288395426711));
#37404=CARTESIAN_POINT('Ctrl Pts',(20.1437115234743,0.219863424754736,40.0237696210619));
#37405=CARTESIAN_POINT('Ctrl Pts',(20.2116206843039,0.224319130113897,40.0186965973205));
#37406=CARTESIAN_POINT('Ctrl Pts',(20.2791964621902,0.228774835473057,40.0100282974194));
#37407=CARTESIAN_POINT('Ctrl Pts',(20.3460371446334,0.233230540832217,39.9978411027886));
#37408=CARTESIAN_POINT('Ctrl Pts',(20.4129887122295,0.237693637970639,39.9856336902473));
#37409=CARTESIAN_POINT('Ctrl Pts',(20.4792022732528,0.242156735109061,39.9698958481344));
#37410=CARTESIAN_POINT('Ctrl Pts',(20.5442894922072,0.246619832247484,39.9507543071874));
#37411=CARTESIAN_POINT('Ctrl Pts',(20.5675366133854,0.248213911110794,39.9439175467746));
#37412=CARTESIAN_POINT('Ctrl Pts',(20.5906402239489,0.249807989974104,39.936647029397));
#37413=CARTESIAN_POINT('Ctrl Pts',(20.6135832762986,0.251402068837415,39.9289500047696));
#37414=CARTESIAN_POINT('Ctrl Pts',(20.6778578532506,0.255867854078437,39.9073869191707));
#37415=CARTESIAN_POINT('Ctrl Pts',(20.7411164687301,0.26033363931946,39.88239059202));
#37416=CARTESIAN_POINT('Ctrl Pts',(20.8029679697888,0.264799424560482,39.8540766791658));
#37417=CARTESIAN_POINT('Ctrl Pts',(20.8677895021583,0.269479651193649,39.8244031678173));
#37418=CARTESIAN_POINT('Ctrl Pts',(20.931064837103,0.274159877826817,39.7910855085163));
#37419=CARTESIAN_POINT('Ctrl Pts',(20.9923620316329,0.278840104459984,39.7543156153145));
#37420=CARTESIAN_POINT('Ctrl Pts',(21.0506972463998,0.283294174958602,39.7193225029326));
#37421=CARTESIAN_POINT('Ctrl Pts',(21.1072405867157,0.287748245457221,39.6812033504462));
#37422=CARTESIAN_POINT('Ctrl Pts',(21.1616427426004,0.29220231595584,39.6401716448058));
#37423=CARTESIAN_POINT('Ctrl Pts',(21.2160135371272,0.296653818804391,39.5991635928237));
#37424=CARTESIAN_POINT('Ctrl Pts',(21.2682452047201,0.301105321652942,39.5552466140312));
#37425=CARTESIAN_POINT('Ctrl Pts',(21.3180179847816,0.305556824501493,39.5086770917043));
#37426=CARTESIAN_POINT('Ctrl Pts',(21.3677790561345,0.310007280164227,39.4621185245412));
#37427=CARTESIAN_POINT('Ctrl Pts',(21.4150820300604,0.31445773582696,39.4129089884313));
#37428=CARTESIAN_POINT('Ctrl Pts',(21.4596421494538,0.318908191489694,39.3613434712393));
#37429=CARTESIAN_POINT('Ctrl Pts',(21.5042069909409,0.323359118772995,39.3097724895824));
#37430=CARTESIAN_POINT('Ctrl Pts',(21.5460280817612,0.327810046056297,39.2558454045799));
#37431=CARTESIAN_POINT('Ctrl Pts',(21.5848604853994,0.332260973339599,39.1998908121807));
#37432=CARTESIAN_POINT('Ctrl Pts',(21.6237354026205,0.336716773482887,39.1438749608848));
#37433=CARTESIAN_POINT('Ctrl Pts',(21.6596148236905,0.341172573626175,39.0858275775493));
#37434=CARTESIAN_POINT('Ctrl Pts',(21.6922973457646,0.345628373769463,39.0261059606859));
#37435=CARTESIAN_POINT('Ctrl Pts',(21.7250006909406,0.350087012848485,38.9663462932307));
#37436=CARTESIAN_POINT('Ctrl Pts',(21.7545028711533,0.354545651927507,38.9049107121163));
#37437=CARTESIAN_POINT('Ctrl Pts',(21.7806498663585,0.35900429100653,38.8421782874333));
#37438=CARTESIAN_POINT('Ctrl Pts',(21.8068410600254,0.36347046689762,38.7793398208647));
#37439=CARTESIAN_POINT('Ctrl Pts',(21.8296655876564,0.367936642788711,38.7152005987841));
#37440=CARTESIAN_POINT('Ctrl Pts',(21.8490189771101,0.372402818679801,38.6501557772003));
#37441=CARTESIAN_POINT('Ctrl Pts',(21.8558396949991,0.373976833705365,38.6272320211717));
#37442=CARTESIAN_POINT('Ctrl Pts',(21.8622297372655,0.375550848730929,38.60419587745));
#37443=CARTESIAN_POINT('Ctrl Pts',(21.8681860530549,0.377124863756493,38.5810648896679));
#37444=CARTESIAN_POINT('Ctrl Pts',(21.8850361759466,0.381577674445521,38.5156284688136));
#37445=CARTESIAN_POINT('Ctrl Pts',(21.8984781796439,0.386030485134548,38.4491732861511));
#37446=CARTESIAN_POINT('Ctrl Pts',(21.9083943940455,0.390483295823575,38.3820875638444));
#37447=CARTESIAN_POINT('Ctrl Pts',(21.9182954981267,0.394929321322826,38.3151040667139));
#37448=CARTESIAN_POINT('Ctrl Pts',(21.9246814026906,0.399375346822077,38.2474924218077));
#37449=CARTESIAN_POINT('Ctrl Pts',(21.9274848519018,0.403821372321328,38.179653641406));
#37450=CARTESIAN_POINT('Ctrl Pts',(21.9302849582794,0.408262096378659,38.111895751983));
#37451=CARTESIAN_POINT('Ctrl Pts',(21.9295110719468,0.41270282043599,38.0439117566393));
#37452=CARTESIAN_POINT('Ctrl Pts',(21.9251476493223,0.417143544493322,37.9761085749184));
#37453=CARTESIAN_POINT('Ctrl Pts',(21.9207869958352,0.421581450355942,37.9083484227949));
#37454=CARTESIAN_POINT('Ctrl Pts',(21.9128413560973,0.426019356218561,37.8407693490899));
#37455=CARTESIAN_POINT('Ctrl Pts',(21.9013472625657,0.430457262081182,37.7737774624066));
#37456=CARTESIAN_POINT('Ctrl Pts',(21.8898564746609,0.434893891630827,37.7068048421559));
#37457=CARTESIAN_POINT('Ctrl Pts',(21.8748193422825,0.439330521180472,37.6404195609068));
#37458=CARTESIAN_POINT('Ctrl Pts',(21.8563239229228,0.443767150730117,37.5750199526796));
#37459=CARTESIAN_POINT('Ctrl Pts',(21.8378274044089,0.448204043941816,37.5096164578545));
#37460=CARTESIAN_POINT('Ctrl Pts',(21.8158723280938,0.452640937153514,37.4451992274802));
#37461=CARTESIAN_POINT('Ctrl Pts',(21.7905967731438,0.457077830365213,37.3821519987442));
#37462=CARTESIAN_POINT('Ctrl Pts',(21.7652943156175,0.461519446078893,37.3190376643447));
#37463=CARTESIAN_POINT('Ctrl Pts',(21.7366645113313,0.465961061792574,37.2572967012708));
#37464=CARTESIAN_POINT('Ctrl Pts',(21.7048934160845,0.470402677506254,37.1972924079793));
#37465=CARTESIAN_POINT('Ctrl Pts',(21.6731030694789,0.474846984569945,37.1372517557216));
#37466=CARTESIAN_POINT('Ctrl Pts',(21.6381678984885,0.479291291633636,37.0789502914494));
#37467=CARTESIAN_POINT('Ctrl Pts',(21.600318260241,0.483735598697328,37.0227237945452));
#37468=CARTESIAN_POINT('Ctrl Pts',(21.5624036754847,0.488187531784446,36.9664008181276));
#37469=CARTESIAN_POINT('Ctrl Pts',(21.5215649411301,0.492639464871564,36.9121603087784));
#37470=CARTESIAN_POINT('Ctrl Pts',(21.4780731799131,0.497091397958683,36.8603055893804));
#37471=CARTESIAN_POINT('Ctrl Pts',(21.4593285198817,0.49901015153098,36.8379565499545));
#37472=CARTESIAN_POINT('Ctrl Pts',(21.4400915149616,0.500928905103276,36.81605022023));
#37473=CARTESIAN_POINT('Ctrl Pts',(21.4203858838668,0.502847658675573,36.7946086801989));
#37474=CARTESIAN_POINT('Ctrl Pts',(21.3745873671793,0.507307098065113,36.7447756794595));
#37475=CARTESIAN_POINT('Ctrl Pts',(21.3260729876969,0.511766537454653,36.6972576874258));
#37476=CARTESIAN_POINT('Ctrl Pts',(21.2751059152635,0.516225976844192,36.6523648727114));
#37477=CARTESIAN_POINT('Ctrl Pts',(21.2216063926417,0.520906996708795,36.6052414253227));
#37478=CARTESIAN_POINT('Ctrl Pts',(21.1654043808122,0.525588016573397,36.5610112966107));
#37479=CARTESIAN_POINT('Ctrl Pts',(21.1068509412939,0.530269036438,36.5199925472781));
#37480=CARTESIAN_POINT('Ctrl Pts',(21.0512203375097,0.534716391939854,36.4810213474542));
#37481=CARTESIAN_POINT('Ctrl Pts',(20.9934678971692,0.539163747441708,36.4449489261502));
#37482=CARTESIAN_POINT('Ctrl Pts',(20.9339294161898,0.543611102943563,36.4120075822222));
#37483=CARTESIAN_POINT('Ctrl Pts',(20.87442687296,0.548055773997544,36.3790861218678));
#37484=CARTESIAN_POINT('Ctrl Pts',(20.8131408580578,0.552500445051526,36.3492922278292));
#37485=CARTESIAN_POINT('Ctrl Pts',(20.750434433992,0.556945116105508,36.3228138203387));
#37486=CARTESIAN_POINT('Ctrl Pts',(20.6877442795779,0.56138863395626,36.2963422828696));
#37487=CARTESIAN_POINT('Ctrl Pts',(20.6236349015592,0.565832151807011,36.2731847156516));
#37488=CARTESIAN_POINT('Ctrl Pts',(20.5584904774809,0.570275669657763,36.2534813991018));
#37489=CARTESIAN_POINT('Ctrl Pts',(20.4933405370955,0.574719563777237,36.2337764141122));
#37490=CARTESIAN_POINT('Ctrl Pts',(20.4271558491791,0.579163457896711,36.2175264004943));
#37491=CARTESIAN_POINT('Ctrl Pts',(20.3603351656064,0.583607352016185,36.2048216112124));
#37492=CARTESIAN_POINT('Ctrl Pts',(20.2934426758394,0.588056021590008,36.1921031692333));
#37493=CARTESIAN_POINT('Ctrl Pts',(20.2259133117688,0.592504691163832,36.1829376452654));
#37494=CARTESIAN_POINT('Ctrl Pts',(20.1581543837085,0.596953360737655,36.177363854544));
#37495=CARTESIAN_POINT('Ctrl Pts',(20.0903531986524,0.601404804667809,36.1717865877988));
#37496=CARTESIAN_POINT('Ctrl Pts',(20.0223226572537,0.605856248597963,36.1698055259595));
#37497=CARTESIAN_POINT('Ctrl Pts',(19.9544707160184,0.610307692528117,36.1714073418163));
#37498=CARTESIAN_POINT('Ctrl Pts',(19.8865043551865,0.614766642985118,36.1730118588357));
#37499=CARTESIAN_POINT('Ctrl Pts',(19.8187176862162,0.619225593442118,36.1782112711688));
#37500=CARTESIAN_POINT('Ctrl Pts',(19.751513220206,0.623684543899118,36.1869404407684));
#37501=CARTESIAN_POINT('Ctrl Pts',(19.7269667149817,0.625313180464296,36.1901287795783));
#37502=CARTESIAN_POINT('Ctrl Pts',(19.7024977718556,0.626941817029474,36.1937875260745));
#37503=CARTESIAN_POINT('Ctrl Pts',(19.6781255600714,0.628570453594653,36.197911831218));
#37504=CARTESIAN_POINT('Ctrl Pts',(19.6114040371796,0.633029019474033,36.2092025553623));
#37505=CARTESIAN_POINT('Ctrl Pts',(19.5451461333542,0.637487585353413,36.2240304178763));
#37506=CARTESIAN_POINT('Ctrl Pts',(19.4797550914421,0.641946151232793,36.2423434676939));
#37507=CARTESIAN_POINT('Ctrl Pts',(19.4510261750782,0.643904978657864,36.2503891274845));
#37508=CARTESIAN_POINT('Ctrl Pts',(19.4224645378388,0.645863806082935,36.2591068223827));
#37509=CARTESIAN_POINT('Ctrl Pts',(19.3941040087494,0.647822633508007,36.2684889831927));
#37510=CARTESIAN_POINT('',(21.2084517554459,0.125,39.6037243469665));
#37511=CARTESIAN_POINT('Origin',(20.,0.125,38.1));
#37512=CARTESIAN_POINT('Ctrl Pts',(21.2084517554458,0.125,39.6037243469665));
#37513=CARTESIAN_POINT('Ctrl Pts',(21.2627376096932,0.129560603484813,39.5600981092233));
#37514=CARTESIAN_POINT('Ctrl Pts',(21.3146994432444,0.134121206969626,39.5134957854694));
#37515=CARTESIAN_POINT('Ctrl Pts',(21.3640099546876,0.138681810454439,39.4641918488296));
#37516=CARTESIAN_POINT('Ctrl Pts',(21.4144857146843,0.143350184807133,39.4137228190044));
#37517=CARTESIAN_POINT('Ctrl Pts',(21.4621828429471,0.148018559159826,39.3604231537668));
#37518=CARTESIAN_POINT('Ctrl Pts',(21.5067884173978,0.152686933512519,39.3046290807115));
#37519=CARTESIAN_POINT('Ctrl Pts',(21.5503322354305,0.157244185511301,39.2501630863971));
#37520=CARTESIAN_POINT('Ctrl Pts',(21.5909297798399,0.161801437510084,39.1933205213499));
#37521=CARTESIAN_POINT('Ctrl Pts',(21.6283303606513,0.166358689508866,39.1344480622444));
#37522=CARTESIAN_POINT('Ctrl Pts',(21.6657316400298,0.170916026627875,39.0755745035207));
#37523=CARTESIAN_POINT('Ctrl Pts',(21.6999355900822,0.175473363746883,39.0146713641847));
#37524=CARTESIAN_POINT('Ctrl Pts',(21.7307355640131,0.180030700865892,38.9521132344708));
#37525=CARTESIAN_POINT('Ctrl Pts',(21.7615445108611,0.184589365668115,38.8895368797768));
#37526=CARTESIAN_POINT('Ctrl Pts',(21.7889473072846,0.189148030470337,38.8253049897284));
#37527=CARTESIAN_POINT('Ctrl Pts',(21.8127844940208,0.19370669527256,38.759814318682));
#37528=CARTESIAN_POINT('Ctrl Pts',(21.8376291849045,0.19845803690977,38.6915556145019));
#37529=CARTESIAN_POINT('Ctrl Pts',(21.8585999537576,0.20320937854698,38.6219298656052));
#37530=CARTESIAN_POINT('Ctrl Pts',(21.8755737871372,0.20796072018419,38.5514039498098));
#37531=CARTESIAN_POINT('Ctrl Pts',(21.8918942303274,0.212529163831136,38.4835928563204));
#37532=CARTESIAN_POINT('Ctrl Pts',(21.9045198179867,0.217097607478081,38.4149501092095));
#37533=CARTESIAN_POINT('Ctrl Pts',(21.9133938566971,0.221666051125027,38.3458993819711));
#37534=CARTESIAN_POINT('Ctrl Pts',(21.9222760848515,0.226238710779403,38.2767849309787));
#37535=CARTESIAN_POINT('Ctrl Pts',(21.9273998345808,0.230811370433779,38.2072622086335));
#37536=CARTESIAN_POINT('Ctrl Pts',(21.9287604628908,0.235384030088155,38.1377575646606));
#37537=CARTESIAN_POINT('Ctrl Pts',(21.930123546716,0.239964941985415,38.0681274862038));
#37538=CARTESIAN_POINT('Ctrl Pts',(21.9277099705963,0.244545853882674,37.9985160104603));
#37539=CARTESIAN_POINT('Ctrl Pts',(21.9215670421166,0.249126765779933,37.9293463755113));
#37540=CARTESIAN_POINT('Ctrl Pts',(21.920853625729,0.249658775492982,37.9213132767601));
#37541=CARTESIAN_POINT('Ctrl Pts',(21.9200899660964,0.25019078520603,37.9132861268745));
#37542=CARTESIAN_POINT('Ctrl Pts',(21.9192761819109,0.250722794919078,37.9052655796997));
#37543=CARTESIAN_POINT('Ctrl Pts',(21.9125225038227,0.25513799787515,37.8387022393567));
#37544=CARTESIAN_POINT('Ctrl Pts',(21.9022856862431,0.259553200831222,37.7723320598081));
#37545=CARTESIAN_POINT('Ctrl Pts',(21.8885821956735,0.263968403787293,37.7065538828697));
#37546=CARTESIAN_POINT('Ctrl Pts',(21.8749016068258,0.268376227911696,37.6408856365733));
#37547=CARTESIAN_POINT('Ctrl Pts',(21.8577659358544,0.272784052036099,37.5758079191562));
#37548=CARTESIAN_POINT('Ctrl Pts',(21.837243454715,0.277191876160502,37.5117151667712));
#37549=CARTESIAN_POINT('Ctrl Pts',(21.8167489415847,0.281593693308219,37.4477097599015));
#37550=CARTESIAN_POINT('Ctrl Pts',(21.7928769325674,0.285995510455937,37.3846871307437));
#37551=CARTESIAN_POINT('Ctrl Pts',(21.765746443274,0.290397327603654,37.3230302097473));
#37552=CARTESIAN_POINT('Ctrl Pts',(21.738635932719,0.29479590327818,37.2614186925579));
#37553=CARTESIAN_POINT('Ctrl Pts',(21.7082719002178,0.299194478952705,37.2011713501745));
#37554=CARTESIAN_POINT('Ctrl Pts',(21.674822208485,0.303593054627231,37.1426530791477));
#37555=CARTESIAN_POINT('Ctrl Pts',(21.641385043491,0.307989983057618,37.0841567229147));
#37556=CARTESIAN_POINT('Ctrl Pts',(21.6048647612107,0.312386911488005,37.0273885910638));
#37557=CARTESIAN_POINT('Ctrl Pts',(21.5654751859442,0.316783839918392,36.97268904064));
#37558=CARTESIAN_POINT('Ctrl Pts',(21.5260861074007,0.321180712901217,36.9179901800062));
#37559=CARTESIAN_POINT('Ctrl Pts',(21.4838281044081,0.325577585884041,36.8653602566341));
#37560=CARTESIAN_POINT('Ctrl Pts',(21.4389571931852,0.329974458866865,36.8151090501212));
#37561=CARTESIAN_POINT('Ctrl Pts',(21.3940403604596,0.334375831669492,36.7648064158379));
#37562=CARTESIAN_POINT('Ctrl Pts',(21.3465056195152,0.33877720447212,36.7168877333888));
#37563=CARTESIAN_POINT('Ctrl Pts',(21.296647206045,0.343178577274747,36.6716272965519));
#37564=CARTESIAN_POINT('Ctrl Pts',(21.2467605011079,0.347582447575469,36.6263411773063));
#37565=CARTESIAN_POINT('Ctrl Pts',(21.194547891955,0.35198631787619,36.5837166223241));
#37566=CARTESIAN_POINT('Ctrl Pts',(21.1403358744458,0.356390188176912,36.5439869376024));
#37567=CARTESIAN_POINT('Ctrl Pts',(21.0860284939024,0.360801805218182,36.504187365364));
#37568=CARTESIAN_POINT('Ctrl Pts',(21.0297151087096,0.365213422259452,36.467293099977));
#37569=CARTESIAN_POINT('Ctrl Pts',(20.9717494139593,0.369625039300722,36.4334929843023));
#37570=CARTESIAN_POINT('Ctrl Pts',(20.9418769245158,0.371898556146533,36.4160741712779));
#37571=CARTESIAN_POINT('Ctrl Pts',(20.9115659819915,0.374172072992344,36.3994763468264));
#37572=CARTESIAN_POINT('Ctrl Pts',(20.880867022521,0.376445589838155,36.3837203475147));
#37573=CARTESIAN_POINT('Ctrl Pts',(20.8206082552473,0.380908259741876,36.3527930095181));
#37574=CARTESIAN_POINT('Ctrl Pts',(20.7586013631052,0.385370929645597,36.3249828044127));
#37575=CARTESIAN_POINT('Ctrl Pts',(20.6952010916089,0.389833599549318,36.3004895112488));
#37576=CARTESIAN_POINT('Ctrl Pts',(20.6318875145553,0.394290167134065,36.276029710566));
#37577=CARTESIAN_POINT('Ctrl Pts',(20.5671847915107,0.398746734718812,36.2548780018324));
#37578=CARTESIAN_POINT('Ctrl Pts',(20.5014711961506,0.403203302303558,36.2371878258044));
#37579=CARTESIAN_POINT('Ctrl Pts',(20.435824970736,0.407655300990293,36.2195157858438));
#37580=CARTESIAN_POINT('Ctrl Pts',(20.369170401583,0.412107299677028,36.2052983645708));
#37581=CARTESIAN_POINT('Ctrl Pts',(20.3019029312493,0.416559298363762,36.1946398825936));
#37582=CARTESIAN_POINT('Ctrl Pts',(20.2346814083733,0.421008256085516,36.1839886809578));
#37583=CARTESIAN_POINT('Ctrl Pts',(20.1668482998834,0.42545721380727,36.1768916692167));
#37584=CARTESIAN_POINT('Ctrl Pts',(20.0988095349356,0.429906171529024,36.1734021611385));
#37585=CARTESIAN_POINT('Ctrl Pts',(20.0307737249861,0.434354936027661,36.1699128046135));
#37586=CARTESIAN_POINT('Ctrl Pts',(19.9625327664683,0.438803700526298,36.1700306803602));
#37587=CARTESIAN_POINT('Ctrl Pts',(19.8944965629556,0.443252465024935,36.1737571332587));
#37588=CARTESIAN_POINT('Ctrl Pts',(19.8264630549438,0.447701053269634,36.1774834385203));
#37589=CARTESIAN_POINT('Ctrl Pts',(19.758634776505,0.452149641514334,36.1848180015745));
#37590=CARTESIAN_POINT('Ctrl Pts',(19.6914182418001,0.456598229759033,36.1957101440678));
#37591=CARTESIAN_POINT('Ctrl Pts',(19.6241487403264,0.461050323500489,36.206610869592));
#37592=CARTESIAN_POINT('Ctrl Pts',(19.5574924290986,0.465502417241944,36.2210746823356));
#37593=CARTESIAN_POINT('Ctrl Pts',(19.4918461247712,0.4699545109834,36.2389996786701));
#37594=CARTESIAN_POINT('Ctrl Pts',(19.4589966743643,0.472182341385503,36.247969357682));
#37595=CARTESIAN_POINT('Ctrl Pts',(19.4263999182602,0.474410171787605,36.257804929465));
#37596=CARTESIAN_POINT('Ctrl Pts',(19.3941040087494,0.476638002189708,36.2684889831927));
#37597=CARTESIAN_POINT('Origin',(20.,-1.3495818343519,38.1));
#37598=CARTESIAN_POINT('',(19.3941040087494,1.44151754323334,36.2684889831927));
#37599=CARTESIAN_POINT('',(19.3941039987112,1.2718084690693,36.2684889865135));
#37600=CARTESIAN_POINT('',(19.3941040087494,-1.3495818343519,36.2684889831927));
#37601=CARTESIAN_POINT('',(18.0708702148579,0.805831834310469,38.0990895178969));
#37602=CARTESIAN_POINT('Ctrl Pts',(18.0708702148576,0.805831834351889,38.0990895185324));
#37603=CARTESIAN_POINT('Ctrl Pts',(18.0708375364269,0.810344728670084,38.1683286368148));
#37604=CARTESIAN_POINT('Ctrl Pts',(18.0745368319364,0.814857622988279,38.2375583631981));
#37605=CARTESIAN_POINT('Ctrl Pts',(18.0819387408898,0.819370517306473,38.306357852287));
#37606=CARTESIAN_POINT('Ctrl Pts',(18.0893440199819,0.823885466375696,38.3751886662445));
#37607=CARTESIAN_POINT('Ctrl Pts',(18.1004552109146,0.828400415444919,38.4435883856162));
#37608=CARTESIAN_POINT('Ctrl Pts',(18.1151913368057,0.832915364514142,38.5111433570518));
#37609=CARTESIAN_POINT('Ctrl Pts',(18.1299502559231,0.837437297118666,38.5788028197055));
#37610=CARTESIAN_POINT('Ctrl Pts',(18.1483451999935,0.841959229723191,38.6456144655361));
#37611=CARTESIAN_POINT('Ctrl Pts',(18.1702446300288,0.846481162327715,38.7111774234718));
#37612=CARTESIAN_POINT('Ctrl Pts',(18.1921629410618,0.85100699359988,38.7767969077215));
#37613=CARTESIAN_POINT('Ctrl Pts',(18.2175915807431,0.855532824872045,38.8411651228237));
#37614=CARTESIAN_POINT('Ctrl Pts',(18.2463509663266,0.86005865614421,38.903901501178));
#37615=CARTESIAN_POINT('Ctrl Pts',(18.2751686126002,0.864593655833861,38.9667649707281));
#37616=CARTESIAN_POINT('Ctrl Pts',(18.3073302582298,0.869128655523511,39.027989586192));
#37617=CARTESIAN_POINT('Ctrl Pts',(18.3426107823526,0.873663655213162,39.0872201062205));
#37618=CARTESIAN_POINT('Ctrl Pts',(18.3590838144112,0.875781117953045,39.114875768361));
#37619=CARTESIAN_POINT('Ctrl Pts',(18.3762361871948,0.877898580692929,39.1420971267213));
#37620=CARTESIAN_POINT('Ctrl Pts',(18.3940419374892,0.880016043432812,39.1688504377866));
#37621=CARTESIAN_POINT('Ctrl Pts',(18.431533734575,0.884474574079813,39.2251822234877));
#37622=CARTESIAN_POINT('Ctrl Pts',(18.4720670317525,0.888933104726814,39.2796501817338));
#37623=CARTESIAN_POINT('Ctrl Pts',(18.515430207209,0.893391635373815,39.331907093588));
#37624=CARTESIAN_POINT('Ctrl Pts',(18.5609583929547,0.898072768831235,39.3867730568011));
#37625=CARTESIAN_POINT('Ctrl Pts',(18.6096062135336,0.902753902288654,39.4392009056546));
#37626=CARTESIAN_POINT('Ctrl Pts',(18.6610762557557,0.907435035746074,39.4888217178598));
#37627=CARTESIAN_POINT('Ctrl Pts',(18.7099658284056,0.911881478849085,39.5359547723224));
#37628=CARTESIAN_POINT('Ctrl Pts',(18.7614010415462,0.916327921952096,39.5805550863722));
#37629=CARTESIAN_POINT('Ctrl Pts',(18.8150864061707,0.920774365055107,39.6223410695565));
#37630=CARTESIAN_POINT('Ctrl Pts',(18.8687393732253,0.925218124857889,39.6641018361046));
#37631=CARTESIAN_POINT('Ctrl Pts',(18.9246394097628,0.929661884660671,39.7030513386402));
#37632=CARTESIAN_POINT('Ctrl Pts',(18.9824571914328,0.934105644463453,39.7389475859933));
#37633=CARTESIAN_POINT('Ctrl Pts',(19.0402600025174,0.938548253656791,39.7748345388383));
#37634=CARTESIAN_POINT('Ctrl Pts',(19.0999791541169,0.942990862850129,39.807669546138));
#37635=CARTESIAN_POINT('Ctrl Pts',(19.1612570588225,0.947433472043467,39.837254395742));
#37636=CARTESIAN_POINT('Ctrl Pts',(19.2225402092415,0.951876461547703,39.866841777966));
#37637=CARTESIAN_POINT('Ctrl Pts',(19.2853819324421,0.956319451051938,39.893178238275));
#37638=CARTESIAN_POINT('Ctrl Pts',(19.3494024709221,0.960762440556174,39.9161127200859));
#37639=CARTESIAN_POINT('Ctrl Pts',(19.4134919925981,0.965210217455566,39.9390719141827));
#37640=CARTESIAN_POINT('Ctrl Pts',(19.4787623989205,0.969657994354959,39.9586216491901));
#37641=CARTESIAN_POINT('Ctrl Pts',(19.5448174874032,0.974105771254351,39.9746603524708));
#37642=CARTESIAN_POINT('Ctrl Pts',(19.6109138654164,0.97855632835772,39.9907090811795));
#37643=CARTESIAN_POINT('Ctrl Pts',(19.677795417065,0.983006885461089,40.0032423202488));
#37644=CARTESIAN_POINT('Ctrl Pts',(19.7450572066299,0.987457442564458,40.0122099071516));
#37645=CARTESIAN_POINT('Ctrl Pts',(19.8124327009231,0.991915523246807,40.0211926535831));
#37646=CARTESIAN_POINT('Ctrl Pts',(19.8801892247977,0.996373603929156,40.0265976818341));
#37647=CARTESIAN_POINT('Ctrl Pts',(19.9479191791693,1.0008316846115,40.0284268575711));
#37648=CARTESIAN_POINT('Ctrl Pts',(19.9727700303623,1.00246740252497,40.0290980018893));
#37649=CARTESIAN_POINT('Ctrl Pts',(19.9976173359428,1.00410312043843,40.0292882585755));
#37650=CARTESIAN_POINT('Ctrl Pts',(20.0224411443908,1.00573883835189,40.028999469139));
#37651=CARTESIAN_POINT('Ctrl Pts',(20.090102396661,1.01019724861627,40.0282123274336));
#37652=CARTESIAN_POINT('Ctrl Pts',(20.1578557735094,1.01465565888065,40.0238594090442));
#37653=CARTESIAN_POINT('Ctrl Pts',(20.2252948295895,1.01911406914503,40.0159292253787));
#37654=CARTESIAN_POINT('Ctrl Pts',(20.2961030813753,1.02379521765028,40.0076028567382));
#37655=CARTESIAN_POINT('Ctrl Pts',(20.3665642414268,1.02847636615553,39.9953323339279));
#37656=CARTESIAN_POINT('Ctrl Pts',(20.4362069181355,1.03315751466077,39.9791663261858));
#37657=CARTESIAN_POINT('Ctrl Pts',(20.5023560627118,1.03760383958525,39.9638112646935));
#37658=CARTESIAN_POINT('Ctrl Pts',(20.5677663119074,1.04205016450972,39.9449422565196));
#37659=CARTESIAN_POINT('Ctrl Pts',(20.6320406205111,1.04649648943419,39.9226538922472));
#37660=CARTESIAN_POINT('Ctrl Pts',(20.6962761567255,1.05094013218837,39.9003789730536));
#37661=CARTESIAN_POINT('Ctrl Pts',(20.759376646732,1.05538377494255,39.8746889507375));
#37662=CARTESIAN_POINT('Ctrl Pts',(20.820959846084,1.05982741769673,39.8457283545895));
#37663=CARTESIAN_POINT('Ctrl Pts',(20.8825271177261,1.06426991115932,39.8167752487307));
#37664=CARTESIAN_POINT('Ctrl Pts',(20.9425774317927,1.06871240462191,39.7845534582554));
#37665=CARTESIAN_POINT('Ctrl Pts',(21.000749884414,1.0731548980845,39.7492550517568));
#37666=CARTESIAN_POINT('Ctrl Pts',(21.0589273367702,1.0775977733651,39.7139536114739));
#37667=CARTESIAN_POINT('Ctrl Pts',(21.115226187162,1.0820406486457,39.6755752883961));
#37668=CARTESIAN_POINT('Ctrl Pts',(21.1693130217081,1.0864835239263,39.6343564169266));
#37669=CARTESIAN_POINT('Ctrl Pts',(21.2234581738335,1.09093118960986,39.5930931023902));
#37670=CARTESIAN_POINT('Ctrl Pts',(21.2753861584475,1.09537885529341,39.5489834279105));
#37671=CARTESIAN_POINT('Ctrl Pts',(21.324796121244,1.09982652097696,39.5023044583959));
#37672=CARTESIAN_POINT('Ctrl Pts',(21.3742369877044,1.10427696847126,39.4555962933283));
#37673=CARTESIAN_POINT('Ctrl Pts',(21.4211563585478,1.10872741596556,39.4063159926053));
#37674=CARTESIAN_POINT('Ctrl Pts',(21.4652917531,1.11317786345986,39.3547759302749));
#37675=CARTESIAN_POINT('Ctrl Pts',(21.5095017936349,1.11763583797482,39.3031486984823));
#37676=CARTESIAN_POINT('Ctrl Pts',(21.550918163011,1.12209381248979,39.2492544697726));
#37677=CARTESIAN_POINT('Ctrl Pts',(21.5893205765428,1.12655178700475,39.1934361718353));
#37678=CARTESIAN_POINT('Ctrl Pts',(21.6034189034892,1.12818840242682,39.1729441104896));
#37679=CARTESIAN_POINT('Ctrl Pts',(21.6171114584664,1.1298250178489,39.1521929770421));
#37680=CARTESIAN_POINT('Ctrl Pts',(21.6303889112557,1.13146163327097,39.1312005406101));
#37681=CARTESIAN_POINT('Ctrl Pts',(21.6665573162937,1.13591985055228,39.0740161577577));
#37682=CARTESIAN_POINT('Ctrl Pts',(21.6997850246439,1.14037806783358,39.0148135949029));
#37683=CARTESIAN_POINT('Ctrl Pts',(21.7298411424651,1.14483628511489,38.9539275020369));
#37684=CARTESIAN_POINT('Ctrl Pts',(21.7614003660684,1.14951745774302,38.8899964970243));
#37685=CARTESIAN_POINT('Ctrl Pts',(21.789462086792,1.15419863037115,38.8242095647201));
#37686=CARTESIAN_POINT('Ctrl Pts',(21.813810486032,1.15887980299928,38.7569886434791));
#37687=CARTESIAN_POINT('Ctrl Pts',(21.8369363081649,1.16332592549403,38.6931430061166));
#37688=CARTESIAN_POINT('Ctrl Pts',(21.856712530907,1.16777204798877,38.6280044457409));
#37689=CARTESIAN_POINT('Ctrl Pts',(21.8730023608158,1.17221817048352,38.5619574799466));
#37690=CARTESIAN_POINT('Ctrl Pts',(21.8892823530286,1.17666160789183,38.4959504010002));
#37691=CARTESIAN_POINT('Ctrl Pts',(21.90208001124,1.18110504530014,38.4290364827223));
#37692=CARTESIAN_POINT('Ctrl Pts',(21.9113084892897,1.18554848270846,38.3616150142273));
#37693=CARTESIAN_POINT('Ctrl Pts',(21.9205345749982,1.18999076822389,38.2942110237121));
#37694=CARTESIAN_POINT('Ctrl Pts',(21.9261932507027,1.19443305373932,38.2263002326203));
#37695=CARTESIAN_POINT('Ctrl Pts',(21.9282491652835,1.19887533925475,38.1582899089341));
#37696=CARTESIAN_POINT('Ctrl Pts',(21.9303052555122,1.20331800429885,38.0902737747551));
#37697=CARTESIAN_POINT('Ctrl Pts',(21.9287579614393,1.20776066934295,38.0221585841003));
#37698=CARTESIAN_POINT('Ctrl Pts',(21.9236240288139,1.21220333438705,37.9543526427636));
#37699=CARTESIAN_POINT('Ctrl Pts',(21.9184845628255,1.21665078774448,37.886473620047));
#37700=CARTESIAN_POINT('Ctrl Pts',(21.9097507825299,1.2210982411019,37.8189050042981));
#37701=CARTESIAN_POINT('Ctrl Pts',(21.8974913247376,1.22554569445933,37.7520499612795));
#37702=CARTESIAN_POINT('Ctrl Pts',(21.8852242028801,1.22999592816582,37.685153123476));
#37703=CARTESIAN_POINT('Ctrl Pts',(21.8694271321472,1.2344461618723,37.6189712256426));
#37704=CARTESIAN_POINT('Ctrl Pts',(21.8502192575874,1.23889639557879,37.5538944646382));
#37705=CARTESIAN_POINT('Ctrl Pts',(21.8309788962331,1.24335415608515,37.4887076375589));
#37706=CARTESIAN_POINT('Ctrl Pts',(21.8083163849743,1.24781191659151,37.4246301410885));
#37707=CARTESIAN_POINT('Ctrl Pts',(21.7823994685512,1.25226967709787,37.3620334076611));
#37708=CARTESIAN_POINT('Ctrl Pts',(21.7728748658489,1.25390792746193,37.3390287798486));
#37709=CARTESIAN_POINT('Ctrl Pts',(21.7629111736797,1.25554617782599,37.3162239086065));
#37710=CARTESIAN_POINT('Ctrl Pts',(21.7525182496752,1.25718442819005,37.2936363466429));
#37711=CARTESIAN_POINT('Ctrl Pts',(21.7242347992446,1.26164278590963,37.2321662359342));
#37712=CARTESIAN_POINT('Ctrl Pts',(21.692657444663,1.26610114362921,37.1720645920368));
#37713=CARTESIAN_POINT('Ctrl Pts',(21.6579412609868,1.27055950134879,37.1137072787364));
#37714=CARTESIAN_POINT('Ctrl Pts',(21.6214902066828,1.27524065642214,37.0524336774676));
#37715=CARTESIAN_POINT('Ctrl Pts',(21.5815785269907,1.27992181149548,36.9930838459159));
#37716=CARTESIAN_POINT('Ctrl Pts',(21.5384427033784,1.28460296656883,36.9360684705183));
#37717=CARTESIAN_POINT('Ctrl Pts',(21.4974713161616,1.28904923421996,36.8819139690597));
#37718=CARTESIAN_POINT('Ctrl Pts',(21.4535918880559,1.29349550187109,36.8298657455208));
#37719=CARTESIAN_POINT('Ctrl Pts',(21.407052543974,1.29794176952222,36.7802478659247));
#37720=CARTESIAN_POINT('Ctrl Pts',(21.3605412908559,1.3023853534238,36.7306599354842));
#37721=CARTESIAN_POINT('Ctrl Pts',(21.311373643304,1.30682893732537,36.683499797911));
#37722=CARTESIAN_POINT('Ctrl Pts',(21.2598373041568,1.31127252122695,36.6390576589219));
#37723=CARTESIAN_POINT('Ctrl Pts',(21.2083143116984,1.31571495434575,36.594627029392));
#37724=CARTESIAN_POINT('Ctrl Pts',(21.1544242188662,1.32015738746455,36.5529133228303));
#37725=CARTESIAN_POINT('Ctrl Pts',(21.0984894509131,1.32459982058335,36.5141678893614));
#37726=CARTESIAN_POINT('Ctrl Pts',(21.0425498931683,1.32904263411545,36.4754191380533));
#37727=CARTESIAN_POINT('Ctrl Pts',(20.9845657196497,1.33348544764756,36.4396394429375));
#37728=CARTESIAN_POINT('Ctrl Pts',(20.9248885832387,1.33792826117966,36.4070370159113));
#37729=CARTESIAN_POINT('Ctrl Pts',(20.8651471238273,1.34237586339826,36.3743994483596));
#37730=CARTESIAN_POINT('Ctrl Pts',(20.8037094941599,1.34682346561685,36.3449462187376));
#37731=CARTESIAN_POINT('Ctrl Pts',(20.7409512806138,1.35127106783545,36.3188392108918));
#37732=CARTESIAN_POINT('Ctrl Pts',(20.6781538291989,1.35572145079656,36.2927158803482));
#37733=CARTESIAN_POINT('Ctrl Pts',(20.6140346155322,1.36017183375768,36.269943099653));
#37734=CARTESIAN_POINT('Ctrl Pts',(20.5489858398327,1.36462221671879,36.2506333233879));
#37735=CARTESIAN_POINT('Ctrl Pts',(20.4838270606544,1.36908012568793,36.2312908925104));
#37736=CARTESIAN_POINT('Ctrl Pts',(20.4177360617848,1.37353803465707,36.2154232658737));
#37737=CARTESIAN_POINT('Ctrl Pts',(20.3511157569468,1.37799594362621,36.2030919152148));
#37738=CARTESIAN_POINT('Ctrl Pts',(20.3266505544972,1.37963303678718,36.1985634311275));
#37739=CARTESIAN_POINT('Ctrl Pts',(20.3021140174735,1.38127012994815,36.1945113448649));
#37740=CARTESIAN_POINT('Ctrl Pts',(20.277526192677,1.38290722310913,36.1909369394181));
#37741=CARTESIAN_POINT('Ctrl Pts',(20.2105625873692,1.3873657574118,36.1812022403332));
#37742=CARTESIAN_POINT('Ctrl Pts',(20.1429538919583,1.39182429171447,36.1749758707396));
#37743=CARTESIAN_POINT('Ctrl Pts',(20.0750998695106,1.39628282601714,36.1723323506114));
#37744=CARTESIAN_POINT('Ctrl Pts',(20.0073627852413,1.40073367657666,36.1696933862695));
#37745=CARTESIAN_POINT('Ctrl Pts',(19.9393817025843,1.40518452713618,36.170625024732));
#37746=CARTESIAN_POINT('Ctrl Pts',(19.871563278678,1.4096353776957,36.1751502485867));
#37747=CARTESIAN_POINT('Ctrl Pts',(19.8038123646269,1.41408179765569,36.1796709678069));
#37748=CARTESIAN_POINT('Ctrl Pts',(19.7362242776704,1.41852821761569,36.1877781444111));
#37749=CARTESIAN_POINT('Ctrl Pts',(19.6692060914125,1.42297463757568,36.1994427272662));
#37750=CARTESIAN_POINT('Ctrl Pts',(19.6022324842504,1.42741809987012,36.2110995510848));
#37751=CARTESIAN_POINT('Ctrl Pts',(19.5358285100785,1.43186156216455,36.2263090000941));
#37752=CARTESIAN_POINT('Ctrl Pts',(19.4703946875471,1.43630502445899,36.2449903585368));
#37753=CARTESIAN_POINT('Ctrl Pts',(19.444808406263,1.4380425307171,36.2522952426684));
#37754=CARTESIAN_POINT('Ctrl Pts',(19.419370360307,1.43978003697522,36.2601304306196));
#37755=CARTESIAN_POINT('Ctrl Pts',(19.3941040087494,1.44151754323334,36.2684889831927));
#37756=CARTESIAN_POINT('Ctrl Pts',(19.3941040087494,0.647822633508007,36.2684889831927));
#37757=CARTESIAN_POINT('Ctrl Pts',(19.3296825780713,0.652272143768435,36.2898007231934));
#37758=CARTESIAN_POINT('Ctrl Pts',(19.2662997849573,0.656721654028864,36.3145443384515));
#37759=CARTESIAN_POINT('Ctrl Pts',(19.2043437516652,0.661171164289292,36.3425946138168));
#37760=CARTESIAN_POINT('Ctrl Pts',(19.1424379591573,0.66561706639612,36.3706221429255));
#37761=CARTESIAN_POINT('Ctrl Pts',(19.0819570792625,0.670062968502948,36.4019508116598));
#37762=CARTESIAN_POINT('Ctrl Pts',(19.0232707684852,0.674508870609776,36.436406730837));
#37763=CARTESIAN_POINT('Ctrl Pts',(18.9646118433448,0.678952698061392,36.4708465713532));
#37764=CARTESIAN_POINT('Ctrl Pts',(18.9077462502621,0.683396525513008,36.5084105175293));
#37765=CARTESIAN_POINT('Ctrl Pts',(18.8530188338067,0.687840352964625,36.5488788695599));
#37766=CARTESIAN_POINT('Ctrl Pts',(18.7982981155217,0.692283636529552,36.5893422686083));
#37767=CARTESIAN_POINT('Ctrl Pts',(18.7457154498577,0.69672692009448,36.6327090737228));
#37768=CARTESIAN_POINT('Ctrl Pts',(18.6955849742837,0.701170203659408,36.6787174814325));
#37769=CARTESIAN_POINT('Ctrl Pts',(18.6454071775631,0.705617681504766,36.7247693192231));
#37770=CARTESIAN_POINT('Ctrl Pts',(18.5976865603997,0.710065159350124,36.7734674081238));
#37771=CARTESIAN_POINT('Ctrl Pts',(18.5527018104802,0.714512637195483,36.8245116592016));
#37772=CARTESIAN_POINT('Ctrl Pts',(18.5076973583265,0.718962062928732,36.8755782664288));
#37773=CARTESIAN_POINT('Ctrl Pts',(18.4654314683306,0.723411488661982,36.9289926967059));
#37774=CARTESIAN_POINT('Ctrl Pts',(18.4261419147534,0.727860914395232,36.9844224435729));
#37775=CARTESIAN_POINT('Ctrl Pts',(18.38677833786,0.732318723050085,37.0399566226185));
#37776=CARTESIAN_POINT('Ctrl Pts',(18.3504025685493,0.736776531704938,37.0975132884453));
#37777=CARTESIAN_POINT('Ctrl Pts',(18.31720819634,0.741234340359791,37.1567321152321));
#37778=CARTESIAN_POINT('Ctrl Pts',(18.284794493295,0.745587309744439,37.2145582266594));
#37779=CARTESIAN_POINT('Ctrl Pts',(18.2554142752578,0.749940279129086,37.2739687353062));
#37780=CARTESIAN_POINT('Ctrl Pts',(18.2292031604449,0.754293248513733,37.3346104848368));
#37781=CARTESIAN_POINT('Ctrl Pts',(18.1996096019636,0.759207951874184,37.4030778191702));
#37782=CARTESIAN_POINT('Ctrl Pts',(18.1739551436919,0.764122655234634,37.4733458910155));
#37783=CARTESIAN_POINT('Ctrl Pts',(18.1524389775309,0.769037358595085,37.5449677260259));
#37784=CARTESIAN_POINT('Ctrl Pts',(18.1309889157911,0.773936962442971,37.6163695162608));
#37785=CARTESIAN_POINT('Ctrl Pts',(18.1136519233921,0.778836566290857,37.6891164859107));
#37786=CARTESIAN_POINT('Ctrl Pts',(18.1005789573201,0.783736170138742,37.7627430363586));
#37787=CARTESIAN_POINT('Ctrl Pts',(18.0875715999345,0.788611184572784,37.8360000806637));
#37788=CARTESIAN_POINT('Ctrl Pts',(18.0787857077949,0.793486199006826,37.9101276018189));
#37789=CARTESIAN_POINT('Ctrl Pts',(18.0743217702651,0.798361213440869,37.9846487432881));
#37790=CARTESIAN_POINT('Ctrl Pts',(18.0720415455723,0.800851420397402,38.0227149003028));
#37791=CARTESIAN_POINT('Ctrl Pts',(18.0708882467697,0.803341627353937,38.0608834971368));
#37792=CARTESIAN_POINT('Ctrl Pts',(18.0708702148579,0.80583183431047,38.0990895178969));
#37793=CARTESIAN_POINT('',(18.0708701424417,0.634793165648104,38.0992586653166));
#37794=CARTESIAN_POINT('Ctrl Pts',(19.3941040087494,0.476638002189708,36.2684889831927));
#37795=CARTESIAN_POINT('Ctrl Pts',(19.3294175465539,0.481100191651656,36.2898884002712));
#37796=CARTESIAN_POINT('Ctrl Pts',(19.2659395802241,0.485562381113605,36.3146945708179));
#37797=CARTESIAN_POINT('Ctrl Pts',(19.2040403110517,0.490024570575553,36.3427320265624));
#37798=CARTESIAN_POINT('Ctrl Pts',(19.1478875166129,0.494072508636116,36.3681665997014));
#37799=CARTESIAN_POINT('Ctrl Pts',(19.0930338622291,0.49812044669668,36.396259611507));
#37800=CARTESIAN_POINT('Ctrl Pts',(19.039736132611,0.502168384757243,36.4268485239264));
#37801=CARTESIAN_POINT('Ctrl Pts',(18.9809367333944,0.506634172094393,36.4605949834068));
#37802=CARTESIAN_POINT('Ctrl Pts',(18.9238067121829,0.511099959431543,36.4975088597523));
#37803=CARTESIAN_POINT('Ctrl Pts',(18.8687069543993,0.515565746768693,36.5374000505966));
#37804=CARTESIAN_POINT('Ctrl Pts',(18.8109614058647,0.520245973139844,36.5792067443038));
#37805=CARTESIAN_POINT('Ctrl Pts',(18.7554465291093,0.524926199510996,36.6242837043234));
#37806=CARTESIAN_POINT('Ctrl Pts',(18.7025482558196,0.529606425882147,36.6723580531438));
#37807=CARTESIAN_POINT('Ctrl Pts',(18.6522060845453,0.534060498632098,36.7181093972183));
#37808=CARTESIAN_POINT('Ctrl Pts',(18.604233914001,0.538514571382049,36.7665747903607));
#37809=CARTESIAN_POINT('Ctrl Pts',(18.5589324175991,0.542968644132,36.8174764018338));
#37810=CARTESIAN_POINT('Ctrl Pts',(18.513657035742,0.547420149282835,36.8683486705144));
#37811=CARTESIAN_POINT('Ctrl Pts',(18.4710495995293,0.551871654433669,36.9216540050198));
#37812=CARTESIAN_POINT('Ctrl Pts',(18.4313733960811,0.556323159584503,36.9770783044318));
#37813=CARTESIAN_POINT('Ctrl Pts',(18.3917065257618,0.56077361759705,37.0324895662522));
#37814=CARTESIAN_POINT('Ctrl Pts',(18.3549698047799,0.565224075609597,37.0900184039082));
#37815=CARTESIAN_POINT('Ctrl Pts',(18.3213846271721,0.569674533622144,37.1493197240892));
#37816=CARTESIAN_POINT('Ctrl Pts',(18.2877958901681,0.574125463299408,37.2086273290932));
#37817=CARTESIAN_POINT('Ctrl Pts',(18.257359599313,0.578576392976672,37.2697073608492));
#37818=CARTESIAN_POINT('Ctrl Pts',(18.2302515115956,0.583027322653936,37.3321895776363));
#37819=CARTESIAN_POINT('Ctrl Pts',(18.2031137457402,0.587483125242418,37.3947402004233));
#37820=CARTESIAN_POINT('Ctrl Pts',(18.179311649001,0.5919389278309,37.4586956198149));
#37821=CARTESIAN_POINT('Ctrl Pts',(18.158972662104,0.596394730419382,37.5236659839818));
#37822=CARTESIAN_POINT('Ctrl Pts',(18.1386207164334,0.600853371976063,37.5886777433394));
#37823=CARTESIAN_POINT('Ctrl Pts',(18.1217363932387,0.605312013532744,37.65470525861));
#37824=CARTESIAN_POINT('Ctrl Pts',(18.108396401476,0.609770655089425,37.7213466189892));
#37825=CARTESIAN_POINT('Ctrl Pts',(18.0950338599389,0.614236833484401,37.7881006291858));
#37826=CARTESIAN_POINT('Ctrl Pts',(18.085227675063,0.618703011879377,37.855470069508));
#37827=CARTESIAN_POINT('Ctrl Pts',(18.0790028157059,0.623169190274353,37.9230469699773));
#37828=CARTESIAN_POINT('Ctrl Pts',(18.076809014704,0.624743186741677,37.9468628127862));
#37829=CARTESIAN_POINT('Ctrl Pts',(18.0750595549418,0.626317183209,37.9707044216641));
#37830=CARTESIAN_POINT('Ctrl Pts',(18.0737539884187,0.627891179676323,37.9945539959639));
#37831=CARTESIAN_POINT('Ctrl Pts',(18.0718456821816,0.630191841666916,38.0294141816267));
#37832=CARTESIAN_POINT('Ctrl Pts',(18.070883565912,0.632492503657509,38.0643275905245));
#37833=CARTESIAN_POINT('Ctrl Pts',(18.0708701424417,0.634793165648104,38.0992586653166));
#37834=CARTESIAN_POINT('Ctrl Pts',(18.0708701850429,0.63643967452627,38.0991550480818));
#37835=CARTESIAN_POINT('Ctrl Pts',(18.0707960163012,0.647136816316794,38.2684914658409));
#37836=CARTESIAN_POINT('Ctrl Pts',(18.0930174737715,0.656903307811155,38.4371308561225));
#37837=CARTESIAN_POINT('Ctrl Pts',(18.1582675041732,0.67210444457396,38.6799011851684));
#37838=CARTESIAN_POINT('Ctrl Pts',(18.1845703861749,0.67714691526514,38.7576297569914));
#37839=CARTESIAN_POINT('Ctrl Pts',(18.2231528068951,0.683593516580006,38.8514900500262));
#37840=CARTESIAN_POINT('Ctrl Pts',(18.2308439642046,0.684841634406725,38.8694219384789));
#37841=CARTESIAN_POINT('Ctrl Pts',(18.2423267411974,0.686655017802892,38.8951111412327));
#37842=CARTESIAN_POINT('Ctrl Pts',(18.2459006862306,0.687212864084422,38.9029648840773));
#37843=CARTESIAN_POINT('Ctrl Pts',(18.2522231826203,0.688188580642212,38.9166149041945));
#37844=CARTESIAN_POINT('Ctrl Pts',(18.2549482000501,0.688605636372264,38.9224219835042));
#37845=CARTESIAN_POINT('Ctrl Pts',(18.2602703673209,0.68941357159051,38.9336181070046));
#37846=CARTESIAN_POINT('Ctrl Pts',(18.2628637245384,0.689804315978265,38.9390088809201));
#37847=CARTESIAN_POINT('Ctrl Pts',(18.2690840747754,0.690734667746149,38.9517865564289));
#37848=CARTESIAN_POINT('Ctrl Pts',(18.2727333199285,0.691275045090943,38.9591624353175));
#37849=CARTESIAN_POINT('Ctrl Pts',(18.285862423631,0.69320032785927,38.9852773252386));
#37850=CARTESIAN_POINT('Ctrl Pts',(18.2956006605865,0.69459423823625,39.003884066555));
#37851=CARTESIAN_POINT('Ctrl Pts',(18.3837937590825,0.706932227740955,39.1658989919137));
#37852=CARTESIAN_POINT('Ctrl Pts',(18.4798637686953,0.718545336308115,39.2989275004827));
#37853=CARTESIAN_POINT('Ctrl Pts',(18.6427729657352,0.735564467313776,39.472990751488));
#37854=CARTESIAN_POINT('Ctrl Pts',(18.6971823194854,0.740901450122557,39.5247232932139));
#37855=CARTESIAN_POINT('Ctrl Pts',(18.7717204429489,0.747657053450741,39.5877440006131));
#37856=CARTESIAN_POINT('Ctrl Pts',(18.7892270350464,0.749206704337762,39.6020259008141));
#37857=CARTESIAN_POINT('Ctrl Pts',(18.8149221637498,0.751423653507232,39.6222467566481));
#37858=CARTESIAN_POINT('Ctrl Pts',(18.8229122385359,0.752105184335773,39.6284335373905));
#37859=CARTESIAN_POINT('Ctrl Pts',(18.8354929635558,0.753165606238019,39.6380177256604));
#37860=CARTESIAN_POINT('Ctrl Pts',(18.840050581204,0.753547194083509,39.6414579171035));
#37861=CARTESIAN_POINT('Ctrl Pts',(18.8486349841852,0.754261010727628,39.6478779829543));
#37862=CARTESIAN_POINT('Ctrl Pts',(18.8526582191138,0.754593545653357,39.6508624984162));
#37863=CARTESIAN_POINT('Ctrl Pts',(18.8595633739831,0.755160790042152,39.6559433016052));
#37864=CARTESIAN_POINT('Ctrl Pts',(18.8624395340883,0.755396029692384,39.6580473173213));
#37865=CARTESIAN_POINT('Ctrl Pts',(18.8680420399243,0.755852238753741,39.6621219700122));
#37866=CARTESIAN_POINT('Ctrl Pts',(18.8707677018916,0.756073269352352,39.664093440276));
#37867=CARTESIAN_POINT('Ctrl Pts',(18.8780292384997,0.756659727816691,39.6693168309437));
#37868=CARTESIAN_POINT('Ctrl Pts',(18.8825741349209,0.757024307240007,39.6725562449382));
#37869=CARTESIAN_POINT('Ctrl Pts',(18.8989158878309,0.758326598704165,39.684097350207));
#37870=CARTESIAN_POINT('Ctrl Pts',(18.9107920682362,0.759257047103402,39.6922866413547));
#37871=CARTESIAN_POINT('Ctrl Pts',(19.0262125319464,0.768158508695826,39.769979778012));
#37872=CARTESIAN_POINT('Ctrl Pts',(19.1361903867827,0.77556621292686,39.8294324552203));
#37873=CARTESIAN_POINT('Ctrl Pts',(19.2552495734574,0.783281716279286,39.8795811647537));
#37874=CARTESIAN_POINT('Ctrl Pts',(19.2593524697077,0.7835472246046,39.8812926642275));
#37875=CARTESIAN_POINT('Ctrl Pts',(19.3930603468818,0.792188489346536,39.9365263085072));
#37876=CARTESIAN_POINT('Ctrl Pts',(19.5280898157622,0.800611551962914,39.9757659507804));
#37877=CARTESIAN_POINT('Ctrl Pts',(19.6814632105573,0.810550973013383,40.0027133225902));
#37878=CARTESIAN_POINT('Ctrl Pts',(19.6967884152628,0.811547629545846,40.0052155748134));
#37879=CARTESIAN_POINT('Ctrl Pts',(19.7199673222899,0.813061003573724,40.0087134121138));
#37880=CARTESIAN_POINT('Ctrl Pts',(19.7277999335788,0.813573425175118,40.0098461485));
#37881=CARTESIAN_POINT('Ctrl Pts',(19.7418935235069,0.814497379522793,40.0117958753232));
#37882=CARTESIAN_POINT('Ctrl Pts',(19.7481519960678,0.814908358030055,40.012630388614));
#37883=CARTESIAN_POINT('Ctrl Pts',(19.761600592569,0.815793009911337,40.0143564902148));
#37884=CARTESIAN_POINT('Ctrl Pts',(19.7687918492438,0.816266981316793,40.015238323999));
#37885=CARTESIAN_POINT('Ctrl Pts',(19.788289058924,0.817554632051001,40.0175177764687));
#37886=CARTESIAN_POINT('Ctrl Pts',(19.8006036118689,0.818370725618757,40.0188374120764));
#37887=CARTESIAN_POINT('Ctrl Pts',(19.8578997288973,0.822181417956825,40.0244197991112));
#37888=CARTESIAN_POINT('Ctrl Pts',(19.9030062547931,0.825220898845349,40.027219678699));
#37889=CARTESIAN_POINT('Ctrl Pts',(19.9803390362335,0.830503549754191,40.0292982725189));
#37890=CARTESIAN_POINT('Ctrl Pts',(20.0125266743961,0.832723378863548,40.0293577368835));
#37891=CARTESIAN_POINT('Ctrl Pts',(20.2134201905368,0.846703066048316,40.0247016366783));
#37892=CARTESIAN_POINT('Ctrl Pts',(20.3808766483001,0.858992780802981,39.9986703579415));
#37893=CARTESIAN_POINT('Ctrl Pts',(20.5792177119029,0.873336611371616,39.9405134148323));
#37894=CARTESIAN_POINT('Ctrl Pts',(20.6153149072154,0.875933970052457,39.9287621010812));
#37895=CARTESIAN_POINT('Ctrl Pts',(20.65816279416,0.878982612702795,39.9134005276838));
#37896=CARTESIAN_POINT('Ctrl Pts',(20.6652660212754,0.879486853049573,39.9108066884641));
#37897=CARTESIAN_POINT('Ctrl Pts',(20.67627343415,0.880266241686463,39.9067136700572));
#37898=CARTESIAN_POINT('Ctrl Pts',(20.6801882100622,0.880543035806873,39.9052434857994));
#37899=CARTESIAN_POINT('Ctrl Pts',(20.6874327623011,0.881054488765561,39.9024959009012));
#37900=CARTESIAN_POINT('Ctrl Pts',(20.6907637579902,0.881289343208352,39.9012220036757));
#37901=CARTESIAN_POINT('Ctrl Pts',(20.6983003141535,0.881820026355001,39.8983157616005));
#37902=CARTESIAN_POINT('Ctrl Pts',(20.7025036839451,0.882115524078313,39.8966779016372));
#37903=CARTESIAN_POINT('Ctrl Pts',(20.7152398133634,0.883009528429194,39.8916636884429));
#37904=CARTESIAN_POINT('Ctrl Pts',(20.723754414842,0.883605364522005,39.8882411241691));
#37905=CARTESIAN_POINT('Ctrl Pts',(20.7960084593035,0.888648508523762,39.8585969768404));
#37906=CARTESIAN_POINT('Ctrl Pts',(20.8583326581129,0.892912407315166,39.8290344517594));
#37907=CARTESIAN_POINT('Ctrl Pts',(21.0162270894044,0.903820048941298,39.7434920364688));
#37908=CARTESIAN_POINT('Ctrl Pts',(21.108794701564,0.910331683279342,39.6825167892982));
#37909=CARTESIAN_POINT('Ctrl Pts',(21.247491056949,0.920987725348736,39.5729820484525));
#37910=CARTESIAN_POINT('Ctrl Pts',(21.2972119206925,0.925019397247569,39.5293880463665));
#37911=CARTESIAN_POINT('Ctrl Pts',(21.3723055270313,0.931559816666425,39.4563972152351));
#37912=CARTESIAN_POINT('Ctrl Pts',(21.3991985193583,0.934003861492606,39.4286380414267));
#37913=CARTESIAN_POINT('Ctrl Pts',(21.4328130327208,0.937205259956507,39.3917877904446));
#37914=CARTESIAN_POINT('Ctrl Pts',(21.4403147516351,0.937929609547148,39.3834182053455));
#37915=CARTESIAN_POINT('Ctrl Pts',(21.4523581108634,0.939108953592014,39.3697429822542));
#37916=CARTESIAN_POINT('Ctrl Pts',(21.4569449012006,0.939562072951377,39.3644773133267));
#37917=CARTESIAN_POINT('Ctrl Pts',(21.4656882296254,0.940433514392385,39.3543291771277));
#37918=CARTESIAN_POINT('Ctrl Pts',(21.4698492204189,0.940851646005231,39.3494506547402));
#37919=CARTESIAN_POINT('Ctrl Pts',(21.479293127305,0.941808531647759,39.3382657547474));
#37920=CARTESIAN_POINT('Ctrl Pts',(21.4845601507583,0.942347919664299,39.3319461802863));
#37921=CARTESIAN_POINT('Ctrl Pts',(21.4983961657164,0.943780213787,39.3151276235494));
#37922=CARTESIAN_POINT('Ctrl Pts',(21.5068950982176,0.944675896160014,39.3045718567451));
#37923=CARTESIAN_POINT('Ctrl Pts',(21.5731329467551,0.951784841024621,39.2205056108505));
#37924=CARTESIAN_POINT('Ctrl Pts',(21.6255621293883,0.958204267880045,39.1429875795964));
#37925=CARTESIAN_POINT('Ctrl Pts',(21.7516517355951,0.975973155484309,38.9238137003631));
#37926=CARTESIAN_POINT('Ctrl Pts',(21.8137055665971,0.987578793068131,38.7763303791634));
#37927=CARTESIAN_POINT('Ctrl Pts',(21.864757995785,1.00055132173768,38.5950335299302));
#37928=CARTESIAN_POINT('Ctrl Pts',(21.8719769585452,1.00252093295614,38.5669936489798));
#37929=CARTESIAN_POINT('Ctrl Pts',(21.8801437592704,1.00492290312263,38.5320304732669));
#37930=CARTESIAN_POINT('Ctrl Pts',(21.8816884571423,1.00538607316343,38.5252522066387));
#37931=CARTESIAN_POINT('Ctrl Pts',(21.884072273019,1.00611501726964,38.514524458376));
#37932=CARTESIAN_POINT('Ctrl Pts',(21.8849356735058,1.00638213170949,38.5105805207751));
#37933=CARTESIAN_POINT('Ctrl Pts',(21.8865400994027,1.00688438491899,38.5031399081467));
#37934=CARTESIAN_POINT('Ctrl Pts',(21.8872837797117,1.0071196651795,38.4996439256088));
#37935=CARTESIAN_POINT('Ctrl Pts',(21.8889655145265,1.00765749491545,38.4916288333961));
#37936=CARTESIAN_POINT('Ctrl Pts',(21.8898970702666,1.00795967389074,38.4871084126011));
#37937=CARTESIAN_POINT('Ctrl Pts',(21.892336662193,1.00876269305062,38.4750514446379));
#37938=CARTESIAN_POINT('Ctrl Pts',(21.8938159160968,1.0092619547087,38.4675090609884));
#37939=CARTESIAN_POINT('Ctrl Pts',(21.9043118566782,1.01289890629662,38.4122458399231));
#37940=CARTESIAN_POINT('Ctrl Pts',(21.9115695930745,1.01594549089061,38.3642039177265));
#37941=CARTESIAN_POINT('Ctrl Pts',(21.9183505489168,1.01967728866055,38.3040045745128));
#37942=CARTESIAN_POINT('Ctrl Pts',(21.9195830202224,1.02041344054866,38.2920617938659));
#37943=CARTESIAN_POINT('Ctrl Pts',(21.9221052624138,1.02206349234712,38.2651641665881));
#37944=CARTESIAN_POINT('Ctrl Pts',(21.9233321530883,1.022975732715,38.2502041447357));
#37945=CARTESIAN_POINT('Ctrl Pts',(21.9360555465332,1.03396548389485,38.0691459421283));
#37946=CARTESIAN_POINT('Ctrl Pts',(21.9261779276229,1.04364714775701,37.902256663981));
#37947=CARTESIAN_POINT('Ctrl Pts',(21.8869798655989,1.05667509858616,37.6966621105194));
#37948=CARTESIAN_POINT('Ctrl Pts',(21.8775675320878,1.05937589815297,37.6548997920163));
#37949=CARTESIAN_POINT('Ctrl Pts',(21.8638423032375,1.0628668092626,37.6022353652431));
#37950=CARTESIAN_POINT('Ctrl Pts',(21.8608082343969,1.06361582274127,37.5910103457486));
#37951=CARTESIAN_POINT('Ctrl Pts',(21.8557684021907,1.06482505419686,37.5730122579171));
#37952=CARTESIAN_POINT('Ctrl Pts',(21.8538265605983,1.06528320764849,37.5662214654952));
#37953=CARTESIAN_POINT('Ctrl Pts',(21.8500597299149,1.06615752388676,37.5533170402039));
#37954=CARTESIAN_POINT('Ctrl Pts',(21.8482416139508,1.06657345907108,37.5472014855224));
#37955=CARTESIAN_POINT('Ctrl Pts',(21.8440241549386,1.06752474309475,37.533268725194));
#37956=CARTESIAN_POINT('Ctrl Pts',(21.8416053913345,1.06806071696698,37.525457572517));
#37957=CARTESIAN_POINT('Ctrl Pts',(21.8351802944888,1.06946009850651,37.5051658578971));
#37958=CARTESIAN_POINT('Ctrl Pts',(21.8310963443489,1.07032602107947,37.492710502936));
#37959=CARTESIAN_POINT('Ctrl Pts',(21.801802083034,1.07637953703526,37.4063508155474));
#37960=CARTESIAN_POINT('Ctrl Pts',(21.7722551273496,1.08170917872181,37.3340046641784));
#37961=CARTESIAN_POINT('Ctrl Pts',(21.6665824691851,1.09871027612872,37.1143555258832));
#37962=CARTESIAN_POINT('Ctrl Pts',(21.5758306126613,1.11077888950312,36.9749475707211));
#37963=CARTESIAN_POINT('Ctrl Pts',(21.4439390251137,1.12489334092605,36.8201545880476));
#37964=CARTESIAN_POINT('Ctrl Pts',(21.4186473943562,1.12747398346793,36.7921757680144));
#37965=CARTESIAN_POINT('Ctrl Pts',(21.3873440277018,1.13050364960865,36.7595240797643));
#37966=CARTESIAN_POINT('Ctrl Pts',(21.3821063372239,1.1310052850008,36.7541243663983));
#37967=CARTESIAN_POINT('Ctrl Pts',(21.3739230311748,1.13178067156206,36.7457860695225));
#37968=CARTESIAN_POINT('Ctrl Pts',(21.3709993403181,1.13205606075559,36.7428262179251));
#37969=CARTESIAN_POINT('Ctrl Pts',(21.3655588450559,1.1325654468632,36.737353955167));
#37970=CARTESIAN_POINT('Ctrl Pts',(21.3630446924697,1.1327996348585,36.7348390682933));
#37971=CARTESIAN_POINT('Ctrl Pts',(21.3573303355864,1.13332920121472,36.7291545660522));
#37972=CARTESIAN_POINT('Ctrl Pts',(21.3541259813858,1.13362424720658,36.7259892026511));
#37973=CARTESIAN_POINT('Ctrl Pts',(21.3443734919628,1.13451655867876,36.716422635718));
#37974=CARTESIAN_POINT('Ctrl Pts',(21.3377907227284,1.13511116180941,36.7100566921425));
#37975=CARTESIAN_POINT('Ctrl Pts',(21.2517062529015,1.14279172802983,36.6279858393434));
#37976=CARTESIAN_POINT('Ctrl Pts',(21.1659154650618,1.1494057570229,36.5591421675447));
#37977=CARTESIAN_POINT('Ctrl Pts',(21.0049569339048,1.1610022196217,36.4511636110249));
#37978=CARTESIAN_POINT('Ctrl Pts',(20.9322112546202,1.16598993992046,36.4089702550115));
#37979=CARTESIAN_POINT('Ctrl Pts',(20.7873145392698,1.17579597998761,36.3371274997301));
#37980=CARTESIAN_POINT('Ctrl Pts',(20.7156642217301,1.18058974441858,36.3068446062097));
#37981=CARTESIAN_POINT('Ctrl Pts',(20.6244491535183,1.18673977146044,36.2746321574692));
#37982=CARTESIAN_POINT('Ctrl Pts',(20.6064177683034,1.18795749820621,36.268562871661));
#37983=CARTESIAN_POINT('Ctrl Pts',(20.5801307918007,1.18973690232629,36.2601455489157));
#37984=CARTESIAN_POINT('Ctrl Pts',(20.5719442699373,1.19029163574229,36.2575842258181));
#37985=CARTESIAN_POINT('Ctrl Pts',(20.5575792945976,1.19126615697577,36.2531948128539));
#37986=CARTESIAN_POINT('Ctrl Pts',(20.5514082131198,1.19168516518386,36.2513429063608));
#37987=CARTESIAN_POINT('Ctrl Pts',(20.5394180026662,1.19250003474943,36.2478100901195));
#37988=CARTESIAN_POINT('Ctrl Pts',(20.5335999996139,1.19289577469736,36.2461256021853));
#37989=CARTESIAN_POINT('Ctrl Pts',(20.5196853622553,1.1938431070439,36.242167821334));
#37990=CARTESIAN_POINT('Ctrl Pts',(20.5115816613939,1.19439551454689,36.2399200340369));
#37991=CARTESIAN_POINT('Ctrl Pts',(20.4823193943168,1.19639290432491,36.2320090166902));
#37992=CARTESIAN_POINT('Ctrl Pts',(20.4610801117618,1.19784768074824,36.2266534288626));
#37993=CARTESIAN_POINT('Ctrl Pts',(20.2939809623087,1.20933667846055,36.1875323367276));
#37994=CARTESIAN_POINT('Ctrl Pts',(20.1447568125222,1.21991551290703,36.1704959383719));
#37995=CARTESIAN_POINT('Ctrl Pts',(19.9115029081894,1.23655862434039,36.1710886469682));
#37996=CARTESIAN_POINT('Ctrl Pts',(19.8280048581693,1.24252374294072,36.1767345175105));
#37997=CARTESIAN_POINT('Ctrl Pts',(19.7092569851297,1.25082747417029,36.1925616790356));
#37998=CARTESIAN_POINT('Ctrl Pts',(19.6735205398377,1.25330204619476,36.1983522867459));
#37999=CARTESIAN_POINT('Ctrl Pts',(19.6306543875835,1.25622455230929,36.2065423744961));
#38000=CARTESIAN_POINT('Ctrl Pts',(19.6233512429974,1.25672084510487,36.2079815859043));
#38001=CARTESIAN_POINT('Ctrl Pts',(19.6119922777559,1.25749004304902,36.2102884444262));
#38002=CARTESIAN_POINT('Ctrl Pts',(19.6079307133826,1.25776453970295,36.2111269415111));
#38003=CARTESIAN_POINT('Ctrl Pts',(19.6003871733627,1.25827331546823,36.212709661152));
#38004=CARTESIAN_POINT('Ctrl Pts',(19.5969045848095,1.25850777947081,36.2134504191743));
#38005=CARTESIAN_POINT('Ctrl Pts',(19.588993945551,1.25903942215689,36.2151559434509));
#38006=CARTESIAN_POINT('Ctrl Pts',(19.5845672387149,1.25933625923392,36.2161266719367));
#38007=CARTESIAN_POINT('Ctrl Pts',(19.5710707273061,1.26023936668985,36.2191361951521));
#38008=CARTESIAN_POINT('Ctrl Pts',(19.5620120387085,1.26084287958441,36.2212249928441));
#38009=CARTESIAN_POINT('Ctrl Pts',(19.4993892157924,1.26499889368438,36.2361424283669));
#38010=CARTESIAN_POINT('Ctrl Pts',(19.4463857933544,1.26843511091169,36.2511932508716));
#38011=CARTESIAN_POINT('Ctrl Pts',(19.3941039987112,1.2718084690693,36.2684889865135));
#38012=CARTESIAN_POINT('Origin',(20.,-1.3495818343519,38.1));
#38013=CARTESIAN_POINT('',(19.3941044697279,2.2350068401775,36.268488830693));
#38014=CARTESIAN_POINT('',(19.3941040086996,2.0626282966298,36.2684889832092));
#38015=CARTESIAN_POINT('',(19.3941040087494,-1.3495818343519,36.2684889831927));
#38016=CARTESIAN_POINT('',(18.0708707501997,1.59958183435189,38.1017013127004));
#38017=CARTESIAN_POINT('Ctrl Pts',(19.3941044697278,2.2350068401775,36.268488830693));
#38018=CARTESIAN_POINT('Ctrl Pts',(19.4507932707691,2.2314404515271,36.2497351961299));
#38019=CARTESIAN_POINT('Ctrl Pts',(19.5083755801345,2.22787598191983,36.2336059050976));
#38020=CARTESIAN_POINT('Ctrl Pts',(19.6569378025591,2.21866594071238,36.1993601201359));
#38021=CARTESIAN_POINT('Ctrl Pts',(19.7485745867547,2.21296672935016,36.1850834272658));
#38022=CARTESIAN_POINT('Ctrl Pts',(19.8543542171333,2.20618824044174,36.1763283007706));
#38023=CARTESIAN_POINT('Ctrl Pts',(19.8678448657718,2.20532023007072,36.1753544466455));
#38024=CARTESIAN_POINT('Ctrl Pts',(19.8895458458601,2.20391782389648,36.1740171453559));
#38025=CARTESIAN_POINT('Ctrl Pts',(19.8977503612361,2.20338620896967,36.1735641499162));
#38026=CARTESIAN_POINT('Ctrl Pts',(19.9123580233041,2.20243709349871,36.1728511977098));
#38027=CARTESIAN_POINT('Ctrl Pts',(19.9187600810145,2.20202023727746,36.1725707026816));
#38028=CARTESIAN_POINT('Ctrl Pts',(19.932141008767,2.20114705455525,36.1720512259766));
#38029=CARTESIAN_POINT('Ctrl Pts',(19.9391200049021,2.20069054826806,36.1718182290058));
#38030=CARTESIAN_POINT('Ctrl Pts',(19.9573427794452,2.19949565762935,36.1713088851594));
#38031=CARTESIAN_POINT('Ctrl Pts',(19.9685878496746,2.1987554089788,36.171092971994));
#38032=CARTESIAN_POINT('Ctrl Pts',(20.0185830385412,2.19545096404046,36.170570322036));
#38033=CARTESIAN_POINT('Ctrl Pts',(20.0573329530689,2.19285393954807,36.171332901201));
#38034=CARTESIAN_POINT('Ctrl Pts',(20.1623034239754,2.18571604444189,36.1765647789792));
#38035=CARTESIAN_POINT('Ctrl Pts',(20.2283544184992,2.18111181523569,36.1832845404902));
#38036=CARTESIAN_POINT('Ctrl Pts',(20.4101714268752,2.16815884595209,36.2113134340679));
#38037=CARTESIAN_POINT('Ctrl Pts',(20.5245315418614,2.15967931616343,36.2398272994171));
#38038=CARTESIAN_POINT('Ctrl Pts',(20.6490561115131,2.15037989891157,36.2832797552791));
#38039=CARTESIAN_POINT('Ctrl Pts',(20.6624801357608,2.14937679889695,36.2881318016347));
#38040=CARTESIAN_POINT('Ctrl Pts',(20.7212649547765,2.1449846921599,36.3101199545975));
#38041=CARTESIAN_POINT('Ctrl Pts',(20.7660285439669,2.14164128144961,36.3288153998273));
#38042=CARTESIAN_POINT('Ctrl Pts',(20.81702038343,2.13787068345194,36.3524075590737));
#38043=CARTESIAN_POINT('Ctrl Pts',(20.8239776408362,2.1373570747388,36.355677065808));
#38044=CARTESIAN_POINT('Ctrl Pts',(20.8350826227637,2.13653884151751,36.360977029408));
#38045=CARTESIAN_POINT('Ctrl Pts',(20.8392428352544,2.13623266628363,36.3629809029084));
#38046=CARTESIAN_POINT('Ctrl Pts',(20.8466122196426,2.13569099391951,36.3665632126058));
#38047=CARTESIAN_POINT('Ctrl Pts',(20.8498242436171,2.13545513439346,36.3681356571261));
#38048=CARTESIAN_POINT('Ctrl Pts',(20.8566546760643,2.13495408795059,36.3715030700618));
#38049=CARTESIAN_POINT('Ctrl Pts',(20.8602718203646,2.13468905424524,36.3733004700711));
#38050=CARTESIAN_POINT('Ctrl Pts',(20.8701047460266,2.13396933174123,36.3782251301066));
#38051=CARTESIAN_POINT('Ctrl Pts',(20.8763093707476,2.13351600313624,36.3813747173965));
#38052=CARTESIAN_POINT('Ctrl Pts',(20.9083037157767,2.13118194764366,36.3978339793025));
#38053=CARTESIAN_POINT('Ctrl Pts',(20.9338093302124,2.12933321831063,36.4116916285343));
#38054=CARTESIAN_POINT('Ctrl Pts',(21.097610775992,2.11747521889453,36.5055362700835));
#38055=CARTESIAN_POINT('Ctrl Pts',(21.2258408462013,2.10821859579922,36.6018709974587));
#38056=CARTESIAN_POINT('Ctrl Pts',(21.4074414563538,2.09296175578713,36.7774046579686));
#38057=CARTESIAN_POINT('Ctrl Pts',(21.4694020364037,2.08725421997025,36.8466029641151));
#38058=CARTESIAN_POINT('Ctrl Pts',(21.5344156480109,2.08046649715671,36.9306864352825));
#38059=CARTESIAN_POINT('Ctrl Pts',(21.5425781792487,2.07959826908749,36.9414758787773));
#38060=CARTESIAN_POINT('Ctrl Pts',(21.5555153509736,2.07819557842961,36.9589557036772));
#38061=CARTESIAN_POINT('Ctrl Pts',(21.5603619919794,2.07766389854119,36.9655924260498));
#38062=CARTESIAN_POINT('Ctrl Pts',(21.5689122600384,2.07671470826916,36.9774591568571));
#38063=CARTESIAN_POINT('Ctrl Pts',(21.5726325324638,2.07629784256363,36.9826770652986));
#38064=CARTESIAN_POINT('Ctrl Pts',(21.5803518669238,2.0754246820855,36.9936188324199));
#38065=CARTESIAN_POINT('Ctrl Pts',(21.5843459827438,2.07496820773579,36.9993460507146));
#38066=CARTESIAN_POINT('Ctrl Pts',(21.59469109849,2.07377349443919,37.0143530473067));
#38067=CARTESIAN_POINT('Ctrl Pts',(21.6009921333417,2.07303339222261,37.0236667869904));
#38068=CARTESIAN_POINT('Ctrl Pts',(21.6286316927265,2.06973055181848,37.0653013372799));
#38069=CARTESIAN_POINT('Ctrl Pts',(21.6490741740066,2.06713502475511,37.0982033557684));
#38070=CARTESIAN_POINT('Ctrl Pts',(21.7017897352187,2.06000246433147,37.1890390361639));
#38071=CARTESIAN_POINT('Ctrl Pts',(21.7320865344145,2.05540219003107,37.2480534855265));
#38072=CARTESIAN_POINT('Ctrl Pts',(21.7856966813067,2.04620233643336,37.3672146369147));
#38073=CARTESIAN_POINT('Ctrl Pts',(21.8091535209082,2.04161238838394,37.4272073576387));
#38074=CARTESIAN_POINT('Ctrl Pts',(21.8633663487556,2.02941308867271,37.5893442381055));
#38075=CARTESIAN_POINT('Ctrl Pts',(21.8887337073943,2.0218109901199,37.6930686912955));
#38076=CARTESIAN_POINT('Ctrl Pts',(21.9077191548918,2.013577731312,37.8129988745062));
#38077=CARTESIAN_POINT('Ctrl Pts',(21.9098669394027,2.0125808918645,37.8276577033432));
#38078=CARTESIAN_POINT('Ctrl Pts',(21.9125991992918,2.01121664867235,37.8479311901059));
#38079=CARTESIAN_POINT('Ctrl Pts',(21.9133281606586,2.01084171467088,37.8535253894243));
#38080=CARTESIAN_POINT('Ctrl Pts',(21.9144539713393,2.01024464933028,37.8624711852676));
#38081=CARTESIAN_POINT('Ctrl Pts',(21.9148665768341,2.01002165268001,37.8658207106375));
#38082=CARTESIAN_POINT('Ctrl Pts',(21.9157070536717,2.00955855915947,37.8727944562693));
#38083=CARTESIAN_POINT('Ctrl Pts',(21.9161334325785,2.00931855246834,37.8764188214585));
#38084=CARTESIAN_POINT('Ctrl Pts',(21.9171374437943,2.00874081014297,37.885167119784));
#38085=CARTESIAN_POINT('Ctrl Pts',(21.917704827661,2.00840364385596,37.8902922502798));
#38086=CARTESIAN_POINT('Ctrl Pts',(21.9196075787314,2.00723425761653,37.9081334344469));
#38087=CARTESIAN_POINT('Ctrl Pts',(21.9208371082332,2.0064077002014,37.9208607801551));
#38088=CARTESIAN_POINT('Ctrl Pts',(21.9273685714265,2.00154867294746,37.9962998842796));
#38089=CARTESIAN_POINT('Ctrl Pts',(21.9297262076623,1.9976590302256,38.0592350121007));
#38090=CARTESIAN_POINT('Ctrl Pts',(21.9280292278797,1.98869101391914,38.2068288926908));
#38091=CARTESIAN_POINT('Ctrl Pts',(21.9214849962555,1.98367277918552,38.2913257055998));
#38092=CARTESIAN_POINT('Ctrl Pts',(21.9040617944663,1.97636140845724,38.4122469062855));
#38093=CARTESIAN_POINT('Ctrl Pts',(21.8976310379399,1.97410943440645,38.4492073559744));
#38094=CARTESIAN_POINT('Ctrl Pts',(21.8726351533664,1.96654513500071,38.5716186951708));
#38095=CARTESIAN_POINT('Ctrl Pts',(21.8493422911781,1.96115271786269,38.6559826809058));
#38096=CARTESIAN_POINT('Ctrl Pts',(21.8159700956865,1.95471227839766,38.7511338384985));
#38097=CARTESIAN_POINT('Ctrl Pts',(21.8113965090545,1.95385093304808,38.7637509596665));
#38098=CARTESIAN_POINT('Ctrl Pts',(21.8038218761256,1.9524572270829,38.7839855310286));
#38099=CARTESIAN_POINT('Ctrl Pts',(21.8009032783104,1.95192759154989,38.7916335346268));
#38100=CARTESIAN_POINT('Ctrl Pts',(21.7956149040682,1.95098073664984,38.8052309422904));
#38101=CARTESIAN_POINT('Ctrl Pts',(21.7932639991833,1.95056415068805,38.8111875935802));
#38102=CARTESIAN_POINT('Ctrl Pts',(21.7882820050351,1.94969022556804,38.8236290500042));
#38103=CARTESIAN_POINT('Ctrl Pts',(21.7856452042971,1.94923270010994,38.8301114529622));
#38104=CARTESIAN_POINT('Ctrl Pts',(21.778652424007,1.94803221223502,38.8470382659769));
#38105=CARTESIAN_POINT('Ctrl Pts',(21.774239763459,1.94728735315036,38.8574588231719));
#38106=CARTESIAN_POINT('Ctrl Pts',(21.7540358815899,1.94393217260906,38.9040252209428));
#38107=CARTESIAN_POINT('Ctrl Pts',(21.7372309517583,1.94128776839284,38.9397182052802));
#38108=CARTESIAN_POINT('Ctrl Pts',(21.644890692471,1.92745172903296,39.1211908134855));
#38109=CARTESIAN_POINT('Ctrl Pts',(21.5520706900964,1.9156531798475,39.2573913118662));
#38110=CARTESIAN_POINT('Ctrl Pts',(21.3896674349672,1.8982745223557,39.4404719560063));
#38111=CARTESIAN_POINT('Ctrl Pts',(21.3324400903879,1.89261746114329,39.4973715463614));
#38112=CARTESIAN_POINT('Ctrl Pts',(21.2647991758318,1.8865714887543,39.5566786271996));
#38113=CARTESIAN_POINT('Ctrl Pts',(21.2577402972361,1.88594783549258,39.5627778134152));
#38114=CARTESIAN_POINT('Ctrl Pts',(21.2471822112282,1.88502615799459,39.5717675362585));
#38115=CARTESIAN_POINT('Ctrl Pts',(21.2437167279855,1.88472539649303,39.5746972063317));
#38116=CARTESIAN_POINT('Ctrl Pts',(21.2375142213121,1.88419027803698,39.5799033014332));
#38117=CARTESIAN_POINT('Ctrl Pts',(21.2347812112329,1.88395558612682,39.5821843983272));
#38118=CARTESIAN_POINT('Ctrl Pts',(21.2288563438598,1.88344917494439,39.5871018056004));
#38119=CARTESIAN_POINT('Ctrl Pts',(21.2256623176153,1.88317764993617,39.5897354053787));
#38120=CARTESIAN_POINT('Ctrl Pts',(21.2167227241839,1.88242172028747,39.5970582382639));
#38121=CARTESIAN_POINT('Ctrl Pts',(21.2109584816305,1.88193891551266,39.601724713925));
#38122=CARTESIAN_POINT('Ctrl Pts',(21.1772248881182,1.87913925505379,39.6287134030862));
#38123=CARTESIAN_POINT('Ctrl Pts',(21.1486636073784,1.87687154210921,39.6502888177987));
#38124=CARTESIAN_POINT('Ctrl Pts',(21.0527748065696,1.86952836687475,39.7186179579998));
#38125=CARTESIAN_POINT('Ctrl Pts',(20.9830645237154,1.86460965496047,39.761880042975));
#38126=CARTESIAN_POINT('Ctrl Pts',(20.7767106452603,1.85061531469911,39.8724005276207));
#38127=CARTESIAN_POINT('Ctrl Pts',(20.6346065649354,1.84159165283577,39.9281004588631));
#38128=CARTESIAN_POINT('Ctrl Pts',(20.4663691426416,1.83057383749607,39.9720354583529));
#38129=CARTESIAN_POINT('Ctrl Pts',(20.4452046962944,1.8291831386634,39.9771813050127));
#38130=CARTESIAN_POINT('Ctrl Pts',(20.4157749063247,1.8272410304509,39.9838110709465));
#38131=CARTESIAN_POINT('Ctrl Pts',(20.4075796596619,1.82669933387507,39.9856011617371));
#38132=CARTESIAN_POINT('Ctrl Pts',(20.3934542282003,1.82576403053848,39.9885901961467));
#38133=CARTESIAN_POINT('Ctrl Pts',(20.3875295508042,1.82537124185823,39.989814806943));
#38134=CARTESIAN_POINT('Ctrl Pts',(20.3752834750821,1.82455830403695,39.9922860206138));
#38135=CARTESIAN_POINT('Ctrl Pts',(20.368961403357,1.82413804138893,39.9935288621059));
#38136=CARTESIAN_POINT('Ctrl Pts',(20.3541954083266,1.82315505378918,39.9963549180992));
#38137=CARTESIAN_POINT('Ctrl Pts',(20.3457469527733,1.82259155677552,39.9979134340911));
#38138=CARTESIAN_POINT('Ctrl Pts',(20.3184745667366,1.82076891427311,40.002756324953));
#38139=CARTESIAN_POINT('Ctrl Pts',(20.2996126491822,1.81950278697212,40.0058173831284));
#38140=CARTESIAN_POINT('Ctrl Pts',(20.2553120899749,1.81651509168533,40.0123329326847));
#38141=CARTESIAN_POINT('Ctrl Pts',(20.2298442977432,1.81478674540491,40.015560753924));
#38142=CARTESIAN_POINT('Ctrl Pts',(20.1382329002551,1.80852957207585,40.0253185101236));
#38143=CARTESIAN_POINT('Ctrl Pts',(20.0718320083648,1.80391760089509,40.0289370902873));
#38144=CARTESIAN_POINT('Ctrl Pts',(19.8583148939675,1.78888284249018,40.0295328244532));
#38145=CARTESIAN_POINT('Ctrl Pts',(19.7116896374633,1.77820835032208,40.0131250442843));
#38146=CARTESIAN_POINT('Ctrl Pts',(19.5346473595094,1.7656275994403,39.9724811158433));
#38147=CARTESIAN_POINT('Ctrl Pts',(19.5011517467772,1.76326395740075,39.963837276327));
#38148=CARTESIAN_POINT('Ctrl Pts',(19.4612129796655,1.76047983247138,39.9523767337198));
#38149=CARTESIAN_POINT('Ctrl Pts',(19.454532011864,1.76001526768932,39.9504204101872));
#38150=CARTESIAN_POINT('Ctrl Pts',(19.4435992758105,1.75925712987044,39.9471547255062));
#38151=CARTESIAN_POINT('Ctrl Pts',(19.4393412581086,1.75896237286127,39.945866767122));
#38152=CARTESIAN_POINT('Ctrl Pts',(19.4316896738131,1.75843368004899,39.9435234089884));
#38153=CARTESIAN_POINT('Ctrl Pts',(19.4282945531312,1.75819944275547,39.9424733563879));
#38154=CARTESIAN_POINT('Ctrl Pts',(19.4208859263506,1.75768907522686,39.9401595449769));
#38155=CARTESIAN_POINT('Ctrl Pts',(19.4168736566528,1.75741316589101,39.9388920386466));
#38156=CARTESIAN_POINT('Ctrl Pts',(19.4055024901755,1.75663251525043,39.9352588418082));
#38157=CARTESIAN_POINT('Ctrl Pts',(19.3981535163404,1.75612954736795,39.932862002616));
#38158=CARTESIAN_POINT('Ctrl Pts',(19.3517824133652,1.75296453728294,39.9174292716258));
#38159=CARTESIAN_POINT('Ctrl Pts',(19.3131680109094,1.75036775200969,39.9031909485795));
#38160=CARTESIAN_POINT('Ctrl Pts',(19.176510405672,1.74121850229434,39.8477731408484));
#38161=CARTESIAN_POINT('Ctrl Pts',(19.0814488912306,1.73492344634107,39.7997392821798));
#38162=CARTESIAN_POINT('Ctrl Pts',(18.8864954628419,1.72124977208803,39.6800745261758));
#38163=CARTESIAN_POINT('Ctrl Pts',(18.7885128372743,1.71387227086999,39.6062607038128));
#38164=CARTESIAN_POINT('Ctrl Pts',(18.6824368869388,1.70476036202682,39.5092642079091));
#38165=CARTESIAN_POINT('Ctrl Pts',(18.666925296935,1.70339704031627,39.4946002807627));
#38166=CARTESIAN_POINT('Ctrl Pts',(18.6457115427248,1.70148720166272,39.4738684530208));
#38167=CARTESIAN_POINT('Ctrl Pts',(18.6398001441199,1.70094997472317,39.4680161184109));
#38168=CARTESIAN_POINT('Ctrl Pts',(18.6296679879405,1.70002031813664,39.4578546000221));
#38169=CARTESIAN_POINT('Ctrl Pts',(18.6254292166203,1.69962868366398,39.4535634814019));
#38170=CARTESIAN_POINT('Ctrl Pts',(18.6166968051763,1.69881617665422,39.4446399071986));
#38171=CARTESIAN_POINT('Ctrl Pts',(18.6122061539806,1.69839518194164,39.4400046448047));
#38172=CARTESIAN_POINT('Ctrl Pts',(18.6033516113706,1.69755872814182,39.4307727107335));
#38173=CARTESIAN_POINT('Ctrl Pts',(18.5989869453034,1.69714331013189,39.4261768916887));
#38174=CARTESIAN_POINT('Ctrl Pts',(18.5847326670758,1.69577630940671,39.4110188019155));
#38175=CARTESIAN_POINT('Ctrl Pts',(18.574939426932,1.69482066243933,39.4003669737457));
#38176=CARTESIAN_POINT('Ctrl Pts',(18.5130762733828,1.68867606895716,39.3315420129649));
#38177=CARTESIAN_POINT('Ctrl Pts',(18.4644652030882,1.68334621637136,39.2703708585176));
#38178=CARTESIAN_POINT('Ctrl Pts',(18.3815354524825,1.67325979233464,39.1519232211013));
#38179=CARTESIAN_POINT('Ctrl Pts',(18.3462208478869,1.66854230017805,39.0954815180123));
#38180=CARTESIAN_POINT('Ctrl Pts',(18.2860631393927,1.65971710801372,38.9872677129937));
#38181=CARTESIAN_POINT('Ctrl Pts',(18.260475091997,1.65562055226872,38.9359885036831));
#38182=CARTESIAN_POINT('Ctrl Pts',(18.2345792689278,1.65110013482322,38.8777364774162));
#38183=CARTESIAN_POINT('Ctrl Pts',(18.2319817614508,1.65064200493078,38.8718133810185));
#38184=CARTESIAN_POINT('Ctrl Pts',(18.2017566778354,1.64525583950333,38.8019378179573));
#38185=CARTESIAN_POINT('Ctrl Pts',(18.17757967331,1.64039450091763,38.7365392125818));
#38186=CARTESIAN_POINT('Ctrl Pts',(18.1542737854331,1.63509422561632,38.6611790690177));
#38187=CARTESIAN_POINT('Ctrl Pts',(18.1516183030349,1.63447923158132,38.6523697287277));
#38188=CARTESIAN_POINT('Ctrl Pts',(18.147754475172,1.63356783121536,38.6392118646773));
#38189=CARTESIAN_POINT('Ctrl Pts',(18.1464982455233,1.63326877405658,38.6348777116633));
#38190=CARTESIAN_POINT('Ctrl Pts',(18.1442787528356,1.6327354971082,38.6271184574297));
#38191=CARTESIAN_POINT('Ctrl Pts',(18.1433097497119,1.63250095182484,38.62369507399));
#38192=CARTESIAN_POINT('Ctrl Pts',(18.1412288149985,1.63199349800191,38.6162649783913));
#38193=CARTESIAN_POINT('Ctrl Pts',(18.1401203671355,1.63172079098415,38.6122573554059));
#38194=CARTESIAN_POINT('Ctrl Pts',(18.1370488062906,1.63095821055714,38.6010106425219));
#38195=CARTESIAN_POINT('Ctrl Pts',(18.1351149148659,1.63046998295604,38.5937635444221));
#38196=CARTESIAN_POINT('Ctrl Pts',(18.1308728542652,1.6293800978456,38.5774862677129));
#38197=CARTESIAN_POINT('Ctrl Pts',(18.1285877430864,1.62877966754483,38.5684502059073));
#38198=CARTESIAN_POINT('Ctrl Pts',(18.0896410123783,1.61829974201645,38.4096078135587));
#38199=CARTESIAN_POINT('Ctrl Pts',(18.0710045347108,1.60929535803221,38.255936396569));
#38200=CARTESIAN_POINT('Ctrl Pts',(18.0708707257347,1.60004847844167,38.1016733417687));
#38201=CARTESIAN_POINT('Ctrl Pts',(19.3941040087494,1.44151754323334,36.2684889831927));
#38202=CARTESIAN_POINT('Ctrl Pts',(19.3295043521928,1.44595990632178,36.2898596834422));
#38203=CARTESIAN_POINT('Ctrl Pts',(19.2660284166685,1.45040226941022,36.3146550158227));
#38204=CARTESIAN_POINT('Ctrl Pts',(19.2040563963221,1.45484463249867,36.3427247407807));
#38205=CARTESIAN_POINT('Ctrl Pts',(19.1415298209384,1.45932674795946,36.3710456469537));
#38206=CARTESIAN_POINT('Ctrl Pts',(19.0805346871417,1.46380886342026,36.4026996559877));
#38207=CARTESIAN_POINT('Ctrl Pts',(19.0214381046462,1.46829097888105,36.4374840831254));
#38208=CARTESIAN_POINT('Ctrl Pts',(18.962786240726,1.47273936514943,36.4720067475649));
#38209=CARTESIAN_POINT('Ctrl Pts',(18.9060048339152,1.47718775141779,36.5096125497364));
#38210=CARTESIAN_POINT('Ctrl Pts',(18.8514234687525,1.48163613768617,36.5500598370365));
#38211=CARTESIAN_POINT('Ctrl Pts',(18.796221321606,1.48613511774317,36.5909671521716));
#38212=CARTESIAN_POINT('Ctrl Pts',(18.7432699822867,1.49063409780018,36.6347806741961));
#38213=CARTESIAN_POINT('Ctrl Pts',(18.6928740704282,1.49513307785719,36.6812102477318));
#38214=CARTESIAN_POINT('Ctrl Pts',(18.6424781585697,1.49963205791419,36.7276398212676));
#38215=CARTESIAN_POINT('Ctrl Pts',(18.5946379872075,1.5041310379712,36.7766850326004));
#38216=CARTESIAN_POINT('Ctrl Pts',(18.5496164787244,1.50863001802821,36.8280211487167));
#38217=CARTESIAN_POINT('Ctrl Pts',(18.5054073944355,1.51304781288349,36.8784308919907));
#38218=CARTESIAN_POINT('Ctrl Pts',(18.4637338189911,1.51746560773877,36.9312575117532));
#38219=CARTESIAN_POINT('Ctrl Pts',(18.4248740293338,1.52188340259406,36.9862133357627));
#38220=CARTESIAN_POINT('Ctrl Pts',(18.3860685084149,1.52629502788034,37.04109241249));
#38221=CARTESIAN_POINT('Ctrl Pts',(18.3500692719598,1.53070665316662,37.0980943932937));
#38222=CARTESIAN_POINT('Ctrl Pts',(18.3171157241828,1.5351182784529,37.1568971047086));
#38223=CARTESIAN_POINT('Ctrl Pts',(18.2841963309236,1.53952533133515,37.2156388703864));
#38224=CARTESIAN_POINT('Ctrl Pts',(18.2543166109693,1.5439323842174,37.2761772294216));
#38225=CARTESIAN_POINT('Ctrl Pts',(18.2276727115185,1.54833943709965,37.3381610804088));
#38226=CARTESIAN_POINT('Ctrl Pts',(18.2010410830137,1.55274446029748,37.4001163845053));
#38227=CARTESIAN_POINT('Ctrl Pts',(18.1776425273966,1.5571494834953,37.4635154036111));
#38228=CARTESIAN_POINT('Ctrl Pts',(18.157626462877,1.56155450669312,37.5279839979432));
#38229=CARTESIAN_POINT('Ctrl Pts',(18.1376167710586,1.56595812742263,37.5924320668078));
#38230=CARTESIAN_POINT('Ctrl Pts',(18.1209875777404,1.57036174815214,37.6579485535264));
#38231=CARTESIAN_POINT('Ctrl Pts',(18.1078387655014,1.57476536888165,37.7241430863206));
#38232=CARTESIAN_POINT('Ctrl Pts',(18.0946818547531,1.57917170185332,37.7903783891114));
#38233=CARTESIAN_POINT('Ctrl Pts',(18.0850097061681,1.58357803482498,37.8572920782553));
#38234=CARTESIAN_POINT('Ctrl Pts',(18.0788710086126,1.58798436779665,37.9244837461924));
#38235=CARTESIAN_POINT('Ctrl Pts',(18.0734853254718,1.59185018998173,37.9834332269135));
#38236=CARTESIAN_POINT('Ctrl Pts',(18.0708186250899,1.59571601216681,38.0425963204681));
#38237=CARTESIAN_POINT('Ctrl Pts',(18.0708707501997,1.59958183435189,38.1017013127004));
#38238=CARTESIAN_POINT('Ctrl Pts',(19.3941039987112,1.2718084690693,36.2684889865135));
#38239=CARTESIAN_POINT('Ctrl Pts',(19.3729704333272,1.27317206199249,36.2754803410098));
#38240=CARTESIAN_POINT('Ctrl Pts',(19.3519547771375,1.27452534683923,36.2828385068952));
#38241=CARTESIAN_POINT('Ctrl Pts',(19.2353762315221,1.28204040096756,36.325936541027));
#38242=CARTESIAN_POINT('Ctrl Pts',(19.1426419244413,1.28805758975417,36.3688476111492));
#38243=CARTESIAN_POINT('Ctrl Pts',(18.9960606939578,1.29819804784758,36.4513555214064));
#38244=CARTESIAN_POINT('Ctrl Pts',(18.9400997606449,1.30223503154551,36.4867631523017));
#38245=CARTESIAN_POINT('Ctrl Pts',(18.8544898325454,1.3087833623047,36.5473102870164));
#38246=CARTESIAN_POINT('Ctrl Pts',(18.8235886346127,1.31122973923878,36.5705900276741));
#38247=CARTESIAN_POINT('Ctrl Pts',(18.7846392504342,1.31443359811905,36.6018120440878));
#38248=CARTESIAN_POINT('Ctrl Pts',(18.7759306338103,1.31515798437925,36.6089188214961));
#38249=CARTESIAN_POINT('Ctrl Pts',(18.7619145414513,1.31633723986449,36.6205623717716));
#38250=CARTESIAN_POINT('Ctrl Pts',(18.7565686311313,1.3167902320251,36.6250526357596));
#38251=CARTESIAN_POINT('Ctrl Pts',(18.7463623132792,1.31766132621961,36.6337202925881));
#38252=CARTESIAN_POINT('Ctrl Pts',(18.7414981096668,1.31807923731729,36.63789308862));
#38253=CARTESIAN_POINT('Ctrl Pts',(18.7304423972041,1.31903547385862,36.6474733651038));
#38254=CARTESIAN_POINT('Ctrl Pts',(18.7242645119804,1.31957443202707,36.6528963088349));
#38255=CARTESIAN_POINT('Ctrl Pts',(18.7080055045157,1.32100527287077,36.6673534892347));
#38256=CARTESIAN_POINT('Ctrl Pts',(18.6979846364914,1.32189992539169,36.6764545042204));
#38257=CARTESIAN_POINT('Ctrl Pts',(18.6198218405995,1.3289811239902,36.7489581842059));
#38258=CARTESIAN_POINT('Ctrl Pts',(18.5562640631192,1.33537206128373,36.8171018831818));
#38259=CARTESIAN_POINT('Ctrl Pts',(18.3977500555834,1.35312131761996,37.013812597373));
#38260=CARTESIAN_POINT('Ctrl Pts',(18.3134311631152,1.36473915158736,37.1500045888991));
#38261=CARTESIAN_POINT('Ctrl Pts',(18.2347590313027,1.37772452529724,37.3213435401196));
#38262=CARTESIAN_POINT('Ctrl Pts',(18.2232659692866,1.37969526278953,37.3479375242969));
#38263=CARTESIAN_POINT('Ctrl Pts',(18.2097614844733,1.38209842981782,37.3812253725997));
#38264=CARTESIAN_POINT('Ctrl Pts',(18.2071822776167,1.38256169758878,37.3876829881169));
#38265=CARTESIAN_POINT('Ctrl Pts',(18.2031605988728,1.38329077114152,37.3979123789754));
#38266=CARTESIAN_POINT('Ctrl Pts',(18.2016949873493,1.38355791769078,37.4016749014544));
#38267=CARTESIAN_POINT('Ctrl Pts',(18.1989536603523,1.38406031978542,37.4087783078228));
#38268=CARTESIAN_POINT('Ctrl Pts',(18.1976754361683,1.38429571638796,37.4121180972454));
#38269=CARTESIAN_POINT('Ctrl Pts',(18.1947676312976,1.38483386531823,37.4197794604327));
#38270=CARTESIAN_POINT('Ctrl Pts',(18.1931442783298,1.38513624670678,37.424103343979));
#38271=CARTESIAN_POINT('Ctrl Pts',(18.1888590532329,1.38593979819903,37.4356430328213));
#38272=CARTESIAN_POINT('Ctrl Pts',(18.1862247447007,1.38643938902646,37.4428690869163));
#38273=CARTESIAN_POINT('Ctrl Pts',(18.1672595705472,1.39007920439081,37.4958745935455));
#38274=CARTESIAN_POINT('Ctrl Pts',(18.1526192543012,1.39312825434638,37.5422453251091));
#38275=CARTESIAN_POINT('Ctrl Pts',(18.1330725053582,1.39767509173209,37.6134209624401));
#38276=CARTESIAN_POINT('Ctrl Pts',(18.1268763229125,1.39921214922491,37.6378472140587));
#38277=CARTESIAN_POINT('Ctrl Pts',(18.0878297021189,1.40964436688018,37.8054898616816));
#38278=CARTESIAN_POINT('Ctrl Pts',(18.0709568775046,1.41821775313881,37.9519275109852));
#38279=CARTESIAN_POINT('Ctrl Pts',(18.0708347172606,1.43096131211979,38.1593364460134));
#38280=CARTESIAN_POINT('Ctrl Pts',(18.0736425407378,1.43474043564055,38.2197719057908));
#38281=CARTESIAN_POINT('Ctrl Pts',(18.0804245816936,1.43939132766768,38.2921521264353));
#38282=CARTESIAN_POINT('Ctrl Pts',(18.0816817258341,1.44017748412289,38.3043213502303));
#38283=CARTESIAN_POINT('Ctrl Pts',(18.083942616572,1.44147814806944,38.3243419198796));
#38284=CARTESIAN_POINT('Ctrl Pts',(18.0848791009267,1.4419905551029,38.3322006297621));
#38285=CARTESIAN_POINT('Ctrl Pts',(18.0866550158689,1.44291731449753,38.3463614160093));
#38286=CARTESIAN_POINT('Ctrl Pts',(18.0874772971379,1.44333112461121,38.3526655596277));
#38287=CARTESIAN_POINT('Ctrl Pts',(18.0893016298007,1.44421780805564,38.3661326864701));
#38288=CARTESIAN_POINT('Ctrl Pts',(18.0903128304379,1.4446909623743,38.373294311514));
#38289=CARTESIAN_POINT('Ctrl Pts',(18.0931640726627,1.44597748389273,38.3926987786005));
#38290=CARTESIAN_POINT('Ctrl Pts',(18.0950817091464,1.44679327318482,38.4049296998816));
#38291=CARTESIAN_POINT('Ctrl Pts',(18.1056612585528,1.45105329528453,38.468408217996));
#38292=CARTESIAN_POINT('Ctrl Pts',(18.1162731819594,1.45455833356645,38.5193045268177));
#38293=CARTESIAN_POINT('Ctrl Pts',(18.1766648431342,1.47157002523195,38.7598744639977));
#38294=CARTESIAN_POINT('Ctrl Pts',(18.2531010698094,1.48591420585538,38.9416098130526));
#38295=CARTESIAN_POINT('Ctrl Pts',(18.3747793559549,1.50206009194551,39.1399746432878));
#38296=CARTESIAN_POINT('Ctrl Pts',(18.3948588477879,1.50457186717874,39.1707061733587));
#38297=CARTESIAN_POINT('Ctrl Pts',(18.4198515539288,1.50750738948235,39.2066723738999));
#38298=CARTESIAN_POINT('Ctrl Pts',(18.4239307876661,1.50798078825759,39.2124741329671));
#38299=CARTESIAN_POINT('Ctrl Pts',(18.4306436305957,1.5087503660928,39.2219105517576));
#38300=CARTESIAN_POINT('Ctrl Pts',(18.433258047894,1.50904778918022,39.2255586865455));
#38301=CARTESIAN_POINT('Ctrl Pts',(18.4379666563443,1.50957930106087,39.2320808430067));
#38302=CARTESIAN_POINT('Ctrl Pts',(18.4400560748509,1.50981370627135,39.2349582163485));
#38303=CARTESIAN_POINT('Ctrl Pts',(18.4446165487979,1.51032218540873,39.2412021360998));
#38304=CARTESIAN_POINT('Ctrl Pts',(18.4470905770178,1.5105960506815,39.2445664334331));
#38305=CARTESIAN_POINT('Ctrl Pts',(18.4540876844341,1.51136513100577,39.2540169708251));
#38306=CARTESIAN_POINT('Ctrl Pts',(18.4586358136344,1.51185865496014,39.260084697769));
#38307=CARTESIAN_POINT('Ctrl Pts',(18.4866157817758,1.51485723981956,39.2969581401084));
#38308=CARTESIAN_POINT('Ctrl Pts',(18.5109364179864,1.51730464163332,39.327082198269));
#38309=CARTESIAN_POINT('Ctrl Pts',(18.6518033981245,1.53075474392431,39.4912011253199));
#38310=CARTESIAN_POINT('Ctrl Pts',(18.7855144180612,1.5409613047013,39.6093414955046));
#38311=CARTESIAN_POINT('Ctrl Pts',(18.9885418136757,1.55587979756541,39.7440364465344));
#38312=CARTESIAN_POINT('Ctrl Pts',(19.0454031862377,1.55999537934415,39.7776909691126));
#38313=CARTESIAN_POINT('Ctrl Pts',(19.1149890050844,1.56502029795779,39.8141924164311));
#38314=CARTESIAN_POINT('Ctrl Pts',(19.1261607057953,1.56582660525961,39.8199142355381));
#38315=CARTESIAN_POINT('Ctrl Pts',(19.1445540069957,1.56715382882963,39.8291092818812));
#38316=CARTESIAN_POINT('Ctrl Pts',(19.1517429361519,1.5676724934482,39.8326473115085));
#38317=CARTESIAN_POINT('Ctrl Pts',(19.1646840285857,1.56860612843992,39.8389164237411));
#38318=CARTESIAN_POINT('Ctrl Pts',(19.1704280988774,1.5690205219728,39.8416640204426));
#38319=CARTESIAN_POINT('Ctrl Pts',(19.1826694018392,1.56990367028045,39.8474451825756));
#38320=CARTESIAN_POINT('Ctrl Pts',(19.1891701412489,1.57037268138688,39.850471053923));
#38321=CARTESIAN_POINT('Ctrl Pts',(19.2066807131758,1.57163614860674,39.8585031543281));
#38322=CARTESIAN_POINT('Ctrl Pts',(19.2177208606355,1.57243288004147,39.8634421372659));
#38323=CARTESIAN_POINT('Ctrl Pts',(19.272992460545,1.57642294459216,39.8875475803889));
#38324=CARTESIAN_POINT('Ctrl Pts',(19.3178815220938,1.57966822717996,39.9051537327229));
#38325=CARTESIAN_POINT('Ctrl Pts',(19.4509857541633,1.58931318161689,39.951685371188));
#38326=CARTESIAN_POINT('Ctrl Pts',(19.5406777150738,1.59584658676708,39.9759463591679));
#38327=CARTESIAN_POINT('Ctrl Pts',(19.7636805904726,1.61201926405306,40.0193117595022));
#38328=CARTESIAN_POINT('Ctrl Pts',(19.8979328690707,1.62170794521142,40.0311116951321));
#38329=CARTESIAN_POINT('Ctrl Pts',(20.0464083560802,1.63176653625457,40.0286231078209));
#38330=CARTESIAN_POINT('Ctrl Pts',(20.0604847424205,1.63271333120259,40.0282329869045));
#38331=CARTESIAN_POINT('Ctrl Pts',(20.0800763341537,1.634020442352,40.0274752543962));
#38332=CARTESIAN_POINT('Ctrl Pts',(20.0855957220287,1.63438750752973,40.0272380366286));
#38333=CARTESIAN_POINT('Ctrl Pts',(20.0944628801919,1.63497524213699,40.0268187669263));
#38334=CARTESIAN_POINT('Ctrl Pts',(20.0978112758904,1.63519672885188,40.0266516942747));
#38335=CARTESIAN_POINT('Ctrl Pts',(20.104822799378,1.63565954981811,40.0262835191699));
#38336=CARTESIAN_POINT('Ctrl Pts',(20.1084858088695,1.63590078209794,40.02608069537));
#38337=CARTESIAN_POINT('Ctrl Pts',(20.1173962873301,1.6364862822048,40.025561815158));
#38338=CARTESIAN_POINT('Ctrl Pts',(20.1226431370371,1.63682994215671,40.0252347531679));
#38339=CARTESIAN_POINT('Ctrl Pts',(20.141278392357,1.63804679783516,40.0239966343775));
#38340=CARTESIAN_POINT('Ctrl Pts',(20.1546589311806,1.63891369879547,40.0229673092837));
#38341=CARTESIAN_POINT('Ctrl Pts',(20.2369541191611,1.64420938180913,40.0157720160734));
#38342=CARTESIAN_POINT('Ctrl Pts',(20.305514124898,1.64846607075289,40.006041171184));
#38343=CARTESIAN_POINT('Ctrl Pts',(20.5095452254164,1.66105352068333,39.9657868197054));
#38344=CARTESIAN_POINT('Ctrl Pts',(20.6423830643676,1.66916889523237,39.9243195392538));
#38345=CARTESIAN_POINT('Ctrl Pts',(20.8296603340419,1.68167847969386,39.8428404238884));
#38346=CARTESIAN_POINT('Ctrl Pts',(20.8883211370104,1.68575988078262,39.813684092192));
#38347=CARTESIAN_POINT('Ctrl Pts',(20.9562984762563,1.69074694824613,39.7754678769476));
#38348=CARTESIAN_POINT('Ctrl Pts',(20.9671544287993,1.69155143618401,39.769224874407));
#38349=CARTESIAN_POINT('Ctrl Pts',(20.9848474163789,1.69287625110042,39.7588195132976));
#38350=CARTESIAN_POINT('Ctrl Pts',(20.9917208030249,1.69339434012079,39.754719449609));
#38351=CARTESIAN_POINT('Ctrl Pts',(21.0040153548731,1.69432732218336,39.7472814733811));
#38352=CARTESIAN_POINT('Ctrl Pts',(21.0094459160056,1.69474164146732,39.7439592532683));
#38353=CARTESIAN_POINT('Ctrl Pts',(21.0209621487264,1.69562504248094,39.7368354634614));
#38354=CARTESIAN_POINT('Ctrl Pts',(21.027043239418,1.69609438263717,39.7330267069481));
#38355=CARTESIAN_POINT('Ctrl Pts',(21.0433368396896,1.6973597401718,39.7226945629928));
#38356=CARTESIAN_POINT('Ctrl Pts',(21.0535092297617,1.6981580450261,39.7161088135706));
#38357=CARTESIAN_POINT('Ctrl Pts',(21.1040881519733,1.70216985736208,39.6826828418386));
#38358=CARTESIAN_POINT('Ctrl Pts',(21.1435310710896,1.70543600372661,39.6544232382592));
#38359=CARTESIAN_POINT('Ctrl Pts',(21.3120581448833,1.72002452814741,39.5237910331012));
#38360=CARTESIAN_POINT('Ctrl Pts',(21.4287772880356,1.73191637436645,39.4066204687615));
#38361=CARTESIAN_POINT('Ctrl Pts',(21.5716378434624,1.74849486570901,39.2208697251584));
#38362=CARTESIAN_POINT('Ctrl Pts',(21.6110865878945,1.75335554094964,39.1633892644592));
#38363=CARTESIAN_POINT('Ctrl Pts',(21.6521305759144,1.75865517169651,39.0960380317368));
#38364=CARTESIAN_POINT('Ctrl Pts',(21.6568620949549,1.75927014380579,39.0881473610174));
#38365=CARTESIAN_POINT('Ctrl Pts',(21.6638298888144,1.76018151390984,39.0763365296709));
#38366=CARTESIAN_POINT('Ctrl Pts',(21.6661090680606,1.76048056260083,39.0724420252314));
#38367=CARTESIAN_POINT('Ctrl Pts',(21.6701608243531,1.76101382713724,39.0654626019151));
#38368=CARTESIAN_POINT('Ctrl Pts',(21.671938545601,1.7612483684443,39.0623807538233));
#38369=CARTESIAN_POINT('Ctrl Pts',(21.6757754234894,1.76175581752478,39.0556864423114));
#38370=CARTESIAN_POINT('Ctrl Pts',(21.6778314252505,1.76202852375884,39.0520722426568));
#38371=CARTESIAN_POINT('Ctrl Pts',(21.6835633381278,1.76279110362143,39.0419200075224));
#38372=CARTESIAN_POINT('Ctrl Pts',(21.6872128780378,1.76327933142902,39.0353670524104));
#38373=CARTESIAN_POINT('Ctrl Pts',(21.7087480064532,1.76617747663021,38.9961633528117));
#38374=CARTESIAN_POINT('Ctrl Pts',(21.7257250011852,1.76853412264443,38.9630192153938));
#38375=CARTESIAN_POINT('Ctrl Pts',(21.8107461283317,1.7808494956279,38.7844759460339));
#38376=CARTESIAN_POINT('Ctrl Pts',(21.8614067773933,1.79013980882812,38.6314921095146));
#38377=CARTESIAN_POINT('Ctrl Pts',(21.9086809738058,1.80493249588095,38.3922650207015));
#38378=CARTESIAN_POINT('Ctrl Pts',(21.9195182800998,1.8100807565815,38.3095920990348));
#38379=CARTESIAN_POINT('Ctrl Pts',(21.9258490491677,1.81624924577941,38.2132434340396));
#38380=CARTESIAN_POINT('Ctrl Pts',(21.9265824110817,1.81710103211466,38.1999941734814));
#38381=CARTESIAN_POINT('Ctrl Pts',(21.927549034963,1.81848793774505,38.17851750765));
#38382=CARTESIAN_POINT('Ctrl Pts',(21.9278664389684,1.81902044523461,38.1702941764443));
#38383=CARTESIAN_POINT('Ctrl Pts',(21.9283368531232,1.81996943415594,38.1556811210317));
#38384=CARTESIAN_POINT('Ctrl Pts',(21.9285107436,1.82038526100485,38.1492921549011));
#38385=CARTESIAN_POINT('Ctrl Pts',(21.9288095661928,1.82126155981125,38.1358587891713));
#38386=CARTESIAN_POINT('Ctrl Pts',(21.9289276623608,1.82172223791559,38.1288143465335));
#38387=CARTESIAN_POINT('Ctrl Pts',(21.9291372827702,1.82294004599769,38.110239762459));
#38388=CARTESIAN_POINT('Ctrl Pts',(21.9291640243603,1.82369917420297,38.0987093145578));
#38389=CARTESIAN_POINT('Ctrl Pts',(21.9288104507416,1.82721689264437,38.0455073419514));
#38390=CARTESIAN_POINT('Ctrl Pts',(21.9271833009245,1.8300137567064,38.0038580460169));
#38391=CARTESIAN_POINT('Ctrl Pts',(21.9122464158868,1.84425778675632,37.7951362214163));
#38392=CARTESIAN_POINT('Ctrl Pts',(21.8785525233989,1.8563314950612,37.6302657114153));
#38393=CARTESIAN_POINT('Ctrl Pts',(21.821276834621,1.86879920534607,37.4639470701502));
#38394=CARTESIAN_POINT('Ctrl Pts',(21.8184995227837,1.86939171258202,37.456049593733));
#38395=CARTESIAN_POINT('Ctrl Pts',(21.8080171955679,1.87158364067586,37.4268510796458));
#38396=CARTESIAN_POINT('Ctrl Pts',(21.7999883944055,1.8731765007669,37.4056675955477));
#38397=CARTESIAN_POINT('Ctrl Pts',(21.7748703005412,1.87790584083554,37.3427613097129));
#38398=CARTESIAN_POINT('Ctrl Pts',(21.7566883111422,1.8810079388215,37.3014876693979));
#38399=CARTESIAN_POINT('Ctrl Pts',(21.733798110862,1.88453847053896,37.254102001857));
#38400=CARTESIAN_POINT('Ctrl Pts',(21.7304814299476,1.88504170944507,37.2473375007421));
#38401=CARTESIAN_POINT('Ctrl Pts',(21.725088156308,1.88584661694057,37.2364988029708));
#38402=CARTESIAN_POINT('Ctrl Pts',(21.7230365978252,1.88614975920024,37.2324123399177));
#38403=CARTESIAN_POINT('Ctrl Pts',(21.7193570866823,1.88668802719513,37.2251477178879));
#38404=CARTESIAN_POINT('Ctrl Pts',(21.7177348193876,1.8869234989278,37.2219667443105));
#38405=CARTESIAN_POINT('Ctrl Pts',(21.7142461608097,1.88742593676269,37.2151727890593));
#38406=CARTESIAN_POINT('Ctrl Pts',(21.7123771785754,1.8876927382315,37.2115612051906));
#38407=CARTESIAN_POINT('Ctrl Pts',(21.7072219181284,1.88842227965474,37.2016759847729));
#38408=CARTESIAN_POINT('Ctrl Pts',(21.7039124500888,1.88888359611933,37.1954144151575));
#38409=CARTESIAN_POINT('Ctrl Pts',(21.6860758786098,1.89133359845821,37.1621125385456));
#38410=CARTESIAN_POINT('Ctrl Pts',(21.6709384949103,1.89328638063969,37.1354018646076));
#38411=CARTESIAN_POINT('Ctrl Pts',(21.5722060715657,1.90533758476987,36.9704885557513));
#38412=CARTESIAN_POINT('Ctrl Pts',(21.47216148179,1.91468603520564,36.8428680513414));
#38413=CARTESIAN_POINT('Ctrl Pts',(21.293926270049,1.92986041538412,36.6663791007295));
#38414=CARTESIAN_POINT('Ctrl Pts',(21.2262067302,1.93536240026429,36.6080455726267));
#38415=CARTESIAN_POINT('Ctrl Pts',(21.1439300959397,1.94192232284586,36.5465692280945));
#38416=CARTESIAN_POINT('Ctrl Pts',(21.1330789265493,1.94278499662619,36.5386366985708));
#38417=CARTESIAN_POINT('Ctrl Pts',(21.1154822977052,1.94418043901437,36.5260530781324));
#38418=CARTESIAN_POINT('Ctrl Pts',(21.10878843039,1.94471047149803,36.521330344062));
#38419=CARTESIAN_POINT('Ctrl Pts',(21.0968080372016,1.9456577817736,36.5129915857391));
#38420=CARTESIAN_POINT('Ctrl Pts',(21.091533170505,1.94607442399018,36.5093589614733));
#38421=CARTESIAN_POINT('Ctrl Pts',(21.0804594993875,1.94694820570668,36.5018139158502));
#38422=CARTESIAN_POINT('Ctrl Pts',(21.0746573184269,1.9474055302054,36.4979066396822));
#38423=CARTESIAN_POINT('Ctrl Pts',(21.0594248996098,1.94860490476069,36.4877688793451));
#38424=CARTESIAN_POINT('Ctrl Pts',(21.0499610422031,1.94934884498679,36.4815896364051));
#38425=CARTESIAN_POINT('Ctrl Pts',(21.0073452738725,1.95269381332018,36.4542956134918));
#38426=CARTESIAN_POINT('Ctrl Pts',(20.9736090501128,1.95532866914261,36.4341151107134));
#38427=CARTESIAN_POINT('Ctrl Pts',(20.7960748347889,1.96913864233127,36.3351520622656));
#38428=CARTESIAN_POINT('Ctrl Pts',(20.643292403629,1.98091936690152,36.2739166757123));
#38429=CARTESIAN_POINT('Ctrl Pts',(20.4062570484523,1.99831113208683,36.2123937851366));
#38430=CARTESIAN_POINT('Ctrl Pts',(20.3266503599643,2.00399593007626,36.1970011097992));
#38431=CARTESIAN_POINT('Ctrl Pts',(20.2370472690983,2.01006770961643,36.1854665745116));
#38432=CARTESIAN_POINT('Ctrl Pts',(20.2277827835748,2.0106916055411,36.1843422390202));
#38433=CARTESIAN_POINT('Ctrl Pts',(20.214000918111,2.01161357294287,36.1827710719501));
#38434=CARTESIAN_POINT('Ctrl Pts',(20.2094897006305,2.01191438407465,36.1822729021368));
#38435=CARTESIAN_POINT('Ctrl Pts',(20.2014369117707,2.01244955790994,36.1814123943049));
#38436=CARTESIAN_POINT('Ctrl Pts',(20.1978960652365,2.01268425583637,36.1810439353046));
#38437=CARTESIAN_POINT('Ctrl Pts',(20.1902359565547,2.01319064215454,36.1802682554683));
#38438=CARTESIAN_POINT('Ctrl Pts',(20.1861164068655,2.01346213648274,36.1798644907141));
#38439=CARTESIAN_POINT('Ctrl Pts',(20.1746146559484,2.01421789236132,36.178774545891));
#38440=CARTESIAN_POINT('Ctrl Pts',(20.167229653574,2.01470055524974,36.178117649049));
#38441=CARTESIAN_POINT('Ctrl Pts',(20.1242160166671,2.0174976912525,36.1745413939392));
#38442=CARTESIAN_POINT('Ctrl Pts',(20.0885128961982,2.01976312541157,36.1725700209739));
#38443=CARTESIAN_POINT('Ctrl Pts',(19.9709981319986,2.02709505233458,36.1693541033206));
#38444=CARTESIAN_POINT('Ctrl Pts',(19.8891566211293,2.03200534347251,36.1723198731452));
#38445=CARTESIAN_POINT('Ctrl Pts',(19.6670110749501,2.04535258710982,36.1945694437807));
#38446=CARTESIAN_POINT('Ctrl Pts',(19.5283038416974,2.05373968933419,36.2240933229587));
#38447=CARTESIAN_POINT('Ctrl Pts',(19.3941040086996,2.0626282966298,36.2684889832092));
#38448=CARTESIAN_POINT('Origin',(20.,-1.3495818343519,38.1));
#38449=CARTESIAN_POINT('',(19.3941040093468,3.02765621357216,36.2684889829951));
#38450=CARTESIAN_POINT('',(19.3941039244954,2.85753017062829,36.2684890110654));
#38451=CARTESIAN_POINT('',(19.3941040087494,-1.3495818343519,36.2684889831927));
#38452=CARTESIAN_POINT('Ctrl Pts',(19.3941040093468,3.02765621357216,36.2684889829951));
#38453=CARTESIAN_POINT('Ctrl Pts',(19.4103477405592,3.0264616496969,36.2631152716041));
#38454=CARTESIAN_POINT('Ctrl Pts',(19.4266683458038,3.02527319948087,36.2579558773622));
#38455=CARTESIAN_POINT('Ctrl Pts',(19.4719784478927,3.02200993305801,36.2442931254959));
#38456=CARTESIAN_POINT('Ctrl Pts',(19.5010979961917,3.01995323104104,36.2362532883861));
#38457=CARTESIAN_POINT('Ctrl Pts',(19.5372307457135,3.01746056567672,36.2271847857557));
#38458=CARTESIAN_POINT('Ctrl Pts',(19.5440747136245,3.01699103180448,36.2255069094698));
#38459=CARTESIAN_POINT('Ctrl Pts',(19.5548749377827,3.01625434343587,36.2229217629558));
#38460=CARTESIAN_POINT('Ctrl Pts',(19.5588250418642,3.01598580184797,36.2219894339839));
#38461=CARTESIAN_POINT('Ctrl Pts',(19.5662574535603,3.01548224395285,36.2202599324133));
#38462=CARTESIAN_POINT('Ctrl Pts',(19.5697389925866,3.01524707815708,36.2194599754244));
#38463=CARTESIAN_POINT('Ctrl Pts',(19.5776944067483,3.01471132296863,36.2176553007359));
#38464=CARTESIAN_POINT('Ctrl Pts',(19.5821696524334,3.01441109248322,36.2166568600859));
#38465=CARTESIAN_POINT('Ctrl Pts',(19.5940492064252,3.01361708429234,36.2140509241906));
#38466=CARTESIAN_POINT('Ctrl Pts',(19.6014595878548,3.01312482665771,36.2124710577546));
#38467=CARTESIAN_POINT('Ctrl Pts',(19.653836902804,3.00966568901347,36.2016266166513));
#38468=CARTESIAN_POINT('Ctrl Pts',(19.6991167777806,3.00678006171815,36.1939253799233));
#38469=CARTESIAN_POINT('Ctrl Pts',(19.7740206317822,3.00211433489331,36.1839219851429));
#38470=CARTESIAN_POINT('Ctrl Pts',(19.8034966126408,3.00030546784903,36.1806750717983));
#38471=CARTESIAN_POINT('Ctrl Pts',(19.9989030140084,2.98842734893121,36.1636992453304));
#38472=CARTESIAN_POINT('Ctrl Pts',(20.1659289182774,2.97874559193828,36.1708213566674));
#38473=CARTESIAN_POINT('Ctrl Pts',(20.3723125048065,2.965708013295,36.2066503281714));
#38474=CARTESIAN_POINT('Ctrl Pts',(20.4143959192395,2.96299624351154,36.2154137948));
#38475=CARTESIAN_POINT('Ctrl Pts',(20.4674693629423,2.95949257503285,36.2283294400888));
#38476=CARTESIAN_POINT('Ctrl Pts',(20.4787640548026,2.95874209845827,36.2311866705605));
#38477=CARTESIAN_POINT('Ctrl Pts',(20.4968720901933,2.95753080157063,36.2359424104362));
#38478=CARTESIAN_POINT('Ctrl Pts',(20.5037021979015,2.95707205373753,36.2377764192104));
#38479=CARTESIAN_POINT('Ctrl Pts',(20.516679695697,2.95619679486494,36.2413377332806));
#38480=CARTESIAN_POINT('Ctrl Pts',(20.5228289085563,2.95578051274444,36.2430580891123));
#38481=CARTESIAN_POINT('Ctrl Pts',(20.5368356559794,2.954828700196,36.2470518237536));
#38482=CARTESIAN_POINT('Ctrl Pts',(20.5446874573377,2.95429254584453,36.2493447009952));
#38483=CARTESIAN_POINT('Ctrl Pts',(20.5650793606633,2.95289322286747,36.2554405437587));
#38484=CARTESIAN_POINT('Ctrl Pts',(20.5775955461457,2.95202754494522,36.2593214180105));
#38485=CARTESIAN_POINT('Ctrl Pts',(20.6650349588565,2.94593100705766,36.2874132595377));
#38486=CARTESIAN_POINT('Ctrl Pts',(20.7384441290456,2.94055573692867,36.316060667094));
#38487=CARTESIAN_POINT('Ctrl Pts',(20.959625679844,2.92355341205621,36.4183701467329));
#38488=CARTESIAN_POINT('Ctrl Pts',(21.0998415565625,2.91153862120623,36.5065439597648));
#38489=CARTESIAN_POINT('Ctrl Pts',(21.2561679375433,2.89747849979775,36.6354176235858));
#38490=CARTESIAN_POINT('Ctrl Pts',(21.2845075876979,2.8949023595772,36.6602082985367));
#38491=CARTESIAN_POINT('Ctrl Pts',(21.317621354433,2.89187685816499,36.6909318208766));
#38492=CARTESIAN_POINT('Ctrl Pts',(21.3231070735429,2.89137512380437,36.6960816107763));
#38493=CARTESIAN_POINT('Ctrl Pts',(21.3315811805419,2.89059944840638,36.7041305761382));
#38494=CARTESIAN_POINT('Ctrl Pts',(21.3345904750762,2.89032387101778,36.7070074826135));
#38495=CARTESIAN_POINT('Ctrl Pts',(21.3401538891474,2.8898142117348,36.7123607221437));
#38496=CARTESIAN_POINT('Ctrl Pts',(21.342710450588,2.88957993808304,36.7148343570985));
#38497=CARTESIAN_POINT('Ctrl Pts',(21.3484895604084,2.88905018827784,36.7204570457118));
#38498=CARTESIAN_POINT('Ctrl Pts',(21.3517079221277,2.888755044586,36.7236103198832));
#38499=CARTESIAN_POINT('Ctrl Pts',(21.3614399995793,2.8878620502191,36.7332126348524));
#38500=CARTESIAN_POINT('Ctrl Pts',(21.3679189430422,2.88726686849352,36.7396969649001));
#38501=CARTESIAN_POINT('Ctrl Pts',(21.4511441669796,2.87960847912856,36.8241873115798));
#38502=CARTESIAN_POINT('Ctrl Pts',(21.5211766932684,2.87301418110241,36.908552847676));
#38503=CARTESIAN_POINT('Ctrl Pts',(21.631305782772,2.86147457275045,37.0668789037245));
#38504=CARTESIAN_POINT('Ctrl Pts',(21.6744379299934,2.85652318184319,37.1383582028391));
#38505=CARTESIAN_POINT('Ctrl Pts',(21.7489218396207,2.84671179155065,37.282090680764));
#38506=CARTESIAN_POINT('Ctrl Pts',(21.780744836716,2.8418729276214,37.3539109035469));
#38507=CARTESIAN_POINT('Ctrl Pts',(21.8147692315096,2.83566884880557,37.4453850083448));
#38508=CARTESIAN_POINT('Ctrl Pts',(21.8211680497288,2.83444510166513,37.4634035470905));
#38509=CARTESIAN_POINT('Ctrl Pts',(21.8300528389004,2.83265861714853,37.4896533707494));
#38510=CARTESIAN_POINT('Ctrl Pts',(21.832753415039,2.83210290710937,37.4978112283146));
#38511=CARTESIAN_POINT('Ctrl Pts',(21.8373834170219,2.83112738288449,37.5121171426652));
#38512=CARTESIAN_POINT('Ctrl Pts',(21.8393367259354,2.83070835478478,37.5182573747399));
#38513=CARTESIAN_POINT('Ctrl Pts',(21.8430641465167,2.82989397374695,37.5301809910386));
#38514=CARTESIAN_POINT('Ctrl Pts',(21.8448418907531,2.82949874463527,37.5359631679815));
#38515=CARTESIAN_POINT('Ctrl Pts',(21.8490191418076,2.82855348514106,37.5497808646332));
#38516=CARTESIAN_POINT('Ctrl Pts',(21.8513934890125,2.82800264663377,37.557823802819));
#38517=CARTESIAN_POINT('Ctrl Pts',(21.8597413942069,2.82601600279909,37.5867961187604));
#38518=CARTESIAN_POINT('Ctrl Pts',(21.8654129075072,2.82457053394606,37.6078101017201));
#38519=CARTESIAN_POINT('Ctrl Pts',(21.9079435708128,2.8129124481545,37.7767037264029));
#38520=CARTESIAN_POINT('Ctrl Pts',(21.9275085337689,2.80213283157299,37.9283544080817));
#38521=CARTESIAN_POINT('Ctrl Pts',(21.9298517307292,2.78542764369942,38.1624490844719));
#38522=CARTESIAN_POINT('Ctrl Pts',(21.9254716135726,2.77959722016018,38.2441815852222));
#38523=CARTESIAN_POINT('Ctrl Pts',(21.9117422408348,2.77145494660324,38.3608855220005));
#38524=CARTESIAN_POINT('Ctrl Pts',(21.9065811577922,2.76901222884761,38.3962572195072));
#38525=CARTESIAN_POINT('Ctrl Pts',(21.8991661056456,2.7661224196174,38.4387707436596));
#38526=CARTESIAN_POINT('Ctrl Pts',(21.8978502273035,2.76562815207771,38.4460665148581));
#38527=CARTESIAN_POINT('Ctrl Pts',(21.8957341509273,2.76486150372461,38.4574237232509));
#38528=CARTESIAN_POINT('Ctrl Pts',(21.8949629006628,2.76458754589498,38.4614903800184));
#38529=CARTESIAN_POINT('Ctrl Pts',(21.8935039703952,2.76407934637782,38.4690500568951));
#38530=CARTESIAN_POINT('Ctrl Pts',(21.8928197166378,2.76384492253005,38.4725436229835));
#38531=CARTESIAN_POINT('Ctrl Pts',(21.8912410664991,2.76331287028463,38.4804870370712));
#38532=CARTESIAN_POINT('Ctrl Pts',(21.890340635975,2.76301558648448,38.484935628402));
#38533=CARTESIAN_POINT('Ctrl Pts',(21.8875406903118,2.7621096323015,38.4985220262328));
#38534=CARTESIAN_POINT('Ctrl Pts',(21.8855905217025,2.76150374571872,38.507649427731));
#38535=CARTESIAN_POINT('Ctrl Pts',(21.8660557509568,2.75566646922722,38.5959375671419));
#38536=CARTESIAN_POINT('Ctrl Pts',(21.8435601883917,2.75069028718033,38.6739402958565));
#38537=CARTESIAN_POINT('Ctrl Pts',(21.7609757076507,2.73590353698134,38.9045883064166));
#38538=CARTESIAN_POINT('Ctrl Pts',(21.686304973013,2.72634491017049,39.0511953319656));
#38539=CARTESIAN_POINT('Ctrl Pts',(21.5718828412208,2.71366463210328,39.2190482510695));
#38540=CARTESIAN_POINT('Ctrl Pts',(21.548779634438,2.7111819205209,39.2508110009356));
#38541=CARTESIAN_POINT('Ctrl Pts',(21.5178024014421,2.7079369139024,39.29077541743));
#38542=CARTESIAN_POINT('Ctrl Pts',(21.5108020730258,2.70720879825165,39.2996446606775));
#38543=CARTESIAN_POINT('Ctrl Pts',(21.4993429186813,2.70602497061475,39.3139037401377));
#38544=CARTESIAN_POINT('Ctrl Pts',(21.4949319131556,2.705571163259,39.3193318051359));
#38545=CARTESIAN_POINT('Ctrl Pts',(21.4864252892428,2.70469951975784,39.3296842843577));
#38546=CARTESIAN_POINT('Ctrl Pts',(21.4823344666383,2.70428188010314,39.3346125331692));
#38547=CARTESIAN_POINT('Ctrl Pts',(21.4729545304108,2.70332768198222,39.3457987980023));
#38548=CARTESIAN_POINT('Ctrl Pts',(21.4676499645987,2.70279050011322,39.3520436380918));
#38549=CARTESIAN_POINT('Ctrl Pts',(21.4535354974341,2.70136743375187,39.3684470518819));
#38550=CARTESIAN_POINT('Ctrl Pts',(21.4446590159347,2.70047882719762,39.3785474875494));
#38551=CARTESIAN_POINT('Ctrl Pts',(21.3759054453228,2.69364286459706,39.4551511625999));
#38552=CARTESIAN_POINT('Ctrl Pts',(21.3115807262736,2.68750718281808,39.5174985928199));
#38553=CARTESIAN_POINT('Ctrl Pts',(21.1192444162555,2.66986429621142,39.6795883737103));
#38554=CARTESIAN_POINT('Ctrl Pts',(20.9826616067041,2.65805951154523,39.7679869209663));
#38555=CARTESIAN_POINT('Ctrl Pts',(20.8095689876326,2.64481552014014,39.8512975871015));
#38556=CARTESIAN_POINT('Ctrl Pts',(20.7821950730113,2.64276987420016,39.8636939358309));
#38557=CARTESIAN_POINT('Ctrl Pts',(20.7480665920808,2.64028869356715,39.8781980820234));
#38558=CARTESIAN_POINT('Ctrl Pts',(20.7415771047436,2.63981994626655,39.8809142165149));
#38559=CARTESIAN_POINT('Ctrl Pts',(20.7313227642944,2.63908421201398,39.8851403369242));
#38560=CARTESIAN_POINT('Ctrl Pts',(20.727567838374,2.63881584384386,39.8866740187865));
#38561=CARTESIAN_POINT('Ctrl Pts',(20.7204962670545,2.63831242771437,39.8895363787909));
#38562=CARTESIAN_POINT('Ctrl Pts',(20.7171808063892,2.63807723132922,39.890867670446));
#38563=CARTESIAN_POINT('Ctrl Pts',(20.7095979773278,2.63754117357786,39.89388804833));
#38564=CARTESIAN_POINT('Ctrl Pts',(20.7053282696522,2.63724067261447,39.8955711215295));
#38565=CARTESIAN_POINT('Ctrl Pts',(20.6939805882409,2.63644547408643,39.8999975339677));
#38566=CARTESIAN_POINT('Ctrl Pts',(20.686892272989,2.63595230386472,39.9027143947518));
#38567=CARTESIAN_POINT('Ctrl Pts',(20.6365228130546,2.63247170303313,39.9216801384828));
#38568=CARTESIAN_POINT('Ctrl Pts',(20.5926819389425,2.62956667003102,39.9364119175139));
#38569=CARTESIAN_POINT('Ctrl Pts',(20.4275985956237,2.61893859112482,39.9853552925194));
#38570=CARTESIAN_POINT('Ctrl Pts',(20.3036236393871,2.61155247367216,40.0092465645142));
#38571=CARTESIAN_POINT('Ctrl Pts',(20.071384872498,2.59753259676736,40.0307909766193));
#38572=CARTESIAN_POINT('Ctrl Pts',(19.9639473736855,2.59097562209409,40.0317725047487));
#38573=CARTESIAN_POINT('Ctrl Pts',(19.8423139832667,2.58318347090327,40.0227309663199));
#38574=CARTESIAN_POINT('Ctrl Pts',(19.8276473386552,2.58223802884719,40.0214717769315));
#38575=CARTESIAN_POINT('Ctrl Pts',(19.8052970532705,2.58078774996471,40.0192949666091));
#38576=CARTESIAN_POINT('Ctrl Pts',(19.7976019209633,2.58028669662734,40.0184987414758));
#38577=CARTESIAN_POINT('Ctrl Pts',(19.7836031582776,2.57937196134497,40.0169651122066));
#38578=CARTESIAN_POINT('Ctrl Pts',(19.7772979519516,2.57895875772002,40.0162428423127));
#38579=CARTESIAN_POINT('Ctrl Pts',(19.7636810505516,2.57806375335962,40.0146148937941));
#38580=CARTESIAN_POINT('Ctrl Pts',(19.756370771401,2.57758162083575,40.0136984176844));
#38581=CARTESIAN_POINT('Ctrl Pts',(19.7365203670184,2.57626786499577,40.0110942263146));
#38582=CARTESIAN_POINT('Ctrl Pts',(19.7239914849026,2.57543370355801,40.0093249973601));
#38583=CARTESIAN_POINT('Ctrl Pts',(19.6620619283136,2.57128518945258,39.9999575140884));
#38584=CARTESIAN_POINT('Ctrl Pts',(19.6129561118462,2.56791510531554,39.9905652459399));
#38585=CARTESIAN_POINT('Ctrl Pts',(19.5384408765842,2.56267277912306,39.9732882726191));
#38586=CARTESIAN_POINT('Ctrl Pts',(19.5127350954418,2.56084064285159,39.9667668809669));
#38587=CARTESIAN_POINT('Ctrl Pts',(19.365874586633,2.55024045298943,39.926269308208));
#38588=CARTESIAN_POINT('Ctrl Pts',(19.2481465339524,2.54119143588346,39.8810350696547));
#38589=CARTESIAN_POINT('Ctrl Pts',(19.0864568095457,2.52835464991372,39.8000035886388));
#38590=CARTESIAN_POINT('Ctrl Pts',(19.0383135496695,2.52448005371354,39.7732403928952));
#38591=CARTESIAN_POINT('Ctrl Pts',(18.9674775824633,2.51876185415784,39.7297932810787));
#38592=CARTESIAN_POINT('Ctrl Pts',(18.9438979976954,2.51685551083962,39.7146137142168));
#38593=CARTESIAN_POINT('Ctrl Pts',(18.914952761141,2.5145196159674,39.6950744182306));
#38594=CARTESIAN_POINT('Ctrl Pts',(18.9092697907039,2.51406120767834,39.6911937419147));
#38595=CARTESIAN_POINT('Ctrl Pts',(18.900298265023,2.51333802126474,39.6849967911428));
#38596=CARTESIAN_POINT('Ctrl Pts',(18.8969960469015,2.51307193817817,39.6827005446481));
#38597=CARTESIAN_POINT('Ctrl Pts',(18.8907680847924,2.51257034434057,39.6783408796276));
#38598=CARTESIAN_POINT('Ctrl Pts',(18.8878409387374,2.51233469928018,39.6762796695677));
#38599=CARTESIAN_POINT('Ctrl Pts',(18.8811274371085,2.51179445268715,39.6715242089815));
#38600=CARTESIAN_POINT('Ctrl Pts',(18.8773450663637,2.51149023211789,39.6688244173586));
#38601=CARTESIAN_POINT('Ctrl Pts',(18.8672503682369,2.51067860581816,39.6615637911655));
#38602=CARTESIAN_POINT('Ctrl Pts',(18.8609557599148,2.5101728294972,39.6569782998532));
#38603=CARTESIAN_POINT('Ctrl Pts',(18.8135966291405,2.50636846243603,39.6220372298172));
#38604=CARTESIAN_POINT('Ctrl Pts',(18.7737201048851,2.50317058316769,39.5900969579077));
#38605=CARTESIAN_POINT('Ctrl Pts',(18.6370708370491,2.49204419624869,39.4714376298351));
#38606=CARTESIAN_POINT('Ctrl Pts',(18.5478355178802,2.48444154210104,39.3765733955574));
#38607=CARTESIAN_POINT('Ctrl Pts',(18.4145035042108,2.47122505034933,39.2025940612386));
#38608=CARTESIAN_POINT('Ctrl Pts',(18.3651889648186,2.46575407074745,39.1280577722659));
#38609=CARTESIAN_POINT('Ctrl Pts',(18.311136379595,2.45878922739923,39.0325774938197));
#38610=CARTESIAN_POINT('Ctrl Pts',(18.3013416839863,2.45748110233096,39.0146152113554));
#38611=CARTESIAN_POINT('Ctrl Pts',(18.28773129818,2.45559396135025,38.9886824067608));
#38612=CARTESIAN_POINT('Ctrl Pts',(18.2836815872703,2.455023147258,38.9808357560809));
#38613=CARTESIAN_POINT('Ctrl Pts',(18.2767523736861,2.45402998562907,38.9671806051903));
#38614=CARTESIAN_POINT('Ctrl Pts',(18.2738479936511,2.45360851143797,38.9613848343723));
#38615=CARTESIAN_POINT('Ctrl Pts',(18.2683170668068,2.45279574552673,38.9502074076196));
#38616=CARTESIAN_POINT('Ctrl Pts',(18.2656862531136,2.45240460759234,38.9448279369723));
#38617=CARTESIAN_POINT('Ctrl Pts',(18.2595344007411,2.45147910845092,38.9320988337403));
#38618=CARTESIAN_POINT('Ctrl Pts',(18.2560348256246,2.4509440155397,38.9247390123206));
#38619=CARTESIAN_POINT('Ctrl Pts',(18.2439642600965,2.44906775947515,38.8989335019963));
#38620=CARTESIAN_POINT('Ctrl Pts',(18.2356386931552,2.44771827324523,38.88037515708));
#38621=CARTESIAN_POINT('Ctrl Pts',(18.1608324141978,2.43505490225917,38.7063067607359));
#38622=CARTESIAN_POINT('Ctrl Pts',(18.114792244157,2.42302274532309,38.5428465110104));
#38623=CARTESIAN_POINT('Ctrl Pts',(18.0805797129769,2.40594633895446,38.305759905488));
#38624=CARTESIAN_POINT('Ctrl Pts',(18.0743427887243,2.40094444206335,38.2354882626051));
#38625=CARTESIAN_POINT('Ctrl Pts',(18.0712319781269,2.39456633323423,38.143255844243));
#38626=CARTESIAN_POINT('Ctrl Pts',(18.0708664568246,2.39307365318261,38.1214711559831));
#38627=CARTESIAN_POINT('Ctrl Pts',(18.0708723612183,2.39063161387751,38.0854280318276));
#38628=CARTESIAN_POINT('Ctrl Pts',(18.0710327202739,2.3896728751938,38.0711720263516));
#38629=CARTESIAN_POINT('Ctrl Pts',(18.0714751079546,2.38835210647864,38.051367410205));
#38630=CARTESIAN_POINT('Ctrl Pts',(18.0716230764981,2.3879831441303,38.0458166924315));
#38631=CARTESIAN_POINT('Ctrl Pts',(18.0718989790891,2.38739317178397,38.0369105057474));
#38632=CARTESIAN_POINT('Ctrl Pts',(18.0720117098403,2.38717133291001,38.0335546498165));
#38633=CARTESIAN_POINT('Ctrl Pts',(18.0722657605068,2.38670848260905,38.0265378970563));
#38634=CARTESIAN_POINT('Ctrl Pts',(18.0724087477532,2.38646757023914,38.0228770900491));
#38635=CARTESIAN_POINT('Ctrl Pts',(18.0727812291302,2.38588405129458,38.0139899240755));
#38636=CARTESIAN_POINT('Ctrl Pts',(18.0730215576221,2.38554204277053,38.0087639975883));
#38637=CARTESIAN_POINT('Ctrl Pts',(18.073945986909,2.38433738415484,37.9902993932441));
#38638=CARTESIAN_POINT('Ctrl Pts',(18.074745300028,2.38348086312548,37.9770664887699));
#38639=CARTESIAN_POINT('Ctrl Pts',(18.0804482971912,2.37829968707831,37.8964658548161));
#38640=CARTESIAN_POINT('Ctrl Pts',(18.0887514985972,2.3741391856421,37.8293783406481));
#38641=CARTESIAN_POINT('Ctrl Pts',(18.1219088814571,2.36264470240885,37.6425712657982));
#38642=CARTESIAN_POINT('Ctrl Pts',(18.1546368139108,2.35547522620142,37.5245842842083));
#38643=CARTESIAN_POINT('Ctrl Pts',(18.227807506339,2.34305210998545,37.3333905924606));
#38644=CARTESIAN_POINT('Ctrl Pts',(18.2622250155511,2.33794882236075,37.2582804772984));
#38645=CARTESIAN_POINT('Ctrl Pts',(18.3076218454999,2.33183000691493,37.1739469731754));
#38646=CARTESIAN_POINT('Ctrl Pts',(18.3140203935903,2.33097967525284,37.1623482634531));
#38647=CARTESIAN_POINT('Ctrl Pts',(18.3245835198597,2.3295946714876,37.1436581223657));
#38648=CARTESIAN_POINT('Ctrl Pts',(18.3286749561505,2.32906259924003,37.1365256810891));
#38649=CARTESIAN_POINT('Ctrl Pts',(18.3360270389649,2.3281140936265,37.1238968386692));
#38650=CARTESIAN_POINT('Ctrl Pts',(18.3392696543895,2.32769831235906,37.1183900397063));
#38651=CARTESIAN_POINT('Ctrl Pts',(18.3461464961397,2.32682180992262,37.1068429952113));
#38652=CARTESIAN_POINT('Ctrl Pts',(18.3497865811584,2.32636088109772,37.1008063658869));
#38653=CARTESIAN_POINT('Ctrl Pts',(18.3594764756729,2.3251417203357,37.0849342588209));
#38654=CARTESIAN_POINT('Ctrl Pts',(18.3655815752862,2.32438148224348,37.0751330350015));
#38655=CARTESIAN_POINT('Ctrl Pts',(18.3942189907791,2.3208508566806,37.0300647857358));
#38656=CARTESIAN_POINT('Ctrl Pts',(18.4178056613398,2.3180418522169,36.9954844377372));
#38657=CARTESIAN_POINT('Ctrl Pts',(18.5412971267982,2.3037937555316,36.8265145133867));
#38658=CARTESIAN_POINT('Ctrl Pts',(18.6572678458037,2.2917302167849,36.7047826648682));
#38659=CARTESIAN_POINT('Ctrl Pts',(18.7964907657336,2.27904327237431,36.5922722474851));
#38660=CARTESIAN_POINT('Ctrl Pts',(18.8055900426846,2.27822171005806,36.5850536931518));
#38661=CARTESIAN_POINT('Ctrl Pts',(18.827182235825,2.2762908871701,36.5682398461245));
#38662=CARTESIAN_POINT('Ctrl Pts',(18.8397287397793,2.27518344950221,36.5587144003546));
#38663=CARTESIAN_POINT('Ctrl Pts',(18.8912966929374,2.27069419711152,36.5205500096734));
#38664=CARTESIAN_POINT('Ctrl Pts',(18.9312764141424,2.26735695047316,36.4932280516757));
#38665=CARTESIAN_POINT('Ctrl Pts',(18.9787475590504,2.26359244768881,36.4633433334009));
#38666=CARTESIAN_POINT('Ctrl Pts',(18.9852743656991,2.26307907681671,36.459288726077));
#38667=CARTESIAN_POINT('Ctrl Pts',(18.9957613189835,2.26226114897953,36.4528604973739));
#38668=CARTESIAN_POINT('Ctrl Pts',(18.9997059817277,2.26195504307505,36.4504619593149));
#38669=CARTESIAN_POINT('Ctrl Pts',(19.0067214963704,2.26141344904227,36.4462306207904));
#38670=CARTESIAN_POINT('Ctrl Pts',(19.0097888779322,2.26117759889086,36.4443921720605));
#38671=CARTESIAN_POINT('Ctrl Pts',(19.0163321473246,2.26067652301233,36.4404951246609));
#38672=CARTESIAN_POINT('Ctrl Pts',(19.0198093890805,2.26041145074962,36.4384389139521));
#38673=CARTESIAN_POINT('Ctrl Pts',(19.0292958248408,2.25969151271216,36.4328694070494));
#38674=CARTESIAN_POINT('Ctrl Pts',(19.0353176884968,2.25923800851437,36.4293776455734));
#38675=CARTESIAN_POINT('Ctrl Pts',(19.0665740660081,2.25690146777443,36.4114790769709));
#38676=CARTESIAN_POINT('Ctrl Pts',(19.0921143856017,2.25505051011215,36.3976102637962));
#38677=CARTESIAN_POINT('Ctrl Pts',(19.2069417831661,2.24694070403176,36.338576797337));
#38678=CARTESIAN_POINT('Ctrl Pts',(19.2992730025973,2.24097284866353,36.299860718032));
#38679=CARTESIAN_POINT('Ctrl Pts',(19.3941044697278,2.2350068401775,36.268488830693));
#38680=CARTESIAN_POINT('',(18.0708706743286,2.22141497567151,38.1016129892876));
#38681=CARTESIAN_POINT('Ctrl Pts',(19.3941040086996,2.0626282966298,36.2684889832092));
#38682=CARTESIAN_POINT('Ctrl Pts',(19.3837674814086,2.06331292737663,36.2719084878653));
#38683=CARTESIAN_POINT('Ctrl Pts',(19.3734576817228,2.06400028375384,36.2754162315735));
#38684=CARTESIAN_POINT('Ctrl Pts',(19.3426326342688,2.0660695318738,36.2861961695889));
#38685=CARTESIAN_POINT('Ctrl Pts',(19.3222132677515,2.06745915353942,36.2937272427941));
#38686=CARTESIAN_POINT('Ctrl Pts',(19.2941088216315,2.06939999429191,36.3046363815698));
#38687=CARTESIAN_POINT('Ctrl Pts',(19.2863113020811,2.06994151740616,36.3077217523744));
#38688=CARTESIAN_POINT('Ctrl Pts',(19.2729239932806,2.07087660059436,36.3131201410377));
#38689=CARTESIAN_POINT('Ctrl Pts',(19.2673244661449,2.07126934347668,36.3154088113464));
#38690=CARTESIAN_POINT('Ctrl Pts',(19.2557828735064,2.07208226101268,36.3201896325796));
#38691=CARTESIAN_POINT('Ctrl Pts',(19.2498423516104,2.07250254950246,36.3226852906081));
#38692=CARTESIAN_POINT('Ctrl Pts',(19.2361661600603,2.07347452345652,36.3285115426101));
#38693=CARTESIAN_POINT('Ctrl Pts',(19.2284396214318,2.07402691172667,36.3318631082023));
#38694=CARTESIAN_POINT('Ctrl Pts',(19.2039324085865,2.07578953688088,36.3426849059176));
#38695=CARTESIAN_POINT('Ctrl Pts',(19.1872367786683,2.07700616077794,36.3503440748035));
#38696=CARTESIAN_POINT('Ctrl Pts',(19.148409691538,2.07987368153634,36.3688317609161));
#38697=CARTESIAN_POINT('Ctrl Pts',(19.126371685827,2.08153081106813,36.3798479716506));
#38698=CARTESIAN_POINT('Ctrl Pts',(19.0491866014652,2.0874415986763,36.420296599831));
#38699=CARTESIAN_POINT('Ctrl Pts',(18.9952697390479,2.09176865068765,36.4519813695081));
#38700=CARTESIAN_POINT('Ctrl Pts',(18.8277802712925,2.10583271508917,36.5616856104231));
#38701=CARTESIAN_POINT('Ctrl Pts',(18.7209901401899,2.11580306557456,36.649261791309));
#38702=CARTESIAN_POINT('Ctrl Pts',(18.5904697249032,2.12883024623558,36.7820037402358));
#38703=CARTESIAN_POINT('Ctrl Pts',(18.5578123162378,2.1321707479992,36.8178200882498));
#38704=CARTESIAN_POINT('Ctrl Pts',(18.5215749130172,2.13593846750677,36.8607014553424));
#38705=CARTESIAN_POINT('Ctrl Pts',(18.5166494151853,2.13645196227061,36.8666011723855));
#38706=CARTESIAN_POINT('Ctrl Pts',(18.5088214395908,2.13727004826609,36.8760921703944));
#38707=CARTESIAN_POINT('Ctrl Pts',(18.5058964312515,2.1375761893785,36.8796646357067));
#38708=CARTESIAN_POINT('Ctrl Pts',(18.5007286692489,2.1381178220528,36.8860227256939));
#38709=CARTESIAN_POINT('Ctrl Pts',(18.4984808031248,2.13835367583354,36.8888041248516));
#38710=CARTESIAN_POINT('Ctrl Pts',(18.4937104067454,2.13885473301535,36.8947404702165));
#38711=CARTESIAN_POINT('Ctrl Pts',(18.4911900506403,2.13911978308861,36.8978970882922));
#38712=CARTESIAN_POINT('Ctrl Pts',(18.484354455053,2.13983960134159,36.9065136905843));
#38713=CARTESIAN_POINT('Ctrl Pts',(18.4800587642489,2.14029300869801,36.9119892121048));
#38714=CARTESIAN_POINT('Ctrl Pts',(18.4579931863945,2.14262820041621,36.9404307952289));
#38715=CARTESIAN_POINT('Ctrl Pts',(18.4407127616884,2.14447794987287,36.9637741056941));
#38716=CARTESIAN_POINT('Ctrl Pts',(18.3383613315816,2.1556261271066,37.1087713845485));
#38717=CARTESIAN_POINT('Ctrl Pts',(18.2670313528305,2.1642745534715,37.239530788041));
#38718=CARTESIAN_POINT('Ctrl Pts',(18.1955004796772,2.17576009324727,37.4165347113017));
#38719=CARTESIAN_POINT('Ctrl Pts',(18.1809038118789,2.17833025404646,37.4563913204045));
#38720=CARTESIAN_POINT('Ctrl Pts',(18.1477329086564,2.18483426385661,37.5571385189386));
#38721=CARTESIAN_POINT('Ctrl Pts',(18.1308367911885,2.18880476548764,37.618523557311));
#38722=CARTESIAN_POINT('Ctrl Pts',(18.1143038206637,2.19366898491016,37.6927569314287));
#38723=CARTESIAN_POINT('Ctrl Pts',(18.1117195549744,2.19446741301666,37.7049127349891));
#38724=CARTESIAN_POINT('Ctrl Pts',(18.1076701947323,2.19578425777799,37.7249079415508));
#38725=CARTESIAN_POINT('Ctrl Pts',(18.10613591901,2.19630048248717,37.7327330891463));
#38726=CARTESIAN_POINT('Ctrl Pts',(18.1034645937295,2.19723142816394,37.746819446872));
#38727=CARTESIAN_POINT('Ctrl Pts',(18.1023099198421,2.19764558579903,37.7530772299217));
#38728=CARTESIAN_POINT('Ctrl Pts',(18.1001323311239,2.19845008584416,37.7652149686975));
#38729=CARTESIAN_POINT('Ctrl Pts',(18.0991056989401,2.19884030576123,37.7710941908712));
#38730=CARTESIAN_POINT('Ctrl Pts',(18.0969243607689,2.19969396873407,37.7839375065397));
#38731=CARTESIAN_POINT('Ctrl Pts',(18.0957805688173,2.2001577500138,37.7909033418525));
#38732=CARTESIAN_POINT('Ctrl Pts',(18.09307340656,2.20129639992165,37.8079758369018));
#38733=CARTESIAN_POINT('Ctrl Pts',(18.0915521365483,2.201972578416,37.8180888610348));
#38734=CARTESIAN_POINT('Ctrl Pts',(18.0772218344598,2.20872315228076,37.9187902017144));
#38735=CARTESIAN_POINT('Ctrl Pts',(18.0707942025025,2.21499668833455,38.0101529632487));
#38736=CARTESIAN_POINT('Ctrl Pts',(18.0708706743286,2.22141497567151,38.1016129892876));
#38737=CARTESIAN_POINT('Ctrl Pts',(18.0708706726244,2.22141483255489,38.101610949888));
#38738=CARTESIAN_POINT('Ctrl Pts',(18.0709609419981,2.22900073837971,38.2097094683175));
#38739=CARTESIAN_POINT('Ctrl Pts',(18.0801371753914,2.23676879516904,38.3176093215099));
#38740=CARTESIAN_POINT('Ctrl Pts',(18.1104940944532,2.24959110593643,38.495695526882));
#38741=CARTESIAN_POINT('Ctrl Pts',(18.1267142218013,2.25468398518988,38.5664870627855));
#38742=CARTESIAN_POINT('Ctrl Pts',(18.1507073391127,2.26052604307724,38.6494070975814));
#38743=CARTESIAN_POINT('Ctrl Pts',(18.1546691527667,2.26144961169759,38.6625705246755));
#38744=CARTESIAN_POINT('Ctrl Pts',(18.1603552841934,2.26271915466431,38.6807564415166));
#38745=CARTESIAN_POINT('Ctrl Pts',(18.1619600210698,2.26307162883516,38.6858154677575));
#38746=CARTESIAN_POINT('Ctrl Pts',(18.1647122872409,2.26366635901946,38.694369496987));
#38747=CARTESIAN_POINT('Ctrl Pts',(18.1658489638607,2.2639092373872,38.6978679327191));
#38748=CARTESIAN_POINT('Ctrl Pts',(18.1680374130316,2.26437163514157,38.7045385057978));
#38749=CARTESIAN_POINT('Ctrl Pts',(18.169087427831,2.26459125823236,38.7077111802016));
#38750=CARTESIAN_POINT('Ctrl Pts',(18.1718775310252,2.26516903548758,38.7160687509546));
#38751=CARTESIAN_POINT('Ctrl Pts',(18.1736314485895,2.26552638672897,38.7212490512517));
#38752=CARTESIAN_POINT('Ctrl Pts',(18.1798720596672,2.26677780406596,38.7394262139612));
#38753=CARTESIAN_POINT('Ctrl Pts',(18.1844757741283,2.26766532294951,38.7523828734396));
#38754=CARTESIAN_POINT('Ctrl Pts',(18.237220697295,2.27746063615847,38.8959437566029));
#38755=CARTESIAN_POINT('Ctrl Pts',(18.2992310100625,2.28566008279396,39.0210397683309));
#38756=CARTESIAN_POINT('Ctrl Pts',(18.4127755032649,2.29827107498648,39.1988189258553));
#38757=CARTESIAN_POINT('Ctrl Pts',(18.4547114529037,2.30257688317349,39.2570510130127));
#38758=CARTESIAN_POINT('Ctrl Pts',(18.5259468670265,2.30953179534874,39.3451670791728));
#38759=CARTESIAN_POINT('Ctrl Pts',(18.5531428812381,2.3121152190768,39.3766666835909));
#38760=CARTESIAN_POINT('Ctrl Pts',(18.6000092488074,2.31647486485586,39.4275269886585));
#38761=CARTESIAN_POINT('Ctrl Pts',(18.6191151506446,2.31822856140567,39.4473896690387));
#38762=CARTESIAN_POINT('Ctrl Pts',(18.6454931391802,2.32062252827853,39.4736620027975));
#38763=CARTESIAN_POINT('Ctrl Pts',(18.6523982104883,2.32124676921118,39.4804367226639));
#38764=CARTESIAN_POINT('Ctrl Pts',(18.6636305877078,2.32225846966197,39.4912924659715));
#38765=CARTESIAN_POINT('Ctrl Pts',(18.6679263862433,2.32264452216654,39.4954059689565));
#38766=CARTESIAN_POINT('Ctrl Pts',(18.6768882345388,2.3234481453241,39.503908418453));
#38767=CARTESIAN_POINT('Ctrl Pts',(18.6815572536949,2.3238658476275,39.5082941150078));
#38768=CARTESIAN_POINT('Ctrl Pts',(18.6922527724101,2.32482053559937,39.518240807613));
#38769=CARTESIAN_POINT('Ctrl Pts',(18.6982930275449,2.32535814693835,39.5237867656403));
#38770=CARTESIAN_POINT('Ctrl Pts',(18.714347158798,2.32678309904504,39.538339573154));
#38771=CARTESIAN_POINT('Ctrl Pts',(18.7244201721483,2.32767317345917,39.5472802226952));
#38772=CARTESIAN_POINT('Ctrl Pts',(18.8015692546965,2.33446137931533,39.6143254645469));
#38773=CARTESIAN_POINT('Ctrl Pts',(18.8724794809763,2.34054455229296,39.6678364830251));
#38774=CARTESIAN_POINT('Ctrl Pts',(19.0812216282755,2.3580150087443,39.8038562215967));
#38775=CARTESIAN_POINT('Ctrl Pts',(19.2260215775423,2.36969488126651,39.8743262352871));
#38776=CARTESIAN_POINT('Ctrl Pts',(19.4082628650795,2.38299358288505,39.9364152078867));
#38777=CARTESIAN_POINT('Ctrl Pts',(19.4389139965967,2.38518310687873,39.9460109552883));
#38778=CARTESIAN_POINT('Ctrl Pts',(19.4766972120311,2.38781324187271,39.9568113310942));
#38779=CARTESIAN_POINT('Ctrl Pts',(19.4836130027279,2.3882918624023,39.9587465131705));
#38780=CARTESIAN_POINT('Ctrl Pts',(19.4944827097626,2.38903956703852,39.9617227345097));
#38781=CARTESIAN_POINT('Ctrl Pts',(19.4984293159343,2.3893101068305,39.9627898755835));
#38782=CARTESIAN_POINT('Ctrl Pts',(19.50582564974,2.3898153299646,39.9647645943081));
#38783=CARTESIAN_POINT('Ctrl Pts',(19.5092744643569,2.39005017496455,39.96567514042));
#38784=CARTESIAN_POINT('Ctrl Pts',(19.5171906144162,2.39058756040116,39.9677416701674));
#38785=CARTESIAN_POINT('Ctrl Pts',(19.5216595813365,2.39088972861176,39.9688911937968));
#38786=CARTESIAN_POINT('Ctrl Pts',(19.5334116883059,2.39168128253318,39.9718691969183));
#38787=CARTESIAN_POINT('Ctrl Pts',(19.5407015408204,2.39216920128345,39.9736712285856));
#38788=CARTESIAN_POINT('Ctrl Pts',(19.5913510317723,2.39553905554356,39.9858782780073));
#38789=CARTESIAN_POINT('Ctrl Pts',(19.6350533939722,2.39834437620869,39.9948207177396));
#38790=CARTESIAN_POINT('Ctrl Pts',(19.8266182305024,2.41035294625213,40.027143922744));
#38791=CARTESIAN_POINT('Ctrl Pts',(19.9766114017382,2.41905134242259,40.0347880714908));
#38792=CARTESIAN_POINT('Ctrl Pts',(20.2043027713724,2.43288062786482,40.0198859857278));
#38793=CARTESIAN_POINT('Ctrl Pts',(20.2822220750879,2.4377189529152,40.0099870102348));
#38794=CARTESIAN_POINT('Ctrl Pts',(20.378101033434,2.44392238238293,39.9918106970656));
#38795=CARTESIAN_POINT('Ctrl Pts',(20.3968312347448,2.44514605375802,39.9879706127031));
#38796=CARTESIAN_POINT('Ctrl Pts',(20.4238920935745,2.44693244664039,39.9820020961753));
#38797=CARTESIAN_POINT('Ctrl Pts',(20.4322708662512,2.44748814181692,39.9800952878166));
#38798=CARTESIAN_POINT('Ctrl Pts',(20.4469095845359,2.44846364779153,39.9766608371438));
#38799=CARTESIAN_POINT('Ctrl Pts',(20.4531751818969,2.44888267258375,39.9751576806381));
#38800=CARTESIAN_POINT('Ctrl Pts',(20.4653083681166,2.44969705297167,39.9721824895531));
#38801=CARTESIAN_POINT('Ctrl Pts',(20.4711768017813,2.45009228476865,39.9707141876015));
#38802=CARTESIAN_POINT('Ctrl Pts',(20.485164032666,2.45103755996511,39.9671445440556));
#38803=CARTESIAN_POINT('Ctrl Pts',(20.4932761691972,2.45158841155734,39.965017829444));
#38804=CARTESIAN_POINT('Ctrl Pts',(20.5223925511194,2.45357515712556,39.9571812937121));
#38805=CARTESIAN_POINT('Ctrl Pts',(20.5433130162198,2.45502071594099,39.9511691538027));
#38806=CARTESIAN_POINT('Ctrl Pts',(20.7098551754629,2.46667804172203,39.9002418840376));
#38807=CARTESIAN_POINT('Ctrl Pts',(20.8497629334488,2.47745669931358,39.8385771134705));
#38808=CARTESIAN_POINT('Ctrl Pts',(21.0513417662641,2.49416159725634,39.7195399100313));
#38809=CARTESIAN_POINT('Ctrl Pts',(21.1190419285904,2.49999266928135,39.6735233920551));
#38810=CARTESIAN_POINT('Ctrl Pts',(21.2118419231335,2.50813571857942,39.6014189822083));
#38811=CARTESIAN_POINT('Ctrl Pts',(21.2394505980905,2.51057858889319,39.578709715305));
#38812=CARTESIAN_POINT('Ctrl Pts',(21.2720066774823,2.51346855251977,39.5503780637209));
#38813=CARTESIAN_POINT('Ctrl Pts',(21.2775710039241,2.51396282775438,39.5454791072874));
#38814=CARTESIAN_POINT('Ctrl Pts',(21.2861978723628,2.5147294848541,39.5377950904769));
#38815=CARTESIAN_POINT('Ctrl Pts',(21.2892798513917,2.5150034437997,39.5350321092801));
#38816=CARTESIAN_POINT('Ctrl Pts',(21.294996006555,2.5155116434555,39.5298743208044));
#38817=CARTESIAN_POINT('Ctrl Pts',(21.2976324218261,2.51574606633729,39.5274821639645));
#38818=CARTESIAN_POINT('Ctrl Pts',(21.3036150682087,2.51627811384295,39.5220235266704));
#38819=CARTESIAN_POINT('Ctrl Pts',(21.3069571037145,2.51657539388721,39.5189525314664));
#38820=CARTESIAN_POINT('Ctrl Pts',(21.317138055274,2.51748132798786,39.5095307735622));
#38821=CARTESIAN_POINT('Ctrl Pts',(21.3239418751051,2.51808719841528,39.5031420377499));
#38822=CARTESIAN_POINT('Ctrl Pts',(21.3893905170916,2.52392281948971,39.4407863375027));
#38823=CARTESIAN_POINT('Ctrl Pts',(21.4445070103362,2.52889752383458,39.3812170001058));
#38824=CARTESIAN_POINT('Ctrl Pts',(21.5992226525299,2.54368379363837,39.1912788415149));
#38825=CARTESIAN_POINT('Ctrl Pts',(21.6861082669779,2.55324315995879,39.0515465072539));
#38826=CARTESIAN_POINT('Ctrl Pts',(21.7706251192927,2.56592484791844,38.8667933744221));
#38827=CARTESIAN_POINT('Ctrl Pts',(21.7858693434932,2.5684081405143,38.8305858888898));
#38828=CARTESIAN_POINT('Ctrl Pts',(21.8040618525085,2.5716538036117,38.783396720437));
#38829=CARTESIAN_POINT('Ctrl Pts',(21.808033834689,2.57238197726352,38.7728178720649));
#38830=CARTESIAN_POINT('Ctrl Pts',(21.8143135761112,2.5735658752575,38.7556353622928));
#38831=CARTESIAN_POINT('Ctrl Pts',(21.8166787971334,2.5740196945362,38.7490528689272));
#38832=CARTESIAN_POINT('Ctrl Pts',(21.8211411402213,2.57489134468714,38.7364185148809));
#38833=CARTESIAN_POINT('Ctrl Pts',(21.823244026951,2.57530897898102,38.730368777164));
#38834=CARTESIAN_POINT('Ctrl Pts',(21.8279682464349,2.5762631422604,38.7165563854847));
#38835=CARTESIAN_POINT('Ctrl Pts',(21.8305703159642,2.57680029449718,38.7087873202346));
#38836=CARTESIAN_POINT('Ctrl Pts',(21.8373114587073,2.57822323363825,38.6882260874263));
#38837=CARTESIAN_POINT('Ctrl Pts',(21.8413663656927,2.57911174183464,38.6754070020759));
#38838=CARTESIAN_POINT('Ctrl Pts',(21.8713651384373,2.58594379149808,38.5770039244058));
#38839=CARTESIAN_POINT('Ctrl Pts',(21.8914597506812,2.59207540821949,38.4897640808411));
#38840=CARTESIAN_POINT('Ctrl Pts',(21.9307315793931,2.60970288143303,38.241536479277));
#38841=CARTESIAN_POINT('Ctrl Pts',(21.9357985521885,2.62149577502337,38.0790797125331));
#38842=CARTESIAN_POINT('Ctrl Pts',(21.9176626776828,2.63474443700944,37.8878055753898));
#38843=CARTESIAN_POINT('Ctrl Pts',(21.9141014895529,2.6368032742196,37.8577762222596));
#38844=CARTESIAN_POINT('Ctrl Pts',(21.9088411887868,2.63929815585782,37.8208628350344));
#38845=CARTESIAN_POINT('Ctrl Pts',(21.9078085128571,2.63976784016104,37.813890016022));
#38846=CARTESIAN_POINT('Ctrl Pts',(21.9061209607066,2.64050471050852,37.8029109290229));
#38847=CARTESIAN_POINT('Ctrl Pts',(21.905491631387,2.6407732847713,37.7989008860716));
#38848=CARTESIAN_POINT('Ctrl Pts',(21.9042846707602,2.64127686862687,37.7913655718566));
#38849=CARTESIAN_POINT('Ctrl Pts',(21.9037099114485,2.64151202791202,37.7878399595895));
#38850=CARTESIAN_POINT('Ctrl Pts',(21.9023751573773,2.64204772341363,37.7797932948486));
#38851=CARTESIAN_POINT('Ctrl Pts',(21.9016088382092,2.64234790101261,37.775273344266));
#38852=CARTESIAN_POINT('Ctrl Pts',(21.8995337617006,2.64314167792473,37.763293288296));
#38853=CARTESIAN_POINT('Ctrl Pts',(21.8981971552068,2.64363375857316,37.7558379944219));
#38854=CARTESIAN_POINT('Ctrl Pts',(21.8884599243563,2.6470887678886,37.7033088455004));
#38855=CARTESIAN_POINT('Ctrl Pts',(21.8784978716309,2.64997066305941,37.6585350753943));
#38856=CARTESIAN_POINT('Ctrl Pts',(21.8594741673796,2.65463465864422,37.585432999102));
#38857=CARTESIAN_POINT('Ctrl Pts',(21.8513376119807,2.65644537548504,37.556886244054));
#38858=CARTESIAN_POINT('Ctrl Pts',(21.7932504613387,2.668320503885,37.3695979596894));
#38859=CARTESIAN_POINT('Ctrl Pts',(21.7236015157723,2.67799748101472,37.2177114922496));
#38860=CARTESIAN_POINT('Ctrl Pts',(21.6124725188639,2.69103523714952,37.0401270388563));
#38861=CARTESIAN_POINT('Ctrl Pts',(21.5884051671132,2.69375326852014,37.0043874308613));
#38862=CARTESIAN_POINT('Ctrl Pts',(21.5563303471501,2.69726398894659,36.9600375646843));
#38863=CARTESIAN_POINT('Ctrl Pts',(21.5494121598154,2.69801504751461,36.9506521619984));
#38864=CARTESIAN_POINT('Ctrl Pts',(21.5381606147526,2.69922705878787,36.9356742195972));
#38865=CARTESIAN_POINT('Ctrl Pts',(21.5338807579841,2.699685934565,36.9300417025522));
#38866=CARTESIAN_POINT('Ctrl Pts',(21.5256792593149,2.70056128992854,36.9193704554545));
#38867=CARTESIAN_POINT('Ctrl Pts',(21.5217633842612,2.70097753976601,36.9143273957617));
#38868=CARTESIAN_POINT('Ctrl Pts',(21.5127761986139,2.70192907157628,36.9028711110164));
#38869=CARTESIAN_POINT('Ctrl Pts',(21.5076890348471,2.70246497613587,36.8964705343582));
#38870=CARTESIAN_POINT('Ctrl Pts',(21.4943507319243,2.70386322411135,36.8799058085624));
#38871=CARTESIAN_POINT('Ctrl Pts',(21.4860366536778,2.70472807050399,36.8697931086134));
#38872=CARTESIAN_POINT('Ctrl Pts',(21.4279109684917,2.71072963489348,36.800541900227));
#38873=CARTESIAN_POINT('Ctrl Pts',(21.3746924570972,2.71600539709617,36.7443676857191));
#38874=CARTESIAN_POINT('Ctrl Pts',(21.1968432062746,2.73298840488644,36.5779086061822));
#38875=CARTESIAN_POINT('Ctrl Pts',(21.0612650157502,2.74510147445316,36.4804614467146));
#38876=CARTESIAN_POINT('Ctrl Pts',(20.8816380553973,2.75926228354161,36.383700874751));
#38877=CARTESIAN_POINT('Ctrl Pts',(20.847873332075,2.76184672217634,36.3667719057651));
#38878=CARTESIAN_POINT('Ctrl Pts',(20.8068027356714,2.76488063783682,36.3476676649037));
#38879=CARTESIAN_POINT('Ctrl Pts',(20.7999560031608,2.76538281956287,36.3445314971458));
#38880=CARTESIAN_POINT('Ctrl Pts',(20.7892945620614,2.76615903509646,36.3397233186012));
#38881=CARTESIAN_POINT('Ctrl Pts',(20.7854926011904,2.76643470884167,36.3380234748825));
#38882=CARTESIAN_POINT('Ctrl Pts',(20.7784329779411,2.76694445519502,36.3348945329433));
#38883=CARTESIAN_POINT('Ctrl Pts',(20.7751768950254,2.76717872013273,36.3334621451137));
#38884=CARTESIAN_POINT('Ctrl Pts',(20.7677893963602,2.76770833463933,36.3302366591734));
#38885=CARTESIAN_POINT('Ctrl Pts',(20.7636556599757,2.76800335245849,36.3284490202931));
#38886=CARTESIAN_POINT('Ctrl Pts',(20.7510988108066,2.76889559023584,36.3230709153021));
#38887=CARTESIAN_POINT('Ctrl Pts',(20.7426562116054,2.76949014786703,36.3195258622957));
#38888=CARTESIAN_POINT('Ctrl Pts',(20.6326846360213,2.77716962817051,36.2742670509938));
#38889=CARTESIAN_POINT('Ctrl Pts',(20.527783909128,2.78378269262661,36.241225594123));
#38890=CARTESIAN_POINT('Ctrl Pts',(20.3386623072263,2.7953768385389,36.1989728909579));
#38891=CARTESIAN_POINT('Ctrl Pts',(20.2555894045633,2.80036323486063,36.1860329601209));
#38892=CARTESIAN_POINT('Ctrl Pts',(20.0945206081371,2.81016808452353,36.1716197982785));
#38893=CARTESIAN_POINT('Ctrl Pts',(20.0167612999912,2.81496205283437,36.1693779979842));
#38894=CARTESIAN_POINT('Ctrl Pts',(19.920071811922,2.82111215505278,36.1724326505139));
#38895=CARTESIAN_POINT('Ctrl Pts',(19.9010695584797,2.82232969974099,36.1733144707299));
#38896=CARTESIAN_POINT('Ctrl Pts',(19.8735245838303,2.82410876170631,36.1750012820883));
#38897=CARTESIAN_POINT('Ctrl Pts',(19.8649688967471,2.82466333443581,36.1755825057665));
#38898=CARTESIAN_POINT('Ctrl Pts',(19.849994708311,2.82563753989242,36.1767001140822));
#38899=CARTESIAN_POINT('Ctrl Pts',(19.8435744420332,2.82605639304065,36.177211638831));
#38900=CARTESIAN_POINT('Ctrl Pts',(19.8311241652542,2.82687093507917,36.1782663647949));
#38901=CARTESIAN_POINT('Ctrl Pts',(19.8250939064596,2.82726650249305,36.1788058220782));
#38902=CARTESIAN_POINT('Ctrl Pts',(19.8106979941921,2.82821337809269,36.1801619968691));
#38903=CARTESIAN_POINT('Ctrl Pts',(19.8023349998851,2.82876550072339,36.1810050152163));
#38904=CARTESIAN_POINT('Ctrl Pts',(19.7722151856953,2.83076157986249,36.1842401730162));
#38905=CARTESIAN_POINT('Ctrl Pts',(19.7504946331037,2.83221532017182,36.1869478204954));
#38906=CARTESIAN_POINT('Ctrl Pts',(19.6150531465257,2.84137334453092,36.2061775242916));
#38907=CARTESIAN_POINT('Ctrl Pts',(19.5030370899688,2.84937933430976,36.2324520023598));
#38908=CARTESIAN_POINT('Ctrl Pts',(19.3941039244954,2.85753017062829,36.2684890110654));
#38909=CARTESIAN_POINT('Origin',(20.,-1.3495818343519,38.1));
#38910=CARTESIAN_POINT('',(19.3941042587802,3.8243647438501,36.2684889004781));
#38911=CARTESIAN_POINT('',(19.3941040086362,3.65343403802913,36.2684889832302));
#38912=CARTESIAN_POINT('',(19.3941040087494,-1.3495818343519,36.2684889831927));
#38913=CARTESIAN_POINT('',(18.0708705425584,3.18824125908482,38.0985531651523));
#38914=CARTESIAN_POINT('Ctrl Pts',(19.3941042587802,3.8243647438501,36.2684889004781));
#38915=CARTESIAN_POINT('Ctrl Pts',(19.5025433210666,3.81660121883645,36.2326153717628));
#38916=CARTESIAN_POINT('Ctrl Pts',(19.6139981162338,3.80853747388574,36.2064285893548));
#38917=CARTESIAN_POINT('Ctrl Pts',(19.8481095679091,3.79167443629537,36.1729819420564));
#38918=CARTESIAN_POINT('Ctrl Pts',(19.9704351967536,3.78290655232174,36.1672298042598));
#38919=CARTESIAN_POINT('Ctrl Pts',(20.107006183639,3.77363918350316,36.1737852183773));
#38920=CARTESIAN_POINT('Ctrl Pts',(20.1215127262511,3.77266167470754,36.174645903566));
#38921=CARTESIAN_POINT('Ctrl Pts',(20.1415918807353,3.77131943144695,36.1760650676144));
#38922=CARTESIAN_POINT('Ctrl Pts',(20.1471734234849,3.77094747330308,36.1764839823665));
#38923=CARTESIAN_POINT('Ctrl Pts',(20.1561088410343,3.77035394411287,36.1771937387333));
#38924=CARTESIAN_POINT('Ctrl Pts',(20.159463861605,3.77013152597861,36.1774690728387));
#38925=CARTESIAN_POINT('Ctrl Pts',(20.1664613743643,3.76966856762079,36.1780617762628));
#38926=CARTESIAN_POINT('Ctrl Pts',(20.1701037009248,3.76942812196083,36.1783807202722));
#38927=CARTESIAN_POINT('Ctrl Pts',(20.1789170405876,3.7688475589309,36.1791777237417));
#38928=CARTESIAN_POINT('Ctrl Pts',(20.1840871227174,3.76850802490127,36.1796663161911));
#38929=CARTESIAN_POINT('Ctrl Pts',(20.2022067486207,3.76732149272778,36.1814525392052));
#38930=CARTESIAN_POINT('Ctrl Pts',(20.2151454297398,3.76648038144531,36.1828603611538));
#38931=CARTESIAN_POINT('Ctrl Pts',(20.2927612751864,3.76146644101594,36.1921012164594));
#38932=CARTESIAN_POINT('Ctrl Pts',(20.3570289023945,3.75744650594636,36.2030763991522));
#38933=CARTESIAN_POINT('Ctrl Pts',(20.5019014198875,3.74844009564498,36.2354428835545));
#38934=CARTESIAN_POINT('Ctrl Pts',(20.5819198626719,3.74350314700833,36.2588458980446));
#38935=CARTESIAN_POINT('Ctrl Pts',(20.6899625171287,3.7366202859837,36.2981955957557));
#38936=CARTESIAN_POINT('Ctrl Pts',(20.719475208269,3.73471737891405,36.3097757838709));
#38937=CARTESIAN_POINT('Ctrl Pts',(20.8334108091746,3.72724693098387,36.3577544224452));
#38938=CARTESIAN_POINT('Ctrl Pts',(20.9154638346477,3.72158924801021,36.3994366071388));
#38939=CARTESIAN_POINT('Ctrl Pts',(21.0058030523098,3.71485681565364,36.4537663432116));
#38940=CARTESIAN_POINT('Ctrl Pts',(21.017305550735,3.71398990064518,36.4608494778251));
#38941=CARTESIAN_POINT('Ctrl Pts',(21.0356793735786,3.71258892387703,36.4724318054191));
#38942=CARTESIAN_POINT('Ctrl Pts',(21.0425981413652,3.71205763378613,36.4768551805027));
#38943=CARTESIAN_POINT('Ctrl Pts',(21.0548647146645,3.71110888958743,36.4848083560577));
#38944=CARTESIAN_POINT('Ctrl Pts',(21.0602236050805,3.71069207800875,36.4883209008967));
#38945=CARTESIAN_POINT('Ctrl Pts',(21.0713879324936,3.70981877517561,36.4957184627461));
#38946=CARTESIAN_POINT('Ctrl Pts',(21.0771899560768,3.70936210307275,36.4996084388377));
#38947=CARTESIAN_POINT('Ctrl Pts',(21.0922876465777,3.70816630228019,36.5098500054185));
#38948=CARTESIAN_POINT('Ctrl Pts',(21.1015489553772,3.70742530404474,36.5162515357664));
#38949=CARTESIAN_POINT('Ctrl Pts',(21.1425281534099,3.70411266899588,36.5451101931637));
#38950=CARTESIAN_POINT('Ctrl Pts',(21.1736172330131,3.70150800319788,36.5684403002368));
#38951=CARTESIAN_POINT('Ctrl Pts',(21.2560428001338,3.69434287162441,36.6342786234473));
#38952=CARTESIAN_POINT('Ctrl Pts',(21.3059120722831,3.68971844521503,36.6785307763896));
#38953=CARTESIAN_POINT('Ctrl Pts',(21.4451927637774,3.67595455738178,36.8156492241863));
#38954=CARTESIAN_POINT('Ctrl Pts',(21.5277087359096,3.66664359036591,36.9149922428716));
#38955=CARTESIAN_POINT('Ctrl Pts',(21.6282058439836,3.6540405146561,37.0641001398016));
#38956=CARTESIAN_POINT('Ctrl Pts',(21.655020567939,3.65051920900012,37.1075027733854));
#38957=CARTESIAN_POINT('Ctrl Pts',(21.6839118589527,3.6465731684424,37.1587008922485));
#38958=CARTESIAN_POINT('Ctrl Pts',(21.6876967045008,3.64605294754337,37.1655038803737));
#38959=CARTESIAN_POINT('Ctrl Pts',(21.6936745738103,3.64522623131345,37.1764034528446));
#38960=CARTESIAN_POINT('Ctrl Pts',(21.695894110163,3.64491813520693,37.1804852844453));
#38961=CARTESIAN_POINT('Ctrl Pts',(21.6997976837887,3.64437429253333,37.1877263529914));
#38962=CARTESIAN_POINT('Ctrl Pts',(21.7014877002396,3.64413817319311,37.1908823070664));
#38963=CARTESIAN_POINT('Ctrl Pts',(21.7050580135407,3.64363793982618,37.1975943772408));
#38964=CARTESIAN_POINT('Ctrl Pts',(21.7069359739587,3.6433739720348,37.2011516707111));
#38965=CARTESIAN_POINT('Ctrl Pts',(21.7119973347179,3.64266015736078,37.2108121320031));
#38966=CARTESIAN_POINT('Ctrl Pts',(21.71515925621,3.64221163318699,37.2169265783588));
#38967=CARTESIAN_POINT('Ctrl Pts',(21.7310457212049,3.63994414737874,37.2480546655005));
#38968=CARTESIAN_POINT('Ctrl Pts',(21.7432568432671,3.63815504853951,37.2733284082068));
#38969=CARTESIAN_POINT('Ctrl Pts',(21.7778079793526,3.63292337642989,37.3490134603445));
#38970=CARTESIAN_POINT('Ctrl Pts',(21.798544501222,3.62955207640777,37.4001281502922));
#38971=CARTESIAN_POINT('Ctrl Pts',(21.8593526728616,3.61861456140839,37.570658033933));
#38972=CARTESIAN_POINT('Ctrl Pts',(21.8899291538575,3.61122580694507,37.6931048355494));
#38973=CARTESIAN_POINT('Ctrl Pts',(21.9121862126765,3.60195472760078,37.8435414122052));
#38974=CARTESIAN_POINT('Ctrl Pts',(21.9154884493044,3.60034923090744,37.8694982773877));
#38975=CARTESIAN_POINT('Ctrl Pts',(21.9235738439877,3.59562963942916,37.9453463586235));
#38976=CARTESIAN_POINT('Ctrl Pts',(21.9269417735406,3.59248140563564,37.9953634372041));
#38977=CARTESIAN_POINT('Ctrl Pts',(21.9287167358271,3.58846138683155,38.0581109541955));
#38978=CARTESIAN_POINT('Ctrl Pts',(21.9289501583924,3.58764662366278,38.0707730724771));
#38979=CARTESIAN_POINT('Ctrl Pts',(21.9291221702567,3.58635158223311,38.0908061356981));
#38980=CARTESIAN_POINT('Ctrl Pts',(21.9291432155285,3.58587386548661,38.0981761559781));
#38981=CARTESIAN_POINT('Ctrl Pts',(21.9291037829279,3.58498233913905,38.111892321641));
#38982=CARTESIAN_POINT('Ctrl Pts',(21.9290542219237,3.58456887436756,38.118238418028));
#38983=CARTESIAN_POINT('Ctrl Pts',(21.9288748005464,3.58364941829366,38.1323165894047));
#38984=CARTESIAN_POINT('Ctrl Pts',(21.9287297598687,3.58314296219173,38.140048328313));
#38985=CARTESIAN_POINT('Ctrl Pts',(21.9281740246796,3.58166917862733,38.1624799190289));
#38986=CARTESIAN_POINT('Ctrl Pts',(21.9276417361844,3.58069809842653,38.1771759444177));
#38987=CARTESIAN_POINT('Ctrl Pts',(21.9218660123355,3.5726452998271,38.2983275216931));
#38988=CARTESIAN_POINT('Ctrl Pts',(21.9079772807468,3.56529257211311,38.4041685881899));
#38989=CARTESIAN_POINT('Ctrl Pts',(21.8576451070652,3.54849997592396,38.6365860869335));
#38990=CARTESIAN_POINT('Ctrl Pts',(21.8168470541981,3.53900638468864,38.7616920046678));
#38991=CARTESIAN_POINT('Ctrl Pts',(21.7466282471285,3.5269331584024,38.9201218589893));
#38992=CARTESIAN_POINT('Ctrl Pts',(21.7283392513016,3.52404578659653,38.9579942591744));
#38993=CARTESIAN_POINT('Ctrl Pts',(21.705398770605,3.52073038495009,39.0017827441544));
#38994=CARTESIAN_POINT('Ctrl Pts',(21.7019343905949,3.52023724293405,39.0083041444553));
#38995=CARTESIAN_POINT('Ctrl Pts',(21.6962621799369,3.51944209482291,39.0188351984868));
#38996=CARTESIAN_POINT('Ctrl Pts',(21.6940774159525,3.51913870681818,39.0228570934297));
#38997=CARTESIAN_POINT('Ctrl Pts',(21.6901662994261,3.51860072651248,39.0299963087989));
#38998=CARTESIAN_POINT('Ctrl Pts',(21.6884456063757,3.51836578469834,39.03311665356));
#38999=CARTESIAN_POINT('Ctrl Pts',(21.6847202587229,3.51786087290266,39.0398282404255));
#39000=CARTESIAN_POINT('Ctrl Pts',(21.6827127670511,3.5175910864004,39.0434178374598));
#39001=CARTESIAN_POINT('Ctrl Pts',(21.6771137977364,3.51684489818896,39.0533546302021));
#39002=CARTESIAN_POINT('Ctrl Pts',(21.6734977383796,3.51637003016424,39.059688004126));
#39003=CARTESIAN_POINT('Ctrl Pts',(21.6529227880819,3.51370654926248,39.0952542194193));
#39004=CARTESIAN_POINT('Ctrl Pts',(21.6352327336523,3.51156166116654,39.1240600318223));
#39005=CARTESIAN_POINT('Ctrl Pts',(21.5762624347535,3.50480633402643,39.2146566429716));
#39006=CARTESIAN_POINT('Ctrl Pts',(21.53216428244,3.50032534346411,39.274536988412));
#39007=CARTESIAN_POINT('Ctrl Pts',(21.3804969029989,3.48609968014812,39.4573559849003));
#39008=CARTESIAN_POINT('Ctrl Pts',(21.2607669663413,3.47647053990753,39.5692336949343));
#39009=CARTESIAN_POINT('Ctrl Pts',(21.1114061524359,3.46479194693231,39.6769455292146));
#39010=CARTESIAN_POINT('Ctrl Pts',(21.0942281774938,3.4634544115764,39.6889133012857));
#39011=CARTESIAN_POINT('Ctrl Pts',(21.0700142047057,3.46157509300193,39.7052041065539));
#39012=CARTESIAN_POINT('Ctrl Pts',(21.0631396684544,3.46104221091463,39.7097654064699));
#39013=CARTESIAN_POINT('Ctrl Pts',(21.051203676807,3.46011803690985,39.717575208539));
#39014=CARTESIAN_POINT('Ctrl Pts',(21.0461558594991,3.45972751810159,39.7208444224199));
#39015=CARTESIAN_POINT('Ctrl Pts',(21.0356502455313,3.45891538211942,39.7275788523453));
#39016=CARTESIAN_POINT('Ctrl Pts',(21.0301901588556,3.45849363418281,39.7310403387302));
#39017=CARTESIAN_POINT('Ctrl Pts',(21.0173205799296,3.45750031016147,39.7391087573173));
#39018=CARTESIAN_POINT('Ctrl Pts',(21.0098970775913,3.45692791301771,39.7436929668037));
#39019=CARTESIAN_POINT('Ctrl Pts',(20.985477352857,3.45504671563211,39.7585449162368));
#39020=CARTESIAN_POINT('Ctrl Pts',(20.9683541306402,3.45373029139789,39.7686003356105));
#39021=CARTESIAN_POINT('Ctrl Pts',(20.8777111089287,3.4467732558458,39.8199642812923));
#39022=CARTESIAN_POINT('Ctrl Pts',(20.8017060280256,3.44097314349407,39.8566780890556));
#39023=CARTESIAN_POINT('Ctrl Pts',(20.5989410530765,3.42561412041804,39.9387175233243));
#39024=CARTESIAN_POINT('Ctrl Pts',(20.4694102680866,3.41589133475475,39.97597007301));
#39025=CARTESIAN_POINT('Ctrl Pts',(20.2855653899182,3.40279403552321,40.0085938696197));
#39026=CARTESIAN_POINT('Ctrl Pts',(20.2337112340199,3.3991794484512,40.0156352250331));
#39027=CARTESIAN_POINT('Ctrl Pts',(20.1730817546099,3.39509119298739,40.02136904098));
#39028=CARTESIAN_POINT('Ctrl Pts',(20.1645278671098,3.39451759588833,40.0221204106642));
#39029=CARTESIAN_POINT('Ctrl Pts',(20.1515386303621,3.39365170658775,40.0231740322234));
#39030=CARTESIAN_POINT('Ctrl Pts',(20.1471069217298,3.39335718477633,40.0235180969446));
#39031=CARTESIAN_POINT('Ctrl Pts',(20.1391301544877,3.39282874161915,40.0241096603328));
#39032=CARTESIAN_POINT('Ctrl Pts',(20.1355855859339,3.39259452008685,40.0243626826556));
#39033=CARTESIAN_POINT('Ctrl Pts',(20.1278396708874,3.39208398713389,40.0248941018442));
#39034=CARTESIAN_POINT('Ctrl Pts',(20.1236381158603,3.39180789770246,40.0251685385727));
#39035=CARTESIAN_POINT('Ctrl Pts',(20.1117076468648,3.3910262159495,40.025908593446));
#39036=CARTESIAN_POINT('Ctrl Pts',(20.1039766723116,3.39052240451841,40.0263414456479));
#39037=CARTESIAN_POINT('Ctrl Pts',(20.0544894142823,3.38731362729925,40.0288134136018));
#39038=CARTESIAN_POINT('Ctrl Pts',(20.0126752242087,3.3846761089191,40.0295414551389));
#39039=CARTESIAN_POINT('Ctrl Pts',(19.8682150890163,3.37571760218043,40.0273596187466));
#39040=CARTESIAN_POINT('Ctrl Pts',(19.76584254203,3.36963052880947,40.0176172765035));
#39041=CARTESIAN_POINT('Ctrl Pts',(19.5314299373878,3.35540641149355,39.976247761211));
#39042=CARTESIAN_POINT('Ctrl Pts',(19.401000942513,3.34725290050035,39.9387649279003));
#39043=CARTESIAN_POINT('Ctrl Pts',(19.2628950097487,3.33773860501639,39.8828084621858));
#39044=CARTESIAN_POINT('Ctrl Pts',(19.2502687592799,3.33686063858492,39.8775356060379));
#39045=CARTESIAN_POINT('Ctrl Pts',(19.2301091772033,3.33544524494969,39.8688637480313));
#39046=CARTESIAN_POINT('Ctrl Pts',(19.222539587481,3.33491068294472,39.8655498128344));
#39047=CARTESIAN_POINT('Ctrl Pts',(19.2091317837365,3.33395819025838,39.8595769870236));
#39048=CARTESIAN_POINT('Ctrl Pts',(19.2032850664722,3.3335409201871,39.856937398372));
#39049=CARTESIAN_POINT('Ctrl Pts',(19.1973148407526,3.33311284200173,39.8542061209186));
#39050=CARTESIAN_POINT('Ctrl Pts',(19.1971780071591,3.33310302966088,39.8541435024978));
#39051=CARTESIAN_POINT('Ctrl Pts',(19.196920628429,3.33308457100355,39.8540256832314));
#39052=CARTESIAN_POINT('Ctrl Pts',(19.1968000813616,3.33307592478898,39.8539704858341));
#39053=CARTESIAN_POINT('Ctrl Pts',(19.1965733244084,3.33305965912167,39.8538666276248));
#39054=CARTESIAN_POINT('Ctrl Pts',(19.1964671125088,3.33305203971096,39.853817969251));
#39055=CARTESIAN_POINT('Ctrl Pts',(19.1962673082783,3.33303770497076,39.8537264118891));
#39056=CARTESIAN_POINT('Ctrl Pts',(19.1961737139265,3.33303098964095,39.8536835145818));
#39057=CARTESIAN_POINT('Ctrl Pts',(19.195997634089,3.33301835508762,39.8536027944615));
#39058=CARTESIAN_POINT('Ctrl Pts',(19.1959151464363,3.33301243582085,39.8535649726778));
#39059=CARTESIAN_POINT('Ctrl Pts',(19.1957599543809,3.33300129859176,39.85349380162));
#39060=CARTESIAN_POINT('Ctrl Pts',(19.1956872477326,3.33299608055567,39.8534604528873));
#39061=CARTESIAN_POINT('Ctrl Pts',(19.1955504354527,3.33298626119168,39.8533976901928));
#39062=CARTESIAN_POINT('Ctrl Pts',(19.1954863363428,3.33298166039979,39.8533682804427));
#39063=CARTESIAN_POINT('Ctrl Pts',(19.1953657212189,3.33297300265714,39.8533129321879));
#39064=CARTESIAN_POINT('Ctrl Pts',(19.1953092047704,3.3329689457278,39.8532869944307));
#39065=CARTESIAN_POINT('Ctrl Pts',(19.1951834533378,3.3329599184834,39.8532292744882));
#39066=CARTESIAN_POINT('Ctrl Pts',(19.1951142190453,3.33295494812582,39.8531974909631));
#39067=CARTESIAN_POINT('Ctrl Pts',(19.1949777051892,3.33294514719756,39.8531348114845));
#39068=CARTESIAN_POINT('Ctrl Pts',(19.1949104215934,3.33294031635255,39.8531039139543));
#39069=CARTESIAN_POINT('Ctrl Pts',(19.1947777435711,3.33293078978758,39.8530429771771));
#39070=CARTESIAN_POINT('Ctrl Pts',(19.1947123483465,3.33292609402465,39.8530129378223));
#39071=CARTESIAN_POINT('Ctrl Pts',(19.1945833879339,3.33291683342051,39.8529536910029));
#39072=CARTESIAN_POINT('Ctrl Pts',(19.194519821919,3.33291226853342,39.8529244834023));
#39073=CARTESIAN_POINT('Ctrl Pts',(19.1943944626362,3.332903265607,39.8528668744925));
#39074=CARTESIAN_POINT('Ctrl Pts',(19.1943326685502,3.33289882752165,39.8528384730369));
#39075=CARTESIAN_POINT('Ctrl Pts',(19.1942107983545,3.33289007430297,39.8527824519268));
#39076=CARTESIAN_POINT('Ctrl Pts',(19.1941507210981,3.33288575909927,39.8527548319614));
#39077=CARTESIAN_POINT('Ctrl Pts',(19.1940322345453,3.33287724808706,39.8527003514805));
#39078=CARTESIAN_POINT('Ctrl Pts',(19.193973824156,3.33287305221163,39.8526734906676));
#39079=CARTESIAN_POINT('Ctrl Pts',(19.1938586030765,3.3328647749856,39.8526204977049));
#39080=CARTESIAN_POINT('Ctrl Pts',(19.1938018015442,3.33286069430381,39.8525943699601));
#39081=CARTESIAN_POINT('Ctrl Pts',(19.1936897607892,3.33285264481112,39.852542826507));
#39082=CARTESIAN_POINT('Ctrl Pts',(19.193634521446,3.33284867600164,39.8525174109245));
#39083=CARTESIAN_POINT('Ctrl Pts',(19.1935255569654,3.33284084682734,39.8524672702022));
#39084=CARTESIAN_POINT('Ctrl Pts',(19.1934718317688,3.33283698646777,39.8524425452058));
#39085=CARTESIAN_POINT('Ctrl Pts',(19.19336584887,3.33282937086509,39.852393764666));
#39086=CARTESIAN_POINT('Ctrl Pts',(19.1933135912527,3.33282561563704,39.8523697093228));
#39087=CARTESIAN_POINT('Ctrl Pts',(19.1932104990866,3.33281820713157,39.8523222481176));
#39088=CARTESIAN_POINT('Ctrl Pts',(19.1931596643523,3.33281455384927,39.8522988423222));
#39089=CARTESIAN_POINT('Ctrl Pts',(19.1930593744085,3.33280734613107,39.8522526606156));
#39090=CARTESIAN_POINT('Ctrl Pts',(19.1930099191916,3.33280379170262,39.8522298848443));
#39091=CARTESIAN_POINT('Ctrl Pts',(19.1862562440235,3.33231837458077,39.849119246355));
#39092=CARTESIAN_POINT('Ctrl Pts',(19.1795698800316,3.33183519942183,39.8459929707942));
#39093=CARTESIAN_POINT('Ctrl Pts',(19.1609340160753,3.33048115245289,39.8371489038218));
#39094=CARTESIAN_POINT('Ctrl Pts',(19.1490254109,3.32960737779564,39.8313463758972));
#39095=CARTESIAN_POINT('Ctrl Pts',(19.122513678488,3.32764261494977,39.8180887987205));
#39096=CARTESIAN_POINT('Ctrl Pts',(19.1079440755324,3.32654944694703,39.8105693684809));
#39097=CARTESIAN_POINT('Ctrl Pts',(19.0626998276581,3.32311185895985,39.7864834023164));
#39098=CARTESIAN_POINT('Ctrl Pts',(19.0323786655581,3.32074552658446,39.7692712705601));
#39099=CARTESIAN_POINT('Ctrl Pts',(18.9152349315449,3.31135278730419,39.6985090626837));
#39100=CARTESIAN_POINT('Ctrl Pts',(18.8322578005596,3.3041327295335,39.6389347527952));
#39101=CARTESIAN_POINT('Ctrl Pts',(18.6634585832339,3.28836582766895,39.4962017405979));
#39102=CARTESIAN_POINT('Ctrl Pts',(18.5798357193322,3.27983032609332,39.4110533821716));
#39103=CARTESIAN_POINT('Ctrl Pts',(18.4953586505283,3.27076582689681,39.307398300588));
#39104=CARTESIAN_POINT('Ctrl Pts',(18.4862523798787,3.26978237502493,39.2959617138258));
#39105=CARTESIAN_POINT('Ctrl Pts',(18.4738317434508,3.26843335481722,39.2799934288007));
#39106=CARTESIAN_POINT('Ctrl Pts',(18.4704061092114,3.26806046925801,39.2755494759969));
#39107=CARTESIAN_POINT('Ctrl Pts',(18.4649547370027,3.26746583835805,39.2684134315649));
#39108=CARTESIAN_POINT('Ctrl Pts',(18.4629166103936,3.26724324026399,39.2657309124936));
#39109=CARTESIAN_POINT('Ctrl Pts',(18.4586825288022,3.26678024264511,39.260127735203));
#39110=CARTESIAN_POINT('Ctrl Pts',(18.4564878356473,3.2665399363093,39.2572061647643));
#39111=CARTESIAN_POINT('Ctrl Pts',(18.4512011675586,3.26596026427782,39.2501267673303));
#39112=CARTESIAN_POINT('Ctrl Pts',(18.4481175873644,3.26562147749728,39.2459626447587));
#39113=CARTESIAN_POINT('Ctrl Pts',(18.4373909288732,3.26444037765165,39.2313544712812));
#39114=CARTESIAN_POINT('Ctrl Pts',(18.4298359957502,3.26360387987085,39.2208456943403));
#39115=CARTESIAN_POINT('Ctrl Pts',(18.3852992776554,3.25863936253422,39.157561766277));
#39116=CARTESIAN_POINT('Ctrl Pts',(18.3508711473351,3.25466098733777,39.1030309771968));
#39117=CARTESIAN_POINT('Ctrl Pts',(18.2569194275424,3.24304235477764,38.9362601942));
#39118=CARTESIAN_POINT('Ctrl Pts',(18.2056753856786,3.23560300123534,38.8197651313276));
#39119=CARTESIAN_POINT('Ctrl Pts',(18.1535277955956,3.22540677745552,38.6601433722484));
#39120=CARTESIAN_POINT('Ctrl Pts',(18.1420520435353,3.22289657108618,38.6208160000969));
#39121=CARTESIAN_POINT('Ctrl Pts',(18.1207279500748,3.2175848628011,38.5380216842226));
#39122=CARTESIAN_POINT('Ctrl Pts',(18.1111166947998,3.21477867284623,38.4945197203968));
#39123=CARTESIAN_POINT('Ctrl Pts',(18.1007824823921,3.21113595460981,38.4386249178573));
#39124=CARTESIAN_POINT('Ctrl Pts',(18.0986609354056,3.21034374109631,38.426502318923));
#39125=CARTESIAN_POINT('Ctrl Pts',(18.0954795121904,3.20908115485691,38.407239896711));
#39126=CARTESIAN_POINT('Ctrl Pts',(18.0943434429813,3.20861318319632,38.4001128570536));
#39127=CARTESIAN_POINT('Ctrl Pts',(18.0923780460689,3.20777176754015,38.387321780416));
#39128=CARTESIAN_POINT('Ctrl Pts',(18.0915338824086,3.2073987946462,38.3816600813881));
#39129=CARTESIAN_POINT('Ctrl Pts',(18.0898485791259,3.2066296217493,38.3700014383462));
#39130=CARTESIAN_POINT('Ctrl Pts',(18.0890104537975,3.2062333315492,38.3640041292778));
#39131=CARTESIAN_POINT('Ctrl Pts',(18.0872001154099,3.20534549390767,38.3505895431773));
#39132=CARTESIAN_POINT('Ctrl Pts',(18.0862427852809,3.20485348607942,38.343170388998));
#39133=CARTESIAN_POINT('Ctrl Pts',(18.0839541868887,3.20361832718392,38.3245829479623));
#39134=CARTESIAN_POINT('Ctrl Pts',(18.0826774073341,3.20287348971464,38.3134083527984));
#39135=CARTESIAN_POINT('Ctrl Pts',(18.0743662104803,3.19760127102859,38.2345597038922));
#39136=CARTESIAN_POINT('Ctrl Pts',(18.0708195264918,3.19296679823777,38.1665751630418));
#39137=CARTESIAN_POINT('Ctrl Pts',(18.0708705425584,3.18824125908482,38.0985531651523));
#39138=CARTESIAN_POINT('Ctrl Pts',(18.0708705408095,3.18824142121201,38.0985554989003));
#39139=CARTESIAN_POINT('Ctrl Pts',(18.0709626172183,3.17969875041658,37.9755875671282));
#39140=CARTESIAN_POINT('Ctrl Pts',(18.0828122062449,3.17086948894766,37.8529133384598));
#39141=CARTESIAN_POINT('Ctrl Pts',(18.1210858155559,3.1565976689777,37.6558418696555));
#39142=CARTESIAN_POINT('Ctrl Pts',(18.1405257136007,3.15112172667708,37.5804300173344));
#39143=CARTESIAN_POINT('Ctrl Pts',(18.168849811871,3.14488776678673,37.4928474918395));
#39144=CARTESIAN_POINT('Ctrl Pts',(18.1733798313619,3.14393089377516,37.4793519769664));
#39145=CARTESIAN_POINT('Ctrl Pts',(18.179827744326,3.14262359023829,37.460825161733));
#39146=CARTESIAN_POINT('Ctrl Pts',(18.1816177931501,3.14226615086213,37.4557503079314));
#39147=CARTESIAN_POINT('Ctrl Pts',(18.184672176106,3.14166547475043,37.4472051709506));
#39148=CARTESIAN_POINT('Ctrl Pts',(18.185925273283,3.14142158738759,37.4437309365291));
#39149=CARTESIAN_POINT('Ctrl Pts',(18.1883264429393,3.14095908577815,37.4371330796245));
#39150=CARTESIAN_POINT('Ctrl Pts',(18.1894726289196,3.14074035911772,37.4340088060122));
#39151=CARTESIAN_POINT('Ctrl Pts',(18.1924976491082,3.14016838021045,37.4258287316373));
#39152=CARTESIAN_POINT('Ctrl Pts',(18.1943896283659,3.13981590032939,37.4207777719108));
#39153=CARTESIAN_POINT('Ctrl Pts',(18.2010203899488,3.13859838487663,37.4032993365387));
#39154=CARTESIAN_POINT('Ctrl Pts',(18.2058666191329,3.13773943792469,37.3909126378704));
#39155=CARTESIAN_POINT('Ctrl Pts',(18.2642861115132,3.12772734579599,37.2460299206992));
#39156=CARTESIAN_POINT('Ctrl Pts',(18.3323038746261,3.11932527790169,37.1198111357329));
#39157=CARTESIAN_POINT('Ctrl Pts',(18.4553914536909,3.1063880510586,36.9419383734885));
#39158=CARTESIAN_POINT('Ctrl Pts',(18.5005321590342,3.10197762000265,36.884056965834));
#39159=CARTESIAN_POINT('Ctrl Pts',(18.5743967845471,3.09507801435943,36.7997305790491));
#39160=CARTESIAN_POINT('Ctrl Pts',(18.6008092646648,3.09266561422367,36.771350275337));
#39161=CARTESIAN_POINT('Ctrl Pts',(18.6404864019471,3.0891032463412,36.7312129838761));
#39162=CARTESIAN_POINT('Ctrl Pts',(18.6530872805532,3.08798046085748,36.7188116663069));
#39163=CARTESIAN_POINT('Ctrl Pts',(18.6759971329724,3.08595285232503,36.6968763178888));
#39164=CARTESIAN_POINT('Ctrl Pts',(18.6862432204556,3.08505080543691,36.687278241609));
#39165=CARTESIAN_POINT('Ctrl Pts',(18.7021770857202,3.08365477265673,36.6726753650743));
#39166=CARTESIAN_POINT('Ctrl Pts',(18.7077912551356,3.08316415732544,36.667590670481));
#39167=CARTESIAN_POINT('Ctrl Pts',(18.7134723617415,3.08266891377676,36.6625059320505));
#39168=CARTESIAN_POINT('Ctrl Pts',(18.7135095662566,3.08266567057094,36.6624726356415));
#39169=CARTESIAN_POINT('Ctrl Pts',(18.7135862850425,3.08265898292055,36.662403981057));
#39170=CARTESIAN_POINT('Ctrl Pts',(18.7136257994007,3.08265553847507,36.6623686231359));
#39171=CARTESIAN_POINT('Ctrl Pts',(18.7137073067292,3.08264843364679,36.6622956954529));
#39172=CARTESIAN_POINT('Ctrl Pts',(18.7137492998584,3.08264477325779,36.662258125928));
#39173=CARTESIAN_POINT('Ctrl Pts',(18.7138359488241,3.08263722051897,36.662180611498));
#39174=CARTESIAN_POINT('Ctrl Pts',(18.7138806049412,3.0826333281534,36.6621406667746));
#39175=CARTESIAN_POINT('Ctrl Pts',(18.7139727813229,3.08262529393003,36.662058223089));
#39176=CARTESIAN_POINT('Ctrl Pts',(18.7140203018249,3.08262115206151,36.6620157244094));
#39177=CARTESIAN_POINT('Ctrl Pts',(18.7141184275495,3.08261259963772,36.6619279770677));
#39178=CARTESIAN_POINT('Ctrl Pts',(18.7141690329902,3.08260818907488,36.661882728778));
#39179=CARTESIAN_POINT('Ctrl Pts',(18.7142735703587,3.08259907822612,36.6617892677862));
#39180=CARTESIAN_POINT('Ctrl Pts',(18.7143275026305,3.08259437792334,36.6617410554282));
#39181=CARTESIAN_POINT('Ctrl Pts',(18.7144389594826,3.08258466446811,36.6616414306731));
#39182=CARTESIAN_POINT('Ctrl Pts',(18.7144964844927,3.08257965129328,36.6615900186419));
#39183=CARTESIAN_POINT('Ctrl Pts',(18.7146154197221,3.08256928661462,36.6614837350708));
#39184=CARTESIAN_POINT('Ctrl Pts',(18.7146768304129,3.08256393508711,36.6614288639749));
#39185=CARTESIAN_POINT('Ctrl Pts',(18.7148038603794,3.08255286557648,36.6613153759958));
#39186=CARTESIAN_POINT('Ctrl Pts',(18.7148694801646,3.0825471475691,36.6612567596582));
#39187=CARTESIAN_POINT('Ctrl Pts',(18.7150052862623,3.08253531396997,36.6611354645343));
#39188=CARTESIAN_POINT('Ctrl Pts',(18.7150754730873,3.08252919835688,36.6610727864506));
#39189=CARTESIAN_POINT('Ctrl Pts',(18.7152208101716,3.08251653503415,36.6609430169612));
#39190=CARTESIAN_POINT('Ctrl Pts',(18.7152959610692,3.082509987296,36.6608759263345));
#39191=CARTESIAN_POINT('Ctrl Pts',(18.7154516675819,3.08249642135833,36.6607369419596));
#39192=CARTESIAN_POINT('Ctrl Pts',(18.7155322240176,3.08248940311891,36.6606650490519));
#39193=CARTESIAN_POINT('Ctrl Pts',(18.7156992338346,3.08247485339189,36.660516025671));
#39194=CARTESIAN_POINT('Ctrl Pts',(18.7157856881107,3.08246732186327,36.6604388962389));
#39195=CARTESIAN_POINT('Ctrl Pts',(18.7159650437198,3.08245169774806,36.6602789147041));
#39196=CARTESIAN_POINT('Ctrl Pts',(18.7160579461528,3.08244360510896,36.6601960637789));
#39197=CARTESIAN_POINT('Ctrl Pts',(18.7162508149785,3.08242680516823,36.66002409576));
#39198=CARTESIAN_POINT('Ctrl Pts',(18.7163507826064,3.08241809780997,36.6599349801068));
#39199=CARTESIAN_POINT('Ctrl Pts',(18.7165584754023,3.08240000817572,36.6597498721897));
#39200=CARTESIAN_POINT('Ctrl Pts',(18.7166662020305,3.08239062583273,36.6596538816284));
#39201=CARTESIAN_POINT('Ctrl Pts',(18.7168587458894,3.08237385719388,36.6594823528331));
#39202=CARTESIAN_POINT('Ctrl Pts',(18.7169435590601,3.0823664710863,36.6594068099702));
#39203=CARTESIAN_POINT('Ctrl Pts',(18.7171507824376,3.0823484253228,36.6592222694792));
#39204=CARTESIAN_POINT('Ctrl Pts',(18.717273203459,3.08233776501619,36.6591132767623));
#39205=CARTESIAN_POINT('Ctrl Pts',(18.7175738838384,3.08231158342707,36.6588456465641));
#39206=CARTESIAN_POINT('Ctrl Pts',(18.717752156434,3.08229606161821,36.6586870286051));
#39207=CARTESIAN_POINT('Ctrl Pts',(18.7227175746267,3.08186376638179,36.6542707004457));
#39208=CARTESIAN_POINT('Ctrl Pts',(18.7275258218925,3.08144600778244,36.6500368742098));
#39209=CARTESIAN_POINT('Ctrl Pts',(18.7385405675419,3.08049088779077,36.6404349986686));
#39210=CARTESIAN_POINT('Ctrl Pts',(18.7447603728366,3.07995289873603,36.6350824706683));
#39211=CARTESIAN_POINT('Ctrl Pts',(18.7612933087796,3.07852629012478,36.6210374555612));
#39212=CARTESIAN_POINT('Ctrl Pts',(18.7716636290791,3.07763492672971,36.6124132902688));
#39213=CARTESIAN_POINT('Ctrl Pts',(18.8514254742044,3.07080422851566,36.5474844678337));
#39214=CARTESIAN_POINT('Ctrl Pts',(18.924553176691,3.06467716519431,36.4959620137343));
#39215=CARTESIAN_POINT('Ctrl Pts',(19.1248584470688,3.04825373440208,36.3747058490964));
#39216=CARTESIAN_POINT('Ctrl Pts',(19.2567338464206,3.03775841435496,36.3139334439782));
#39217=CARTESIAN_POINT('Ctrl Pts',(19.3941040093468,3.02765621357216,36.2684889829951));
#39218=CARTESIAN_POINT('Ctrl Pts',(19.3941039244954,2.85753017062829,36.2684890110654));
#39219=CARTESIAN_POINT('Ctrl Pts',(19.3606565940364,2.86003284017505,36.2795539767597));
#39220=CARTESIAN_POINT('Ctrl Pts',(19.3274997762525,2.86254735914615,36.291539331038));
#39221=CARTESIAN_POINT('Ctrl Pts',(19.217090903976,2.87101193801834,36.3349098074678));
#39222=CARTESIAN_POINT('Ctrl Pts',(19.1415620849291,2.87695947541409,36.3703826759163));
#39223=CARTESIAN_POINT('Ctrl Pts',(19.0369204836252,2.88524193442019,36.4280771993552));
#39224=CARTESIAN_POINT('Ctrl Pts',(19.0057737880163,2.88771226505888,36.4464091623806));
#39225=CARTESIAN_POINT('Ctrl Pts',(18.9688575436691,2.89063021769136,36.4695573921715));
#39226=CARTESIAN_POINT('Ctrl Pts',(18.9625797377048,2.8911260707425,36.4735446312671));
#39227=CARTESIAN_POINT('Ctrl Pts',(18.9528396766222,2.89189463614446,36.4798101998695));
#39228=CARTESIAN_POINT('Ctrl Pts',(18.9493615242401,2.89216893803576,36.4820634977358));
#39229=CARTESIAN_POINT('Ctrl Pts',(18.942909585528,2.892677444386,36.4862729221553));
#39230=CARTESIAN_POINT('Ctrl Pts',(18.939933979045,2.89291183305399,36.4882260525492));
#39231=CARTESIAN_POINT('Ctrl Pts',(18.933182269606,2.8934433820139,36.4926845294928));
#39232=CARTESIAN_POINT('Ctrl Pts',(18.9294095840057,2.89374020034283,36.4951949483408));
#39233=CARTESIAN_POINT('Ctrl Pts',(18.9179241961722,2.89464332956517,36.5028960774762));
#39234=CARTESIAN_POINT('Ctrl Pts',(18.9102399994164,2.89524688189357,36.5081293601266));
#39235=CARTESIAN_POINT('Ctrl Pts',(18.8388727186767,2.90084906322997,36.5574926490255));
#39236=CARTESIAN_POINT('Ctrl Pts',(18.7778561464931,2.90561493726354,36.6053719517119));
#39237=CARTESIAN_POINT('Ctrl Pts',(18.6412756796865,2.91665279091833,36.7265189500819));
#39238=CARTESIAN_POINT('Ctrl Pts',(18.5684994543961,2.92284534630685,36.802545196496));
#39239=CARTESIAN_POINT('Ctrl Pts',(18.4619008066149,2.93305337383519,36.9338538260545));
#39240=CARTESIAN_POINT('Ctrl Pts',(18.4240317057074,2.93696623387303,36.9855633991839));
#39241=CARTESIAN_POINT('Ctrl Pts',(18.3680051820332,2.94333261595461,37.0706477270633));
#39242=CARTESIAN_POINT('Ctrl Pts',(18.348138474401,2.94572578419467,37.1028408433733));
#39243=CARTESIAN_POINT('Ctrl Pts',(18.3236564332125,2.94886929523905,37.1452543884238));
#39244=CARTESIAN_POINT('Ctrl Pts',(18.3181650374371,2.94958809106539,37.1549613304519));
#39245=CARTESIAN_POINT('Ctrl Pts',(18.309382863252,2.95076047560509,37.1708042597458));
#39246=CARTESIAN_POINT('Ctrl Pts',(18.3060405412513,2.95121222798076,37.1769115011092));
#39247=CARTESIAN_POINT('Ctrl Pts',(18.2996823790901,2.95208246985336,37.188680247262));
#39248=CARTESIAN_POINT('Ctrl Pts',(18.2966615697999,2.9525007767508,37.1943389738711));
#39249=CARTESIAN_POINT('Ctrl Pts',(18.2898152521597,2.95346007202808,37.2073192484962));
#39250=CARTESIAN_POINT('Ctrl Pts',(18.28600845766,2.95400170734519,37.2146504729416));
#39251=CARTESIAN_POINT('Ctrl Pts',(18.276025428328,2.95544435569914,37.2341817636596));
#39252=CARTESIAN_POINT('Ctrl Pts',(18.2699317166256,2.95634821223243,37.2464232543445));
#39253=CARTESIAN_POINT('Ctrl Pts',(18.2206881797153,2.96384976562581,37.3480412096713));
#39254=CARTESIAN_POINT('Ctrl Pts',(18.1843712913556,2.97068114028936,37.4405461961855));
#39255=CARTESIAN_POINT('Ctrl Pts',(18.1283939640001,2.98415466143783,37.6234425681543));
#39256=CARTESIAN_POINT('Ctrl Pts',(18.1077895144003,2.99075596854252,37.7132773812141));
#39257=CARTESIAN_POINT('Ctrl Pts',(18.0894152127722,2.99927813992268,37.8317068334954));
#39258=CARTESIAN_POINT('Ctrl Pts',(18.0857471412592,3.00124835183975,37.8592687770811));
#39259=CARTESIAN_POINT('Ctrl Pts',(18.0766766357657,3.00702870372052,37.9408791946194));
#39260=CARTESIAN_POINT('Ctrl Pts',(18.0729588246628,3.01080012689968,37.9950921738115));
#39261=CARTESIAN_POINT('Ctrl Pts',(18.0712230541167,3.01526575877315,38.0612387957881));
#39262=CARTESIAN_POINT('Ctrl Pts',(18.07102136121,3.01606024452581,38.0730859472011));
#39263=CARTESIAN_POINT('Ctrl Pts',(18.0708897744506,3.01718189750547,38.0899351242414));
#39264=CARTESIAN_POINT('Ctrl Pts',(18.0708701650209,3.01751376283918,38.0949358885933));
#39265=CARTESIAN_POINT('Ctrl Pts',(18.0708698822856,3.01808411229999,38.1035581921408));
#39266=CARTESIAN_POINT('Ctrl Pts',(18.0708799610129,3.01832310323502,38.107179684489));
#39267=CARTESIAN_POINT('Ctrl Pts',(18.0709220493142,3.01881797255005,38.1146966758045));
#39268=CARTESIAN_POINT('Ctrl Pts',(18.0709556599471,3.01907376149468,38.118592118772));
#39269=CARTESIAN_POINT('Ctrl Pts',(18.0710746585202,3.0197423732211,38.1287999393209));
#39270=CARTESIAN_POINT('Ctrl Pts',(18.0711792328244,3.02015414569974,38.1351121109923));
#39271=CARTESIAN_POINT('Ctrl Pts',(18.0717819535514,3.02197780612953,38.1631747124895));
#39272=CARTESIAN_POINT('Ctrl Pts',(18.0726170531775,3.0233720777768,38.1849173283251));
#39273=CARTESIAN_POINT('Ctrl Pts',(18.0759119799343,3.02714858187199,38.2444305307918));
#39274=CARTESIAN_POINT('Ctrl Pts',(18.079115810438,3.02949823566847,38.2821515514698));
#39275=CARTESIAN_POINT('Ctrl Pts',(18.0939605533097,3.03748445652043,38.4116178669593));
#39276=CARTESIAN_POINT('Ctrl Pts',(18.1110848353842,3.04296581959771,38.5026082776116));
#39277=CARTESIAN_POINT('Ctrl Pts',(18.1678688506281,3.05627763384533,38.7178843701909));
#39278=CARTESIAN_POINT('Ctrl Pts',(18.2137147134431,3.06413886766502,38.8400430351));
#39279=CARTESIAN_POINT('Ctrl Pts',(18.2776273340055,3.07332731941447,38.9690023519358));
#39280=CARTESIAN_POINT('Ctrl Pts',(18.2838825347054,3.07421198771667,38.9812908247222));
#39281=CARTESIAN_POINT('Ctrl Pts',(18.2941104295105,3.07563611745089,39.0008618787903));
#39282=CARTESIAN_POINT('Ctrl Pts',(18.2979993733752,3.07617265626179,39.0081878741759));
#39283=CARTESIAN_POINT('Ctrl Pts',(18.3049818771035,3.07712742112649,39.0211391486641));
#39284=CARTESIAN_POINT('Ctrl Pts',(18.3080565194163,3.07754497562069,39.0267745275963));
#39285=CARTESIAN_POINT('Ctrl Pts',(18.3145166126529,3.07841644298993,39.0384756586106));
#39286=CARTESIAN_POINT('Ctrl Pts',(18.3179068081447,3.07887051990703,39.0445386718518));
#39287=CARTESIAN_POINT('Ctrl Pts',(18.326790392616,3.08005206612961,39.0602265257058));
#39288=CARTESIAN_POINT('Ctrl Pts',(18.3323340424217,3.08078132343595,39.0698224663245));
#39289=CARTESIAN_POINT('Ctrl Pts',(18.356818837048,3.08396810926838,39.1113743937927));
#39290=CARTESIAN_POINT('Ctrl Pts',(18.3765969939247,3.08645565417387,39.1428254195511));
#39291=CARTESIAN_POINT('Ctrl Pts',(18.4320071721571,3.09320842091878,39.2255383624308));
#39292=CARTESIAN_POINT('Ctrl Pts',(18.4692375184685,3.09752884194965,39.2756713045008));
#39293=CARTESIAN_POINT('Ctrl Pts',(18.5959967078172,3.11156251566992,39.4301107518972));
#39294=CARTESIAN_POINT('Ctrl Pts',(18.6942546102255,3.12150813881917,39.5266906211271));
#39295=CARTESIAN_POINT('Ctrl Pts',(18.8118494723276,3.13201024246337,39.6198687195273));
#39296=CARTESIAN_POINT('Ctrl Pts',(18.8218421960231,3.13289243296248,39.6276278351887));
#39297=CARTESIAN_POINT('Ctrl Pts',(18.8615795268422,3.13635838779042,39.6578610831623));
#39298=CARTESIAN_POINT('Ctrl Pts',(18.8918988828837,3.13891087913397,39.6795710458001));
#39299=CARTESIAN_POINT('Ctrl Pts',(18.9287491881109,3.14188839636503,39.7043737568169));
#39300=CARTESIAN_POINT('Ctrl Pts',(18.9346898163073,3.14236463810694,39.7083244914924));
#39301=CARTESIAN_POINT('Ctrl Pts',(18.9444141773534,3.14313791895853,39.7147140270134));
#39302=CARTESIAN_POINT('Ctrl Pts',(18.9481847049677,3.14343622135924,39.7171726574992));
#39303=CARTESIAN_POINT('Ctrl Pts',(18.9549502058018,3.14396868716129,39.7215505348805));
#39304=CARTESIAN_POINT('Ctrl Pts',(18.9579419022527,3.14420317184882,39.7234747091133));
#39305=CARTESIAN_POINT('Ctrl Pts',(18.9644493866687,3.14471110848823,39.7276347388192));
#39306=CARTESIAN_POINT('Ctrl Pts',(18.9679670926901,3.14498435562395,39.7298674776873));
#39307=CARTESIAN_POINT('Ctrl Pts',(18.9778701396599,3.1457499689596,39.736108169004));
#39308=CARTESIAN_POINT('Ctrl Pts',(18.984271867837,3.1462406682692,39.740090167696));
#39309=CARTESIAN_POINT('Ctrl Pts',(19.0230029439931,3.14918511777159,39.7638678879222));
#39310=CARTESIAN_POINT('Ctrl Pts',(19.0558892159563,3.15158359635412,39.7827462338069));
#39311=CARTESIAN_POINT('Ctrl Pts',(19.2373648379795,3.16439516233087,39.8799255526703));
#39312=CARTESIAN_POINT('Ctrl Pts',(19.3951456018111,3.17408508161758,39.9395405972609));
#39313=CARTESIAN_POINT('Ctrl Pts',(19.5950314304877,3.18658919610805,39.9865148925349));
#39314=CARTESIAN_POINT('Ctrl Pts',(19.6316350870102,3.18888475112402,39.9940023886546));
#39315=CARTESIAN_POINT('Ctrl Pts',(19.7102353174229,3.19384976857441,40.0077158410235));
#39316=CARTESIAN_POINT('Ctrl Pts',(19.7522655753833,3.19652629059773,40.0136275852931));
#39317=CARTESIAN_POINT('Ctrl Pts',(19.8064844367045,3.20002178832332,40.0194375922835));
#39318=CARTESIAN_POINT('Ctrl Pts',(19.8185262460074,3.20080079419798,40.0206134982633));
#39319=CARTESIAN_POINT('Ctrl Pts',(19.8377216143814,3.20204715013185,40.0223058312568));
#39320=CARTESIAN_POINT('Ctrl Pts',(19.8448685024871,3.20251220527648,40.0228957848792));
#39321=CARTESIAN_POINT('Ctrl Pts',(19.8577316769104,3.20335110410796,40.0238854216106));
#39322=CARTESIAN_POINT('Ctrl Pts',(19.8634467968227,3.20372449420392,40.0242995122275));
#39323=CARTESIAN_POINT('Ctrl Pts',(19.8768527272242,3.20460195704782,40.0252108200386));
#39324=CARTESIAN_POINT('Ctrl Pts',(19.8845447963421,3.20510666537722,40.0256874215289));
#39325=CARTESIAN_POINT('Ctrl Pts',(19.906796583996,3.2065703811387,40.0269323429763));
#39326=CARTESIAN_POINT('Ctrl Pts',(19.9213621617662,3.20753306285815,40.0275816978332));
#39327=CARTESIAN_POINT('Ctrl Pts',(20.0370742272766,3.21521864588983,40.0314266298124));
#39328=CARTESIAN_POINT('Ctrl Pts',(20.1383057442437,3.22218461519501,40.0268235137575));
#39329=CARTESIAN_POINT('Ctrl Pts',(20.3575865011105,3.23775651747657,39.9994813268921));
#39330=CARTESIAN_POINT('Ctrl Pts',(20.4748322496389,3.24639959752661,39.9736142241968));
#39331=CARTESIAN_POINT('Ctrl Pts',(20.6003917854264,3.25567756394384,39.9333623264736));
#39332=CARTESIAN_POINT('Ctrl Pts',(20.6118303366539,3.25652278487469,39.9295768267147));
#39333=CARTESIAN_POINT('Ctrl Pts',(20.6673239656198,3.26062114142124,39.9106329973402));
#39334=CARTESIAN_POINT('Ctrl Pts',(20.710859670402,3.2638298946142,39.8939878679183));
#39335=CARTESIAN_POINT('Ctrl Pts',(20.7607557653881,3.26746699746689,39.8728088125102));
#39336=CARTESIAN_POINT('Ctrl Pts',(20.7677403915589,3.2679751838393,39.8697952186996));
#39337=CARTESIAN_POINT('Ctrl Pts',(20.7789144816431,3.26878645291078,39.8648954338632));
#39338=CARTESIAN_POINT('Ctrl Pts',(20.7831152646312,3.26909104581512,39.8630354918629));
#39339=CARTESIAN_POINT('Ctrl Pts',(20.7905715975828,3.26963093854884,39.8597022118905));
#39340=CARTESIAN_POINT('Ctrl Pts',(20.7938297421493,3.26986659222329,39.8582348155809));
#39341=CARTESIAN_POINT('Ctrl Pts',(20.8007748522966,3.27036834685185,39.8550836506415));
#39342=CARTESIAN_POINT('Ctrl Pts',(20.8044605884069,3.27063428870413,39.8533973158611));
#39343=CARTESIAN_POINT('Ctrl Pts',(20.8145170219371,3.27135905557493,39.8487578116812));
#39344=CARTESIAN_POINT('Ctrl Pts',(20.820877031485,3.2718164880243,39.8457814198315));
#39345=CARTESIAN_POINT('Ctrl Pts',(20.8542038708978,3.27420928072242,39.829962551754));
#39346=CARTESIAN_POINT('Ctrl Pts',(20.8808877082171,3.27611069433907,39.8165289883437));
#39347=CARTESIAN_POINT('Ctrl Pts',(21.0503796740883,3.28816318876497,39.7262068387402));
#39348=CARTESIAN_POINT('Ctrl Pts',(21.1833339428641,3.29754861330043,39.6321812574369));
#39349=CARTESIAN_POINT('Ctrl Pts',(21.368990712367,3.31277746034923,39.462139432262));
#39350=CARTESIAN_POINT('Ctrl Pts',(21.4307202180323,3.31829438936203,39.3971491521977));
#39351=CARTESIAN_POINT('Ctrl Pts',(21.4962705972888,3.32487084475763,39.3177428700691));
#39352=CARTESIAN_POINT('Ctrl Pts',(21.5047227649264,3.32573391964674,39.3072832244121));
#39353=CARTESIAN_POINT('Ctrl Pts',(21.5181479012924,3.32712988330401,39.2903094762243));
#39354=CARTESIAN_POINT('Ctrl Pts',(21.5231900190743,3.32766003256288,39.2838504389381));
#39355=CARTESIAN_POINT('Ctrl Pts',(21.5320997429895,3.32860747302606,39.2722857832726));
#39356=CARTESIAN_POINT('Ctrl Pts',(21.5359833825756,3.32902412799145,39.2671926263201));
#39357=CARTESIAN_POINT('Ctrl Pts',(21.5440547353663,3.32989785572525,39.2564974922133));
#39358=CARTESIAN_POINT('Ctrl Pts',(21.5482374831827,3.3303551130889,39.2508919014435));
#39359=CARTESIAN_POINT('Ctrl Pts',(21.5590969714671,3.3315541306618,39.2361720111342));
#39360=CARTESIAN_POINT('Ctrl Pts',(21.5657242102423,3.3322977790176,39.2270216917204));
#39361=CARTESIAN_POINT('Ctrl Pts',(21.5950201538103,3.33563956212094,39.1858152331914));
#39362=CARTESIAN_POINT('Ctrl Pts',(21.6167860662026,3.33827144585541,39.1531317331278));
#39363=CARTESIAN_POINT('Ctrl Pts',(21.7241729661074,3.35207317478636,38.9806972879289));
#39364=CARTESIAN_POINT('Ctrl Pts',(21.792716199008,3.36384821357922,38.8311298154114));
#39365=CARTESIAN_POINT('Ctrl Pts',(21.8656912555979,3.38124435133031,38.5973109541305));
#39366=CARTESIAN_POINT('Ctrl Pts',(21.8849528545098,3.38693818482651,38.5184232493386));
#39367=CARTESIAN_POINT('Ctrl Pts',(21.9008291882576,3.393018358466,38.4293600797896));
#39368=CARTESIAN_POINT('Ctrl Pts',(21.9024004326275,3.393642326996,38.4201597532931));
#39369=CARTESIAN_POINT('Ctrl Pts',(21.9046364626845,3.39456437833259,38.4064687620989));
#39370=CARTESIAN_POINT('Ctrl Pts',(21.9053522425979,3.39486520157069,38.401986737793));
#39371=CARTESIAN_POINT('Ctrl Pts',(21.9066012054349,3.39540038691316,38.3939848185075));
#39372=CARTESIAN_POINT('Ctrl Pts',(21.9071404684264,3.39563508431498,38.3904659437615));
#39373=CARTESIAN_POINT('Ctrl Pts',(21.9082856586623,3.39614145866971,38.3828524944419));
#39374=CARTESIAN_POINT('Ctrl Pts',(21.9088881488409,3.39641294161807,38.3787574656925));
#39375=CARTESIAN_POINT('Ctrl Pts',(21.9105329131224,3.39716863498561,38.3673228381058));
#39376=CARTESIAN_POINT('Ctrl Pts',(21.9115460815999,3.39765124716439,38.3599790263823));
#39377=CARTESIAN_POINT('Ctrl Pts',(21.9171965677959,3.40044749505698,38.3172023349757));
#39378=CARTESIAN_POINT('Ctrl Pts',(21.9208913192791,3.40271212805838,38.2816492978243));
#39379=CARTESIAN_POINT('Ctrl Pts',(21.929784166013,3.4100401041277,38.1644924340166));
#39380=CARTESIAN_POINT('Ctrl Pts',(21.9307841933275,3.41494743721398,38.0826553543596));
#39381=CARTESIAN_POINT('Ctrl Pts',(21.918766757882,3.42894686422972,37.8488000130439));
#39382=CARTESIAN_POINT('Ctrl Pts',(21.8929412888471,3.43798567802056,37.6980866919558));
#39383=CARTESIAN_POINT('Ctrl Pts',(21.8434727859557,3.44902021139449,37.5311200991605));
#39384=CARTESIAN_POINT('Ctrl Pts',(21.8369375769129,3.45040992751758,37.5103589806116));
#39385=CARTESIAN_POINT('Ctrl Pts',(21.8273997796909,3.45235087965272,37.4817581967076));
#39386=CARTESIAN_POINT('Ctrl Pts',(21.8246950267113,3.45289241822277,37.4738203628228));
#39387=CARTESIAN_POINT('Ctrl Pts',(21.8199502567549,3.45382752121336,37.4601873604978));
#39388=CARTESIAN_POINT('Ctrl Pts',(21.8179350321529,3.45422026836438,37.4544836421762));
#39389=CARTESIAN_POINT('Ctrl Pts',(21.8137179363228,3.45503318827303,37.4427243177723));
#39390=CARTESIAN_POINT('Ctrl Pts',(21.8115124883044,3.45545347483833,37.4366700835791));
#39391=CARTESIAN_POINT('Ctrl Pts',(21.8062950554161,3.45643663635152,37.4225676606151));
#39392=CARTESIAN_POINT('Ctrl Pts',(21.8032595617032,3.45700028419012,37.4145283734796));
#39393=CARTESIAN_POINT('Ctrl Pts',(21.7932968783317,3.45882391198117,37.3886671180075));
#39394=CARTESIAN_POINT('Ctrl Pts',(21.7861585833522,3.4600908843147,37.3709282384805));
#39395=CARTESIAN_POINT('Ctrl Pts',(21.7483754508612,3.46660414451008,37.2809229456293));
#39396=CARTESIAN_POINT('Ctrl Pts',(21.7136079033426,3.47198792406805,37.2104781801012));
#39397=CARTESIAN_POINT('Ctrl Pts',(21.6332505120093,3.48331934721461,37.0699559286707));
#39398=CARTESIAN_POINT('Ctrl Pts',(21.5872008859281,3.48926990723426,37.0003228609735));
#39399=CARTESIAN_POINT('Ctrl Pts',(21.4706451992611,3.50302697117811,36.8467160860199));
#39400=CARTESIAN_POINT('Ctrl Pts',(21.397190430497,3.51081236917967,36.7653155435785));
#39401=CARTESIAN_POINT('Ctrl Pts',(21.3105229159966,3.51878263051532,36.6843177365225));
#39402=CARTESIAN_POINT('Ctrl Pts',(21.3037810629325,3.519395333194,36.6781063567993));
#39403=CARTESIAN_POINT('Ctrl Pts',(21.2936596427981,3.52030401011307,36.6689138436782));
#39404=CARTESIAN_POINT('Ctrl Pts',(21.290313611638,3.52060261254146,36.6658962231185));
#39405=CARTESIAN_POINT('Ctrl Pts',(21.2843069233402,3.52113540054059,36.6605171281088));
#39406=CARTESIAN_POINT('Ctrl Pts',(21.2816502880951,3.52136990906736,36.6581512730098));
#39407=CARTESIAN_POINT('Ctrl Pts',(21.2758704535842,3.52187765304127,36.6530326632327));
#39408=CARTESIAN_POINT('Ctrl Pts',(21.2727448907782,3.52215068498439,36.650282671757));
#39409=CARTESIAN_POINT('Ctrl Pts',(21.2639458820651,3.52291508614333,36.6425913518342));
#39410=CARTESIAN_POINT('Ctrl Pts',(21.2582523196022,3.52340479692815,36.6376729964587));
#39411=CARTESIAN_POINT('Ctrl Pts',(21.2239073391883,3.52633056760956,36.6083533628937));
#39412=CARTESIAN_POINT('Ctrl Pts',(21.1945734436347,3.52871216800814,36.5847595545678));
#39413=CARTESIAN_POINT('Ctrl Pts',(21.0331277234954,3.54131866137796,36.4625107149812));
#39414=CARTESIAN_POINT('Ctrl Pts',(20.8894641921953,3.55084323614717,36.3802360006423));
#39415=CARTESIAN_POINT('Ctrl Pts',(20.6642805108857,3.56565781676785,36.2871352227005));
#39416=CARTESIAN_POINT('Ctrl Pts',(20.5897198160718,3.57053650479522,36.2615290164322));
#39417=CARTESIAN_POINT('Ctrl Pts',(20.5011492577656,3.57640794543208,36.2370548903965));
#39418=CARTESIAN_POINT('Ctrl Pts',(20.4884545017127,3.57725115478762,36.2336861876901));
#39419=CARTESIAN_POINT('Ctrl Pts',(20.4677906724299,3.57862682006475,36.2284280670368));
#39420=CARTESIAN_POINT('Ctrl Pts',(20.4598420855925,3.57915673395525,36.2264592701559));
#39421=CARTESIAN_POINT('Ctrl Pts',(20.4456725551757,3.58010281668604,36.2230452011473));
#39422=CARTESIAN_POINT('Ctrl Pts',(20.4394564787172,3.58051834554433,36.2215800935219));
#39423=CARTESIAN_POINT('Ctrl Pts',(20.426346663231,3.58139578418474,36.2185587906178));
#39424=CARTESIAN_POINT('Ctrl Pts',(20.4194514319023,3.58185790900996,36.2170095603926));
#39425=CARTESIAN_POINT('Ctrl Pts',(20.401188663845,3.58308363503248,36.2130115449745));
#39426=CARTESIAN_POINT('Ctrl Pts',(20.3898073719483,3.58384928145929,36.210627623742));
#39427=CARTESIAN_POINT('Ctrl Pts',(20.3365028435584,3.58744402788592,36.1999646106391));
#39428=CARTESIAN_POINT('Ctrl Pts',(20.2943363829374,3.590313478552,36.1929776484724));
#39429=CARTESIAN_POINT('Ctrl Pts',(20.0866916685304,3.60458156266655,36.1656215506618));
#39430=CARTESIAN_POINT('Ctrl Pts',(19.919300113629,3.6165942432145,36.1653669394137));
#39431=CARTESIAN_POINT('Ctrl Pts',(19.7245752579247,3.63050769669728,36.1904021273118));
#39432=CARTESIAN_POINT('Ctrl Pts',(19.6952383133604,3.63259952211904,36.1948639784605));
#39433=CARTESIAN_POINT('Ctrl Pts',(19.6207342097879,3.63788445187441,36.2079604331612));
#39434=CARTESIAN_POINT('Ctrl Pts',(19.5757480278968,3.64104970535346,36.2175369025958));
#39435=CARTESIAN_POINT('Ctrl Pts',(19.5237909081485,3.64464354099556,36.2305549199736));
#39436=CARTESIAN_POINT('Ctrl Pts',(19.5164493996503,3.6451498843845,36.2324404084693));
#39437=CARTESIAN_POINT('Ctrl Pts',(19.5046839739135,3.64595878512668,36.2355361030975));
#39438=CARTESIAN_POINT('Ctrl Pts',(19.500253017933,3.64626283901879,36.2367188769425));
#39439=CARTESIAN_POINT('Ctrl Pts',(19.4923780768534,3.64680212770163,36.2388510801924));
#39440=CARTESIAN_POINT('Ctrl Pts',(19.4889324658017,3.64703771342144,36.2397942869541));
#39441=CARTESIAN_POINT('Ctrl Pts',(19.4815783484048,3.64753971901391,36.2418293900072));
#39442=CARTESIAN_POINT('Ctrl Pts',(19.477670667882,3.64780597774356,36.2429240472601));
#39443=CARTESIAN_POINT('Ctrl Pts',(19.4669894898028,3.64853250512679,36.2459525432283));
#39444=CARTESIAN_POINT('Ctrl Pts',(19.4602230009392,3.64899136983806,36.2479111870733));
#39445=CARTESIAN_POINT('Ctrl Pts',(19.4335812699271,3.65079313461476,36.2557813737182));
#39446=CARTESIAN_POINT('Ctrl Pts',(19.4137909377445,3.65212070577368,36.2619762015326));
#39447=CARTESIAN_POINT('Ctrl Pts',(19.3941040086362,3.65343403802913,36.2684889832302));
#39448=CARTESIAN_POINT('Origin',(20.,-1.3495818343519,38.1));
#39449=CARTESIAN_POINT('',(19.3941040488142,4.61690666843697,36.2684889699386));
#39450=CARTESIAN_POINT('',(19.3941039894965,4.44426476764078,36.2684889895619));
#39451=CARTESIAN_POINT('',(19.3941040087494,-1.3495818343519,36.2684889831927));
#39452=CARTESIAN_POINT('Ctrl Pts',(19.3941040488142,4.61690666843697,36.2684889699386));
#39453=CARTESIAN_POINT('Ctrl Pts',(19.4217433849466,4.61516042926103,36.259345393088));
#39454=CARTESIAN_POINT('Ctrl Pts',(19.4495925545255,4.61340744069853,36.2508265292804));
#39455=CARTESIAN_POINT('Ctrl Pts',(19.5534307922853,4.6068707433316,36.2216180341652));
#39456=CARTESIAN_POINT('Ctrl Pts',(19.6304573128013,4.60201702819168,36.2049593908931));
#39457=CARTESIAN_POINT('Ctrl Pts',(19.7272129739756,4.5957950934203,36.1901579568729));
#39458=CARTESIAN_POINT('Ctrl Pts',(19.7461871599995,4.59456930132189,36.1875438850572));
#39459=CARTESIAN_POINT('Ctrl Pts',(19.77373178223,4.59278037058269,36.1841661879457));
#39460=CARTESIAN_POINT('Ctrl Pts',(19.7822737569181,4.59222428668319,36.183176643265));
#39461=CARTESIAN_POINT('Ctrl Pts',(19.7972283433773,4.59124832893086,36.1815454807755));
#39462=CARTESIAN_POINT('Ctrl Pts',(19.8036381325037,4.5908292433062,36.1808788202984));
#39463=CARTESIAN_POINT('Ctrl Pts',(19.8160693562865,4.59001491468124,36.1796488213164));
#39464=CARTESIAN_POINT('Ctrl Pts',(19.822090343592,4.58961979627771,36.1790816561008));
#39465=CARTESIAN_POINT('Ctrl Pts',(19.8364603098112,4.58867506534529,36.1777961742714));
#39466=CARTESIAN_POINT('Ctrl Pts',(19.8448114414141,4.58812464675447,36.1771039327467));
#39467=CARTESIAN_POINT('Ctrl Pts',(19.8748290181767,4.58614106413554,36.1748125358137));
#39468=CARTESIAN_POINT('Ctrl Pts',(19.8965169300648,4.58469827538078,36.1735250492253));
#39469=CARTESIAN_POINT('Ctrl Pts',(20.0711483949763,4.57299900619799,36.1661154940672));
#39470=CARTESIAN_POINT('Ctrl Pts',(20.2242756992017,4.56216998168005,36.1778517810998));
#39471=CARTESIAN_POINT('Ctrl Pts',(20.4541170603095,4.54545143079664,36.2233198843081));
#39472=CARTESIAN_POINT('Ctrl Pts',(20.5327895805914,4.53965580306748,36.2441208314317));
#39473=CARTESIAN_POINT('Ctrl Pts',(20.6437100857044,4.53155527609672,36.2810858953062));
#39474=CARTESIAN_POINT('Ctrl Pts',(20.6771853761131,4.52912085015314,36.2932815499375));
#39475=CARTESIAN_POINT('Ctrl Pts',(20.7171920528624,4.52623949880148,36.3091250832975));
#39476=CARTESIAN_POINT('Ctrl Pts',(20.7240622727002,4.52574571201067,36.3118917153617));
#39477=CARTESIAN_POINT('Ctrl Pts',(20.7347455796272,4.52497964515902,36.3162655440651));
#39478=CARTESIAN_POINT('Ctrl Pts',(20.738569626017,4.52470579187046,36.3178455217364));
#39479=CARTESIAN_POINT('Ctrl Pts',(20.7456745932028,4.52419768553872,36.3208078707606));
#39480=CARTESIAN_POINT('Ctrl Pts',(20.748956739662,4.52396325095684,36.3221870081106));
#39481=CARTESIAN_POINT('Ctrl Pts',(20.7564166140534,4.523431045377,36.3253459258456));
#39482=CARTESIAN_POINT('Ctrl Pts',(20.7605918812098,4.52313361977978,36.3271313731109));
#39483=CARTESIAN_POINT('Ctrl Pts',(20.7733394338673,4.5222268032921,36.3326358635828));
#39484=CARTESIAN_POINT('Ctrl Pts',(20.7818911922611,4.52162020392953,36.3364025281686));
#39485=CARTESIAN_POINT('Ctrl Pts',(20.8772129033101,4.51487464809053,36.379217104958));
#39486=CARTESIAN_POINT('Ctrl Pts',(20.9610203061125,4.50908852955465,36.4245772284742));
#39487=CARTESIAN_POINT('Ctrl Pts',(21.1876794987629,4.49292381154619,36.5698835996926));
#39488=CARTESIAN_POINT('Ctrl Pts',(21.3208086480482,4.4827138251842,36.6832084689386));
#39489=CARTESIAN_POINT('Ctrl Pts',(21.4506174311852,4.4703644713334,36.8281225635701));
#39490=CARTESIAN_POINT('Ctrl Pts',(21.4640560335353,4.46905321659646,36.8436150970497));
#39491=CARTESIAN_POINT('Ctrl Pts',(21.4829291148577,4.46716235299635,36.866086745611));
#39492=CARTESIAN_POINT('Ctrl Pts',(21.4885668701474,4.46659099124767,36.8728939133538));
#39493=CARTESIAN_POINT('Ctrl Pts',(21.4982591741286,4.46559718583685,36.884761731152));
#39494=CARTESIAN_POINT('Ctrl Pts',(21.5023353868492,4.46517561871386,36.8898045667551));
#39495=CARTESIAN_POINT('Ctrl Pts',(21.5101257319498,4.46436289364722,36.8995423094714));
#39496=CARTESIAN_POINT('Ctrl Pts',(21.513843592365,4.46397189053471,36.904234149364));
#39497=CARTESIAN_POINT('Ctrl Pts',(21.5225661776168,4.46304705141315,36.9153476978905));
#39498=CARTESIAN_POINT('Ctrl Pts',(21.5275521750585,4.4625124862287,36.9217838945412));
#39499=CARTESIAN_POINT('Ctrl Pts',(21.5448231133803,4.46063986048519,36.9443720712433));
#39500=CARTESIAN_POINT('Ctrl Pts',(21.5568934593972,4.45929351914829,36.9606857043561));
#39501=CARTESIAN_POINT('Ctrl Pts',(21.6673829967903,4.446605864438,37.1150526713218));
#39502=CARTESIAN_POINT('Ctrl Pts',(21.7474382586424,4.43454217570489,37.2653008480401));
#39503=CARTESIAN_POINT('Ctrl Pts',(21.8314283322691,4.417455576334,37.4897997992774));
#39504=CARTESIAN_POINT('Ctrl Pts',(21.8524272067254,4.41247314441218,37.5568712449273));
#39505=CARTESIAN_POINT('Ctrl Pts',(21.8777682402318,4.40536145964218,37.6566080470622));
#39506=CARTESIAN_POINT('Ctrl Pts',(21.8850086484524,4.4031328345844,37.6884751580249));
#39507=CARTESIAN_POINT('Ctrl Pts',(21.8928566472806,4.40046240012044,37.7275911044223));
#39508=CARTESIAN_POINT('Ctrl Pts',(21.8942370361446,4.3999812255997,37.7346772281675));
#39509=CARTESIAN_POINT('Ctrl Pts',(21.896338357497,4.39923042633378,37.7457964244269));
#39510=CARTESIAN_POINT('Ctrl Pts',(21.8970862593421,4.3989593263756,37.7498242377682));
#39511=CARTESIAN_POINT('Ctrl Pts',(21.8984611350802,4.39845362546502,37.7573623052131));
#39512=CARTESIAN_POINT('Ctrl Pts',(21.8990912005849,4.39821885947163,37.7608718775434));
#39513=CARTESIAN_POINT('Ctrl Pts',(21.9005120707179,4.39768239405247,37.7689145140589));
#39514=CARTESIAN_POINT('Ctrl Pts',(21.9012963892106,4.39738106212558,37.7734486695756));
#39515=CARTESIAN_POINT('Ctrl Pts',(21.903310698097,4.39659314028827,37.7853467273748));
#39516=CARTESIAN_POINT('Ctrl Pts',(21.9045141915785,4.39610799566289,37.7927151257903));
#39517=CARTESIAN_POINT('Ctrl Pts',(21.9124680268063,4.39279847236769,37.8432551140782));
#39518=CARTESIAN_POINT('Ctrl Pts',(21.9177932487008,4.39004763771808,37.8866420248929));
#39519=CARTESIAN_POINT('Ctrl Pts',(21.9228476258785,4.38649579342051,37.9438347610123));
#39520=CARTESIAN_POINT('Ctrl Pts',(21.923909070375,4.38565231098272,37.9575062183754));
#39521=CARTESIAN_POINT('Ctrl Pts',(21.9335429046849,4.37681852324583,38.1014637308141));
#39522=CARTESIAN_POINT('Ctrl Pts',(21.9290133508093,4.36918038076055,38.23229255749));
#39523=CARTESIAN_POINT('Ctrl Pts',(21.9029529552375,4.35756703534153,38.4226467440222));
#39524=CARTESIAN_POINT('Ctrl Pts',(21.8916914845443,4.3538010728418,38.4831882853689));
#39525=CARTESIAN_POINT('Ctrl Pts',(21.8691069165198,4.34765100144082,38.5788896328528));
#39526=CARTESIAN_POINT('Ctrl Pts',(21.859635324769,4.34532202008999,38.6144435088058));
#39527=CARTESIAN_POINT('Ctrl Pts',(21.8460065451228,4.34225140838157,38.6602895395444));
#39528=CARTESIAN_POINT('Ctrl Pts',(21.8427686969458,4.34153950605068,38.6708485386371));
#39529=CARTESIAN_POINT('Ctrl Pts',(21.8373494684938,4.340375580395,38.6879945797138));
#39530=CARTESIAN_POINT('Ctrl Pts',(21.8352228701748,4.33992534350943,38.694598780567));
#39531=CARTESIAN_POINT('Ctrl Pts',(21.8310592407894,4.3390560883792,38.7072938836381));
#39532=CARTESIAN_POINT('Ctrl Pts',(21.8290273250354,4.33863724229716,38.713386376593));
#39533=CARTESIAN_POINT('Ctrl Pts',(21.8242957285344,4.33767396763443,38.7273410179269));
#39534=CARTESIAN_POINT('Ctrl Pts',(21.8215755920188,4.3371288737969,38.7351960459889));
#39535=CARTESIAN_POINT('Ctrl Pts',(21.8141875661497,4.33567096171994,38.756092911195));
#39536=CARTESIAN_POINT('Ctrl Pts',(21.8094299016325,4.33475520357829,38.7691022697902));
#39537=CARTESIAN_POINT('Ctrl Pts',(21.7642749665455,4.32626881146562,38.8885692907445));
#39538=CARTESIAN_POINT('Ctrl Pts',(21.7146740153783,4.31838631654346,38.9912869176095));
#39539=CARTESIAN_POINT('Ctrl Pts',(21.6177503413988,4.30499866869008,39.1536059286512));
#39540=CARTESIAN_POINT('Ctrl Pts',(21.5754389511386,4.29961028037633,39.2158822993459));
#39541=CARTESIAN_POINT('Ctrl Pts',(21.4757661322168,4.28797381560509,39.3455769904254));
#39542=CARTESIAN_POINT('Ctrl Pts',(21.4171758110747,4.28175231499799,39.4118553150817));
#39543=CARTESIAN_POINT('Ctrl Pts',(21.3478531271193,4.27521459194621,39.4801865658333));
#39544=CARTESIAN_POINT('Ctrl Pts',(21.3414212306577,4.27461522385891,39.4864386385234));
#39545=CARTESIAN_POINT('Ctrl Pts',(21.3317216674679,4.27372240785382,39.4957363303852));
#39546=CARTESIAN_POINT('Ctrl Pts',(21.3284867614135,4.2734264618551,39.4988157238562));
#39547=CARTESIAN_POINT('Ctrl Pts',(21.3226579274001,4.27289651133477,39.5043258882336));
#39548=CARTESIAN_POINT('Ctrl Pts',(21.3200679614774,4.27266219866563,39.5067607369466));
#39549=CARTESIAN_POINT('Ctrl Pts',(21.3144080112681,4.2721526803333,39.5120523083578));
#39550=CARTESIAN_POINT('Ctrl Pts',(21.3113354454917,4.27187769004966,39.5149061777545));
#39551=CARTESIAN_POINT('Ctrl Pts',(21.3027750743043,4.27111591751082,39.5228054094895));
#39552=CARTESIAN_POINT('Ctrl Pts',(21.2972672210801,4.27063073813734,39.5278290825652));
#39553=CARTESIAN_POINT('Ctrl Pts',(21.2678904883271,4.26806824552355,39.5543130749083));
#39554=CARTESIAN_POINT('Ctrl Pts',(21.2435163190861,4.26602991525139,39.5752085495293));
#39555=CARTESIAN_POINT('Ctrl Pts',(21.2044588721818,4.26287767657497,39.6070353572671));
#39556=CARTESIAN_POINT('Ctrl Pts',(21.1901235277678,4.2617437771043,39.6183816290915));
#39557=CARTESIAN_POINT('Ctrl Pts',(21.1670523668197,4.25995138218209,39.6361146885293));
#39558=CARTESIAN_POINT('Ctrl Pts',(21.1584206669402,4.25928785530989,39.6426344766061));
#39559=CARTESIAN_POINT('Ctrl Pts',(21.0527369742636,4.25124336914657,39.721073338999));
#39560=CARTESIAN_POINT('Ctrl Pts',(20.9491887758372,4.24415496626519,39.7837984905317));
#39561=CARTESIAN_POINT('Ctrl Pts',(20.7806899345176,4.23287103583038,39.8653536938381));
#39562=CARTESIAN_POINT('Ctrl Pts',(20.7194811566678,4.22882190487687,39.8911717373543));
#39563=CARTESIAN_POINT('Ctrl Pts',(20.6206182379638,4.22225575545189,39.9269861548686));
#39564=CARTESIAN_POINT('Ctrl Pts',(20.5837820304635,4.21980417738075,39.9390877145324));
#39565=CARTESIAN_POINT('Ctrl Pts',(20.5358204633695,4.21659443345015,39.9532580827717));
#39566=CARTESIAN_POINT('Ctrl Pts',(20.5250052674994,4.2158695191197,39.9563508695044));
#39567=CARTESIAN_POINT('Ctrl Pts',(20.5074331657714,4.21468962242291,39.961210064743));
#39568=CARTESIAN_POINT('Ctrl Pts',(20.5006925242289,4.21423652111762,39.9630347063014));
#39569=CARTESIAN_POINT('Ctrl Pts',(20.4877476869706,4.21336536606425,39.9664634512382));
#39570=CARTESIAN_POINT('Ctrl Pts',(20.4815451035329,4.21294750406135,39.9680733209807));
#39571=CARTESIAN_POINT('Ctrl Pts',(20.4673716744068,4.21199158792222,39.9716767303187));
#39572=CARTESIAN_POINT('Ctrl Pts',(20.4593959259106,4.21145290244669,39.9736502994404));
#39573=CARTESIAN_POINT('Ctrl Pts',(20.4382601031204,4.2100232353587,39.9787372134501));
#39574=CARTESIAN_POINT('Ctrl Pts',(20.42507967225,4.20912949103839,39.981763186927));
#39575=CARTESIAN_POINT('Ctrl Pts',(20.3214640492965,4.20208506045868,40.0044071980833));
#39576=CARTESIAN_POINT('Ctrl Pts',(20.229768955051,4.19573243692902,40.0176307021517));
#39577=CARTESIAN_POINT('Ctrl Pts',(19.9779362599118,4.17799848806848,40.0356248046861));
#39578=CARTESIAN_POINT('Ctrl Pts',(19.8175932114207,4.16635202614621,40.0271366259504));
#39579=CARTESIAN_POINT('Ctrl Pts',(19.6315140946171,4.15333098510131,39.9938337962496));
#39580=CARTESIAN_POINT('Ctrl Pts',(19.6030046674812,4.15135218311773,39.9880633574922));
#39581=CARTESIAN_POINT('Ctrl Pts',(19.5678434950929,4.14894058054307,39.9801148345455));
#39582=CARTESIAN_POINT('Ctrl Pts',(19.5610604139643,4.14847669313282,39.9785428074112));
#39583=CARTESIAN_POINT('Ctrl Pts',(19.5503551106908,4.14774685554124,39.9760006270133));
#39584=CARTESIAN_POINT('Ctrl Pts',(19.5464272522642,4.14747956020597,39.9750548371428));
#39585=CARTESIAN_POINT('Ctrl Pts',(19.5390282997567,4.14697701039571,39.9732486318485));
#39586=CARTESIAN_POINT('Ctrl Pts',(19.5355566683336,4.14674161409593,39.9723909145936));
#39587=CARTESIAN_POINT('Ctrl Pts',(19.5276093306862,4.1462036373515,39.9704039453093));
#39588=CARTESIAN_POINT('Ctrl Pts',(19.5231352799169,4.14590142676041,39.9692682800802));
#39589=CARTESIAN_POINT('Ctrl Pts',(19.511227158127,4.14509869132121,39.9662000602069));
#39590=CARTESIAN_POINT('Ctrl Pts',(19.5038003875913,4.14459974024977,39.9642391222873));
#39591=CARTESIAN_POINT('Ctrl Pts',(19.4497188737165,4.14097742868771,39.9496135470395));
#39592=CARTESIAN_POINT('Ctrl Pts',(19.403538669408,4.13794424025762,39.9352423184952));
#39593=CARTESIAN_POINT('Ctrl Pts',(19.2286555086251,4.12651739352343,39.873518457891));
#39594=CARTESIAN_POINT('Ctrl Pts',(19.1045937590485,4.11851291204389,39.8142324447551));
#39595=CARTESIAN_POINT('Ctrl Pts',(18.9342427767939,4.10642791696285,39.7092454047518));
#39596=CARTESIAN_POINT('Ctrl Pts',(18.8822802126492,4.10257805189969,39.6735980176834));
#39597=CARTESIAN_POINT('Ctrl Pts',(18.8024027811172,4.09630430654009,39.6128452939391));
#39598=CARTESIAN_POINT('Ctrl Pts',(18.7733145362388,4.09393850633659,39.5893563914937));
#39599=CARTESIAN_POINT('Ctrl Pts',(18.7364936118458,4.09082606188915,39.5578125819219));
#39600=CARTESIAN_POINT('Ctrl Pts',(18.7281215207411,4.09011018212417,39.5505140614705));
#39601=CARTESIAN_POINT('Ctrl Pts',(18.7146124517329,4.08894137578081,39.5385304088354));
#39602=CARTESIAN_POINT('Ctrl Pts',(18.709436875754,4.0884902643654,39.5338890147518));
#39603=CARTESIAN_POINT('Ctrl Pts',(18.6995318221263,4.08762044365133,39.5249092125008));
#39604=CARTESIAN_POINT('Ctrl Pts',(18.6947986773494,4.08720191255303,39.5205749720512));
#39605=CARTESIAN_POINT('Ctrl Pts',(18.6840069619233,4.08624095344394,39.5105933076828));
#39606=CARTESIAN_POINT('Ctrl Pts',(18.6779629909669,4.08569787083798,39.5049303538213));
#39607=CARTESIAN_POINT('Ctrl Pts',(18.6619837517628,4.08424884318147,39.489764043791));
#39608=CARTESIAN_POINT('Ctrl Pts',(18.6521134399902,4.08334001453743,39.4801932410899));
#39609=CARTESIAN_POINT('Ctrl Pts',(18.5482248853404,4.07362454576865,39.377279842162));
#39610=CARTESIAN_POINT('Ctrl Pts',(18.463976987028,4.06438730890076,39.2746128333193));
#39611=CARTESIAN_POINT('Ctrl Pts',(18.3330469446396,4.04749993939522,39.0766360533751));
#39612=CARTESIAN_POINT('Ctrl Pts',(18.2824058367384,4.03995694287053,38.9845463062223));
#39613=CARTESIAN_POINT('Ctrl Pts',(18.2222187684088,4.02970522874001,38.8502155841056));
#39614=CARTESIAN_POINT('Ctrl Pts',(18.2062052112214,4.0268035576142,38.8110769433286));
#39615=CARTESIAN_POINT('Ctrl Pts',(18.1887866336923,4.02344994537789,38.7641603745008));
#39616=CARTESIAN_POINT('Ctrl Pts',(18.1861277177054,4.02293190793254,38.7568639203817));
#39617=CARTESIAN_POINT('Ctrl Pts',(18.18209354727,4.02213655403118,38.7455822604908));
#39618=CARTESIAN_POINT('Ctrl Pts',(18.1806872117192,4.02185746843808,38.7416083736819));
#39619=CARTESIAN_POINT('Ctrl Pts',(18.1781194327421,4.02134455089018,38.7342762659293));
#39620=CARTESIAN_POINT('Ctrl Pts',(18.1769542493074,4.02111050661599,38.7309194672511));
#39621=CARTESIAN_POINT('Ctrl Pts',(18.1743542712047,4.0205853091986,38.7233618008505));
#39622=CARTESIAN_POINT('Ctrl Pts',(18.1729247008032,4.02029446404498,38.7191591991306));
#39623=CARTESIAN_POINT('Ctrl Pts',(18.1693003873996,4.0195516512404,38.7083827061063));
#39624=CARTESIAN_POINT('Ctrl Pts',(18.1671265174731,4.01910087231834,38.7018017856725));
#39625=CARTESIAN_POINT('Ctrl Pts',(18.1544639546345,4.01644280918484,38.6627634873682));
#39626=CARTESIAN_POINT('Ctrl Pts',(18.1448013836846,4.0142800591071,38.6300419561242));
#39627=CARTESIAN_POINT('Ctrl Pts',(18.1318640824568,4.01114533297078,38.5815285709754));
#39628=CARTESIAN_POINT('Ctrl Pts',(18.127911811724,4.01014796905676,38.5659264033361));
#39629=CARTESIAN_POINT('Ctrl Pts',(18.12166518197,4.00849958209285,38.5399030247195));
#39630=CARTESIAN_POINT('Ctrl Pts',(18.1192612623421,4.0078452027334,38.5295092163879));
#39631=CARTESIAN_POINT('Ctrl Pts',(18.0864220122501,3.99860538724657,38.3819578687861));
#39632=CARTESIAN_POINT('Ctrl Pts',(18.0709715023171,3.990411626189,38.2418930328489));
#39633=CARTESIAN_POINT('Ctrl Pts',(18.0708133507936,3.97704079803533,38.0218888399083));
#39634=CARTESIAN_POINT('Ctrl Pts',(18.0756701924695,3.97211873391506,37.9424724237382));
#39635=CARTESIAN_POINT('Ctrl Pts',(18.0870228991789,3.96619961696205,37.8505321041372));
#39636=CARTESIAN_POINT('Ctrl Pts',(18.0887685376542,3.96535505979258,37.8374930421612));
#39637=CARTESIAN_POINT('Ctrl Pts',(18.0918178427118,3.96397762631338,37.8163618973671));
#39638=CARTESIAN_POINT('Ctrl Pts',(18.0930399808263,3.96344730292806,37.8082583325577));
#39639=CARTESIAN_POINT('Ctrl Pts',(18.095306441344,3.96250076037313,37.7938533013139));
#39640=CARTESIAN_POINT('Ctrl Pts',(18.0963305019229,3.96208518347924,37.7875487334658));
#39641=CARTESIAN_POINT('Ctrl Pts',(18.0985529863079,3.96120792316165,37.7742827799156));
#39642=CARTESIAN_POINT('Ctrl Pts',(18.0997583715633,3.96074602610255,37.7673226718487));
#39643=CARTESIAN_POINT('Ctrl Pts',(18.1030464125094,3.95952155342855,37.7489380395507));
#39644=CARTESIAN_POINT('Ctrl Pts',(18.1051940225579,3.95875694007456,37.7375255718641));
#39645=CARTESIAN_POINT('Ctrl Pts',(18.1156931406398,3.9551745548734,37.684377835485));
#39646=CARTESIAN_POINT('Ctrl Pts',(18.1253207915251,3.95231676982322,37.6429097398547));
#39647=CARTESIAN_POINT('Ctrl Pts',(18.17940113469,3.93805261648679,37.4406049801355));
#39648=CARTESIAN_POINT('Ctrl Pts',(18.243217800543,3.92603020671464,37.2857025341727));
#39649=CARTESIAN_POINT('Ctrl Pts',(18.3408459147008,3.91211244182069,37.1153042894467));
#39650=CARTESIAN_POINT('Ctrl Pts',(18.3561433708184,3.9100263589118,37.0899735523866));
#39651=CARTESIAN_POINT('Ctrl Pts',(18.3878201486455,3.90590107481111,37.0401480252906));
#39652=CARTESIAN_POINT('Ctrl Pts',(18.4041904291212,3.90386220833471,37.0156559200628));
#39653=CARTESIAN_POINT('Ctrl Pts',(18.4327579898231,3.90046761559812,36.9749641939155));
#39654=CARTESIAN_POINT('Ctrl Pts',(18.4446610693517,3.89909752675677,36.9585649493338));
#39655=CARTESIAN_POINT('Ctrl Pts',(18.4606563544544,3.89731662600097,36.9372426953686));
#39656=CARTESIAN_POINT('Ctrl Pts',(18.4645172768703,3.89689121337132,36.932148888612));
#39657=CARTESIAN_POINT('Ctrl Pts',(18.4707826805114,3.89620813275404,36.9239675775284));
#39658=CARTESIAN_POINT('Ctrl Pts',(18.4731713234128,3.8959493914636,36.9208680896699));
#39659=CARTESIAN_POINT('Ctrl Pts',(18.4777842585066,3.89545296259651,36.9149198949708));
#39660=CARTESIAN_POINT('Ctrl Pts',(18.4800071305063,3.89521518462695,36.912070163743));
#39661=CARTESIAN_POINT('Ctrl Pts',(18.4852977000073,3.89465262446539,36.9053267936235));
#39662=CARTESIAN_POINT('Ctrl Pts',(18.4883724463787,3.89432833679257,36.9014386673542));
#39663=CARTESIAN_POINT('Ctrl Pts',(18.4986882039736,3.89324902140899,36.8884968646558));
#39664=CARTESIAN_POINT('Ctrl Pts',(18.5059960069998,3.8924985530324,36.8794963987493));
#39665=CARTESIAN_POINT('Ctrl Pts',(18.5237112512491,3.89071130191849,36.8580754285004));
#39666=CARTESIAN_POINT('Ctrl Pts',(18.5341950690072,3.88967939715213,36.8457189098154));
#39667=CARTESIAN_POINT('Ctrl Pts',(18.5740379519883,3.88584646319466,36.7999409272007));
#39668=CARTESIAN_POINT('Ctrl Pts',(18.6043961770208,3.88310177944765,36.7674040820889));
#39669=CARTESIAN_POINT('Ctrl Pts',(18.7572310768449,3.869938882807,36.6145591389673));
#39670=CARTESIAN_POINT('Ctrl Pts',(18.8942622520232,3.85999975198645,36.5099193007882));
#39671=CARTESIAN_POINT('Ctrl Pts',(19.0835316410962,3.84647620676696,36.4018330473647));
#39672=CARTESIAN_POINT('Ctrl Pts',(19.1245385067943,3.84356252770913,36.3803337860971));
#39673=CARTESIAN_POINT('Ctrl Pts',(19.177390605636,3.83980747959394,36.355004803175));
#39674=CARTESIAN_POINT('Ctrl Pts',(19.188555370052,3.83901429386234,36.3497851406876));
#39675=CARTESIAN_POINT('Ctrl Pts',(19.2064040899856,3.83774598759691,36.3416481410624));
#39676=CARTESIAN_POINT('Ctrl Pts',(19.2130560237657,3.83727325202138,36.3386610479307));
#39677=CARTESIAN_POINT('Ctrl Pts',(19.2255340378444,3.83638628934142,36.3331425127215));
#39678=CARTESIAN_POINT('Ctrl Pts',(19.2313560130903,3.83597237758754,36.3306019874924));
#39679=CARTESIAN_POINT('Ctrl Pts',(19.2443854937682,3.83504583251551,36.3249927776994));
#39680=CARTESIAN_POINT('Ctrl Pts',(19.251599324856,3.83453269855067,36.3219391608706));
#39681=CARTESIAN_POINT('Ctrl Pts',(19.2728556870746,3.83302014159584,36.3130936111078));
#39682=CARTESIAN_POINT('Ctrl Pts',(19.2869479973391,3.83201665617838,36.3074236100906));
#39683=CARTESIAN_POINT('Ctrl Pts',(19.3318333028841,3.82881750908881,36.2899771627739));
#39684=CARTESIAN_POINT('Ctrl Pts',(19.3628434160786,3.82660281497636,36.2788305312031));
#39685=CARTESIAN_POINT('Ctrl Pts',(19.3941042587802,3.8243647438501,36.2684889004782));
#39686=CARTESIAN_POINT('',(18.0708708501867,3.80900185377495,38.0984559108978));
#39687=CARTESIAN_POINT('Ctrl Pts',(19.3941040086362,3.65343403802913,36.2684889832302));
#39688=CARTESIAN_POINT('Ctrl Pts',(19.3851461582278,3.6540316240628,36.2714523973751));
#39689=CARTESIAN_POINT('Ctrl Pts',(19.376209716234,3.65462626174559,36.274481640278));
#39690=CARTESIAN_POINT('Ctrl Pts',(19.2143176168196,3.665377095241,36.3306869478762));
#39691=CARTESIAN_POINT('Ctrl Pts',(19.0686201053574,3.67474886595825,36.4028525906517));
#39692=CARTESIAN_POINT('Ctrl Pts',(18.8591032064564,3.68995776020145,36.5418287318295));
#39693=CARTESIAN_POINT('Ctrl Pts',(18.7881024655457,3.69546934998093,36.5963895351481));
#39694=CARTESIAN_POINT('Ctrl Pts',(18.7110812495807,3.7020398960586,36.6645865436071));
#39695=CARTESIAN_POINT('Ctrl Pts',(18.7011084297453,3.70290282511424,36.6736045393984));
#39696=CARTESIAN_POINT('Ctrl Pts',(18.6852114632913,3.70429859839293,36.6882844507502));
#39697=CARTESIAN_POINT('Ctrl Pts',(18.6792275888118,3.70482870432481,36.6938812558347));
#39698=CARTESIAN_POINT('Ctrl Pts',(18.6686299225227,3.70577609535566,36.7039207416122));
#39699=CARTESIAN_POINT('Ctrl Pts',(18.6640022332416,3.70619274445471,36.7083486268206));
#39700=CARTESIAN_POINT('Ctrl Pts',(18.6551197200089,3.70699823954631,36.716932768572));
#39701=CARTESIAN_POINT('Ctrl Pts',(18.650861893487,3.7073869444375,36.7210858248666));
#39702=CARTESIAN_POINT('Ctrl Pts',(18.6397221004987,3.70841080590348,36.7320524938786));
#39703=CARTESIAN_POINT('Ctrl Pts',(18.632872186243,3.7090473648826,36.738898285045));
#39704=CARTESIAN_POINT('Ctrl Pts',(18.6066950002682,3.71150734331433,36.7654566848019));
#39705=CARTESIAN_POINT('Ctrl Pts',(18.5877409668395,3.71334674823657,36.7855309162192));
#39706=CARTESIAN_POINT('Ctrl Pts',(18.5412428655149,3.71801112839031,36.8369440007918));
#39707=CARTESIAN_POINT('Ctrl Pts',(18.5142735756319,3.72085817615058,36.8687813375002));
#39708=CARTESIAN_POINT('Ctrl Pts',(18.443101699652,3.7287742189638,36.9585462645469));
#39709=CARTESIAN_POINT('Ctrl Pts',(18.4011174950201,3.73391154060393,37.0181395350112));
#39710=CARTESIAN_POINT('Ctrl Pts',(18.2898554733521,3.74888281311257,37.196739959117));
#39711=CARTESIAN_POINT('Ctrl Pts',(18.2298021928285,3.75881332750799,37.3209760806627));
#39712=CARTESIAN_POINT('Ctrl Pts',(18.1787739075928,3.76907883473651,37.4637035632299));
#39713=CARTESIAN_POINT('Ctrl Pts',(18.174214655466,3.77001787057233,37.4769064769561));
#39714=CARTESIAN_POINT('Ctrl Pts',(18.1680585730791,3.77131608307844,37.4953815436534));
#39715=CARTESIAN_POINT('Ctrl Pts',(18.1663404446504,3.77168189194893,37.5006123905705));
#39716=CARTESIAN_POINT('Ctrl Pts',(18.163613323029,3.7722681245345,37.509036596841));
#39717=CARTESIAN_POINT('Ctrl Pts',(18.1625902257339,3.77248935809529,37.5122253041435));
#39718=CARTESIAN_POINT('Ctrl Pts',(18.160462785769,3.77295212726625,37.5189157755266));
#39719=CARTESIAN_POINT('Ctrl Pts',(18.1593601307929,3.77319355900465,37.5224180485165));
#39720=CARTESIAN_POINT('Ctrl Pts',(18.1566982254109,3.77378032214086,37.5309578815979));
#39721=CARTESIAN_POINT('Ctrl Pts',(18.1551496031556,3.77412503928215,37.5359987769598));
#39722=CARTESIAN_POINT('Ctrl Pts',(18.1497028783146,3.77534978853889,37.553990803865));
#39723=CARTESIAN_POINT('Ctrl Pts',(18.1459202150976,3.77622341707248,37.5669768702197));
#39724=CARTESIAN_POINT('Ctrl Pts',(18.1233332138771,3.78159423302404,37.6476703710395));
#39725=CARTESIAN_POINT('Ctrl Pts',(18.108101300561,3.78591400750198,37.716331040995));
#39726=CARTESIAN_POINT('Ctrl Pts',(18.0795757838454,3.79650422848749,37.8890643503315));
#39727=CARTESIAN_POINT('Ctrl Pts',(18.0709545923284,3.80268017310218,37.9936686640546));
#39728=CARTESIAN_POINT('Ctrl Pts',(18.0708706194525,3.80900133785267,38.0984540347479));
#39729=CARTESIAN_POINT('Ctrl Pts',(18.0708706179307,3.80900145248059,38.0984559349242));
#39730=CARTESIAN_POINT('Ctrl Pts',(18.0707947923802,3.81471634261588,38.1931911243054));
#39731=CARTESIAN_POINT('Ctrl Pts',(18.0776971394593,3.82053333068208,38.2877941798662));
#39732=CARTESIAN_POINT('Ctrl Pts',(18.093157633927,3.82729189732055,38.3926103313709));
#39733=CARTESIAN_POINT('Ctrl Pts',(18.0948928930901,3.8280110044117,38.4037030091995));
#39734=CARTESIAN_POINT('Ctrl Pts',(18.0979441529452,3.82921372139165,38.4221520597585));
#39735=CARTESIAN_POINT('Ctrl Pts',(18.0992062626677,3.82969565035746,38.4295171626478));
#39736=CARTESIAN_POINT('Ctrl Pts',(18.1015682108665,3.83057042720451,38.4428351554627));
#39737=CARTESIAN_POINT('Ctrl Pts',(18.1026533446979,3.8309628094676,38.4487905819368));
#39738=CARTESIAN_POINT('Ctrl Pts',(18.1049217777222,3.83176423758432,38.4609162787321));
#39739=CARTESIAN_POINT('Ctrl Pts',(18.1061072243265,3.832173346761,38.4670860682454));
#39740=CARTESIAN_POINT('Ctrl Pts',(18.1087603598732,3.83306837939916,38.4805395996859));
#39741=CARTESIAN_POINT('Ctrl Pts',(18.1102400285953,3.83355467649597,38.4878208493566));
#39742=CARTESIAN_POINT('Ctrl Pts',(18.1144090411457,3.83489067886773,38.5077454834846));
#39743=CARTESIAN_POINT('Ctrl Pts',(18.1171834174452,3.83574306760818,38.520370486736));
#39744=CARTESIAN_POINT('Ctrl Pts',(18.1320954752845,3.84014542221406,38.5851177975624));
#39745=CARTESIAN_POINT('Ctrl Pts',(18.146270338236,3.843759680657,38.6367420093424));
#39746=CARTESIAN_POINT('Ctrl Pts',(18.1686210206925,3.84880017406108,38.7066200778223));
#39747=CARTESIAN_POINT('Ctrl Pts',(18.1749621381135,3.85017258128813,38.7254387618747));
#39748=CARTESIAN_POINT('Ctrl Pts',(18.1963508949265,3.85462350888188,38.7858177604959));
#39749=CARTESIAN_POINT('Ctrl Pts',(18.2125360145041,3.8577301327015,38.8269582009965));
#39750=CARTESIAN_POINT('Ctrl Pts',(18.2820911310179,3.87010975576839,38.9873537031444));
#39751=CARTESIAN_POINT('Ctrl Pts',(18.3461018488333,3.87955491100009,39.1016133572993));
#39752=CARTESIAN_POINT('Ctrl Pts',(18.4417131540731,3.8910842723752,39.237788599667));
#39753=CARTESIAN_POINT('Ctrl Pts',(18.4630685339686,3.89352810661431,39.2664745437915));
#39754=CARTESIAN_POINT('Ctrl Pts',(18.4898015691682,3.89641905347886,39.3003742029435));
#39755=CARTESIAN_POINT('Ctrl Pts',(18.4944262063977,3.89691338464032,39.3061695917191));
#39756=CARTESIAN_POINT('Ctrl Pts',(18.5016846572643,3.89768010947562,39.3151587650595));
#39757=CARTESIAN_POINT('Ctrl Pts',(18.5042954709908,3.8979540806697,39.3183709013594));
#39758=CARTESIAN_POINT('Ctrl Pts',(18.5091708857992,3.89846229136008,39.3243299320042));
#39759=CARTESIAN_POINT('Ctrl Pts',(18.511432730272,3.89869671310012,39.3270789355076));
#39760=CARTESIAN_POINT('Ctrl Pts',(18.5165954776466,3.89922874309039,39.3333183600506));
#39761=CARTESIAN_POINT('Ctrl Pts',(18.5195010916272,3.89952600685379,39.3368048097913));
#39762=CARTESIAN_POINT('Ctrl Pts',(18.5284184699448,3.90043184171811,39.3474283285124));
#39763=CARTESIAN_POINT('Ctrl Pts',(18.5344698474112,3.90103763008039,39.3545321895879));
#39764=CARTESIAN_POINT('Ctrl Pts',(18.6041366317163,3.90791462501313,39.435123700652));
#39765=CARTESIAN_POINT('Ctrl Pts',(18.6731767948973,3.91381742707861,39.5037576541927));
#39766=CARTESIAN_POINT('Ctrl Pts',(18.8137574594692,3.92491061097863,39.6238287961646));
#39767=CARTESIAN_POINT('Ctrl Pts',(18.8842096715816,3.93010199453674,39.6761463789056));
#39768=CARTESIAN_POINT('Ctrl Pts',(19.0105557631346,3.93917167817195,39.7572405920793));
#39769=CARTESIAN_POINT('Ctrl Pts',(19.064741284564,3.94299216359648,39.7884124033291));
#39770=CARTESIAN_POINT('Ctrl Pts',(19.1422607324923,3.94843825056907,39.8281297797831));
#39771=CARTESIAN_POINT('Ctrl Pts',(19.1643932457876,3.94999080473494,39.8389394631922));
#39772=CARTESIAN_POINT('Ctrl Pts',(19.203375459722,3.9527253816497,39.8570626117074));
#39773=CARTESIAN_POINT('Ctrl Pts',(19.2201341844663,3.95390099984628,39.8645648053796));
#39774=CARTESIAN_POINT('Ctrl Pts',(19.2447328591887,3.95562774081858,39.8751577519031));
#39775=CARTESIAN_POINT('Ctrl Pts',(19.2524903583109,3.95617245320859,39.8784383121204));
#39776=CARTESIAN_POINT('Ctrl Pts',(19.2662200143533,3.95713691605105,39.8841387303443));
#39777=CARTESIAN_POINT('Ctrl Pts',(19.2721833177304,3.95755595060967,39.8865796796629));
#39778=CARTESIAN_POINT('Ctrl Pts',(19.2837683311647,3.95837032232637,39.8912541262576));
#39779=CARTESIAN_POINT('Ctrl Pts',(19.2893885444216,3.95876553555612,39.8934911502654));
#39780=CARTESIAN_POINT('Ctrl Pts',(19.3028244097915,3.95971072190131,39.8987659841149));
#39781=CARTESIAN_POINT('Ctrl Pts',(19.3106494769708,3.96026150286192,39.9017793210725));
#39782=CARTESIAN_POINT('Ctrl Pts',(19.3388505279036,3.96224773221152,39.9124285968339));
#39783=CARTESIAN_POINT('Ctrl Pts',(19.3593350813199,3.96369283888489,39.9197704359376));
#39784=CARTESIAN_POINT('Ctrl Pts',(19.5242615405982,3.97535100038137,39.9757516728927));
#39785=CARTESIAN_POINT('Ctrl Pts',(19.6738541567207,3.98613112942657,40.0074544589115));
#39786=CARTESIAN_POINT('Ctrl Pts',(19.9070093673327,4.00283686335771,40.0286213644422));
#39787=CARTESIAN_POINT('Ctrl Pts',(19.9888295576126,4.00866730234184,40.0308300080046));
#39788=CARTESIAN_POINT('Ctrl Pts',(20.1062599411118,4.01680959273827,40.0265327607195));
#39789=CARTESIAN_POINT('Ctrl Pts',(20.1419322031541,4.01925231262961,40.0242336924855));
#39790=CARTESIAN_POINT('Ctrl Pts',(20.1849044448613,4.02214212305744,40.0202624455215));
#39791=CARTESIAN_POINT('Ctrl Pts',(20.1922824105571,4.02263638976483,40.0195377027788));
#39792=CARTESIAN_POINT('Ctrl Pts',(20.2037730102829,4.02340303664124,40.0183420573855));
#39793=CARTESIAN_POINT('Ctrl Pts',(20.2078885184056,4.02367699382209,40.0179004284812));
#39794=CARTESIAN_POINT('Ctrl Pts',(20.2155410339602,4.02418519201142,40.0170543270868));
#39795=CARTESIAN_POINT('Ctrl Pts',(20.219078310005,4.02441961518055,40.0166533136512));
#39796=CARTESIAN_POINT('Ctrl Pts',(20.2271229430049,4.02495166568013,40.0157187490872));
#39797=CARTESIAN_POINT('Ctrl Pts',(20.231629532756,4.02524894841625,40.0151790823415));
#39798=CARTESIAN_POINT('Ctrl Pts',(20.2453970696942,4.02615489862516,40.0134811052951));
#39799=CARTESIAN_POINT('Ctrl Pts',(20.2546517202256,4.02676078232643,40.0122714692245));
#39800=CARTESIAN_POINT('Ctrl Pts',(20.3442221218273,4.03259786305619,39.9999023083397));
#39801=CARTESIAN_POINT('Ctrl Pts',(20.4237787133241,4.03757387118289,39.9837549595009));
#39802=CARTESIAN_POINT('Ctrl Pts',(20.6603214717497,4.05236056551573,39.919992832387));
#39803=CARTESIAN_POINT('Ctrl Pts',(20.8124617553576,4.0619192798298,39.857356961039));
#39804=CARTESIAN_POINT('Ctrl Pts',(20.9889775521523,4.07459972680413,39.7568066109195));
#39805=CARTESIAN_POINT('Ctrl Pts',(21.0224967928877,4.07708250928336,39.7363327028243));
#39806=CARTESIAN_POINT('Ctrl Pts',(21.0648245507893,4.08032759491892,39.7086699172734));
#39807=CARTESIAN_POINT('Ctrl Pts',(21.0742282376522,4.08105571654924,39.7024056637775));
#39808=CARTESIAN_POINT('Ctrl Pts',(21.0893629683993,4.08223955071998,39.6921305855099));
#39809=CARTESIAN_POINT('Ctrl Pts',(21.0951282713931,4.08269335858177,39.6881705025905));
#39810=CARTESIAN_POINT('Ctrl Pts',(21.1061314609013,4.08356500088651,39.6805242075244));
#39811=CARTESIAN_POINT('Ctrl Pts',(21.1113727840046,4.08398263882805,39.6768430843576));
#39812=CARTESIAN_POINT('Ctrl Pts',(21.1232772356027,4.08493683001412,39.6683934278243));
#39813=CARTESIAN_POINT('Ctrl Pts',(21.129928474271,4.08547400663796,39.6636084330832));
#39814=CARTESIAN_POINT('Ctrl Pts',(21.1474138524656,4.08689705256441,39.6508593781358));
#39815=CARTESIAN_POINT('Ctrl Pts',(21.15819540032,4.08778564381312,39.6428242799398));
#39816=CARTESIAN_POINT('Ctrl Pts',(21.2400747733902,4.09462105085333,39.5804605951504));
#39817=CARTESIAN_POINT('Ctrl Pts',(21.3073887318384,4.10075615692725,39.5213653705352));
#39818=CARTESIAN_POINT('Ctrl Pts',(21.4844053032464,4.11839680302824,39.3427151607361));
#39819=CARTESIAN_POINT('Ctrl Pts',(21.5834939711443,4.13019984127311,39.2137071533373));
#39820=CARTESIAN_POINT('Ctrl Pts',(21.6804686634817,4.14344449952014,39.0478775849321));
#39821=CARTESIAN_POINT('Ctrl Pts',(21.6950409003734,4.14549206611985,39.021565753956));
#39822=CARTESIAN_POINT('Ctrl Pts',(21.7122572772988,4.14797524146931,38.988688409879));
#39823=CARTESIAN_POINT('Ctrl Pts',(21.7154875763281,4.14844412489215,38.982436656508));
#39824=CARTESIAN_POINT('Ctrl Pts',(21.720526001411,4.14918002380946,38.9725533164912));
#39825=CARTESIAN_POINT('Ctrl Pts',(21.7223569652164,4.14944842153987,38.9689335399071));
#39826=CARTESIAN_POINT('Ctrl Pts',(21.7257790516253,4.14995186101042,38.9621148334923));
#39827=CARTESIAN_POINT('Ctrl Pts',(21.7273726869371,4.15018705136142,38.958917296267));
#39828=CARTESIAN_POINT('Ctrl Pts',(21.7309928787426,4.1507230545483,38.9516027631778));
#39829=CARTESIAN_POINT('Ctrl Pts',(21.7330136341461,4.15102350724563,38.9474829540736));
#39830=CARTESIAN_POINT('Ctrl Pts',(21.7383371160596,4.15181849474477,38.9365310585155));
#39831=CARTESIAN_POINT('Ctrl Pts',(21.741614303752,4.15231150348907,38.9296865447176));
#39832=CARTESIAN_POINT('Ctrl Pts',(21.7645455375516,4.15578831687783,38.881059317478));
#39833=CARTESIAN_POINT('Ctrl Pts',(21.782736079792,4.1586899264795,38.8385983155602));
#39834=CARTESIAN_POINT('Ctrl Pts',(21.8483775526835,4.16992840428705,38.6687770040998));
#39835=CARTESIAN_POINT('Ctrl Pts',(21.8838432672033,4.17786655621265,38.5372034155286));
#39836=CARTESIAN_POINT('Ctrl Pts',(21.9191137959813,4.19141067832588,38.315421440436));
#39837=CARTESIAN_POINT('Ctrl Pts',(21.9269846003561,4.19684608140065,38.2270104531669));
#39838=CARTESIAN_POINT('Ctrl Pts',(21.9291537598222,4.20376805584826,38.1179970318635));
#39839=CARTESIAN_POINT('Ctrl Pts',(21.9292362129113,4.2050715705259,38.0976111477534));
#39840=CARTESIAN_POINT('Ctrl Pts',(21.9288915150063,4.20695322516967,38.068411605514));
#39841=CARTESIAN_POINT('Ctrl Pts',(21.928726988708,4.20752322980213,38.0595957660128));
#39842=CARTESIAN_POINT('Ctrl Pts',(21.9283366924082,4.20851543935505,38.0443030012272));
#39843=CARTESIAN_POINT('Ctrl Pts',(21.9281387086835,4.20893677564073,38.0378254607376));
#39844=CARTESIAN_POINT('Ctrl Pts',(21.9276948829095,4.20974960126028,38.0253615982893));
#39845=CARTESIAN_POINT('Ctrl Pts',(21.9274537837915,4.21014093835591,38.0193751738267));
#39846=CARTESIAN_POINT('Ctrl Pts',(21.9268183977011,4.21106741450524,38.0052370052318));
#39847=CARTESIAN_POINT('Ctrl Pts',(21.9264002623773,4.21160328901597,37.9970864996381));
#39848=CARTESIAN_POINT('Ctrl Pts',(21.9247554625591,4.2134849361767,37.9685637064755));
#39849=CARTESIAN_POINT('Ctrl Pts',(21.9232572733435,4.21483909494981,37.9482090373677));
#39850=CARTESIAN_POINT('Ctrl Pts',(21.9064037448299,4.22746569907763,37.760064279581));
#39851=CARTESIAN_POINT('Ctrl Pts',(21.8694524115591,4.23945025086013,37.5949698099316));
#39852=CARTESIAN_POINT('Ctrl Pts',(21.7871829664574,4.25651136278032,37.3702429510733));
#39853=CARTESIAN_POINT('Ctrl Pts',(21.7591590766849,4.26154278820361,37.3050603489156));
#39854=CARTESIAN_POINT('Ctrl Pts',(21.7129866767364,4.26871480059313,37.2121380036875));
#39855=CARTESIAN_POINT('Ctrl Pts',(21.6976142696946,4.27095650673691,37.1830875789581));
#39856=CARTESIAN_POINT('Ctrl Pts',(21.677961535863,4.2736404054824,37.1481386985485));
#39857=CARTESIAN_POINT('Ctrl Pts',(21.674381497976,4.2741224216295,37.1418552007371));
#39858=CARTESIAN_POINT('Ctrl Pts',(21.6687168063217,4.27487423995726,37.1320415392366));
#39859=CARTESIAN_POINT('Ctrl Pts',(21.6666561360965,4.27514552381159,37.128497716805));
#39860=CARTESIAN_POINT('Ctrl Pts',(21.6627821554753,4.2756513815485,37.1218840704373));
#39861=CARTESIAN_POINT('Ctrl Pts',(21.6609716506212,4.27588612158526,37.1188127373699));
#39862=CARTESIAN_POINT('Ctrl Pts',(21.6568070868866,4.27642228579682,37.1117925481952));
#39863=CARTESIAN_POINT('Ctrl Pts',(21.6544474228948,4.27672334401686,37.1078470798733));
#39864=CARTESIAN_POINT('Ctrl Pts',(21.6482260141954,4.2775100801253,37.0975285085451));
#39865=CARTESIAN_POINT('Ctrl Pts',(21.644341362562,4.27799431976521,37.0911692050837));
#39866=CARTESIAN_POINT('Ctrl Pts',(21.6175784991601,4.28128425784461,37.0479228137583));
#39867=CARTESIAN_POINT('Ctrl Pts',(21.5934958457844,4.28401739571738,37.0117912588766));
#39868=CARTESIAN_POINT('Ctrl Pts',(21.5534248197869,4.28827490104779,36.955859006142));
#39869=CARTESIAN_POINT('Ctrl Pts',(21.5382305669739,4.28982961080912,36.9355112308473));
#39870=CARTESIAN_POINT('Ctrl Pts',(21.4486015717401,4.29870298450599,36.8202989404192));
#39871=CARTESIAN_POINT('Ctrl Pts',(21.3658040358976,4.30577897366711,36.7322783520488));
#39872=CARTESIAN_POINT('Ctrl Pts',(21.2133281107126,4.31806957201341,36.5979328302725));
#39873=CARTESIAN_POINT('Ctrl Pts',(21.147888554101,4.32315217372693,36.5473505450703));
#39874=CARTESIAN_POINT('Ctrl Pts',(21.0631302496849,4.32964939455875,36.4901296304019));
#39875=CARTESIAN_POINT('Ctrl Pts',(21.0466807556305,4.33090631266937,36.4793865712917));
#39876=CARTESIAN_POINT('Ctrl Pts',(21.022725075516,4.33273243435239,36.464258134442));
#39877=CARTESIAN_POINT('Ctrl Pts',(21.0153484750424,4.33329415957168,36.4596690879567));
#39878=CARTESIAN_POINT('Ctrl Pts',(21.0024342418164,4.33427667781277,36.4517555210775));
#39879=CARTESIAN_POINT('Ctrl Pts',(20.9969104008234,4.3346966501722,36.448408669644));
#39880=CARTESIAN_POINT('Ctrl Pts',(20.9862025156749,4.33551026580209,36.4419941377709));
#39881=CARTESIAN_POINT('Ctrl Pts',(20.9810206986211,4.33590377303715,36.438922870964));
#39882=CARTESIAN_POINT('Ctrl Pts',(20.9686756167973,4.3368407782313,36.4316838463642));
#39883=CARTESIAN_POINT('Ctrl Pts',(20.9614997588273,4.33738505222762,36.4275379079875));
#39884=CARTESIAN_POINT('Ctrl Pts',(20.9359092066987,4.33932484826928,36.4129717865646));
#39885=CARTESIAN_POINT('Ctrl Pts',(20.9173506101544,4.34072945105316,36.4028087809869));
#39886=CARTESIAN_POINT('Ctrl Pts',(20.756386023795,4.35289808897262,36.3180732612595));
#39887=CARTESIAN_POINT('Ctrl Pts',(20.6053678323279,4.36430167294635,36.2612798463929));
#39888=CARTESIAN_POINT('Ctrl Pts',(20.3752160984411,4.38118371141086,36.2061872339147));
#39889=CARTESIAN_POINT('Ctrl Pts',(20.3003486242425,4.38658789881675,36.1928801400193));
#39890=CARTESIAN_POINT('Ctrl Pts',(20.1908774864044,4.39421567876447,36.1800310086192));
#39891=CARTESIAN_POINT('Ctrl Pts',(20.1567649979087,4.39655398616931,36.1769450777623));
#39892=CARTESIAN_POINT('Ctrl Pts',(20.1152795055091,4.39933707090263,36.1743035562436));
#39893=CARTESIAN_POINT('Ctrl Pts',(20.107970298142,4.39982513317179,36.1738799162987));
#39894=CARTESIAN_POINT('Ctrl Pts',(20.0965453393124,4.40058427269459,36.173282968261));
#39895=CARTESIAN_POINT('Ctrl Pts',(20.0924312397086,4.40085687836332,36.1730812187198));
#39896=CARTESIAN_POINT('Ctrl Pts',(20.0847577217977,4.4013638820609,36.1727295527508));
#39897=CARTESIAN_POINT('Ctrl Pts',(20.0811985701908,4.40159845418485,36.1725763203838));
#39898=CARTESIAN_POINT('Ctrl Pts',(20.0730749645417,4.40213253328741,36.172249116207));
#39899=CARTESIAN_POINT('Ctrl Pts',(20.068510309905,4.40243168509094,36.1720814957827));
#39900=CARTESIAN_POINT('Ctrl Pts',(20.0565955241875,4.40321016756088,36.1716863381664));
#39901=CARTESIAN_POINT('Ctrl Pts',(20.0492445272754,4.40368810854533,36.1714846092153));
#39902=CARTESIAN_POINT('Ctrl Pts',(20.0004644558289,4.40684509281832,36.1704250657989));
#39903=CARTESIAN_POINT('Ctrl Pts',(19.9590146427892,4.40945807098029,36.1708601835775));
#39904=CARTESIAN_POINT('Ctrl Pts',(19.9019037469233,4.41300153502812,36.1733015947855));
#39905=CARTESIAN_POINT('Ctrl Pts',(19.8862082919163,4.41396942925759,36.1741648333168));
#39906=CARTESIAN_POINT('Ctrl Pts',(19.7264549288851,4.42377583884161,36.1849110474046));
#39907=CARTESIAN_POINT('Ctrl Pts',(19.5839246020199,4.43218535577949,36.2107466641812));
#39908=CARTESIAN_POINT('Ctrl Pts',(19.4283607395475,4.44206076905504,36.2574215664436));
#39909=CARTESIAN_POINT('Ctrl Pts',(19.4111917622181,4.44316001812163,36.2628360542198));
#39910=CARTESIAN_POINT('Ctrl Pts',(19.3941039894965,4.44426476764078,36.2684889895619));
#39911=CARTESIAN_POINT('Origin',(20.,-1.3495818343519,38.1));
#39912=CARTESIAN_POINT('',(19.3941040111825,5.40852741588127,36.2684889823878));
#39913=CARTESIAN_POINT('',(19.3941040060237,5.23819447890751,36.2684889840944));
#39914=CARTESIAN_POINT('',(19.3941040087494,-1.3495818343519,36.2684889831927));
#39915=CARTESIAN_POINT('',(18.0708700373369,4.77280515976688,38.1003795462754));
#39916=CARTESIAN_POINT('Ctrl Pts',(19.3941040111825,5.40852741588127,36.2684889823878));
#39917=CARTESIAN_POINT('Ctrl Pts',(19.3991880386128,5.40816538004886,36.2668070968859));
#39918=CARTESIAN_POINT('Ctrl Pts',(19.4042794078024,5.40780435168272,36.2651462681862));
#39919=CARTESIAN_POINT('Ctrl Pts',(19.4182817146625,5.40681577153768,36.2606430827172));
#39920=CARTESIAN_POINT('Ctrl Pts',(19.4272063677185,5.40619047202091,36.2578443344489));
#39921=CARTESIAN_POINT('Ctrl Pts',(19.4404955126092,5.40526684166842,36.2537828077251));
#39922=CARTESIAN_POINT('Ctrl Pts',(19.4448445160974,5.40496575700304,36.2524704110074));
#39923=CARTESIAN_POINT('Ctrl Pts',(19.452610240741,5.40443028746982,36.2501568488366));
#39924=CARTESIAN_POINT('Ctrl Pts',(19.4560251273567,5.40419556585668,36.249149770754));
#39925=CARTESIAN_POINT('Ctrl Pts',(19.463413492578,5.40368934441415,36.2469930960361));
#39926=CARTESIAN_POINT('Ctrl Pts',(19.4673878774805,5.40341803749983,36.2458468256842));
#39927=CARTESIAN_POINT('Ctrl Pts',(19.4784833004892,5.40266333395217,36.242685363713));
#39928=CARTESIAN_POINT('Ctrl Pts',(19.4856123876216,5.40218152877578,36.2406983260948));
#39929=CARTESIAN_POINT('Ctrl Pts',(19.5270290774137,5.39939953049861,36.2294110067447));
#39930=CARTESIAN_POINT('Ctrl Pts',(19.5615594513908,5.39714775831503,36.2210175763786));
#39931=CARTESIAN_POINT('Ctrl Pts',(19.6754367559842,5.38988300878024,36.1966477094285));
#39932=CARTESIAN_POINT('Ctrl Pts',(19.755563058445,5.38502298326522,36.1847078517655));
#39933=CARTESIAN_POINT('Ctrl Pts',(19.9892148545015,5.37100147069778,36.1647978810955));
#39934=CARTESIAN_POINT('Ctrl Pts',(20.1432110042299,5.36189891966423,36.1700756734619));
#39935=CARTESIAN_POINT('Ctrl Pts',(20.3163850670617,5.35079429111706,36.1968674091198));
#39936=CARTESIAN_POINT('Ctrl Pts',(20.3377654206367,5.34940903980329,36.2005454389709));
#39937=CARTESIAN_POINT('Ctrl Pts',(20.367306935802,5.34747333968377,36.206141951392));
#39938=CARTESIAN_POINT('Ctrl Pts',(20.3755249855877,5.34693251874736,36.2077543301815));
#39939=CARTESIAN_POINT('Ctrl Pts',(20.389657692763,5.34599832276291,36.2106228545689));
#39940=CARTESIAN_POINT('Ctrl Pts',(20.3955774703059,5.345605761296,36.211853401133));
#39941=CARTESIAN_POINT('Ctrl Pts',(20.407795319013,5.34479291347448,36.2144531099749));
#39942=CARTESIAN_POINT('Ctrl Pts',(20.4140925016412,5.34437251192991,36.2158260443658));
#39943=CARTESIAN_POINT('Ctrl Pts',(20.4287796832729,5.34338853929661,36.219105381491));
#39944=CARTESIAN_POINT('Ctrl Pts',(20.4371639901137,5.34282419148356,36.2210363961933));
#39945=CARTESIAN_POINT('Ctrl Pts',(20.4641954662249,5.34099600686718,36.2274528152222));
#39946=CARTESIAN_POINT('Ctrl Pts',(20.4827882596725,5.33972512874099,36.2321601135299));
#39947=CARTESIAN_POINT('Ctrl Pts',(20.5775418096149,5.33317740889568,36.2576589345189));
#39948=CARTESIAN_POINT('Ctrl Pts',(20.6524352235758,5.32776143054545,36.2828317214629));
#39949=CARTESIAN_POINT('Ctrl Pts',(20.8244499607132,5.31476284712281,36.3526553247381));
#39950=CARTESIAN_POINT('Ctrl Pts',(20.9198261878247,5.3071043875358,36.4009272180223));
#39951=CARTESIAN_POINT('Ctrl Pts',(21.0833401702788,5.29345537040106,36.5015048252585));
#39952=CARTESIAN_POINT('Ctrl Pts',(21.1529342694767,5.28745766014602,36.5509490243489));
#39953=CARTESIAN_POINT('Ctrl Pts',(21.2262930487584,5.28109591982131,36.6107600549694));
#39954=CARTESIAN_POINT('Ctrl Pts',(21.2335081166738,5.28046981538039,36.6167306414235));
#39955=CARTESIAN_POINT('Ctrl Pts',(21.2441599536157,5.27954523057099,36.6256766895956));
#39956=CARTESIAN_POINT('Ctrl Pts',(21.2476300144534,5.27924398825386,36.6286120287744));
#39957=CARTESIAN_POINT('Ctrl Pts',(21.253799918635,5.27870834755838,36.6338686969156));
#39958=CARTESIAN_POINT('Ctrl Pts',(21.256503733473,5.2784736115598,36.6361852568228));
#39959=CARTESIAN_POINT('Ctrl Pts',(21.2623335794094,5.27796748288926,36.641208175672));
#39960=CARTESIAN_POINT('Ctrl Pts',(21.2654573212146,5.2776962824748,36.6439170966567));
#39961=CARTESIAN_POINT('Ctrl Pts',(21.2741421257917,5.27694217628809,36.6514976502051));
#39962=CARTESIAN_POINT('Ctrl Pts',(21.279684002884,5.27646085788835,36.6563913026208));
#39963=CARTESIAN_POINT('Ctrl Pts',(21.3115989454433,5.27368739919953,36.6849014090007));
#39964=CARTESIAN_POINT('Ctrl Pts',(21.33734801797,5.27144333296209,36.7092101241971));
#39965=CARTESIAN_POINT('Ctrl Pts',(21.4193583595566,5.26421625782154,36.7910181642371));
#39966=CARTESIAN_POINT('Ctrl Pts',(21.4726982577235,5.25938439338078,36.8513312674988));
#39967=CARTESIAN_POINT('Ctrl Pts',(21.6168920359138,5.24534938687466,37.0365159122747));
#39968=CARTESIAN_POINT('Ctrl Pts',(21.6967120389538,5.23620868997918,37.1691400404125));
#39969=CARTESIAN_POINT('Ctrl Pts',(21.7687537429784,5.22506217988023,37.329596580366));
#39970=CARTESIAN_POINT('Ctrl Pts',(21.7772875536383,5.22367973924915,37.3494934217528));
#39971=CARTESIAN_POINT('Ctrl Pts',(21.7886528771772,5.22174734839289,37.3772735934065));
#39972=CARTESIAN_POINT('Ctrl Pts',(21.791770835588,5.22120698238419,37.3850385724048));
#39973=CARTESIAN_POINT('Ctrl Pts',(21.7970539114562,5.22027336167576,37.3984471994491));
#39974=CARTESIAN_POINT('Ctrl Pts',(21.7992432202646,5.21988091822332,37.4040812363545));
#39975=CARTESIAN_POINT('Ctrl Pts',(21.8037125515931,5.2190681166288,37.4157448271036));
#39976=CARTESIAN_POINT('Ctrl Pts',(21.8059888997665,5.21864764242066,37.4217756988706));
#39977=CARTESIAN_POINT('Ctrl Pts',(21.8112351841841,5.2176631552338,37.4358887101227));
#39978=CARTESIAN_POINT('Ctrl Pts',(21.8141813016587,5.21709836309307,37.4439794984682));
#39979=CARTESIAN_POINT('Ctrl Pts',(21.823526929673,5.21526727872232,37.470189434586));
#39980=CARTESIAN_POINT('Ctrl Pts',(21.8297097400797,5.21399391392181,37.4883840801368));
#39981=CARTESIAN_POINT('Ctrl Pts',(21.8599896001415,5.20742419681477,37.5820622514077));
#39982=CARTESIAN_POINT('Ctrl Pts',(21.8796883574583,5.20198765216723,37.6588768843063));
#39983=CARTESIAN_POINT('Ctrl Pts',(21.9148823678888,5.18890137058507,37.8424016046207));
#39984=CARTESIAN_POINT('Ctrl Pts',(21.9262707062528,5.18117351364258,37.9496339572141));
#39985=CARTESIAN_POINT('Ctrl Pts',(21.9305178212104,5.1675522919379,38.1412273996601));
#39986=CARTESIAN_POINT('Ctrl Pts',(21.9268924371506,5.16164723017443,38.2252508842666));
#39987=CARTESIAN_POINT('Ctrl Pts',(21.9167865730074,5.15537112069426,38.3180810335139));
#39988=CARTESIAN_POINT('Ctrl Pts',(21.9157062698766,5.1547455644404,38.3273754601042));
#39989=CARTESIAN_POINT('Ctrl Pts',(21.914000984888,5.15382162964296,38.341170954119));
#39990=CARTESIAN_POINT('Ctrl Pts',(21.9134276764655,5.15352049468112,38.3456780968006));
#39991=CARTESIAN_POINT('Ctrl Pts',(21.9123767133476,5.15298497055235,38.3537134981451));
#39992=CARTESIAN_POINT('Ctrl Pts',(21.9119052106441,5.15275024436098,38.3572424909046));
#39993=CARTESIAN_POINT('Ctrl Pts',(21.9108648716343,5.15224405256711,38.3648680880695));
#39994=CARTESIAN_POINT('Ctrl Pts',(21.9102926320763,5.1519727796697,38.368964165555));
#39995=CARTESIAN_POINT('Ctrl Pts',(21.9086600405253,5.15121826693924,38.3803821320283));
#39996=CARTESIAN_POINT('Ctrl Pts',(21.9075707218813,5.15073661725777,38.3876999054512));
#39997=CARTESIAN_POINT('Ctrl Pts',(21.9010125764314,5.14795735063021,38.4300803265439));
#39998=CARTESIAN_POINT('Ctrl Pts',(21.8946188116473,5.14570804350205,38.4649955927218));
#39999=CARTESIAN_POINT('Ctrl Pts',(21.870530159364,5.13845536235766,38.5787301842942));
#40000=CARTESIAN_POINT('Ctrl Pts',(21.8488484789114,5.13360436001436,38.6566211905362));
#40001=CARTESIAN_POINT('Ctrl Pts',(21.7718904546084,5.11957855216328,38.8782007162131));
#40002=CARTESIAN_POINT('Ctrl Pts',(21.704253625311,5.11046379542079,39.0168999175403));
#40003=CARTESIAN_POINT('Ctrl Pts',(21.6091173859968,5.0993457601127,39.164309069245));
#40004=CARTESIAN_POINT('Ctrl Pts',(21.5970556067822,5.09796139676457,39.1823242977118));
#40005=CARTESIAN_POINT('Ctrl Pts',(21.5799185485579,5.09602674192398,39.2070095011182));
#40006=CARTESIAN_POINT('Ctrl Pts',(21.5750992730607,5.09548606449814,39.2138558847679));
#40007=CARTESIAN_POINT('Ctrl Pts',(21.5667235417695,5.09455205000147,39.2255916007818));
#40008=CARTESIAN_POINT('Ctrl Pts',(21.5631883589015,5.09415952577516,39.2304960244514));
#40009=CARTESIAN_POINT('Ctrl Pts',(21.5558367501928,5.09334669260483,39.2405946290237));
#40010=CARTESIAN_POINT('Ctrl Pts',(21.5520172342859,5.09292626819478,39.2457864564574));
#40011=CARTESIAN_POINT('Ctrl Pts',(21.543037332928,5.09194213351084,39.2578654533845));
#40012=CARTESIAN_POINT('Ctrl Pts',(21.5378567697963,5.09137764574495,39.264737382631));
#40013=CARTESIAN_POINT('Ctrl Pts',(21.5209758615354,5.08954854810378,39.2868206545022));
#40014=CARTESIAN_POINT('Ctrl Pts',(21.5090947730772,5.08827688707479,39.3018917414638));
#40015=CARTESIAN_POINT('Ctrl Pts',(21.4471388807125,5.081722245921,39.3781152364297));
#40016=CARTESIAN_POINT('Ctrl Pts',(21.3935710607686,5.0762997974627,39.4363181945111));
#40017=CARTESIAN_POINT('Ctrl Pts',(21.2594148184122,5.06327242541221,39.5652207857936));
#40018=CARTESIAN_POINT('Ctrl Pts',(21.1762041270946,5.05559087341416,39.6328205580282));
#40019=CARTESIAN_POINT('Ctrl Pts',(21.0774565754292,5.04709028615795,39.7002460795997));
#40020=CARTESIAN_POINT('Ctrl Pts',(21.0670190235063,5.04619911305068,39.7072245010125));
#40021=CARTESIAN_POINT('Ctrl Pts',(20.9958672822816,5.04017643008372,39.7537970694446));
#40022=CARTESIAN_POINT('Ctrl Pts',(20.9330238544696,5.03511094492634,39.7900489264387));
#40023=CARTESIAN_POINT('Ctrl Pts',(20.8600341311524,5.02961846174217,39.8268379082042));
#40024=CARTESIAN_POINT('Ctrl Pts',(20.8517562293733,5.02900104103948,39.8309359323856));
#40025=CARTESIAN_POINT('Ctrl Pts',(20.8393842972494,5.02808675963082,39.836950484352));
#40026=CARTESIAN_POINT('Ctrl Pts',(20.835312597504,5.02778722399254,39.8389122603063));
#40027=CARTESIAN_POINT('Ctrl Pts',(20.8280228471142,5.02725343063717,39.8423930050124));
#40028=CARTESIAN_POINT('Ctrl Pts',(20.8248074634435,5.02701884477712,39.8439173914519));
#40029=CARTESIAN_POINT('Ctrl Pts',(20.817830389544,5.02651168629267,39.8472015502006));
#40030=CARTESIAN_POINT('Ctrl Pts',(20.8140672379939,5.02623931314037,39.8489580715139));
#40031=CARTESIAN_POINT('Ctrl Pts',(20.8035134062977,5.02547862131503,39.8538428267433));
#40032=CARTESIAN_POINT('Ctrl Pts',(20.7967100787733,5.02499193530327,39.856943798148));
#40033=CARTESIAN_POINT('Ctrl Pts',(20.7563064467096,5.02212234113683,39.8750769120927));
#40034=CARTESIAN_POINT('Ctrl Pts',(20.7222969509855,5.0197914882729,39.8891855766013));
#40035=CARTESIAN_POINT('Ctrl Pts',(20.6074214476066,5.01213089552774,39.9330309380568));
#40036=CARTESIAN_POINT('Ctrl Pts',(20.5249668171731,5.00697376221909,39.9583260107477));
#40037=CARTESIAN_POINT('Ctrl Pts',(20.2985948255472,4.99308047694332,40.0114939398307));
#40038=CARTESIAN_POINT('Ctrl Pts',(20.1527711204213,4.98437252386747,40.0286323320604));
#40039=CARTESIAN_POINT('Ctrl Pts',(19.9843492298928,4.97370358268398,40.029192758108));
#40040=CARTESIAN_POINT('Ctrl Pts',(19.9622804120588,4.97229465559702,40.0288874549252));
#40041=CARTESIAN_POINT('Ctrl Pts',(19.9317928362042,4.97033115840127,40.0279422878542));
#40042=CARTESIAN_POINT('Ctrl Pts',(19.9233652031772,4.96978658820653,40.0276256863591));
#40043=CARTESIAN_POINT('Ctrl Pts',(19.9088841305744,4.96884764690859,40.026986559511));
#40044=CARTESIAN_POINT('Ctrl Pts',(19.9028295875198,4.96845410868939,40.0266907410753));
#40045=CARTESIAN_POINT('Ctrl Pts',(19.8903491526946,4.96764085612944,40.0260219830605));
#40046=CARTESIAN_POINT('Ctrl Pts',(19.8839235394651,4.96722103375196,40.0256454089933));
#40047=CARTESIAN_POINT('Ctrl Pts',(19.8689673897648,4.96624120850582,40.0246937709874));
#40048=CARTESIAN_POINT('Ctrl Pts',(19.860438605458,4.96568044855747,40.024094142762));
#40049=CARTESIAN_POINT('Ctrl Pts',(19.8330882180428,4.96387556747299,40.0219884319284));
#40050=CARTESIAN_POINT('Ctrl Pts',(19.8142851176624,4.96262465351862,40.0202627463547));
#40051=CARTESIAN_POINT('Ctrl Pts',(19.7192938011134,4.95625210490988,40.0101365527305));
#40052=CARTESIAN_POINT('Ctrl Pts',(19.6436383609901,4.95099958533525,39.9974776316555));
#40053=CARTESIAN_POINT('Ctrl Pts',(19.4862357178023,4.93970717476183,39.9613943682751));
#40054=CARTESIAN_POINT('Ctrl Pts',(19.4048730934031,4.93365443209155,39.9369989096747));
#40055=CARTESIAN_POINT('Ctrl Pts',(19.2221401898552,4.91973806694476,39.8687909955374));
#40056=CARTESIAN_POINT('Ctrl Pts',(19.1223734372587,4.91189504265054,39.821471747952));
#40057=CARTESIAN_POINT('Ctrl Pts',(19.0192827156919,4.90387420619512,39.7612705672334));
#40058=CARTESIAN_POINT('Ctrl Pts',(19.0114135771843,4.90326259359369,39.7565998859226));
#40059=CARTESIAN_POINT('Ctrl Pts',(18.9997223945682,4.90235521155407,39.7495476778188));
#40060=CARTESIAN_POINT('Ctrl Pts',(18.9958751114022,4.90205682467886,39.7472085594865));
#40061=CARTESIAN_POINT('Ctrl Pts',(18.9890760845084,4.90152992900205,39.7430421312622));
#40062=CARTESIAN_POINT('Ctrl Pts',(18.9861210599646,4.90130107177643,39.7412203092905));
#40063=CARTESIAN_POINT('Ctrl Pts',(18.9797363722117,4.9008069180052,39.7372602177558));
#40064=CARTESIAN_POINT('Ctrl Pts',(18.976308514043,4.9005418079512,39.7351191495283));
#40065=CARTESIAN_POINT('Ctrl Pts',(18.9692168010084,4.89999368540055,39.7306585654015));
#40066=CARTESIAN_POINT('Ctrl Pts',(18.9655539828095,4.89971077855935,39.7283374339005));
#40067=CARTESIAN_POINT('Ctrl Pts',(18.9562632785317,4.89899359971221,39.7224059048746));
#40068=CARTESIAN_POINT('Ctrl Pts',(18.950646225,4.89856038749363,39.7187785277426));
#40069=CARTESIAN_POINT('Ctrl Pts',(18.9344906281144,4.89731516510938,39.7082261490912));
#40070=CARTESIAN_POINT('Ctrl Pts',(18.9240007615181,4.89650759034226,39.7012267877368));
#40071=CARTESIAN_POINT('Ctrl Pts',(18.8837340273822,4.89340818782832,39.6737844039996));
#40072=CARTESIAN_POINT('Ctrl Pts',(18.8544632186173,4.89115635348185,39.6526084161405));
#40073=CARTESIAN_POINT('Ctrl Pts',(18.6825985095421,4.87783010040515,39.5207645270164));
#40074=CARTESIAN_POINT('Ctrl Pts',(18.5555166480364,4.86744540559465,39.3913538853965));
#40075=CARTESIAN_POINT('Ctrl Pts',(18.4175652353201,4.85309467892754,39.2045874550899));
#40076=CARTESIAN_POINT('Ctrl Pts',(18.3885465122739,4.84985078677518,39.1618051392593));
#40077=CARTESIAN_POINT('Ctrl Pts',(18.35453675329,4.84572370455568,39.1070534604185));
#40078=CARTESIAN_POINT('Ctrl Pts',(18.3478998601058,4.84490138031002,39.0961280457177));
#40079=CARTESIAN_POINT('Ctrl Pts',(18.3375945820565,4.84359697460574,39.0787775562806));
#40080=CARTESIAN_POINT('Ctrl Pts',(18.3338536573346,4.8431175178173,39.0723958250589));
#40081=CARTESIAN_POINT('Ctrl Pts',(18.3269724457064,4.84222435823489,39.0605007114706));
#40082=CARTESIAN_POINT('Ctrl Pts',(18.3238224657101,4.84181101045498,39.054993029345));
#40083=CARTESIAN_POINT('Ctrl Pts',(18.3169098517817,4.84089384334767,39.0427668876078));
#40084=CARTESIAN_POINT('Ctrl Pts',(18.3131601737517,4.84038957097797,39.0360412646298));
#40085=CARTESIAN_POINT('Ctrl Pts',(18.3024426141714,4.83892836677434,39.0165441288778));
#40086=CARTESIAN_POINT('Ctrl Pts',(18.2955789367443,4.83796778011384,39.003716237477));
#40087=CARTESIAN_POINT('Ctrl Pts',(18.2427058215877,4.8303671046717,38.902153598844));
#40088=CARTESIAN_POINT('Ctrl Pts',(18.2035182023266,4.82349015899611,38.8100567514915));
#40089=CARTESIAN_POINT('Ctrl Pts',(18.1185161939014,4.80472129942341,38.5574958819093));
#40090=CARTESIAN_POINT('Ctrl Pts',(18.0860555955714,4.79257447840611,38.3934294727711));
#40091=CARTESIAN_POINT('Ctrl Pts',(18.0739063613322,4.7800373981577,38.2096236511995));
#40092=CARTESIAN_POINT('Ctrl Pts',(18.0729840017851,4.77884665265958,38.1919969931562));
#40093=CARTESIAN_POINT('Ctrl Pts',(18.0720702781831,4.77726412508938,38.1683095854994));
#40094=CARTESIAN_POINT('Ctrl Pts',(18.0718653881356,4.77686141086359,38.1622585953465));
#40095=CARTESIAN_POINT('Ctrl Pts',(18.0715882886031,4.7762312450856,38.1527519949349));
#40096=CARTESIAN_POINT('Ctrl Pts',(18.0714968750493,4.77600275151252,38.1492970500773));
#40097=CARTESIAN_POINT('Ctrl Pts',(18.0713331534435,4.77554829423259,38.1424092147729));
#40098=CARTESIAN_POINT('Ctrl Pts',(18.0712607265042,4.77532233398187,38.1389764229896));
#40099=CARTESIAN_POINT('Ctrl Pts',(18.0711324168621,4.77486506854656,38.1320135525227));
#40100=CARTESIAN_POINT('Ctrl Pts',(18.071077059447,4.77463379472688,38.1284835167032));
#40101=CARTESIAN_POINT('Ctrl Pts',(18.070974109491,4.77411359661182,38.1205251656839));
#40102=CARTESIAN_POINT('Ctrl Pts',(18.0709320739607,4.77382497325852,38.1160967804167));
#40103=CARTESIAN_POINT('Ctrl Pts',(18.0708825280288,4.77329258062598,38.1079054148909));
#40104=CARTESIAN_POINT('Ctrl Pts',(18.0708707776788,4.77304859236824,38.1041425018261));
#40105=CARTESIAN_POINT('Ctrl Pts',(18.0708700373369,4.77280515976688,38.1003795462754));
#40106=CARTESIAN_POINT('Ctrl Pts',(18.0708700375362,4.77280522521772,38.1003805580074));
#40107=CARTESIAN_POINT('Ctrl Pts',(18.0708659381183,4.7714608743111,38.0795997316186));
#40108=CARTESIAN_POINT('Ctrl Pts',(18.0711976193021,4.77013355924366,38.0588190267461));
#40109=CARTESIAN_POINT('Ctrl Pts',(18.074831050733,4.76298387999448,37.945738140098));
#40110=CARTESIAN_POINT('Ctrl Pts',(18.0844224177032,4.75742956583471,37.8537511740746));
#40111=CARTESIAN_POINT('Ctrl Pts',(18.115987995365,4.74662860232346,37.6759454899839));
#40112=CARTESIAN_POINT('Ctrl Pts',(18.1373451636114,4.74139091150783,37.5902551835509));
#40113=CARTESIAN_POINT('Ctrl Pts',(18.1868297277635,4.73161359693041,37.4372586891911));
#40114=CARTESIAN_POINT('Ctrl Pts',(18.2130484885359,4.72712347764275,37.3695104302234));
#40115=CARTESIAN_POINT('Ctrl Pts',(18.2505950579448,4.72133855539074,37.2866971946763));
#40116=CARTESIAN_POINT('Ctrl Pts',(18.2584080737755,4.72016375086269,37.270098421495));
#40117=CARTESIAN_POINT('Ctrl Pts',(18.2701642514357,4.71843591550264,37.2460197536588));
#40118=CARTESIAN_POINT('Ctrl Pts',(18.2739219028291,4.71788927179635,37.2384500148661));
#40119=CARTESIAN_POINT('Ctrl Pts',(18.2806221909896,4.71692420705392,37.2251721623131));
#40120=CARTESIAN_POINT('Ctrl Pts',(18.2835438385288,4.71650652039566,37.2194535561385));
#40121=CARTESIAN_POINT('Ctrl Pts',(18.2892925807152,4.71569065020415,37.2083387452328));
#40122=CARTESIAN_POINT('Ctrl Pts',(18.2921167933324,4.71529257131145,37.2029411286855));
#40123=CARTESIAN_POINT('Ctrl Pts',(18.2997688409181,4.71422122988123,37.1884837081666));
#40124=CARTESIAN_POINT('Ctrl Pts',(18.3046434530014,4.71354632791796,37.1794490148496));
#40125=CARTESIAN_POINT('Ctrl Pts',(18.3229109258643,4.71104442305891,37.1462290184723));
#40126=CARTESIAN_POINT('Ctrl Pts',(18.3367505631413,4.70920166940098,37.1222945102947));
#40127=CARTESIAN_POINT('Ctrl Pts',(18.3528646417998,4.70711193484323,37.0957593724653));
#40128=CARTESIAN_POINT('Ctrl Pts',(18.3546378323777,4.70688270825547,37.0928567811197));
#40129=CARTESIAN_POINT('Ctrl Pts',(18.4417382973849,4.69565830386941,36.9511232431792));
#40130=CARTESIAN_POINT('Ctrl Pts',(18.5442928323567,4.6840110782204,36.8236793464117));
#40131=CARTESIAN_POINT('Ctrl Pts',(18.7274353646957,4.66590323811408,36.6472522025695));
#40132=CARTESIAN_POINT('Ctrl Pts',(18.7976941549391,4.65945113761711,36.588589507283));
#40133=CARTESIAN_POINT('Ctrl Pts',(18.8775045924654,4.65283130777619,36.5310528679023));
#40134=CARTESIAN_POINT('Ctrl Pts',(18.8831751334614,4.6523646207483,36.5270113591505));
#40135=CARTESIAN_POINT('Ctrl Pts',(18.8925059175718,4.65160282285846,36.5204370148893));
#40136=CARTESIAN_POINT('Ctrl Pts',(18.8961532054959,4.65130656698276,36.5178860275668));
#40137=CARTESIAN_POINT('Ctrl Pts',(18.9031995789978,4.65073719188104,36.5129938792128));
#40138=CARTESIAN_POINT('Ctrl Pts',(18.9065974090099,4.6504639582083,36.5106509616404));
#40139=CARTESIAN_POINT('Ctrl Pts',(18.9100169678687,4.65019032563652,36.5083092175733));
#40140=CARTESIAN_POINT('Ctrl Pts',(18.9100311645579,4.65018918964293,36.5082994958344));
#40141=CARTESIAN_POINT('Ctrl Pts',(18.9100596875963,4.65018690732738,36.5082799641273));
#40142=CARTESIAN_POINT('Ctrl Pts',(18.9100740139145,4.65018576100832,36.5082701541854));
#40143=CARTESIAN_POINT('Ctrl Pts',(18.9101027990276,4.65018345781774,36.5082504441591));
#40144=CARTESIAN_POINT('Ctrl Pts',(18.9101172577129,4.65018230095543,36.5082405441551));
#40145=CARTESIAN_POINT('Ctrl Pts',(18.9101463102378,4.65017997646543,36.5082206521868));
#40146=CARTESIAN_POINT('Ctrl Pts',(18.910160904294,4.65017880882086,36.5082106600798));
#40147=CARTESIAN_POINT('Ctrl Pts',(18.9101902306377,4.65017646252155,36.5081905818154));
#40148=CARTESIAN_POINT('Ctrl Pts',(18.9102049627863,4.65017528387839,36.5081804957587));
#40149=CARTESIAN_POINT('Ctrl Pts',(18.9102345682621,4.65017291534747,36.5081602275939));
#40150=CARTESIAN_POINT('Ctrl Pts',(18.9102494417545,4.65017172544699,36.5081500453785));
#40151=CARTESIAN_POINT('Ctrl Pts',(18.9102793332182,4.65016933413889,36.5081295826545));
#40152=CARTESIAN_POINT('Ctrl Pts',(18.9102943509284,4.65016813275265,36.5081193023305));
#40153=CARTESIAN_POINT('Ctrl Pts',(18.9103245340155,4.65016571821952,36.5080986412252));
#40154=CARTESIAN_POINT('Ctrl Pts',(18.9103396993734,4.65016450507465,36.5080882604629));
#40155=CARTESIAN_POINT('Ctrl Pts',(18.9103701810668,4.65016206676097,36.5080673962331));
#40156=CARTESIAN_POINT('Ctrl Pts',(18.9103854972447,4.65016084160528,36.5080569128798));
#40157=CARTESIAN_POINT('Ctrl Pts',(18.9104162836217,4.6501583790281,36.5080358414039));
#40158=CARTESIAN_POINT('Ctrl Pts',(18.9104317542608,4.65015714157195,36.5080252529866));
#40159=CARTESIAN_POINT('Ctrl Pts',(18.9104628534336,4.65015465408568,36.5080039687516));
#40160=CARTESIAN_POINT('Ctrl Pts',(18.9104784815412,4.6501534040902,36.5079932732322));
#40161=CARTESIAN_POINT('Ctrl Pts',(18.9105098989393,4.65015089126395,36.5079717725629));
#40162=CARTESIAN_POINT('Ctrl Pts',(18.9105256887033,4.6501496283959,36.5079609670958));
#40163=CARTESIAN_POINT('Ctrl Pts',(18.9105574331311,4.650147089529,36.5079392440086));
#40164=CARTESIAN_POINT('Ctrl Pts',(18.9105733878038,4.65014581353005,36.5079283263897));
#40165=CARTESIAN_POINT('Ctrl Pts',(18.910605466169,4.65014324807367,36.5079063762012));
#40166=CARTESIAN_POINT('Ctrl Pts',(18.9106215896509,4.65014195863372,36.5078953437833));
#40167=CARTESIAN_POINT('Ctrl Pts',(18.910654009238,4.65013936600904,36.5078731615538));
#40168=CARTESIAN_POINT('Ctrl Pts',(18.9106703057407,4.65013806279318,36.507862011478));
#40169=CARTESIAN_POINT('Ctrl Pts',(18.9107030758268,4.6501354422622,36.5078395909064));
#40170=CARTESIAN_POINT('Ctrl Pts',(18.9107195489025,4.65013412498835,36.5078283207659));
#40171=CARTESIAN_POINT('Ctrl Pts',(18.9107526761783,4.65013147602005,36.5078056573225));
#40172=CARTESIAN_POINT('Ctrl Pts',(18.9107693305324,4.65013014431397,36.5077942639224));
#40173=CARTESIAN_POINT('Ctrl Pts',(18.9108028243766,4.65012746616255,36.5077713512406));
#40174=CARTESIAN_POINT('Ctrl Pts',(18.9108196641439,4.65012611969576,36.5077598317777));
#40175=CARTESIAN_POINT('Ctrl Pts',(18.9136961643979,4.64989612733629,36.5057921911733));
#40176=CARTESIAN_POINT('Ctrl Pts',(18.9165610486414,4.64966801310293,36.5038438046669));
#40177=CARTESIAN_POINT('Ctrl Pts',(18.923219567189,4.64914001170268,36.4993415825901));
#40178=CARTESIAN_POINT('Ctrl Pts',(18.9270170416057,4.64884051157304,36.4967935124357));
#40179=CARTESIAN_POINT('Ctrl Pts',(18.9382979926108,4.64795550385276,36.4892821352962));
#40180=CARTESIAN_POINT('Ctrl Pts',(18.9458072294981,4.64737249428316,36.4843574645493));
#40181=CARTESIAN_POINT('Ctrl Pts',(19.045155588486,4.63973533297612,36.4201908855883));
#40182=CARTESIAN_POINT('Ctrl Pts',(19.1418482235563,4.63314897649412,36.368795374594));
#40183=CARTESIAN_POINT('Ctrl Pts',(19.2921450377107,4.62337030233198,36.3046139053964));
#40184=CARTESIAN_POINT('Ctrl Pts',(19.3427625414602,4.62015039871559,36.2854736404772));
#40185=CARTESIAN_POINT('Ctrl Pts',(19.3941040488142,4.61690666843697,36.2684889699386));
#40186=CARTESIAN_POINT('Ctrl Pts',(19.3941039894965,4.44426476764078,36.2684889895619));
#40187=CARTESIAN_POINT('Ctrl Pts',(19.342277380928,4.44761543374737,36.2856341419474));
#40188=CARTESIAN_POINT('Ctrl Pts',(19.2911978070745,4.45101761072027,36.3049726973428));
#40189=CARTESIAN_POINT('Ctrl Pts',(19.2241346286758,4.45565854241324,36.3336727032339));
#40190=CARTESIAN_POINT('Ctrl Pts',(19.2073710249909,4.45683350062566,36.3411314816783));
#40191=CARTESIAN_POINT('Ctrl Pts',(19.1830448952451,4.4585615195637,36.352373511768));
#40192=CARTESIAN_POINT('Ctrl Pts',(19.1753964688773,4.45910819119435,36.3559693241574));
#40193=CARTESIAN_POINT('Ctrl Pts',(19.1619785271181,4.46007328703411,36.3623855987767));
#40194=CARTESIAN_POINT('Ctrl Pts',(19.1561989663204,4.46049097670208,36.3651848483913));
#40195=CARTESIAN_POINT('Ctrl Pts',(19.1449643782537,4.46130683904334,36.3706955874682));
#40196=CARTESIAN_POINT('Ctrl Pts',(19.1395079999423,4.46170490701279,36.3734041636602));
#40197=CARTESIAN_POINT('Ctrl Pts',(19.1248917813527,4.46277618548764,36.3807462275481));
#40198=CARTESIAN_POINT('Ctrl Pts',(19.1157560450749,4.46345103507833,36.3854270065885));
#40199=CARTESIAN_POINT('Ctrl Pts',(19.0821602772416,4.46595251512275,36.4029800291943));
#40200=CARTESIAN_POINT('Ctrl Pts',(19.0579413626133,4.46779488933996,36.4163040868929));
#40201=CARTESIAN_POINT('Ctrl Pts',(19.0283577232081,4.47009545444076,36.4334176875645));
#40202=CARTESIAN_POINT('Ctrl Pts',(19.0227141205297,4.47053661958971,36.436720821322));
#40203=CARTESIAN_POINT('Ctrl Pts',(18.8723464484676,4.48235256536877,36.5257587411399));
#40204=CARTESIAN_POINT('Ctrl Pts',(18.7394577072785,4.49441976552719,36.6300168299211));
#40205=CARTESIAN_POINT('Ctrl Pts',(18.5806972833031,4.51054637765621,36.792111353641));
#40206=CARTESIAN_POINT('Ctrl Pts',(18.5415308272271,4.5146892878991,36.8359345002157));
#40207=CARTESIAN_POINT('Ctrl Pts',(18.4859577526585,4.52075047293521,36.9041433057419));
#40208=CARTESIAN_POINT('Ctrl Pts',(18.4680088508538,4.52273981546695,36.9272252953545));
#40209=CARTESIAN_POINT('Ctrl Pts',(18.446435470455,4.52516240532702,36.9563092860602));
#40210=CARTESIAN_POINT('Ctrl Pts',(18.4423108607557,4.52562707034779,36.9619333298244));
#40211=CARTESIAN_POINT('Ctrl Pts',(18.4358437074141,4.52635785116144,36.9708525375414));
#40212=CARTESIAN_POINT('Ctrl Pts',(18.4334809164361,4.52662531785492,36.9741328403451));
#40213=CARTESIAN_POINT('Ctrl Pts',(18.4290478014908,4.52712800397608,36.9803283824271));
#40214=CARTESIAN_POINT('Ctrl Pts',(18.4269752952509,4.52736336629001,36.9832419153261));
#40215=CARTESIAN_POINT('Ctrl Pts',(18.4222482479448,4.52790102807053,36.989926474489));
#40216=CARTESIAN_POINT('Ctrl Pts',(18.419599121025,4.52820295922552,36.9937012672988));
#40217=CARTESIAN_POINT('Ctrl Pts',(18.412582147445,4.52900446264744,37.0037765323985));
#40218=CARTESIAN_POINT('Ctrl Pts',(18.4082382242734,4.52950246876849,37.0100936812771));
#40219=CARTESIAN_POINT('Ctrl Pts',(18.3769791101784,4.53310085410958,37.0561377576694));
#40220=CARTESIAN_POINT('Ctrl Pts',(18.3515142958922,4.5361124003198,37.0968345348454));
#40221=CARTESIAN_POINT('Ctrl Pts',(18.3213839965201,4.53983806415834,37.1492392644417));
#40222=CARTESIAN_POINT('Ctrl Pts',(18.3152809186123,4.54060195138256,37.1600961269484));
#40223=CARTESIAN_POINT('Ctrl Pts',(18.3034703547882,4.54210017000668,37.1815908145188));
#40224=CARTESIAN_POINT('Ctrl Pts',(18.2977567494189,4.54283465246564,37.192224591303));
#40225=CARTESIAN_POINT('Ctrl Pts',(18.2232987221485,4.55254578243759,37.3339760846133));
#40226=CARTESIAN_POINT('Ctrl Pts',(18.1697706234556,4.56117957338409,37.4725272174811));
#40227=CARTESIAN_POINT('Ctrl Pts',(18.1171271108378,4.57406590158306,37.675571076523));
#40228=CARTESIAN_POINT('Ctrl Pts',(18.1045166643854,4.57792289396945,37.7360055646947));
#40229=CARTESIAN_POINT('Ctrl Pts',(18.0927790913086,4.58270641230505,37.8097924337942));
#40230=CARTESIAN_POINT('Ctrl Pts',(18.0908642036136,4.58354381987234,37.8226689278753));
#40231=CARTESIAN_POINT('Ctrl Pts',(18.0880691824803,4.58486190149556,37.8428668340428));
#40232=CARTESIAN_POINT('Ctrl Pts',(18.0871004317981,4.58533979580818,37.8501757507832));
#40233=CARTESIAN_POINT('Ctrl Pts',(18.0854560257531,4.58619002910327,37.8631529770334));
#40234=CARTESIAN_POINT('Ctrl Pts',(18.0847635831155,4.58656183773636,37.8688191013864));
#40235=CARTESIAN_POINT('Ctrl Pts',(18.083224381568,4.58742130389915,37.8818958515913));
#40236=CARTESIAN_POINT('Ctrl Pts',(18.0823954379501,4.58790951242751,37.8893084435798));
#40237=CARTESIAN_POINT('Ctrl Pts',(18.0802342125939,4.5892557559151,37.9097048808603));
#40238=CARTESIAN_POINT('Ctrl Pts',(18.0789906993057,4.59011654245713,37.9226975370993));
#40239=CARTESIAN_POINT('Ctrl Pts',(18.0731723313726,4.59464386352464,37.9907663842874));
#40240=CARTESIAN_POINT('Ctrl Pts',(18.0708343488707,4.59837915537304,38.0460028132912));
#40241=CARTESIAN_POINT('Ctrl Pts',(18.0709498218806,4.6105497491215,38.2229377848043));
#40242=CARTESIAN_POINT('Ctrl Pts',(18.0825413521376,4.61923104985422,38.3443233771193));
#40243=CARTESIAN_POINT('Ctrl Pts',(18.1175539347502,4.63247233532486,38.5266582564846));
#40244=CARTESIAN_POINT('Ctrl Pts',(18.1327481058244,4.63702310965439,38.5888882362978));
#40245=CARTESIAN_POINT('Ctrl Pts',(18.1628406294784,4.64437027935933,38.6900072829057));
#40246=CARTESIAN_POINT('Ctrl Pts',(18.1759523338027,4.64721803189036,38.7293757661469));
#40247=CARTESIAN_POINT('Ctrl Pts',(18.1928726174228,4.65049360651855,38.7751942585372));
#40248=CARTESIAN_POINT('Ctrl Pts',(18.1954603018088,4.65098481885081,38.7820800140119));
#40249=CARTESIAN_POINT('Ctrl Pts',(18.1997188412586,4.65177747286423,38.7932179858108));
#40250=CARTESIAN_POINT('Ctrl Pts',(18.2013654968813,4.65208028268403,38.7974792840132));
#40251=CARTESIAN_POINT('Ctrl Pts',(18.2043231834156,4.65261763016177,38.8050532027856));
#40252=CARTESIAN_POINT('Ctrl Pts',(18.2056282656372,4.65285251413309,38.8083680738398));
#40253=CARTESIAN_POINT('Ctrl Pts',(18.2084619366215,4.65335774364732,38.8155074330495));
#40254=CARTESIAN_POINT('Ctrl Pts',(18.2099935888636,4.65362790338111,38.819330638968));
#40255=CARTESIAN_POINT('Ctrl Pts',(18.2142811644712,4.65437618159171,38.8299344961409));
#40256=CARTESIAN_POINT('Ctrl Pts',(18.2170634865512,4.65485275228769,38.8367045007419));
#40257=CARTESIAN_POINT('Ctrl Pts',(18.2330687612004,4.65754471675089,38.8750270634534));
#40258=CARTESIAN_POINT('Ctrl Pts',(18.2470916078546,4.65971528021714,38.9062415701925));
#40259=CARTESIAN_POINT('Ctrl Pts',(18.294849317494,4.66659047889873,39.005404080609));
#40260=CARTESIAN_POINT('Ctrl Pts',(18.3317646423561,4.67116031697851,39.0717448757472));
#40261=CARTESIAN_POINT('Ctrl Pts',(18.4588856630847,4.68533373287125,39.2714952433936));
#40262=CARTESIAN_POINT('Ctrl Pts',(18.5619101512575,4.69483691691506,39.3958881181633));
#40263=CARTESIAN_POINT('Ctrl Pts',(18.694585457383,4.70637894286772,39.5205218948371));
#40264=CARTESIAN_POINT('Ctrl Pts',(18.7102319339443,4.70772955475721,39.5347431343674));
#40265=CARTESIAN_POINT('Ctrl Pts',(18.7323301588831,4.70962436014981,39.5541748073917));
#40266=CARTESIAN_POINT('Ctrl Pts',(18.7385869069945,4.71015945634237,39.5596054952692));
#40267=CARTESIAN_POINT('Ctrl Pts',(18.7494522552614,4.71108642096732,39.5689142831526));
#40268=CARTESIAN_POINT('Ctrl Pts',(18.754044429717,4.7114775050539,39.5728114436807));
#40269=CARTESIAN_POINT('Ctrl Pts',(18.7635989688621,4.71228981663906,39.5808432621517));
#40270=CARTESIAN_POINT('Ctrl Pts',(18.7685639931474,4.71271117049215,39.5849746247623));
#40271=CARTESIAN_POINT('Ctrl Pts',(18.7802574504655,4.71370180042368,39.5946056964064));
#40272=CARTESIAN_POINT('Ctrl Pts',(18.7870024393359,4.71427188478842,39.6000849937698));
#40273=CARTESIAN_POINT('Ctrl Pts',(18.8091275158877,4.71613775018829,39.6178115240582));
#40274=CARTESIAN_POINT('Ctrl Pts',(18.8246574318935,4.71744098423163,39.6298689143832));
#40275=CARTESIAN_POINT('Ctrl Pts',(18.9064990489981,4.72427808287934,39.6914288509686));
#40276=CARTESIAN_POINT('Ctrl Pts',(18.9757526096318,4.72996532305593,39.7368580035714));
#40277=CARTESIAN_POINT('Ctrl Pts',(19.1534151282146,4.744298405395,39.8377033741452));
#40278=CARTESIAN_POINT('Ctrl Pts',(19.2645636725165,4.75306117534925,39.887582050363));
#40279=CARTESIAN_POINT('Ctrl Pts',(19.4006362288088,4.76321379989973,39.9337929606624));
#40280=CARTESIAN_POINT('Ctrl Pts',(19.4217395676946,4.76477198998715,39.9405565682163));
#40281=CARTESIAN_POINT('Ctrl Pts',(19.4863777360521,4.76948675067154,39.9600515438007));
#40282=CARTESIAN_POINT('Ctrl Pts',(19.5302526670263,4.77260806761195,39.9716136827948));
#40283=CARTESIAN_POINT('Ctrl Pts',(19.5818610045382,4.77615794681975,39.9832841847271));
#40284=CARTESIAN_POINT('Ctrl Pts',(19.5892336646776,4.77666220547482,39.9849059823511));
#40285=CARTESIAN_POINT('Ctrl Pts',(19.6010915652467,4.77746842633347,39.9874415397527));
#40286=CARTESIAN_POINT('Ctrl Pts',(19.6055707784907,4.77777186968143,39.9883826666202));
#40287=CARTESIAN_POINT('Ctrl Pts',(19.6135509108052,4.7783104753695,39.9900297384878));
#40288=CARTESIAN_POINT('Ctrl Pts',(19.6170504853764,4.77854598533409,39.9907419128352));
#40289=CARTESIAN_POINT('Ctrl Pts',(19.6245364066285,4.77904828079251,39.992243684227));
#40290=CARTESIAN_POINT('Ctrl Pts',(19.6285232695767,4.77931490281072,39.9930304038639));
#40291=CARTESIAN_POINT('Ctrl Pts',(19.6394527850218,4.78004344960864,39.9951512451545));
#40292=CARTESIAN_POINT('Ctrl Pts',(19.6464004175966,4.7805039573514,39.9964598269787));
#40293=CARTESIAN_POINT('Ctrl Pts',(19.683379692014,4.78294192613025,40.0032145661169));
#40294=CARTESIAN_POINT('Ctrl Pts',(19.7135321584205,4.78488389977208,40.0079859888287));
#40295=CARTESIAN_POINT('Ctrl Pts',(19.9040046584549,4.79693521884287,40.0335092507176));
#40296=CARTESIAN_POINT('Ctrl Pts',(20.0663012845189,4.80629132519967,40.034758246382));
#40297=CARTESIAN_POINT('Ctrl Pts',(20.3155850214231,4.82147711394626,40.0052375149436));
#40298=CARTESIAN_POINT('Ctrl Pts',(20.4034554672686,4.82698233833473,39.9885826587018));
#40299=CARTESIAN_POINT('Ctrl Pts',(20.5028508970182,4.8335458410066,39.962488721553));
#40300=CARTESIAN_POINT('Ctrl Pts',(20.5158166831166,4.83440859713363,39.9589395894699));
#40301=CARTESIAN_POINT('Ctrl Pts',(20.5366228987346,4.83580414465906,39.9530098595545));
#40302=CARTESIAN_POINT('Ctrl Pts',(20.5444872513672,4.83633419921038,39.9507142688019));
#40303=CARTESIAN_POINT('Ctrl Pts',(20.5584732448124,4.837281531624,39.946534920405));
#40304=CARTESIAN_POINT('Ctrl Pts',(20.5646006122407,4.83769817376975,39.9446706276343));
#40305=CARTESIAN_POINT('Ctrl Pts',(20.5774003127164,4.83857193752337,39.9407064851533));
#40306=CARTESIAN_POINT('Ctrl Pts',(20.5840707243191,4.83902924403982,39.9386007920264));
#40307=CARTESIAN_POINT('Ctrl Pts',(20.6014880601843,4.84022853143058,39.9329981980774));
#40308=CARTESIAN_POINT('Ctrl Pts',(20.6122158399032,4.8409724020142,39.9294430947388));
#40309=CARTESIAN_POINT('Ctrl Pts',(20.6601016342244,4.84431664075935,39.9131057557495));
#40310=CARTESIAN_POINT('Ctrl Pts',(20.6968928428725,4.84695081894416,39.8992850338736));
#40311=CARTESIAN_POINT('Ctrl Pts',(20.8848668751928,4.86075879263345,39.8220418423178));
#40312=CARTESIAN_POINT('Ctrl Pts',(21.0279194483491,4.87253809144303,39.7406648473613));
#40313=CARTESIAN_POINT('Ctrl Pts',(21.2237036021823,4.88993102610018,39.5935383074111));
#40314=CARTESIAN_POINT('Ctrl Pts',(21.2853532811074,4.89561816039348,39.5408252320486));
#40315=CARTESIAN_POINT('Ctrl Pts',(21.3502080209599,4.90169210515697,39.4778853180082));
#40316=CARTESIAN_POINT('Ctrl Pts',(21.3568580220524,4.90231601697693,39.4713372911271));
#40317=CARTESIAN_POINT('Ctrl Pts',(21.3666711732614,4.90323800104945,39.4615333487666));
#40318=CARTESIAN_POINT('Ctrl Pts',(21.3698706523434,4.90353881316319,39.4583142318775));
#40319=CARTESIAN_POINT('Ctrl Pts',(21.3755593901868,4.90407398644391,39.4525500338436));
#40320=CARTESIAN_POINT('Ctrl Pts',(21.3780529864199,4.90430868284638,39.4500093323073));
#40321=CARTESIAN_POINT('Ctrl Pts',(21.3834307348243,4.90481506381943,39.4444995692016));
#40322=CARTESIAN_POINT('Ctrl Pts',(21.3863123623672,4.90508655433879,39.4415281302991));
#40323=CARTESIAN_POINT('Ctrl Pts',(21.3943285134723,4.90584229019585,39.4332087294934));
#40324=CARTESIAN_POINT('Ctrl Pts',(21.3994418735401,4.9063249370019,39.4278403393497));
#40325=CARTESIAN_POINT('Ctrl Pts',(21.4290270663364,4.90912179785404,39.3964188438827));
#40326=CARTESIAN_POINT('Ctrl Pts',(21.4528037903716,4.91138698408081,39.3697171795512));
#40327=CARTESIAN_POINT('Ctrl Pts',(21.5284992334853,4.91871768947291,39.2797975068625));
#40328=CARTESIAN_POINT('Ctrl Pts',(21.5771440251221,4.92362706595328,39.2139349292004));
#40329=CARTESIAN_POINT('Ctrl Pts',(21.7040033439792,4.93762555468609,39.0171284753932));
#40330=CARTESIAN_POINT('Ctrl Pts',(21.7710745324893,4.94666162442545,38.8797696853767));
#40331=CARTESIAN_POINT('Ctrl Pts',(21.828466368515,4.95769313693434,38.7154080938952));
#40332=CARTESIAN_POINT('Ctrl Pts',(21.8352936917446,4.95908303897571,38.694738082623));
#40333=CARTESIAN_POINT('Ctrl Pts',(21.844264745739,4.96102420973584,38.6659509144996));
#40334=CARTESIAN_POINT('Ctrl Pts',(21.8467076340912,4.96156577810975,38.6579281320697));
#40335=CARTESIAN_POINT('Ctrl Pts',(21.8508224571725,4.9625009188033,38.6440913381381));
#40336=CARTESIAN_POINT('Ctrl Pts',(21.8525195125849,4.96289367370031,38.6382848746909));
#40337=CARTESIAN_POINT('Ctrl Pts',(21.8559676899572,4.96370659672256,38.6262775008843));
#40338=CARTESIAN_POINT('Ctrl Pts',(21.8577151093522,4.96412687859823,38.6200756146));
#40339=CARTESIAN_POINT('Ctrl Pts',(21.8617203017572,4.96511000673922,38.6055827451913));
#40340=CARTESIAN_POINT('Ctrl Pts',(21.8639537999014,4.96567362573729,38.5972852521614));
#40341=CARTESIAN_POINT('Ctrl Pts',(21.8709776734886,4.96749706573402,38.5704791350283));
#40342=CARTESIAN_POINT('Ctrl Pts',(21.8755482414878,4.96876387709983,38.5519146164357));
#40343=CARTESIAN_POINT('Ctrl Pts',(21.8974678164881,4.97527571878104,38.4568149401438));
#40344=CARTESIAN_POINT('Ctrl Pts',(21.9104088242946,4.98065817330465,38.3793498136241));
#40345=CARTESIAN_POINT('Ctrl Pts',(21.9273014311957,4.99198917349072,38.2183621204622));
#40346=CARTESIAN_POINT('Ctrl Pts',(21.9306161324608,4.99794073320218,38.1349311393365));
#40347=CARTESIAN_POINT('Ctrl Pts',(21.9257731676811,5.0116994142719,37.942147511928));
#40348=CARTESIAN_POINT('Ctrl Pts',(21.9137194480088,5.01948543557693,37.8331603430171));
#40349=CARTESIAN_POINT('Ctrl Pts',(21.8907061079507,5.02745623692624,37.7167807508679));
#40350=CARTESIAN_POINT('Ctrl Pts',(21.8888638321568,5.02806892141685,37.7078010565084));
#40351=CARTESIAN_POINT('Ctrl Pts',(21.8860206207703,5.0289775767237,37.6944274716329));
#40352=CARTESIAN_POINT('Ctrl Pts',(21.8850682164858,5.02927617554833,37.6900235641458));
#40353=CARTESIAN_POINT('Ctrl Pts',(21.8833362569335,5.02980895967447,37.6821486447314));
#40354=CARTESIAN_POINT('Ctrl Pts',(21.882562524802,5.03004346791209,37.678676427575));
#40355=CARTESIAN_POINT('Ctrl Pts',(21.8808624579974,5.03055121418796,37.6711453597908));
#40356=CARTESIAN_POINT('Ctrl Pts',(21.8799325904454,5.03082424870648,37.6670873707968));
#40357=CARTESIAN_POINT('Ctrl Pts',(21.8772853829871,5.03158866436852,37.655704204242));
#40358=CARTESIAN_POINT('Ctrl Pts',(21.8755382930089,5.03207838698002,37.6483859177401));
#40359=CARTESIAN_POINT('Ctrl Pts',(21.8647948725178,5.03500438017196,37.6045212473273));
#40360=CARTESIAN_POINT('Ctrl Pts',(21.8547727083196,5.03738618161752,37.5682314730051));
#40361=CARTESIAN_POINT('Ctrl Pts',(21.7951628779253,5.04999507732401,37.374654458616));
#40362=CARTESIAN_POINT('Ctrl Pts',(21.7266213534196,5.05952158743345,37.2239147701008));
#40363=CARTESIAN_POINT('Ctrl Pts',(21.5982546892794,5.07433635976592,37.0167994864123));
#40364=CARTESIAN_POINT('Ctrl Pts',(21.5527245537006,5.07921281669275,36.9524872164008));
#40365=CARTESIAN_POINT('Ctrl Pts',(21.4951674091427,5.08508180599626,36.8809062997951));
#40366=CARTESIAN_POINT('Ctrl Pts',(21.4868337240754,5.08592494610814,36.8707561289538));
#40367=CARTESIAN_POINT('Ctrl Pts',(21.4731367890637,5.08730052057886,36.8544167595934));
#40368=CARTESIAN_POINT('Ctrl Pts',(21.4678365295584,5.08783041346588,36.8481751212059));
#40369=CARTESIAN_POINT('Ctrl Pts',(21.4583320402329,5.08877647267157,36.8371258957064));
#40370=CARTESIAN_POINT('Ctrl Pts',(21.4541433467099,5.08919199912621,36.8323050570223));
#40371=CARTESIAN_POINT('Ctrl Pts',(21.4452690711753,5.09006944711691,36.8221933573419));
#40372=CARTESIAN_POINT('Ctrl Pts',(21.4405782068667,5.09053158376879,36.8169072785704));
#40373=CARTESIAN_POINT('Ctrl Pts',(21.4280920831633,5.0917573746796,36.8029915983102));
#40374=CARTESIAN_POINT('Ctrl Pts',(21.4202477535029,5.09252307455564,36.7944066097323));
#40375=CARTESIAN_POINT('Ctrl Pts',(21.3832112425436,5.0961184610611,36.7546018966228));
#40376=CARTESIAN_POINT('Ctrl Pts',(21.3530663110709,5.09898851586971,36.724289105002));
#40377=CARTESIAN_POINT('Ctrl Pts',(21.2005296125092,5.11325680516196,36.5807693799915));
#40378=CARTESIAN_POINT('Ctrl Pts',(21.0648346954229,5.12526898369485,36.4827671092162));
#40379=CARTESIAN_POINT('Ctrl Pts',(20.8529616273825,5.14234243127466,36.3680893506393));
#40380=CARTESIAN_POINT('Ctrl Pts',(20.7856535134988,5.14753740641177,36.3365348787401));
#40381=CARTESIAN_POINT('Ctrl Pts',(20.7080770219719,5.15315252945747,36.305492973338));
#40382=CARTESIAN_POINT('Ctrl Pts',(20.6994431352856,5.15377239852827,36.3021101683576));
#40383=CARTESIAN_POINT('Ctrl Pts',(20.6865583914808,5.15468958591064,36.2971687201692));
#40384=CARTESIAN_POINT('Ctrl Pts',(20.6823260534746,5.15498960356391,36.295562634438));
#40385=CARTESIAN_POINT('Ctrl Pts',(20.6747561814766,5.15552391680469,36.2927204646941));
#40386=CARTESIAN_POINT('Ctrl Pts',(20.6714208535493,5.15575854321636,36.2914787086399));
#40387=CARTESIAN_POINT('Ctrl Pts',(20.6641910518689,5.15626540310884,36.2888097818465));
#40388=CARTESIAN_POINT('Ctrl Pts',(20.6602954151002,5.15653743918178,36.2873859414326));
#40389=CARTESIAN_POINT('Ctrl Pts',(20.6493873156038,5.15729623848541,36.2834389051495));
#40390=CARTESIAN_POINT('Ctrl Pts',(20.6423646856287,5.15778138212288,36.2809437303762));
#40391=CARTESIAN_POINT('Ctrl Pts',(20.600960135752,5.16062291662159,36.2665021714051));
#40392=CARTESIAN_POINT('Ctrl Pts',(20.5662575413089,5.16292843149796,36.2554891749415));
#40393=CARTESIAN_POINT('Ctrl Pts',(20.4500868132194,5.1704603187242,36.2222102143629));
#40394=CARTESIAN_POINT('Ctrl Pts',(20.3674658963873,5.17552060783291,36.2043091438547));
#40395=CARTESIAN_POINT('Ctrl Pts',(20.1368642148808,5.18945313932156,36.1699952007557));
#40396=CARTESIAN_POINT('Ctrl Pts',(19.9877791211154,5.19828839344691,36.1651887155832));
#40397=CARTESIAN_POINT('Ctrl Pts',(19.8177404989281,5.20909825597186,36.1793734285027));
#40398=CARTESIAN_POINT('Ctrl Pts',(19.7958865349046,5.21050048275683,36.1815728880997));
#40399=CARTESIAN_POINT('Ctrl Pts',(19.765716316612,5.2124561273091,36.1851306672613));
#40400=CARTESIAN_POINT('Ctrl Pts',(19.7573637124702,5.2129996512369,36.186171106377));
#40401=CARTESIAN_POINT('Ctrl Pts',(19.7430123168325,5.21393726686614,36.1880542422949));
#40402=CARTESIAN_POINT('Ctrl Pts',(19.7370101447233,5.21433053107951,36.1888705997918));
#40403=CARTESIAN_POINT('Ctrl Pts',(19.7246359191213,5.21514366437997,36.1906130198412));
#40404=CARTESIAN_POINT('Ctrl Pts',(19.7182644655896,5.2155636434842,36.1915427424207));
#40405=CARTESIAN_POINT('Ctrl Pts',(19.7034292212697,5.21654460516421,36.1937834110971));
#40406=CARTESIAN_POINT('Ctrl Pts',(19.6949693217924,5.217106350211,36.1951188509591));
#40407=CARTESIAN_POINT('Ctrl Pts',(19.6678076492659,5.2189176150415,36.1995920442451));
#40408=CARTESIAN_POINT('Ctrl Pts',(19.6491436320554,5.22017399527336,36.202949151489));
#40409=CARTESIAN_POINT('Ctrl Pts',(19.5546885209125,5.22659426539678,36.2213803976675));
#40410=CARTESIAN_POINT('Ctrl Pts',(19.47981183807,5.23189126104924,36.2407217802112));
#40411=CARTESIAN_POINT('Ctrl Pts',(19.4022328836949,5.23759496523851,36.2658148015992));
#40412=CARTESIAN_POINT('Ctrl Pts',(19.3981661044488,5.23789458476241,36.2671451706303));
#40413=CARTESIAN_POINT('Ctrl Pts',(19.3941040060237,5.23819447890751,36.2684889840944));
#40414=CARTESIAN_POINT('Origin',(20.,-1.3495818343519,38.1));
#40415=CARTESIAN_POINT('',(19.3941044301425,6.20523851046618,36.2684888437885));
#40416=CARTESIAN_POINT('',(19.3941040087491,6.0347666134114,36.2684889831928));
#40417=CARTESIAN_POINT('',(19.3941040087494,-1.3495818343519,36.2684889831927));
#40418=CARTESIAN_POINT('Ctrl Pts',(19.3941044301425,6.20523851046618,36.2684888437885));
#40419=CARTESIAN_POINT('Ctrl Pts',(19.4822432513283,6.19878335600331,36.2393309972159));
#40420=CARTESIAN_POINT('Ctrl Pts',(19.5724357244974,6.19216553628329,36.2165523121689));
#40421=CARTESIAN_POINT('Ctrl Pts',(19.7436130437267,6.17976140007284,36.1862740556517));
#40422=CARTESIAN_POINT('Ctrl Pts',(19.8240511750841,6.17399724520281,36.1772090783427));
#40423=CARTESIAN_POINT('Ctrl Pts',(19.9402921846074,6.16593451612745,36.1714672648057));
#40424=CARTESIAN_POINT('Ctrl Pts',(19.9758036483548,6.16350762489711,36.1706948235368));
#40425=CARTESIAN_POINT('Ctrl Pts',(20.0187183346558,6.16063396175617,36.1709466218819));
#40426=CARTESIAN_POINT('Ctrl Pts',(20.026117691962,6.16014061356754,36.1710326124547));
#40427=CARTESIAN_POINT('Ctrl Pts',(20.037652006817,6.15937507726548,36.1712330387734));
#40428=CARTESIAN_POINT('Ctrl Pts',(20.0417873028063,6.15910131937754,36.1713181997907));
#40429=CARTESIAN_POINT('Ctrl Pts',(20.0494816682068,6.15859329796945,36.1715014136885));
#40430=CARTESIAN_POINT('Ctrl Pts',(20.0530407063175,6.1583588534782,36.1715960182871));
#40431=CARTESIAN_POINT('Ctrl Pts',(20.0611405370733,6.15782650745258,36.171833764969));
#40432=CARTESIAN_POINT('Ctrl Pts',(20.0656810919062,6.15752895205417,36.1719830938511));
#40433=CARTESIAN_POINT('Ctrl Pts',(20.0795693041563,6.15662134580215,36.1724889658003));
#40434=CARTESIAN_POINT('Ctrl Pts',(20.0889151022645,6.15601409356413,36.172897466594));
#40435=CARTESIAN_POINT('Ctrl Pts',(20.181816670481,6.15000929031957,36.1776354396856));
#40436=CARTESIAN_POINT('Ctrl Pts',(20.2650216845902,6.14488360631636,36.1873290673491));
#40437=CARTESIAN_POINT('Ctrl Pts',(20.4534639566784,6.13333374171192,36.2218222269987));
#40438=CARTESIAN_POINT('Ctrl Pts',(20.5577667113382,6.12697587877511,36.250114066817));
#40439=CARTESIAN_POINT('Ctrl Pts',(20.7337013499291,6.11563504166003,36.3140783753764));
#40440=CARTESIAN_POINT('Ctrl Pts',(20.8064940554379,6.11074745710291,36.3457483472262));
#40441=CARTESIAN_POINT('Ctrl Pts',(20.8942502506202,6.10448479787618,36.3905472483516));
#40442=CARTESIAN_POINT('Ctrl Pts',(20.9112424539752,6.10325435372867,36.3995443644372));
#40443=CARTESIAN_POINT('Ctrl Pts',(20.9356471144982,6.101459859361,36.4129371060808));
#40444=CARTESIAN_POINT('Ctrl Pts',(20.9431694241123,6.10090292641884,36.4171309723042));
#40445=CARTESIAN_POINT('Ctrl Pts',(20.9562727041929,6.09992598348296,36.4245518123248));
#40446=CARTESIAN_POINT('Ctrl Pts',(20.9618660919218,6.09950676658568,36.4277566762275));
#40447=CARTESIAN_POINT('Ctrl Pts',(20.97267224793,6.0986925544318,36.4340204730334));
#40448=CARTESIAN_POINT('Ctrl Pts',(20.9778869171874,6.09829768551515,36.4370759903217));
#40449=CARTESIAN_POINT('Ctrl Pts',(20.99028491116,6.09735414688972,36.4444190342199));
#40450=CARTESIAN_POINT('Ctrl Pts',(20.9974548262675,6.09680467576843,36.4487288516537));
#40451=CARTESIAN_POINT('Ctrl Pts',(21.0230673571342,6.09482796197246,36.4643521581027));
#40452=CARTESIAN_POINT('Ctrl Pts',(21.041346803438,6.09339118124781,36.4759287421795));
#40453=CARTESIAN_POINT('Ctrl Pts',(21.1885466558558,6.08160266163336,36.5726589671292));
#40454=CARTESIAN_POINT('Ctrl Pts',(21.3069812570654,6.07066621435029,36.67269649903));
#40455=CARTESIAN_POINT('Ctrl Pts',(21.4668816674368,6.05391841409738,36.8445145378579));
#40456=CARTESIAN_POINT('Ctrl Pts',(21.5178484619017,6.0481979847951,36.9066336428185));
#40457=CARTESIAN_POINT('Ctrl Pts',(21.5854794326913,6.0401878291225,37.0004328849294));
#40458=CARTESIAN_POINT('Ctrl Pts',(21.6053687260439,6.0377714610864,37.029680181294));
#40459=CARTESIAN_POINT('Ctrl Pts',(21.6284304905822,6.03490853968064,37.0656831655258));
#40460=CARTESIAN_POINT('Ctrl Pts',(21.6323810986507,6.03441580686973,37.0719294139738));
#40461=CARTESIAN_POINT('Ctrl Pts',(21.6384855103003,6.03365101500111,37.0817049148649));
#40462=CARTESIAN_POINT('Ctrl Pts',(21.6406639780363,6.03337739100775,37.0852185654806));
#40463=CARTESIAN_POINT('Ctrl Pts',(21.6446976326068,6.03286948860585,37.0917713890723));
#40464=CARTESIAN_POINT('Ctrl Pts',(21.6465556829605,6.03263503002397,37.0948086660625));
#40465=CARTESIAN_POINT('Ctrl Pts',(21.6507668083596,6.03210248605153,37.1017354231787));
#40466=CARTESIAN_POINT('Ctrl Pts',(21.6531145481167,6.0318047478323,37.1056280812657));
#40467=CARTESIAN_POINT('Ctrl Pts',(21.6602587098763,6.03089602857227,37.1175686557316));
#40468=CARTESIAN_POINT('Ctrl Pts',(21.6650103716209,6.03028785615089,37.1256433913094));
#40469=CARTESIAN_POINT('Ctrl Pts',(21.7127721725587,6.02413249154624,37.2081771506125));
#40470=CARTESIAN_POINT('Ctrl Pts',(21.7508231573516,6.01887262410412,37.285408789996));
#40471=CARTESIAN_POINT('Ctrl Pts',(21.82036617698,6.00787961922313,37.4541505431114));
#40472=CARTESIAN_POINT('Ctrl Pts',(21.8503895024448,6.00217898479395,37.54600222832));
#40473=CARTESIAN_POINT('Ctrl Pts',(21.8941623185904,5.99110590989602,37.7241628826058));
#40474=CARTESIAN_POINT('Ctrl Pts',(21.9091746180942,5.98577008352513,37.8099069539371));
#40475=CARTESIAN_POINT('Ctrl Pts',(21.9204822979266,5.97896805468455,37.9164311892186));
#40476=CARTESIAN_POINT('Ctrl Pts',(21.9222973441895,5.97767752511486,37.9365294014957));
#40477=CARTESIAN_POINT('Ctrl Pts',(21.9244492596902,5.97581132781192,37.9654090669302));
#40478=CARTESIAN_POINT('Ctrl Pts',(21.9250419790922,5.97524360956797,37.9741705641129));
#40479=CARTESIAN_POINT('Ctrl Pts',(21.9259677356479,5.97425408224029,37.9893982066896));
#40480=CARTESIAN_POINT('Ctrl Pts',(21.9263280809159,5.97383312849229,37.9958625983837));
#40481=CARTESIAN_POINT('Ctrl Pts',(21.9269596492374,5.97302011059117,38.0083208515063));
#40482=CARTESIAN_POINT('Ctrl Pts',(21.9272354643227,5.97262819426452,38.0143144134008));
#40483=CARTESIAN_POINT('Ctrl Pts',(21.9278218463977,5.97169889575878,38.0284972345285));
#40484=CARTESIAN_POINT('Ctrl Pts',(21.9281081968538,5.97116076728817,38.0366873263278));
#40485=CARTESIAN_POINT('Ctrl Pts',(21.9289312386083,5.96926353659834,38.065480400967));
#40486=CARTESIAN_POINT('Ctrl Pts',(21.9291899241039,5.96789586467031,38.0860893198323));
#40487=CARTESIAN_POINT('Ctrl Pts',(21.9285399900468,5.95538031402947,38.2732858805206));
#40488=CARTESIAN_POINT('Ctrl Pts',(21.9063854731736,5.94353862930264,38.4390663180682));
#40489=CARTESIAN_POINT('Ctrl Pts',(21.8472899255557,5.92727732416627,38.659328776421));
#40490=CARTESIAN_POINT('Ctrl Pts',(21.828509872196,5.92290516627813,38.7179653710899));
#40491=CARTESIAN_POINT('Ctrl Pts',(21.7919583368256,5.9156333187595,38.8157250558177));
#40492=CARTESIAN_POINT('Ctrl Pts',(21.7756251084725,5.91269230318268,38.8553364594794));
#40493=CARTESIAN_POINT('Ctrl Pts',(21.7547764147761,5.9092992987042,38.901475521571));
#40494=CARTESIAN_POINT('Ctrl Pts',(21.7515246310143,5.90877945588525,38.9085572024044));
#40495=CARTESIAN_POINT('Ctrl Pts',(21.7464453256649,5.90798192555351,38.9194443842238));
#40496=CARTESIAN_POINT('Ctrl Pts',(21.7446481211574,5.90770245392579,38.9232638146796));
#40497=CARTESIAN_POINT('Ctrl Pts',(21.7413151072408,5.90718917043526,38.9302872260679));
#40498=CARTESIAN_POINT('Ctrl Pts',(21.7397829924394,5.90695514400767,38.9334928434621));
#40499=CARTESIAN_POINT('Ctrl Pts',(21.7363197172861,5.90643041405077,38.9406878372925));
#40500=CARTESIAN_POINT('Ctrl Pts',(21.7343836647681,5.90614001595643,38.94467479231));
#40501=CARTESIAN_POINT('Ctrl Pts',(21.7293949568701,5.90539911004154,38.954858678108));
#40502=CARTESIAN_POINT('Ctrl Pts',(21.7263226936957,5.90494978061176,38.9610460133503));
#40503=CARTESIAN_POINT('Ctrl Pts',(21.7080375700732,5.90231522966862,38.9973797637081));
#40504=CARTESIAN_POINT('Ctrl Pts',(21.6920674722899,5.90017363840033,39.0271411891221));
#40505=CARTESIAN_POINT('Ctrl Pts',(21.6049326071823,5.88919733066095,39.1797638940138));
#40506=CARTESIAN_POINT('Ctrl Pts',(21.5211403435531,5.88090984170965,39.2949222132794));
#40507=CARTESIAN_POINT('Ctrl Pts',(21.3546431338181,5.86604598799769,39.4775088090038));
#40508=CARTESIAN_POINT('Ctrl Pts',(21.2776090012152,5.85961472128681,39.5492409018788));
#40509=CARTESIAN_POINT('Ctrl Pts',(21.1836064877648,5.85196384181909,39.6234282148855));
#40510=CARTESIAN_POINT('Ctrl Pts',(21.1719856048784,5.85102143023252,39.6323862328502));
#40511=CARTESIAN_POINT('Ctrl Pts',(21.1540912960282,5.84957484812811,39.6458575395051));
#40512=CARTESIAN_POINT('Ctrl Pts',(21.1478908854923,5.84907443102439,39.6504672728417));
#40513=CARTESIAN_POINT('Ctrl Pts',(21.1365476259435,5.84816035969162,39.6587951509015));
#40514=CARTESIAN_POINT('Ctrl Pts',(21.1314137791914,5.84774718020282,39.6625254196853));
#40515=CARTESIAN_POINT('Ctrl Pts',(21.1202734470035,5.84685165847174,39.6705363293988));
#40516=CARTESIAN_POINT('Ctrl Pts',(21.1142606478879,5.84636898139062,39.6748079768821));
#40517=CARTESIAN_POINT('Ctrl Pts',(21.0978374765458,5.84505232226313,39.686334276449));
#40518=CARTESIAN_POINT('Ctrl Pts',(21.0873799348007,5.84421578333222,39.6935207641981));
#40519=CARTESIAN_POINT('Ctrl Pts',(21.0350226044427,5.84003595650712,39.728745679715));
#40520=CARTESIAN_POINT('Ctrl Pts',(20.9921092579191,5.83663591963841,39.7552349398685));
#40521=CARTESIAN_POINT('Ctrl Pts',(20.9257899008653,5.83141517878617,39.7926660815341));
#40522=CARTESIAN_POINT('Ctrl Pts',(20.9031185176103,5.829636314123,39.80487015761));
#40523=CARTESIAN_POINT('Ctrl Pts',(20.7681266099557,5.81908203876234,39.8740884677347));
#40524=CARTESIAN_POINT('Ctrl Pts',(20.6506893908832,5.8100236668565,39.9204413149286));
#40525=CARTESIAN_POINT('Ctrl Pts',(20.4765536923185,5.7971696661141,39.9701553630643));
#40526=CARTESIAN_POINT('Ctrl Pts',(20.4228898522023,5.79328772155628,39.9830160803579));
#40527=CARTESIAN_POINT('Ctrl Pts',(20.3411913455789,5.78756007788422,39.9989257549943));
#40528=CARTESIAN_POINT('Ctrl Pts',(20.3135219233485,5.78565141581237,40.0036897765092));
#40529=CARTESIAN_POINT('Ctrl Pts',(20.2789485652591,5.78331309348411,40.0088681580263));
#40530=CARTESIAN_POINT('Ctrl Pts',(20.2721349393605,5.78285450632853,40.009851440584));
#40531=CARTESIAN_POINT('Ctrl Pts',(20.2613316498728,5.78213110273757,40.0113514871298));
#40532=CARTESIAN_POINT('Ctrl Pts',(20.2573454636272,5.78186498003601,40.01189226989));
#40533=CARTESIAN_POINT('Ctrl Pts',(20.2498086164001,5.78136335539612,40.0128907517678));
#40534=CARTESIAN_POINT('Ctrl Pts',(20.2462584160669,5.78112771890116,40.0133510304608));
#40535=CARTESIAN_POINT('Ctrl Pts',(20.2380978357383,5.78058754836809,40.0143859491658));
#40536=CARTESIAN_POINT('Ctrl Pts',(20.2334866464242,5.78028339492254,40.0149538189731));
#40537=CARTESIAN_POINT('Ctrl Pts',(20.221144423303,5.77947206595061,40.016428524816));
#40538=CARTESIAN_POINT('Ctrl Pts',(20.2134097790597,5.77896651795911,40.017305248996));
#40539=CARTESIAN_POINT('Ctrl Pts',(20.1549888239815,5.77516845213332,40.0235693701652));
#40540=CARTESIAN_POINT('Ctrl Pts',(20.1041071307877,5.7719762708601,40.0269933563339));
#40541=CARTESIAN_POINT('Ctrl Pts',(20.0287861529177,5.76734349246639,40.0290691299038));
#40542=CARTESIAN_POINT('Ctrl Pts',(20.0044162800825,5.76585889800198,40.0292788586491));
#40543=CARTESIAN_POINT('Ctrl Pts',(19.8132179178463,5.75428047380752,40.0273013180944));
#40544=CARTESIAN_POINT('Ctrl Pts',(19.6473241436326,5.74457853297607,40.0039428669454));
#40545=CARTESIAN_POINT('Ctrl Pts',(19.4454861020688,5.73154157048244,39.9482065493981));
#40546=CARTESIAN_POINT('Ctrl Pts',(19.4048592104452,5.7288561049549,39.9355272067644));
#40547=CARTESIAN_POINT('Ctrl Pts',(19.3537229976297,5.7253820757576,39.9176917848358));
#40548=CARTESIAN_POINT('Ctrl Pts',(19.3427939927123,5.72463406497428,39.9137689055848));
#40549=CARTESIAN_POINT('Ctrl Pts',(19.3252748708879,5.72342579793691,39.9073014275896));
#40550=CARTESIAN_POINT('Ctrl Pts',(19.3186620421644,5.7229675953757,39.9048188371798));
#40551=CARTESIAN_POINT('Ctrl Pts',(19.3060957229741,5.72209275132529,39.900022280003));
#40552=CARTESIAN_POINT('Ctrl Pts',(19.3001397870552,5.72167633523702,39.8977149481714));
#40553=CARTESIAN_POINT('Ctrl Pts',(19.2865680407102,5.72072333692431,39.8923795818158));
#40554=CARTESIAN_POINT('Ctrl Pts',(19.2789598892179,5.72018612509789,39.8893325238756));
#40555=CARTESIAN_POINT('Ctrl Pts',(19.2591892385596,5.71878223835577,39.8812678275729));
#40556=CARTESIAN_POINT('Ctrl Pts',(19.2470584126493,5.71791302719372,39.8761741494971));
#40557=CARTESIAN_POINT('Ctrl Pts',(19.1619696801723,5.71175980833699,39.839417463353));
#40558=CARTESIAN_POINT('Ctrl Pts',(19.0909886049048,5.70632837801804,39.8033975502764));
#40559=CARTESIAN_POINT('Ctrl Pts',(18.9192101207218,5.69242054684472,39.7024275326795));
#40560=CARTESIAN_POINT('Ctrl Pts',(18.821858723836,5.68381081135653,39.6322728083569));
#40561=CARTESIAN_POINT('Ctrl Pts',(18.6902151316299,5.6714103984125,39.5174025295035));
#40562=CARTESIAN_POINT('Ctrl Pts',(18.6503438718174,5.66754044564485,39.4794910454738));
#40563=CARTESIAN_POINT('Ctrl Pts',(18.5926847037875,5.66182821534024,39.4197693562484));
#40564=CARTESIAN_POINT('Ctrl Pts',(18.5736650592451,5.65992333859906,39.3991906467642));
#40565=CARTESIAN_POINT('Ctrl Pts',(18.5505409397331,5.65758897922564,39.3730507922824));
#40566=CARTESIAN_POINT('Ctrl Pts',(18.546010099586,5.6571306841945,39.3678735189847));
#40567=CARTESIAN_POINT('Ctrl Pts',(18.5388746590869,5.65640763530124,39.3596314814215));
#40568=CARTESIAN_POINT('Ctrl Pts',(18.5362518332966,5.65614157730287,39.3565826817423));
#40569=CARTESIAN_POINT('Ctrl Pts',(18.5313121681438,5.65564000302225,39.3508043121125));
#40570=CARTESIAN_POINT('Ctrl Pts',(18.5289934211186,5.65540435258617,39.3480765280027));
#40571=CARTESIAN_POINT('Ctrl Pts',(18.5236819557448,5.65486405794854,39.3417927321904));
#40572=CARTESIAN_POINT('Ctrl Pts',(18.5206944845256,5.65455979494514,39.3382323491632));
#40573=CARTESIAN_POINT('Ctrl Pts',(18.5127343523278,5.6537479804716,39.328675762971));
#40574=CARTESIAN_POINT('Ctrl Pts',(18.5077850307439,5.65324205959919,39.3226601031099));
#40575=CARTESIAN_POINT('Ctrl Pts',(18.4706293960813,5.64943368896291,39.276937539467));
#40576=CARTESIAN_POINT('Ctrl Pts',(18.4399733439583,5.64623218931489,39.235990444263));
#40577=CARTESIAN_POINT('Ctrl Pts',(18.3341684526893,5.63476097894051,39.0822917690576));
#40578=CARTESIAN_POINT('Ctrl Pts',(18.2693209693156,5.62684882176493,38.9629290559913));
#40579=CARTESIAN_POINT('Ctrl Pts',(18.1937665496239,5.61491080162595,38.780381034055));
#40580=CARTESIAN_POINT('Ctrl Pts',(18.1728071869465,5.61111319388683,38.7219028036021));
#40581=CARTESIAN_POINT('Ctrl Pts',(18.1439119645423,5.60491643761425,38.627114534684));
#40582=CARTESIAN_POINT('Ctrl Pts',(18.1341410058778,5.60257352010517,38.5914086447976));
#40583=CARTESIAN_POINT('Ctrl Pts',(18.122790506048,5.59948706945885,38.5446904249656));
#40584=CARTESIAN_POINT('Ctrl Pts',(18.12027012231,5.59877365446295,38.5339131674132));
#40585=CARTESIAN_POINT('Ctrl Pts',(18.1163197655994,5.59760787276709,38.5163406565997));
#40586=CARTESIAN_POINT('Ctrl Pts',(18.1148334735088,5.59715730340966,38.5095582170079));
#40587=CARTESIAN_POINT('Ctrl Pts',(18.1120433268395,5.59628783481803,38.4964888169572));
#40588=CARTESIAN_POINT('Ctrl Pts',(18.1107341787303,5.5958691100482,38.4902030710009));
#40589=CARTESIAN_POINT('Ctrl Pts',(18.1078044650007,5.59490672312035,38.4757758942859));
#40590=CARTESIAN_POINT('Ctrl Pts',(18.1062050302295,5.59436239979195,38.4676303499996));
#40591=CARTESIAN_POINT('Ctrl Pts',(18.1020844522911,5.59290789353568,38.4459044806841));
#40592=CARTESIAN_POINT('Ctrl Pts',(18.0996565416603,5.59199479235371,38.4323071764955));
#40593=CARTESIAN_POINT('Ctrl Pts',(18.0796387155648,5.58394337882969,38.3127961029939));
#40594=CARTESIAN_POINT('Ctrl Pts',(18.070776073483,5.57652955287812,38.205629665528));
#40595=CARTESIAN_POINT('Ctrl Pts',(18.070936804357,5.56365420413341,38.0234158365994));
#40596=CARTESIAN_POINT('Ctrl Pts',(18.0753628644005,5.55829502373828,37.9486024083819));
#40597=CARTESIAN_POINT('Ctrl Pts',(18.0951992911711,5.54622044985506,37.780265021749));
#40598=CARTESIAN_POINT('Ctrl Pts',(18.1131734656301,5.53953413727261,37.6872212455289));
#40599=CARTESIAN_POINT('Ctrl Pts',(18.1403561849151,5.53254281768199,37.5868185160983));
#40600=CARTESIAN_POINT('Ctrl Pts',(18.1428707668839,5.53191635532452,37.5777918282836));
#40601=CARTESIAN_POINT('Ctrl Pts',(18.1467029012921,5.53099134614687,37.5644133243045));
#40602=CARTESIAN_POINT('Ctrl Pts',(18.1479701815966,5.53069003376427,37.5600474316597));
#40603=CARTESIAN_POINT('Ctrl Pts',(18.1502575293761,5.53015431696555,37.5522701150643));
#40604=CARTESIAN_POINT('Ctrl Pts',(18.1512716169498,5.5299195745406,37.5488570050266));
#40605=CARTESIAN_POINT('Ctrl Pts',(18.1534835300465,5.52941348695002,37.5414871777931));
#40606=CARTESIAN_POINT('Ctrl Pts',(18.1546846230418,5.52914233375021,37.5375315060078));
#40607=CARTESIAN_POINT('Ctrl Pts',(18.1580681568925,5.52838849234725,37.5265156934679));
#40608=CARTESIAN_POINT('Ctrl Pts',(18.1602784912671,5.52790738970793,37.5194640931869));
#40609=CARTESIAN_POINT('Ctrl Pts',(18.1732950888228,5.52513770503684,37.4787584376956));
#40610=CARTESIAN_POINT('Ctrl Pts',(18.184984928231,5.52289704418227,37.4453912751023));
#40611=CARTESIAN_POINT('Ctrl Pts',(18.2261779439051,5.51568656916191,37.3374175431053));
#40612=CARTESIAN_POINT('Ctrl Pts',(18.2594188211567,5.51086710659127,37.2643230285115));
#40613=CARTESIAN_POINT('Ctrl Pts',(18.3697477118434,5.49682607433729,37.0570661953431));
#40614=CARTESIAN_POINT('Ctrl Pts',(18.4585019598398,5.48766852923149,36.9298671068564));
#40615=CARTESIAN_POINT('Ctrl Pts',(18.5758871927758,5.47650353778058,36.7984958442563));
#40616=CARTESIAN_POINT('Ctrl Pts',(18.5905680500564,5.47512237199681,36.7826117224649));
#40617=CARTESIAN_POINT('Ctrl Pts',(18.6112921514894,5.47319148273305,36.7609320290025));
#40618=CARTESIAN_POINT('Ctrl Pts',(18.6171110815387,5.47265132370543,36.7549235133055));
#40619=CARTESIAN_POINT('Ctrl Pts',(18.6272014253716,5.47171796469598,36.7446391049315));
#40620=CARTESIAN_POINT('Ctrl Pts',(18.6314542309351,5.47132557490013,36.7403450588554));
#40621=CARTESIAN_POINT('Ctrl Pts',(18.6402850262368,5.47051279412684,36.7315120362935));
#40622=CARTESIAN_POINT('Ctrl Pts',(18.6448657255471,5.47009228668394,36.7269758876113));
#40623=CARTESIAN_POINT('Ctrl Pts',(18.6556197289896,5.46910756455982,36.7164327131544));
#40624=CARTESIAN_POINT('Ctrl Pts',(18.6618106603213,5.46854256960355,36.7104439423232));
#40625=CARTESIAN_POINT('Ctrl Pts',(18.6819542025523,5.46671016060605,36.6912176400474));
#40626=CARTESIAN_POINT('Ctrl Pts',(18.6960643609658,5.46543565969649,36.6781475935093));
#40627=CARTESIAN_POINT('Ctrl Pts',(18.7693934869399,5.45885587924319,36.6122334220224));
#40628=CARTESIAN_POINT('Ctrl Pts',(18.8316300572949,5.4534099229347,36.562875885249));
#40629=CARTESIAN_POINT('Ctrl Pts',(18.9853373531442,5.44028725917251,36.4557154231495));
#40630=CARTESIAN_POINT('Ctrl Pts',(19.0789820055309,5.4325315878804,36.4014902797712));
#40631=CARTESIAN_POINT('Ctrl Pts',(19.2473134335991,5.4193034660997,36.3220493428573));
#40632=CARTESIAN_POINT('Ctrl Pts',(19.3199273763348,5.4138095667175,36.2930279150429));
#40633=CARTESIAN_POINT('Ctrl Pts',(19.3941040111825,5.40852741588127,36.2684889823878));
#40634=CARTESIAN_POINT('',(18.0708696352982,5.3988988782065,38.1006192288316));
#40635=CARTESIAN_POINT('Ctrl Pts',(19.3941040060237,5.23819447890751,36.2684889840944));
#40636=CARTESIAN_POINT('Ctrl Pts',(19.3180587870711,5.24380869932756,36.2936460774039));
#40637=CARTESIAN_POINT('Ctrl Pts',(19.2436543448456,5.24952393634133,36.3235148555594));
#40638=CARTESIAN_POINT('Ctrl Pts',(19.0720726325909,5.26308032836566,36.4051333609403));
#40639=CARTESIAN_POINT('Ctrl Pts',(18.9770259977916,5.27090122199522,36.4607464563682));
#40640=CARTESIAN_POINT('Ctrl Pts',(18.8797410055104,5.278903014203,36.5294439590056));
#40641=CARTESIAN_POINT('Ctrl Pts',(18.8722947274666,5.27951537793363,36.5347820218623));
#40642=CARTESIAN_POINT('Ctrl Pts',(18.8612442407492,5.28042365209288,36.5428236548198));
#40643=CARTESIAN_POINT('Ctrl Pts',(18.857611147912,5.28072218736542,36.5454870341925));
#40644=CARTESIAN_POINT('Ctrl Pts',(18.8512123172242,5.28124779628259,36.550212492777));
#40645=CARTESIAN_POINT('Ctrl Pts',(18.8484427580593,5.28147522588062,36.5522692815515));
#40646=CARTESIAN_POINT('Ctrl Pts',(18.845664805945,5.28170327521311,36.55434388787));
#40647=CARTESIAN_POINT('Ctrl Pts',(18.8456509506368,5.28170441262985,36.5543542354623));
#40648=CARTESIAN_POINT('Ctrl Pts',(18.845623427101,5.28170667210218,36.5543747915057));
#40649=CARTESIAN_POINT('Ctrl Pts',(18.8456097587989,5.28170779416393,36.5543850000047));
#40650=CARTESIAN_POINT('Ctrl Pts',(18.8455826057029,5.28171002321967,36.5544052805061));
#40651=CARTESIAN_POINT('Ctrl Pts',(18.8455691208838,5.28171113021578,36.5544153525199));
#40652=CARTESIAN_POINT('Ctrl Pts',(18.8455423305775,5.28171332948321,36.5544353631481));
#40653=CARTESIAN_POINT('Ctrl Pts',(18.84552902539,5.28171442172997,36.5544453015313));
#40654=CARTESIAN_POINT('Ctrl Pts',(18.8455025920378,5.2817165916884,36.5544650466013));
#40655=CARTESIAN_POINT('Ctrl Pts',(18.845489463514,5.28171766942958,36.5544748535494));
#40656=CARTESIAN_POINT('Ctrl Pts',(18.8454633789171,5.28171981075229,36.5544943391433));
#40657=CARTESIAN_POINT('Ctrl Pts',(18.8454504232254,5.28172087430256,36.5545040174976));
#40658=CARTESIAN_POINT('Ctrl Pts',(18.8454246820194,5.28172298743017,36.5545232475819));
#40659=CARTESIAN_POINT('Ctrl Pts',(18.8454118961795,5.28172403703428,36.5545327995487));
#40660=CARTESIAN_POINT('Ctrl Pts',(18.8453864913349,5.28172612254409,36.5545517793351));
#40661=CARTESIAN_POINT('Ctrl Pts',(18.8453738721528,5.28172715846437,36.554561207281));
#40662=CARTESIAN_POINT('Ctrl Pts',(18.8453487973774,5.28172921687311,36.5545799414322));
#40663=CARTESIAN_POINT('Ctrl Pts',(18.8453363417272,5.28173023936627,36.5545892476736));
#40664=CARTESIAN_POINT('Ctrl Pts',(18.8453115910356,5.28173227116552,36.5546077406242));
#40665=CARTESIAN_POINT('Ctrl Pts',(18.8452992959989,5.28173328047124,36.5546169273236));
#40666=CARTESIAN_POINT('Ctrl Pts',(18.8420006721966,5.28200406581114,36.5570816795884));
#40667=CARTESIAN_POINT('Ctrl Pts',(18.8387221471511,5.28227311036255,36.5595477495515));
#40668=CARTESIAN_POINT('Ctrl Pts',(18.8319311333881,5.28283026786957,36.5646898756521));
#40669=CARTESIAN_POINT('Ctrl Pts',(18.8284199111907,5.28311826687096,36.5673675745606));
#40670=CARTESIAN_POINT('Ctrl Pts',(18.8194628901142,5.28385284418345,36.5742470711878));
#40671=CARTESIAN_POINT('Ctrl Pts',(18.8140302584486,5.28429828707388,36.5784660230361));
#40672=CARTESIAN_POINT('Ctrl Pts',(18.798297929349,5.28558834868718,36.5908191186834));
#40673=CARTESIAN_POINT('Ctrl Pts',(18.7880583086152,5.28642813795777,36.5990295949475));
#40674=CARTESIAN_POINT('Ctrl Pts',(18.7526196625938,5.28933823752594,36.6280446321233));
#40675=CARTESIAN_POINT('Ctrl Pts',(18.7278648618391,5.29137757418001,36.6493853872163));
#40676=CARTESIAN_POINT('Ctrl Pts',(18.5880166134659,5.30301704850862,36.7762813920258));
#40677=CARTESIAN_POINT('Ctrl Pts',(18.4855340531755,5.31207123245999,36.8948743762722));
#40678=CARTESIAN_POINT('Ctrl Pts',(18.3776507371344,5.32385523265671,37.0555291130434));
#40679=CARTESIAN_POINT('Ctrl Pts',(18.3577412832574,5.3261494613199,37.0871216027717));
#40680=CARTESIAN_POINT('Ctrl Pts',(18.317133253641,5.33111965503504,37.1559067487322));
#40681=CARTESIAN_POINT('Ctrl Pts',(18.2967239919146,5.33380288792504,37.1932459157702));
#40682=CARTESIAN_POINT('Ctrl Pts',(18.2721130645705,5.33730601563086,37.2420396577662));
#40683=CARTESIAN_POINT('Ctrl Pts',(18.2667614041317,5.33808572160354,37.2529030932484));
#40684=CARTESIAN_POINT('Ctrl Pts',(18.2584030466508,5.33933293788077,37.2702807280347));
#40685=CARTESIAN_POINT('Ctrl Pts',(18.2553297364744,5.33979814769447,37.2767626785326));
#40686=CARTESIAN_POINT('Ctrl Pts',(18.249866856376,5.34063717813907,37.2884524863122));
#40687=CARTESIAN_POINT('Ctrl Pts',(18.2474641884693,5.34101054424518,37.2936541588725));
#40688=CARTESIAN_POINT('Ctrl Pts',(18.2418856455968,5.34188775818746,37.3058741807215));
#40689=CARTESIAN_POINT('Ctrl Pts',(18.2387285838179,5.34239224043633,37.3129009619827));
#40690=CARTESIAN_POINT('Ctrl Pts',(18.2297248228618,5.34385465559077,37.3332663724761));
#40691=CARTESIAN_POINT('Ctrl Pts',(18.2239870805046,5.34481625270566,37.3466523057182));
#40692=CARTESIAN_POINT('Ctrl Pts',(18.179837001073,5.35245761640374,37.4529611091737));
#40693=CARTESIAN_POINT('Ctrl Pts',(18.1485976195904,5.35937720480023,37.5486779431821));
#40694=CARTESIAN_POINT('Ctrl Pts',(18.0889769732398,5.37723970142802,37.7951195524543));
#40695=CARTESIAN_POINT('Ctrl Pts',(18.0708211705784,5.38836245992606,37.94760092491));
#40696=CARTESIAN_POINT('Ctrl Pts',(18.070870098622,5.39889951889677,38.1006168544168));
#40697=CARTESIAN_POINT('Ctrl Pts',(18.070870099365,5.39889967859844,38.1006191735561));
#40698=CARTESIAN_POINT('Ctrl Pts',(18.0708758483007,5.40013312137755,38.1185308618298));
#40699=CARTESIAN_POINT('Ctrl Pts',(18.0711310585434,5.40135730436667,38.1364424185093));
#40700=CARTESIAN_POINT('Ctrl Pts',(18.0719614696151,5.40335315052469,38.1659065598357));
#40701=CARTESIAN_POINT('Ctrl Pts',(18.0723911311066,5.40413133583061,38.1774616899035));
#40702=CARTESIAN_POINT('Ctrl Pts',(18.0731479842833,5.40522773943072,38.1938471596201));
#40703=CARTESIAN_POINT('Ctrl Pts',(18.0733894908621,5.40555030754759,38.1986809360689));
#40704=CARTESIAN_POINT('Ctrl Pts',(18.0738420528639,5.40611074099713,38.2071029344015));
#40705=CARTESIAN_POINT('Ctrl Pts',(18.0740449489794,5.40634903990194,38.2106915436682));
#40706=CARTESIAN_POINT('Ctrl Pts',(18.0744579567,5.40681019046718,38.2176511966592));
#40707=CARTESIAN_POINT('Ctrl Pts',(18.074666894603,5.40703310640091,38.2210223059762));
#40708=CARTESIAN_POINT('Ctrl Pts',(18.075102271927,5.40747772334534,38.2277602428641));
#40709=CARTESIAN_POINT('Ctrl Pts',(18.0753286918662,5.40769942559883,38.2311270348945));
#40710=CARTESIAN_POINT('Ctrl Pts',(18.0759570893528,5.40829032588631,38.2401186445076));
#40711=CARTESIAN_POINT('Ctrl Pts',(18.0763749018921,5.40865865077766,38.245742376939));
#40712=CARTESIAN_POINT('Ctrl Pts',(18.0779785913214,5.40998890025745,38.2661183044184));
#40713=CARTESIAN_POINT('Ctrl Pts',(18.079309594352,5.41094314272288,38.2808590177023));
#40714=CARTESIAN_POINT('Ctrl Pts',(18.0834634488418,5.41356290889723,38.3216192853597));
#40715=CARTESIAN_POINT('Ctrl Pts',(18.0866464121309,5.41521142985344,38.3475997807835));
#40716=CARTESIAN_POINT('Ctrl Pts',(18.1123867324077,5.42651647163107,38.5273191130625));
#40717=CARTESIAN_POINT('Ctrl Pts',(18.152919352461,5.43552899386554,38.6779169439124));
#40718=CARTESIAN_POINT('Ctrl Pts',(18.2444468565024,5.45033123750452,38.9046866070681));
#40719=CARTESIAN_POINT('Ctrl Pts',(18.2834916888199,5.45582869757392,38.9849200305202));
#40720=CARTESIAN_POINT('Ctrl Pts',(18.3350382802463,5.46243534677084,39.0744986678629));
#40721=CARTESIAN_POINT('Ctrl Pts',(18.3422740423502,5.46334997999109,39.0867572212886));
#40722=CARTESIAN_POINT('Ctrl Pts',(18.3535977412813,5.46476264200826,39.1054652852563));
#40723=CARTESIAN_POINT('Ctrl Pts',(18.35758951867,5.46525718787271,39.1119726505313));
#40724=CARTESIAN_POINT('Ctrl Pts',(18.3649365830653,5.46616130031312,39.1237918004788));
#40725=CARTESIAN_POINT('Ctrl Pts',(18.3682794093943,5.46657040710039,39.1291112382836));
#40726=CARTESIAN_POINT('Ctrl Pts',(18.3756329817706,5.46746553320255,39.1406870686856));
#40727=CARTESIAN_POINT('Ctrl Pts',(18.3796540020045,5.46795192668774,39.1469367836803));
#40728=CARTESIAN_POINT('Ctrl Pts',(18.3907711961082,5.46928844498812,39.1639983383249));
#40729=CARTESIAN_POINT('Ctrl Pts',(18.3979400344247,5.47014125668199,39.1747621412021));
#40730=CARTESIAN_POINT('Ctrl Pts',(18.4353772815578,5.4745498315613,39.2297661961875));
#40731=CARTESIAN_POINT('Ctrl Pts',(18.4673692106458,5.47817010583034,39.272799139087));
#40732=CARTESIAN_POINT('Ctrl Pts',(18.5134914169344,5.48320397748046,39.3297242363422));
#40733=CARTESIAN_POINT('Ctrl Pts',(18.5261068954014,5.48456341285575,39.3448166691896));
#40734=CARTESIAN_POINT('Ctrl Pts',(18.6261196246063,5.4952053052101,39.4608141361822));
#40735=CARTESIAN_POINT('Ctrl Pts',(18.7235428738316,5.50482058275442,39.5525885494307));
#40736=CARTESIAN_POINT('Ctrl Pts',(18.8705854940537,5.5179285444647,39.6648060545403));
#40737=CARTESIAN_POINT('Ctrl Pts',(18.9127656915284,5.52154545008529,39.6944019052689));
#40738=CARTESIAN_POINT('Ctrl Pts',(18.9710987046413,5.52631309463113,39.7319385803451));
#40739=CARTESIAN_POINT('Ctrl Pts',(18.9862487934323,5.52753091123424,39.7413926853754));
#40740=CARTESIAN_POINT('Ctrl Pts',(19.0088560514611,5.52931580059844,39.7550678441187));
#40741=CARTESIAN_POINT('Ctrl Pts',(19.0162131404572,5.52989166956653,39.7594515108055));
#40742=CARTESIAN_POINT('Ctrl Pts',(19.0295865114951,5.53092912644573,39.7672997360742));
#40743=CARTESIAN_POINT('Ctrl Pts',(19.0355927230888,5.53139169342091,39.7707810617926));
#40744=CARTESIAN_POINT('Ctrl Pts',(19.0450865995588,5.53211740654303,39.7762156576));
#40745=CARTESIAN_POINT('Ctrl Pts',(19.0485616931984,5.53238189901771,39.7781905976965));
#40746=CARTESIAN_POINT('Ctrl Pts',(19.0520533045682,5.53264648385942,39.7801605934141));
#40747=CARTESIAN_POINT('Ctrl Pts',(19.0520636696433,5.53264726928643,39.7801664413479));
#40748=CARTESIAN_POINT('Ctrl Pts',(19.0520844520583,5.53264884408027,39.7801781664495));
#40749=CARTESIAN_POINT('Ctrl Pts',(19.0520948692226,5.53264963343369,39.780184043517));
#40750=CARTESIAN_POINT('Ctrl Pts',(19.0521157551074,5.53265121602636,39.7801958264824));
#40751=CARTESIAN_POINT('Ctrl Pts',(19.0521262249653,5.53265200935169,39.7802017330208));
#40752=CARTESIAN_POINT('Ctrl Pts',(19.0521483760127,5.53265368776555,39.7802142291936));
#40753=CARTESIAN_POINT('Ctrl Pts',(19.0521600563483,5.53265457278681,39.7802208183147));
#40754=CARTESIAN_POINT('Ctrl Pts',(19.0521836722353,5.53265636214071,39.780234140205));
#40755=CARTESIAN_POINT('Ctrl Pts',(19.0521956085007,5.53265726652686,39.7802408733698));
#40756=CARTESIAN_POINT('Ctrl Pts',(19.0550720166701,5.53287520274175,39.7818633949258));
#40757=CARTESIAN_POINT('Ctrl Pts',(19.0579405781833,5.53309175577294,39.7834718348901));
#40758=CARTESIAN_POINT('Ctrl Pts',(19.0647331726977,5.53360269576753,39.7872577328871));
#40759=CARTESIAN_POINT('Ctrl Pts',(19.0686606989361,5.53389667753351,39.7894288392055));
#40760=CARTESIAN_POINT('Ctrl Pts',(19.0805543489085,5.53478268062025,39.7959494767319));
#40761=CARTESIAN_POINT('Ctrl Pts',(19.0885437654327,5.53537209393245,39.8002565904101));
#40762=CARTESIAN_POINT('Ctrl Pts',(19.1530609736911,5.54008815712808,39.8344525155766));
#40763=CARTESIAN_POINT('Ctrl Pts',(19.2110191533079,5.54405698001466,39.8615738287022));
#40764=CARTESIAN_POINT('Ctrl Pts',(19.3813399937013,5.55526541653116,39.9311775281476));
#40765=CARTESIAN_POINT('Ctrl Pts',(19.4964545312734,5.56231026438453,39.9661177640241));
#40766=CARTESIAN_POINT('Ctrl Pts',(19.6761381419853,5.5733835185158,40.0028054669264));
#40767=CARTESIAN_POINT('Ctrl Pts',(19.7387845514535,5.57725465579278,40.0124122560933));
#40768=CARTESIAN_POINT('Ctrl Pts',(19.8391194556964,5.58355970276966,40.0227762821035));
#40769=CARTESIAN_POINT('Ctrl Pts',(19.8765548817508,5.58593477002806,40.0255420498551));
#40770=CARTESIAN_POINT('Ctrl Pts',(19.9251565513025,5.58905773563377,40.0277097086844));
#40771=CARTESIAN_POINT('Ctrl Pts',(19.9362717033187,5.58977460568774,40.0281091666567));
#40772=CARTESIAN_POINT('Ctrl Pts',(19.9543422733671,5.5909446265755,40.0286021637212));
#40773=CARTESIAN_POINT('Ctrl Pts',(19.9612959432389,5.59139595506338,40.028754242459));
#40774=CARTESIAN_POINT('Ctrl Pts',(19.9746660451756,5.59226591657799,40.0289743185801));
#40775=CARTESIAN_POINT('Ctrl Pts',(19.9810823026998,5.59268436990603,40.0290479128508));
#40776=CARTESIAN_POINT('Ctrl Pts',(19.9957735647982,5.59364475790508,40.029143117989));
#40777=CARTESIAN_POINT('Ctrl Pts',(20.0040485345194,5.59418734454889,40.0291434986057));
#40778=CARTESIAN_POINT('Ctrl Pts',(20.0260459265559,5.59563418678428,40.029002977985));
#40779=CARTESIAN_POINT('Ctrl Pts',(20.0397670742948,5.59654131220904,40.0287688930256));
#40780=CARTESIAN_POINT('Ctrl Pts',(20.1550606952596,5.60420392711273,40.0255711999786));
#40781=CARTESIAN_POINT('Ctrl Pts',(20.2562387416506,5.61120490286912,40.0147333841997));
#40782=CARTESIAN_POINT('Ctrl Pts',(20.4436840943488,5.62465253914239,39.9795298158322));
#40783=CARTESIAN_POINT('Ctrl Pts',(20.5300414479743,5.6310433905727,39.9570252858446));
#40784=CARTESIAN_POINT('Ctrl Pts',(20.6895375932326,5.64300963546121,39.9034251217219));
#40785=CARTESIAN_POINT('Ctrl Pts',(20.7629327994287,5.64858338844913,39.8736235593879));
#40786=CARTESIAN_POINT('Ctrl Pts',(20.8472400956338,5.65491695871823,39.8331857540802));
#40787=CARTESIAN_POINT('Ctrl Pts',(20.8601144796393,5.65588207762976,39.8268328667703));
#40788=CARTESIAN_POINT('Ctrl Pts',(20.8777320072592,5.65719870596666,39.8178935448074));
#40789=CARTESIAN_POINT('Ctrl Pts',(20.8825366028216,5.6575573530647,39.8154302242512));
#40790=CARTESIAN_POINT('Ctrl Pts',(20.8906134889532,5.65815947805892,39.8112462819061));
#40791=CARTESIAN_POINT('Ctrl Pts',(20.8938912620062,5.65840361349351,39.8095363805677));
#40792=CARTESIAN_POINT('Ctrl Pts',(20.9001073469168,5.65886615405571,39.8062708969972));
#40793=CARTESIAN_POINT('Ctrl Pts',(20.9030465758143,5.65908467367462,39.8047171296851));
#40794=CARTESIAN_POINT('Ctrl Pts',(20.9107280252094,5.65965530092272,39.8006310363675));
#40795=CARTESIAN_POINT('Ctrl Pts',(20.9154637449066,5.66000664326744,39.7980864498669));
#40796=CARTESIAN_POINT('Ctrl Pts',(20.9317864223115,5.66121625382766,39.7892278535447));
#40797=CARTESIAN_POINT('Ctrl Pts',(20.9433195096781,5.66206853811522,39.7828146076584));
#40798=CARTESIAN_POINT('Ctrl Pts',(21.0795538457874,5.67211860184255,39.7052175383931));
#40799=CARTESIAN_POINT('Ctrl Pts',(21.196017600816,5.68055720790592,39.6204324714698));
#40800=CARTESIAN_POINT('Ctrl Pts',(21.3964109581428,5.69680120294204,39.4371417801357));
#40801=CARTESIAN_POINT('Ctrl Pts',(21.4819803115996,5.70453913883986,39.3416277133483));
#40802=CARTESIAN_POINT('Ctrl Pts',(21.5663455485792,5.7136693137624,39.2262019470784));
#40803=CARTESIAN_POINT('Ctrl Pts',(21.5750863987229,5.71463594782367,39.2139443518821));
#40804=CARTESIAN_POINT('Ctrl Pts',(21.5881399291552,5.71611205694871,39.1951780906876));
#40805=CARTESIAN_POINT('Ctrl Pts',(21.5925581750365,5.71661753508635,39.1887432852019));
#40806=CARTESIAN_POINT('Ctrl Pts',(21.6004998562707,5.71753692526343,39.1770251127813));
#40807=CARTESIAN_POINT('Ctrl Pts',(21.6040365039909,5.71795033412957,39.1717507992725));
#40808=CARTESIAN_POINT('Ctrl Pts',(21.6115896604104,5.71884192049574,39.160365408868));
#40809=CARTESIAN_POINT('Ctrl Pts',(21.6155975802933,5.71932040924536,39.1542487799098));
#40810=CARTESIAN_POINT('Ctrl Pts',(21.6263159373185,5.72061477769129,39.1376864509129));
#40811=CARTESIAN_POINT('Ctrl Pts',(21.6329603796871,5.72143307177949,39.1271986587672));
#40812=CARTESIAN_POINT('Ctrl Pts',(21.6644309550074,5.72538709054735,39.0764474454335));
#40813=CARTESIAN_POINT('Ctrl Pts',(21.6878699205483,5.72857247786237,39.0353472563209));
#40814=CARTESIAN_POINT('Ctrl Pts',(21.7242511987213,5.73394578996075,38.965723751978));
#40815=CARTESIAN_POINT('Ctrl Pts',(21.738052750229,5.73610481513327,38.9376707474733));
#40816=CARTESIAN_POINT('Ctrl Pts',(21.8217739162041,5.75000267504645,38.7565137052161));
#40817=CARTESIAN_POINT('Ctrl Pts',(21.8720766019104,5.76226643378934,38.5951681773285));
#40818=CARTESIAN_POINT('Ctrl Pts',(21.9072842820847,5.77658140775331,38.3919734362554));
#40819=CARTESIAN_POINT('Ctrl Pts',(21.9126577120263,5.77917832794206,38.3544066993405));
#40820=CARTESIAN_POINT('Ctrl Pts',(21.9177670640176,5.78222489540596,38.309210193155));
#40821=CARTESIAN_POINT('Ctrl Pts',(21.9185701869868,5.78272774784621,38.3017123173458));
#40822=CARTESIAN_POINT('Ctrl Pts',(21.9197488176348,5.78350477372963,38.2900641889728));
#40823=CARTESIAN_POINT('Ctrl Pts',(21.9201548666475,5.78378059249129,38.2859172064261));
#40824=CARTESIAN_POINT('Ctrl Pts',(21.9208826378231,5.78429047111685,38.2782276668159));
#40825=CARTESIAN_POINT('Ctrl Pts',(21.9212079958109,5.78452472416589,38.2746855652051));
#40826=CARTESIAN_POINT('Ctrl Pts',(21.9219228477075,5.78505413959939,38.2666594767871));
#40827=CARTESIAN_POINT('Ctrl Pts',(21.922306447129,5.78534897129088,38.2621750229971));
#40828=CARTESIAN_POINT('Ctrl Pts',(21.9234216232755,5.78624008727771,38.2485778938532));
#40829=CARTESIAN_POINT('Ctrl Pts',(21.924104135412,5.78683371906063,38.2394611612914));
#40830=CARTESIAN_POINT('Ctrl Pts',(21.932180418756,5.79455311016005,38.1201989694553));
#40831=CARTESIAN_POINT('Ctrl Pts',(21.9301723148688,5.80120146158693,38.0096030486418));
#40832=CARTESIAN_POINT('Ctrl Pts',(21.9098718888338,5.81290228251413,37.8150715432262));
#40833=CARTESIAN_POINT('Ctrl Pts',(21.8954341166906,5.81795856576337,37.7310503273799));
#40834=CARTESIAN_POINT('Ctrl Pts',(21.8576407027621,5.82775202300741,37.5741428802481));
#40835=CARTESIAN_POINT('Ctrl Pts',(21.8354124924511,5.83245790202405,37.5011563819534));
#40836=CARTESIAN_POINT('Ctrl Pts',(21.8023844611312,5.83850211502345,37.4120266652434));
#40837=CARTESIAN_POINT('Ctrl Pts',(21.7955842961783,5.83970740846969,37.3944689585096));
#40838=CARTESIAN_POINT('Ctrl Pts',(21.785327833543,5.84147180180845,37.3690964383539));
#40839=CARTESIAN_POINT('Ctrl Pts',(21.782074749021,5.84202411927537,37.3612002472254));
#40840=CARTESIAN_POINT('Ctrl Pts',(21.7762786512293,5.8429957162594,37.3473924521641));
#40841=CARTESIAN_POINT('Ctrl Pts',(21.7737582694162,5.84341422908841,37.3414714455733));
#40842=CARTESIAN_POINT('Ctrl Pts',(21.7688051610563,5.84422911463879,37.3299950396324));
#40843=CARTESIAN_POINT('Ctrl Pts',(21.7663757668086,5.84462537059331,37.3244382772515));
#40844=CARTESIAN_POINT('Ctrl Pts',(21.760501062464,5.84557552158884,37.3111718343784));
#40845=CARTESIAN_POINT('Ctrl Pts',(21.7570312765878,5.84613024390353,37.3034731924908));
#40846=CARTESIAN_POINT('Ctrl Pts',(21.7442809250743,5.84814575762447,37.2756718762842));
#40847=CARTESIAN_POINT('Ctrl Pts',(21.7347052847342,5.84961658378573,37.2557072147597));
#40848=CARTESIAN_POINT('Ctrl Pts',(21.6599882317999,5.86078648508399,37.1065659452504));
#40849=CARTESIAN_POINT('Ctrl Pts',(21.5808558218101,5.87099035312545,36.9849432105268));
#40850=CARTESIAN_POINT('Ctrl Pts',(21.4333081790877,5.88754632416385,36.8058542820126));
#40851=CARTESIAN_POINT('Ctrl Pts',(21.373192692474,5.89379416816922,36.7422337980891));
#40852=CARTESIAN_POINT('Ctrl Pts',(21.2817034810973,5.90243389457611,36.6577253623186));
#40853=CARTESIAN_POINT('Ctrl Pts',(21.2537177505086,5.9049730145111,36.633332965432));
#40854=CARTESIAN_POINT('Ctrl Pts',(21.2192544383971,5.9079609395254,36.6050025648526));
#40855=CARTESIAN_POINT('Ctrl Pts',(21.2134375959729,5.90846065063173,36.6002773850281));
#40856=CARTESIAN_POINT('Ctrl Pts',(21.2043517295514,5.90923388039877,36.5929841586359));
#40857=CARTESIAN_POINT('Ctrl Pts',(21.2011017700371,5.90950901924342,36.5903926426322));
#40858=CARTESIAN_POINT('Ctrl Pts',(21.1950543718507,5.91001827957521,36.5856023425361));
#40859=CARTESIAN_POINT('Ctrl Pts',(21.1922592508739,5.91025259023174,36.5834008124568));
#40860=CARTESIAN_POINT('Ctrl Pts',(21.1859038388258,5.91078294755072,36.57842350782));
#40861=CARTESIAN_POINT('Ctrl Pts',(21.1823398917859,5.91107865852928,36.5756524944056));
#40862=CARTESIAN_POINT('Ctrl Pts',(21.1714753566938,5.91197508073917,36.5672662090657));
#40863=CARTESIAN_POINT('Ctrl Pts',(21.1641441225627,5.91257309287245,36.5616905853233));
#40864=CARTESIAN_POINT('Ctrl Pts',(21.1006849705012,5.91769327945025,36.5141414892252));
#40865=CARTESIAN_POINT('Ctrl Pts',(21.0423411681404,5.92202547657566,36.4751978863419));
#40866=CARTESIAN_POINT('Ctrl Pts',(20.8405689638211,5.93625292473153,36.3558712590347));
#40867=CARTESIAN_POINT('Ctrl Pts',(20.6890364644856,5.94579881061955,36.2906432455044));
#40868=CARTESIAN_POINT('Ctrl Pts',(20.4844856463549,5.95898810760875,36.2320696059507));
#40869=CARTESIAN_POINT('Ctrl Pts',(20.4374217475012,5.96203680082886,36.220491580796));
#40870=CARTESIAN_POINT('Ctrl Pts',(20.3781110988416,5.96591887000632,36.2082491447454));
#40871=CARTESIAN_POINT('Ctrl Pts',(20.3662248029209,5.96669881469924,36.2059121761912));
#40872=CARTESIAN_POINT('Ctrl Pts',(20.347265069235,5.96794632433479,36.2023696351068));
#40873=CARTESIAN_POINT('Ctrl Pts',(20.3402054209525,5.96841158688436,36.2010912872572));
#40874=CARTESIAN_POINT('Ctrl Pts',(20.3268681731558,5.9692920620867,36.1987529658753));
#40875=CARTESIAN_POINT('Ctrl Pts',(20.3205921221781,5.96970700474749,36.1976846273648));
#40876=CARTESIAN_POINT('Ctrl Pts',(20.306412999504,5.97064591576889,36.1953431517874));
#40877=CARTESIAN_POINT('Ctrl Pts',(20.2985070994508,5.97117044577746,36.1940881069593));
#40878=CARTESIAN_POINT('Ctrl Pts',(20.2782086909663,5.97251989372608,36.1909951725188));
#40879=CARTESIAN_POINT('Ctrl Pts',(20.2658058307352,5.97334703522875,36.1892287539085));
#40880=CARTESIAN_POINT('Ctrl Pts',(20.188383105047,5.97852727952747,36.1789705797588));
#40881=CARTESIAN_POINT('Ctrl Pts',(20.1229898042634,5.98297928611301,36.1736786299597));
#40882=CARTESIAN_POINT('Ctrl Pts',(19.9188178335748,5.99712366081145,36.1675945669214));
#40883=CARTESIAN_POINT('Ctrl Pts',(19.7801431764037,6.0071133681178,36.1784285868496));
#40884=CARTESIAN_POINT('Ctrl Pts',(19.5758830278839,6.02184670502054,36.216797957994));
#40885=CARTESIAN_POINT('Ctrl Pts',(19.5086436346707,6.02669149321243,36.2332123581034));
#40886=CARTESIAN_POINT('Ctrl Pts',(19.4295815711161,6.03227815320782,36.2570823786264));
#40887=CARTESIAN_POINT('Ctrl Pts',(19.4167786148593,6.03317925292829,36.2610939709181));
#40888=CARTESIAN_POINT('Ctrl Pts',(19.4007105215328,6.03430474293813,36.2663133385327));
#40889=CARTESIAN_POINT('Ctrl Pts',(19.3974058055968,6.03453593175069,36.2673966908421));
#40890=CARTESIAN_POINT('Ctrl Pts',(19.3941040087491,6.0347666134114,36.2684889831928));
#40891=CARTESIAN_POINT('Origin',(20.,-1.3495818343519,38.1));
#40892=CARTESIAN_POINT('',(19.394104010982,6.99874099840483,36.2684889824541));
#40893=CARTESIAN_POINT('',(19.3941039843085,6.82605087843334,36.2684889912782));
#40894=CARTESIAN_POINT('',(19.3941040087494,-1.3495818343519,36.2684889831927));
#40895=CARTESIAN_POINT('',(18.0708702248395,6.36356089767328,38.1009313909468));
#40896=CARTESIAN_POINT('Ctrl Pts',(19.394104010982,6.99874099840483,36.2684889824541));
#40897=CARTESIAN_POINT('Ctrl Pts',(19.3969825380143,6.99855649777902,36.2675367151915));
#40898=CARTESIAN_POINT('Ctrl Pts',(19.3998634709182,6.99837185025014,36.266591180833));
#40899=CARTESIAN_POINT('Ctrl Pts',(19.4294489278064,6.9964756380809,36.2569583233041));
#40900=CARTESIAN_POINT('Ctrl Pts',(19.4563368713021,6.9947523103515,36.2488486131989));
#40901=CARTESIAN_POINT('Ctrl Pts',(19.5306214382265,6.98997810224285,36.2282015816547));
#40902=CARTESIAN_POINT('Ctrl Pts',(19.5783310892964,6.98689693497634,36.2168801816735));
#40903=CARTESIAN_POINT('Ctrl Pts',(19.6387578306271,6.98295202472202,36.2049525394638));
#40904=CARTESIAN_POINT('Ctrl Pts',(19.6511217809934,6.98214268879871,36.2026374203114));
#40905=CARTESIAN_POINT('Ctrl Pts',(19.670745012419,6.98085437036893,36.1991613064221));
#40906=CARTESIAN_POINT('Ctrl Pts',(19.6779899539549,6.98037790445743,36.1979205816724));
#40907=CARTESIAN_POINT('Ctrl Pts',(19.6915042094846,6.97948754014319,36.1956856363961));
#40908=CARTESIAN_POINT('Ctrl Pts',(19.6977717016498,6.97907397921481,36.1946808922749));
#40909=CARTESIAN_POINT('Ctrl Pts',(19.7117095625718,6.9781528200299,36.1925170097395));
#40910=CARTESIAN_POINT('Ctrl Pts',(19.7193821615316,6.97764474828788,36.1913731741848));
#40911=CARTESIAN_POINT('Ctrl Pts',(19.7417343778093,6.97616162673869,36.1881785856046));
#40912=CARTESIAN_POINT('Ctrl Pts',(19.7564307212911,6.97518275070171,36.1862507379818));
#40913=CARTESIAN_POINT('Ctrl Pts',(19.8826959645587,6.96673876574513,36.1711653788264));
#40914=CARTESIAN_POINT('Ctrl Pts',(19.9951751024177,6.958970909739,36.1676097961494));
#40915=CARTESIAN_POINT('Ctrl Pts',(20.2313615024685,6.94223280054393,36.1807679512967));
#40916=CARTESIAN_POINT('Ctrl Pts',(20.3544560244407,6.93325909401283,36.1996471662492));
#40917=CARTESIAN_POINT('Ctrl Pts',(20.5165591029919,6.92159881364518,36.2408178029232));
#40918=CARTESIAN_POINT('Ctrl Pts',(20.5578763458919,6.91864371940896,36.2527949790388));
#40919=CARTESIAN_POINT('Ctrl Pts',(20.6058270547113,6.91526036063549,36.2684511004375));
#40920=CARTESIAN_POINT('Ctrl Pts',(20.6128787721056,6.91476399180772,36.2707986970317));
#40921=CARTESIAN_POINT('Ctrl Pts',(20.624264642262,6.91396467560942,36.2746624166818));
#40922=CARTESIAN_POINT('Ctrl Pts',(20.628607175102,6.9136603231646,36.2761533350788));
#40923=CARTESIAN_POINT('Ctrl Pts',(20.6363117517574,6.91312128537265,36.2788293274865));
#40924=CARTESIAN_POINT('Ctrl Pts',(20.6396758700575,6.91288624517374,36.2800082291756));
#40925=CARTESIAN_POINT('Ctrl Pts',(20.6469053502762,6.91238185347314,36.2825642071469));
#40926=CARTESIAN_POINT('Ctrl Pts',(20.6507695843416,6.91211268160553,36.2839442898876));
#40927=CARTESIAN_POINT('Ctrl Pts',(20.6614485842059,6.91136992831127,36.2877966781647));
#40928=CARTESIAN_POINT('Ctrl Pts',(20.6682539499171,6.910897857536,36.2902951147475));
#40929=CARTESIAN_POINT('Ctrl Pts',(20.7060775625588,6.90828031079725,36.3044236555528));
#40930=CARTESIAN_POINT('Ctrl Pts',(20.7368084816679,6.90617680768287,36.3168136627134));
#40931=CARTESIAN_POINT('Ctrl Pts',(20.8331328662127,6.89961154936868,36.3585652669897));
#40932=CARTESIAN_POINT('Ctrl Pts',(20.897416268238,6.89527099233744,36.390803976408));
#40933=CARTESIAN_POINT('Ctrl Pts',(21.1045964293148,6.88095703353016,36.509626238483));
#40934=CARTESIAN_POINT('Ctrl Pts',(21.2380230987505,6.87112558392545,36.611136333886));
#40935=CARTESIAN_POINT('Ctrl Pts',(21.3713356552431,6.85922844029134,36.7430165321513));
#40936=CARTESIAN_POINT('Ctrl Pts',(21.3857252286921,6.85791399777198,36.7577142069176));
#40937=CARTESIAN_POINT('Ctrl Pts',(21.4055105618989,6.85606206603671,36.7785804365622));
#40938=CARTESIAN_POINT('Ctrl Pts',(21.4111065399666,6.85553313681933,36.7845578949552));
#40939=CARTESIAN_POINT('Ctrl Pts',(21.4207355664862,6.85461393846064,36.7949754849916));
#40940=CARTESIAN_POINT('Ctrl Pts',(21.4247863042118,6.85422442247484,36.7993991693705));
#40941=CARTESIAN_POINT('Ctrl Pts',(21.4331672555705,6.85341256146144,36.8086378860833));
#40942=CARTESIAN_POINT('Ctrl Pts',(21.4374939804497,6.85299007768223,36.8134559680452));
#40943=CARTESIAN_POINT('Ctrl Pts',(21.4476356187059,6.85199178602018,36.8248643534782));
#40944=CARTESIAN_POINT('Ctrl Pts',(21.4534298761918,6.85141513348374,36.8314727467411));
#40945=CARTESIAN_POINT('Ctrl Pts',(21.4724059782312,6.84950548961063,36.8534158259916));
#40946=CARTESIAN_POINT('Ctrl Pts',(21.485391504689,6.84816455162974,36.8689177554752));
#40947=CARTESIAN_POINT('Ctrl Pts',(21.6122812323686,6.83471025071618,37.025327642816));
#40948=CARTESIAN_POINT('Ctrl Pts',(21.7060184952387,6.82175756306093,37.1813906103987));
#40949=CARTESIAN_POINT('Ctrl Pts',(21.811065691505,6.80257897925162,37.4296233467429));
#40950=CARTESIAN_POINT('Ctrl Pts',(21.839894841344,6.79634838858619,37.5133530302575));
#40951=CARTESIAN_POINT('Ctrl Pts',(21.8653146567028,6.78977242212699,37.6078295910765));
#40952=CARTESIAN_POINT('Ctrl Pts',(21.8676849226925,6.78914550667107,37.6169021649875));
#40953=CARTESIAN_POINT('Ctrl Pts',(21.8711063327219,6.78821996030603,37.6303998222863));
#40954=CARTESIAN_POINT('Ctrl Pts',(21.8722080901398,6.78791855925692,37.6348117547409));
#40955=CARTESIAN_POINT('Ctrl Pts',(21.8741447165574,6.78738274612209,37.642685210517));
#40956=CARTESIAN_POINT('Ctrl Pts',(21.8749856102546,6.78714799553545,37.6461451803262));
#40957=CARTESIAN_POINT('Ctrl Pts',(21.8767818734168,6.78664195979787,37.6536263467126));
#40958=CARTESIAN_POINT('Ctrl Pts',(21.8777338995115,6.78637086624412,37.6576482822989));
#40959=CARTESIAN_POINT('Ctrl Pts',(21.8803510883801,6.78561735930349,37.6688655820768));
#40960=CARTESIAN_POINT('Ctrl Pts',(21.8819878899519,6.78513652919693,37.6760675899872));
#40961=CARTESIAN_POINT('Ctrl Pts',(21.8912036071185,6.78237160188965,37.7177227250984));
#40962=CARTESIAN_POINT('Ctrl Pts',(21.8978782734341,6.78013523352681,37.7523716958706));
#40963=CARTESIAN_POINT('Ctrl Pts',(21.9165617854201,6.77294564065268,37.8660686897191));
#40964=CARTESIAN_POINT('Ctrl Pts',(21.9246097121476,6.76814177338919,37.9456869201821));
#40965=CARTESIAN_POINT('Ctrl Pts',(21.933671696441,6.75409309085649,38.1804205253587));
#40966=CARTESIAN_POINT('Ctrl Pts',(21.9209726281809,6.74491431598283,38.3353967079668));
#40967=CARTESIAN_POINT('Ctrl Pts',(21.8855412358311,6.73372605163393,38.5083423550071));
#40968=CARTESIAN_POINT('Ctrl Pts',(21.8808505259981,6.73234652151058,38.5294304020046));
#40969=CARTESIAN_POINT('Ctrl Pts',(21.8738547967794,6.73041755936212,38.5585636817234));
#40970=CARTESIAN_POINT('Ctrl Pts',(21.8718499714003,6.72987766646406,38.5666799016223));
#40971=CARTESIAN_POINT('Ctrl Pts',(21.8683053353252,6.72894464390395,38.5806394107818));
#40972=CARTESIAN_POINT('Ctrl Pts',(21.8667906967817,6.72855232306394,38.5864890155315));
#40973=CARTESIAN_POINT('Ctrl Pts',(21.8636032018085,6.72773956886715,38.5985651722654));
#40974=CARTESIAN_POINT('Ctrl Pts',(21.861926565001,6.72731901853094,38.6047906394163));
#40975=CARTESIAN_POINT('Ctrl Pts',(21.857936080698,6.72633399356797,38.6193171844776));
#40976=CARTESIAN_POINT('Ctrl Pts',(21.8555977703904,6.72576873723137,38.6276113422916));
#40977=CARTESIAN_POINT('Ctrl Pts',(21.8478552642206,6.72393462016671,38.6543863489355));
#40978=CARTESIAN_POINT('Ctrl Pts',(21.8422300733944,6.7226586541112,38.6728015473309));
#40979=CARTESIAN_POINT('Ctrl Pts',(21.8119580477984,6.71606588349043,38.7668409999778));
#40980=CARTESIAN_POINT('Ctrl Pts',(21.7829299582975,6.71060777549491,38.8409633722076));
#40981=CARTESIAN_POINT('Ctrl Pts',(21.7037027030375,6.69744168595572,39.0114289246818));
#40982=CARTESIAN_POINT('Ctrl Pts',(21.6497796241485,6.68965383587968,39.1057485432105));
#40983=CARTESIAN_POINT('Ctrl Pts',(21.5411951110403,6.67606128978428,39.2632386874165));
#40984=CARTESIAN_POINT('Ctrl Pts',(21.4898159376284,6.67024053973609,39.3283560046677));
#40985=CARTESIAN_POINT('Ctrl Pts',(21.4281513997816,6.66404252628375,39.3969246399541));
#40986=CARTESIAN_POINT('Ctrl Pts',(21.4218499535432,6.66341755326085,39.4038299968424));
#40987=CARTESIAN_POINT('Ctrl Pts',(21.4124126944714,6.6624943100908,39.4140219040444));
#40988=CARTESIAN_POINT('Ctrl Pts',(21.4093151843065,6.66219328940394,39.4173434996779));
#40989=CARTESIAN_POINT('Ctrl Pts',(21.4037686768452,6.66165788930268,39.4232493090076));
#40990=CARTESIAN_POINT('Ctrl Pts',(21.4013242352707,6.6614231734979,39.4258377050916));
#40991=CARTESIAN_POINT('Ctrl Pts',(21.3960237986257,6.66091691427163,39.431419252269));
#40992=CARTESIAN_POINT('Ctrl Pts',(21.3931653433328,6.66064556403257,39.4344099814424));
#40993=CARTESIAN_POINT('Ctrl Pts',(21.3851645586827,6.65989061743674,39.4427272682827));
#40994=CARTESIAN_POINT('Ctrl Pts',(21.3800010857659,6.65940861419971,39.4480335230369));
#40995=CARTESIAN_POINT('Ctrl Pts',(21.3498491593686,6.65662313134406,39.4786644069264));
#40996=CARTESIAN_POINT('Ctrl Pts',(21.3241926738326,6.65436821456068,39.5033254974281));
#40997=CARTESIAN_POINT('Ctrl Pts',(21.2378457610063,6.64708804678187,39.5818440786651));
#40998=CARTESIAN_POINT('Ctrl Pts',(21.1744363575599,6.64221649046842,39.6325878261729));
#40999=CARTESIAN_POINT('Ctrl Pts',(20.9825460307795,6.62820067217016,39.7672247193048));
#41000=CARTESIAN_POINT('Ctrl Pts',(20.8470495907457,6.61911393828452,39.8399815208395));
#41001=CARTESIAN_POINT('Ctrl Pts',(20.6841635625951,6.6080265344754,39.9038664818191));
#41002=CARTESIAN_POINT('Ctrl Pts',(20.66381679908,6.60663998564747,39.9114528040681));
#41003=CARTESIAN_POINT('Ctrl Pts',(20.6354485273231,6.60470275848451,39.9214878307396));
#41004=CARTESIAN_POINT('Ctrl Pts',(20.6275320908898,6.60416172820722,39.9242303088401));
#41005=CARTESIAN_POINT('Ctrl Pts',(20.6138713285764,6.60322726746436,39.928863340316));
#41006=CARTESIAN_POINT('Ctrl Pts',(20.6081354688641,6.60283465165433,39.9307786255385));
#41007=CARTESIAN_POINT('Ctrl Pts',(20.5962683568232,6.60202178234736,39.934679300877));
#41008=CARTESIAN_POINT('Ctrl Pts',(20.5901359785164,6.60160141406334,39.9366609963707));
#41009=CARTESIAN_POINT('Ctrl Pts',(20.5757966488048,6.60061767737159,39.9412155629398));
#41010=CARTESIAN_POINT('Ctrl Pts',(20.5675822441648,6.60005353335721,39.9437643347397));
#41011=CARTESIAN_POINT('Ctrl Pts',(20.5410123345249,6.59822667774027,39.9518140817853));
#41012=CARTESIAN_POINT('Ctrl Pts',(20.5225923083016,6.59695693911199,39.9570963825587));
#41013=CARTESIAN_POINT('Ctrl Pts',(20.4280209854922,6.59041928603718,39.982698152294));
#41014=CARTESIAN_POINT('Ctrl Pts',(20.3507641302908,6.58501271663675,39.9986089553149));
#41015=CARTESIAN_POINT('Ctrl Pts',(20.1675891288131,6.57205793162762,40.0247708492753));
#41016=CARTESIAN_POINT('Ctrl Pts',(20.0613624672085,6.56443508439255,40.0310776731067));
#41017=CARTESIAN_POINT('Ctrl Pts',(19.8692923521259,6.55077320081843,40.0266126605239));
#41018=CARTESIAN_POINT('Ctrl Pts',(19.7836365842105,6.54472917887144,40.0188828441445));
#41019=CARTESIAN_POINT('Ctrl Pts',(19.6895190004305,6.53832471488099,40.0040041670876));
#41020=CARTESIAN_POINT('Ctrl Pts',(19.6802762960399,6.53769837899685,40.002473937062));
#41021=CARTESIAN_POINT('Ctrl Pts',(19.6665657957742,6.53677351977116,40.0001012739759));
#41022=CARTESIAN_POINT('Ctrl Pts',(19.6620894083864,6.53647223214436,39.999310309833));
#41023=CARTESIAN_POINT('Ctrl Pts',(19.654111800291,6.53593654223697,39.9978715940657));
#41024=CARTESIAN_POINT('Ctrl Pts',(19.6506095459945,6.53570180208498,39.9972299664592));
#41025=CARTESIAN_POINT('Ctrl Pts',(19.6430445554174,6.53519569999051,39.9958223701336));
#41026=CARTESIAN_POINT('Ctrl Pts',(19.6389825078954,6.53492453011686,39.9950530387575));
#41027=CARTESIAN_POINT('Ctrl Pts',(19.6276655914382,6.53417059520872,39.9928719634991));
#41028=CARTESIAN_POINT('Ctrl Pts',(19.6204162199084,6.53368941637665,39.9914315584222));
#41029=CARTESIAN_POINT('Ctrl Pts',(19.5785277529631,6.53091839974047,39.9828580492342));
#41030=CARTESIAN_POINT('Ctrl Pts',(19.5440792115373,6.52867653703816,39.9748146324447));
#41031=CARTESIAN_POINT('Ctrl Pts',(19.4322136963471,6.52146020680714,39.9454288672245));
#41032=CARTESIAN_POINT('Ctrl Pts',(19.3559010866419,6.51663637029006,39.9201999162813));
#41033=CARTESIAN_POINT('Ctrl Pts',(19.1380268531737,6.50259686181839,39.8327450075071));
#41034=CARTESIAN_POINT('Ctrl Pts',(19.0021238529748,6.49344466030962,39.7582038205337));
#41035=CARTESIAN_POINT('Ctrl Pts',(18.8589846658551,6.48228591568714,39.6556652487622));
#41036=CARTESIAN_POINT('Ctrl Pts',(18.8416155327358,6.48090474431667,39.64277533204));
#41037=CARTESIAN_POINT('Ctrl Pts',(18.8178352584306,6.47897384847177,39.6244996042947));
#41038=CARTESIAN_POINT('Ctrl Pts',(18.8112364962756,6.47843368853627,39.6193596836539));
#41039=CARTESIAN_POINT('Ctrl Pts',(18.7999277945118,6.47750032837893,39.6104323169352));
#41040=CARTESIAN_POINT('Ctrl Pts',(18.7952018050785,6.47710793834776,39.6066653213515));
#41041=CARTESIAN_POINT('Ctrl Pts',(18.7856080547246,6.47630657305666,39.5989443248001));
#41042=CARTESIAN_POINT('Ctrl Pts',(18.7807417212316,6.47589753491458,39.5949886734358));
#41043=CARTESIAN_POINT('Ctrl Pts',(18.7695209755349,6.47494839202759,39.5857765430355));
#41044=CARTESIAN_POINT('Ctrl Pts',(18.7631808464915,6.47440760170953,39.580502935978));
#41045=CARTESIAN_POINT('Ctrl Pts',(18.7498597478808,6.47326173017266,39.569277395175));
#41046=CARTESIAN_POINT('Ctrl Pts',(18.7428870491596,6.47265627168856,39.5633160075158));
#41047=CARTESIAN_POINT('Ctrl Pts',(18.7243748144791,6.47103342299823,39.5472587970561));
#41048=CARTESIAN_POINT('Ctrl Pts',(18.7129128676791,6.47001243973116,39.5370749216743));
#41049=CARTESIAN_POINT('Ctrl Pts',(18.6781035098765,6.46686101442338,39.5053964916249));
#41050=CARTESIAN_POINT('Ctrl Pts',(18.655165055665,6.46471261591111,39.4834624698534));
#41051=CARTESIAN_POINT('Ctrl Pts',(18.5674150114258,6.45620484620139,39.3953096311315));
#41052=CARTESIAN_POINT('Ctrl Pts',(18.5068737927178,6.44968275297695,39.3250295020811));
#41053=CARTESIAN_POINT('Ctrl Pts',(18.3713312135895,6.43350636978183,39.1426407143452));
#41054=CARTESIAN_POINT('Ctrl Pts',(18.3025638048707,6.42380144561958,39.0264867065912));
#41055=CARTESIAN_POINT('Ctrl Pts',(18.2405727776872,6.41372738985213,38.8913008498265));
#41056=CARTESIAN_POINT('Ctrl Pts',(18.2348385626528,6.41277972647638,38.8784255353265));
#41057=CARTESIAN_POINT('Ctrl Pts',(18.2270529553291,6.41147163928579,38.860415591817));
#41058=CARTESIAN_POINT('Ctrl Pts',(18.2248819158808,6.41110445253878,38.8553336248158));
#41059=CARTESIAN_POINT('Ctrl Pts',(18.2214288496999,6.41051658635887,38.8471535723329));
#41060=CARTESIAN_POINT('Ctrl Pts',(18.2201330297544,6.4102950887833,38.8440613993401));
#41061=CARTESIAN_POINT('Ctrl Pts',(18.2174363673209,6.40983228791064,38.8375790855304));
#41062=CARTESIAN_POINT('Ctrl Pts',(18.2160371250829,6.40959108637183,38.8341883090793));
#41063=CARTESIAN_POINT('Ctrl Pts',(18.2126569354433,6.40900575680729,38.825930395567));
#41064=CARTESIAN_POINT('Ctrl Pts',(18.2106861675562,6.40866223586658,38.8210590684853));
#41065=CARTESIAN_POINT('Ctrl Pts',(18.2037584896539,6.40744639338624,38.8037319853082));
#41066=CARTESIAN_POINT('Ctrl Pts',(18.1989113963547,6.40658035292994,38.7912323319331));
#41067=CARTESIAN_POINT('Ctrl Pts',(18.1699016773208,6.40129418109856,38.714044720243));
#41068=CARTESIAN_POINT('Ctrl Pts',(18.1490937454587,6.39704547988534,38.6481413778059));
#41069=CARTESIAN_POINT('Ctrl Pts',(18.0914385626056,6.38305589527803,38.4243364055669));
#41070=CARTESIAN_POINT('Ctrl Pts',(18.0709484539361,6.37362273943145,38.2629622546331));
#41071=CARTESIAN_POINT('Ctrl Pts',(18.0708702248395,6.36356089767328,38.1009313909468));
#41072=CARTESIAN_POINT('Ctrl Pts',(18.0708702237818,6.36356076147475,38.1009291976744));
#41073=CARTESIAN_POINT('Ctrl Pts',(18.0708562063867,6.36175358491646,38.0718273444537));
#41074=CARTESIAN_POINT('Ctrl Pts',(18.0715007119562,6.35992981219923,38.0427297870862));
#41075=CARTESIAN_POINT('Ctrl Pts',(18.0736406571234,6.35690143396561,37.9949647470844));
#41076=CARTESIAN_POINT('Ctrl Pts',(18.0747501044797,6.35570839004714,37.976284505585));
#41077=CARTESIAN_POINT('Ctrl Pts',(18.0767324183429,6.35398389679972,37.9494983321484));
#41078=CARTESIAN_POINT('Ctrl Pts',(18.077385212855,6.35345921675814,37.9413767998481));
#41079=CARTESIAN_POINT('Ctrl Pts',(18.0786303395921,6.35252871628467,37.9270250030368));
#41080=CARTESIAN_POINT('Ctrl Pts',(18.0792015807072,6.35212355364348,37.9207929900014));
#41081=CARTESIAN_POINT('Ctrl Pts',(18.0803895083089,6.35132158265804,37.9084919591246));
#41082=CARTESIAN_POINT('Ctrl Pts',(18.0810046784413,6.35092482598635,37.9024228658381));
#41083=CARTESIAN_POINT('Ctrl Pts',(18.0822871368229,6.35013285896987,37.890341900644));
#41084=CARTESIAN_POINT('Ctrl Pts',(18.0829539354062,6.34973766824377,37.8843300460232));
#41085=CARTESIAN_POINT('Ctrl Pts',(18.0846123961175,6.34879259196734,37.8699931002906));
#41086=CARTESIAN_POINT('Ctrl Pts',(18.085630070801,6.34824189900749,37.861671198856));
#41087=CARTESIAN_POINT('Ctrl Pts',(18.0894829000983,6.34625631742746,37.8317835068272));
#41088=CARTESIAN_POINT('Ctrl Pts',(18.0926284098237,6.34481177875687,37.8102600687578));
#41089=CARTESIAN_POINT('Ctrl Pts',(18.1028322013195,6.3405779460009,37.7478361709861));
#41090=CARTESIAN_POINT('Ctrl Pts',(18.110846892159,6.33775966578563,37.7071067325128));
#41091=CARTESIAN_POINT('Ctrl Pts',(18.1485410876324,6.32621569665157,37.5435853421105));
#41092=CARTESIAN_POINT('Ctrl Pts',(18.1889312797888,6.31718958373903,37.423597660045));
#41093=CARTESIAN_POINT('Ctrl Pts',(18.2693947177375,6.30321180285362,37.2447678583331));
#41094=CARTESIAN_POINT('Ctrl Pts',(18.301478403927,6.29825939999035,37.1826982972689));
#41095=CARTESIAN_POINT('Ctrl Pts',(18.3533550519394,6.29118474245683,37.0944340600152));
#41096=CARTESIAN_POINT('Ctrl Pts',(18.3705603682652,6.28896418145649,37.0667869336636));
#41097=CARTESIAN_POINT('Ctrl Pts',(18.3924224547157,6.28630205199639,37.0335624740425));
#41098=CARTESIAN_POINT('Ctrl Pts',(18.3964202646315,6.28582139978791,37.0275604458819));
#41099=CARTESIAN_POINT('Ctrl Pts',(18.4027408403546,6.28507123328818,37.0181855510038));
#41100=CARTESIAN_POINT('Ctrl Pts',(18.4050407976533,6.28480024778613,37.0147974987346));
#41101=CARTESIAN_POINT('Ctrl Pts',(18.4093637939755,6.28429464473436,37.0084727519365));
#41102=CARTESIAN_POINT('Ctrl Pts',(18.4113841657191,6.28405986283447,37.0055343748968));
#41103=CARTESIAN_POINT('Ctrl Pts',(18.4160317686924,6.28352321064337,36.9988150035654));
#41104=CARTESIAN_POINT('Ctrl Pts',(18.4186643929506,6.2832217088112,36.995037804662));
#41105=CARTESIAN_POINT('Ctrl Pts',(18.4256064295058,6.28243304975194,36.985153233965));
#41106=CARTESIAN_POINT('Ctrl Pts',(18.4299379091413,6.28194734219636,36.9790613478903));
#41107=CARTESIAN_POINT('Ctrl Pts',(18.4599380788764,6.2786255817164,36.9373835301914));
#41108=CARTESIAN_POINT('Ctrl Pts',(18.4867812079084,6.27586369073988,36.9026540382753));
#41109=CARTESIAN_POINT('Ctrl Pts',(18.5304810475113,6.27162833310501,36.8499354817733));
#41110=CARTESIAN_POINT('Ctrl Pts',(18.5465353117829,6.27012270054339,36.8313047136528));
#41111=CARTESIAN_POINT('Ctrl Pts',(18.6743530848435,6.2584742901393,36.6885856107018));
#41112=CARTESIAN_POINT('Ctrl Pts',(18.8014415101232,6.24878708483426,36.5791809730441));
#41113=CARTESIAN_POINT('Ctrl Pts',(18.9679201675323,6.2364442271233,36.4698502029863));
#41114=CARTESIAN_POINT('Ctrl Pts',(18.9952419015739,6.23443105596157,36.4528697287211));
#41115=CARTESIAN_POINT('Ctrl Pts',(19.0363226672433,6.23141379058955,36.4287405328961));
#41116=CARTESIAN_POINT('Ctrl Pts',(19.0497646678353,6.23042803453266,36.4210613471948));
#41117=CARTESIAN_POINT('Ctrl Pts',(19.0713699993932,6.2288452218387,36.4090611628361));
#41118=CARTESIAN_POINT('Ctrl Pts',(19.0794746384419,6.22825182802206,36.4046354719387));
#41119=CARTESIAN_POINT('Ctrl Pts',(19.0949518123392,6.22711913397922,36.3963275677258));
#41120=CARTESIAN_POINT('Ctrl Pts',(19.1023183530476,6.22658022474019,36.3924345881853));
#41121=CARTESIAN_POINT('Ctrl Pts',(19.1153132812418,6.22562982141283,36.3856745166606));
#41122=CARTESIAN_POINT('Ctrl Pts',(19.1209310009561,6.22521904542373,36.3827870992462));
#41123=CARTESIAN_POINT('Ctrl Pts',(19.1319534649751,6.22441318341607,36.3771899922128));
#41124=CARTESIAN_POINT('Ctrl Pts',(19.1373569718154,6.22401818289392,36.3744780168223));
#41125=CARTESIAN_POINT('Ctrl Pts',(19.150274093921,6.22307401512768,36.368070858894));
#41126=CARTESIAN_POINT('Ctrl Pts',(19.1577991433123,6.22252404401851,36.364399130405));
#41127=CARTESIAN_POINT('Ctrl Pts',(19.1848963545166,6.22054371190507,36.3513951957271));
#41128=CARTESIAN_POINT('Ctrl Pts',(19.2046010206094,6.21910376725725,36.3423444270437));
#41129=CARTESIAN_POINT('Ctrl Pts',(19.2800002401795,6.21359222191381,36.309239503984));
#41130=CARTESIAN_POINT('Ctrl Pts',(19.3366154081508,6.20944891981682,36.2875072066427));
#41131=CARTESIAN_POINT('Ctrl Pts',(19.3941044301425,6.20523851046618,36.2684888437885));
#41132=CARTESIAN_POINT('Ctrl Pts',(19.3941040087491,6.0347666134114,36.2684889831928));
#41133=CARTESIAN_POINT('Ctrl Pts',(19.3924153457498,6.03488459268239,36.2690476225526));
#41134=CARTESIAN_POINT('Ctrl Pts',(19.3907274462916,6.03500243929733,36.2696086003447));
#41135=CARTESIAN_POINT('Ctrl Pts',(19.3855607656699,6.03536292103602,36.2713336987786));
#41136=CARTESIAN_POINT('Ctrl Pts',(19.3820844874754,6.03560511749658,36.2725054215932));
#41137=CARTESIAN_POINT('Ctrl Pts',(19.3754378577733,6.03606750803258,36.2747668846138));
#41138=CARTESIAN_POINT('Ctrl Pts',(19.3722669887204,6.03628779962772,36.2758549778093));
#41139=CARTESIAN_POINT('Ctrl Pts',(19.3638783399758,6.03686983846296,36.2787580310786));
#41140=CARTESIAN_POINT('Ctrl Pts',(19.3586654439502,6.03723076014707,36.2805871648327));
#41141=CARTESIAN_POINT('Ctrl Pts',(19.3401922360461,6.03850727993246,36.287158420741));
#41142=CARTESIAN_POINT('Ctrl Pts',(19.3269756848599,6.03941598046567,36.2920234581286));
#41143=CARTESIAN_POINT('Ctrl Pts',(19.1882219720687,6.04891937150135,36.3448313980802));
#41144=CARTESIAN_POINT('Ctrl Pts',(19.0679489723965,6.05685666503879,36.4056292305197));
#41145=CARTESIAN_POINT('Ctrl Pts',(18.8769423966935,6.07043508463694,36.5287269355388));
#41146=CARTESIAN_POINT('Ctrl Pts',(18.8026596233994,6.07600554504561,36.5845688921628));
#41147=CARTESIAN_POINT('Ctrl Pts',(18.6963411986952,6.08474835009224,36.6772067979981));
#41148=CARTESIAN_POINT('Ctrl Pts',(18.6611959560312,6.08778210198083,36.7102266764293));
#41149=CARTESIAN_POINT('Ctrl Pts',(18.6188283076276,6.09164743379935,36.7531319330377));
#41150=CARTESIAN_POINT('Ctrl Pts',(18.6104115764933,6.09242614981,36.7618173383008));
#41151=CARTESIAN_POINT('Ctrl Pts',(18.5971360218893,6.09367214953448,36.7757769720279));
#41152=CARTESIAN_POINT('Ctrl Pts',(18.59222388284,6.09413714064111,36.7810002386087));
#41153=CARTESIAN_POINT('Ctrl Pts',(18.5830050565253,6.09501738958114,36.7909131327815));
#41154=CARTESIAN_POINT('Ctrl Pts',(18.5786922345679,6.09543237910192,36.7955969449378));
#41155=CARTESIAN_POINT('Ctrl Pts',(18.5690050657556,6.09637178452624,36.8062224912053));
#41156=CARTESIAN_POINT('Ctrl Pts',(18.5636444142977,6.09689676448525,36.8121764980176));
#41157=CARTESIAN_POINT('Ctrl Pts',(18.5499819690965,6.09824813352873,36.8275426243712));
#41158=CARTESIAN_POINT('Ctrl Pts',(18.5417347582905,6.09907675688633,36.8370025594008));
#41159=CARTESIAN_POINT('Ctrl Pts',(18.4906860455431,6.10428813669584,36.8967244081054));
#41160=CARTESIAN_POINT('Ctrl Pts',(18.4504005192885,6.10877118961416,36.9490697399866));
#41161=CARTESIAN_POINT('Ctrl Pts',(18.3342219547872,6.1229271842419,37.1172117339158));
#41162=CARTESIAN_POINT('Ctrl Pts',(18.2680454643907,6.13289331917305,37.2391775512269));
#41163=CARTESIAN_POINT('Ctrl Pts',(18.1892710269677,6.14759263097347,37.430995708373));
#41164=CARTESIAN_POINT('Ctrl Pts',(18.1664939981097,6.15242742182652,37.4962087044611));
#41165=CARTESIAN_POINT('Ctrl Pts',(18.1435258249744,6.15800376285889,37.5753803112153));
#41166=CARTESIAN_POINT('Ctrl Pts',(18.1399257848916,6.15890394154564,37.5882909817938));
#41167=CARTESIAN_POINT('Ctrl Pts',(18.1351020252303,6.1601468724167,37.6063141609065));
#41168=CARTESIAN_POINT('Ctrl Pts',(18.1337643026059,6.16049577770303,37.6113953669916));
#41169=CARTESIAN_POINT('Ctrl Pts',(18.1315279963284,6.16108624932854,37.6200329361435));
#41170=CARTESIAN_POINT('Ctrl Pts',(18.1306187712523,6.16132841781359,37.6235864891544));
#41171=CARTESIAN_POINT('Ctrl Pts',(18.1288978593356,6.1617908092281,37.6303931674237));
#41172=CARTESIAN_POINT('Ctrl Pts',(18.1280845137114,6.16201112941796,37.633645831344));
#41173=CARTESIAN_POINT('Ctrl Pts',(18.1259529183884,6.16259334946537,37.6422657565937));
#41174=CARTESIAN_POINT('Ctrl Pts',(18.1246492342355,6.16295442280109,37.6476366406582));
#41175=CARTESIAN_POINT('Ctrl Pts',(18.1201022823649,6.16423202907998,37.6667265808073));
#41176=CARTESIAN_POINT('Ctrl Pts',(18.1169862338227,6.16514164902678,37.6804759019064));
#41177=CARTESIAN_POINT('Ctrl Pts',(18.0854605341825,6.17473626197454,37.8270145805573));
#41178=CARTESIAN_POINT('Ctrl Pts',(18.0709925084668,6.18275015076872,37.9624361503233));
#41179=CARTESIAN_POINT('Ctrl Pts',(18.0707504547577,6.19889168787557,38.2325285113259));
#41180=CARTESIAN_POINT('Ctrl Pts',(18.0846447830548,6.20698376711884,38.3664110565059));
#41181=CARTESIAN_POINT('Ctrl Pts',(18.115142026472,6.21642789560342,38.5111449305759));
#41182=CARTESIAN_POINT('Ctrl Pts',(18.1181051737762,6.21730575751372,38.5245015687808));
#41183=CARTESIAN_POINT('Ctrl Pts',(18.1230853481117,6.21872101409651,38.5458724250899));
#41184=CARTESIAN_POINT('Ctrl Pts',(18.1250122754564,6.21925554445668,38.5539073245145));
#41185=CARTESIAN_POINT('Ctrl Pts',(18.1285267788492,6.2202079998532,38.5681577620249));
#41186=CARTESIAN_POINT('Ctrl Pts',(18.1300938611968,6.22062526445002,38.5743782647217));
#41187=CARTESIAN_POINT('Ctrl Pts',(18.1334260860808,6.22149740723373,38.5873323682973));
#41188=CARTESIAN_POINT('Ctrl Pts',(18.1351967051138,6.22195245580394,38.5940644518317));
#41189=CARTESIAN_POINT('Ctrl Pts',(18.1398976831533,6.22313934278524,38.6115527440189));
#41190=CARTESIAN_POINT('Ctrl Pts',(18.1428848803213,6.22387299959467,38.6222932724997));
#41191=CARTESIAN_POINT('Ctrl Pts',(18.1564037328379,6.22710634532274,38.6693178346578));
#41192=CARTESIAN_POINT('Ctrl Pts',(18.1679062844646,6.22963714710759,38.7053117140126));
#41193=CARTESIAN_POINT('Ctrl Pts',(18.2017063989139,6.23654096026965,38.801265298302));
#41194=CARTESIAN_POINT('Ctrl Pts',(18.2259399042036,6.24097229274876,38.8604881714271));
#41195=CARTESIAN_POINT('Ctrl Pts',(18.2843857005264,6.25065853846148,38.9852458457732));
#41196=CARTESIAN_POINT('Ctrl Pts',(18.3195146560722,6.25592788052557,39.0502424464043));
#41197=CARTESIAN_POINT('Ctrl Pts',(18.4155554548618,6.26897584032833,39.2058814744104));
#41198=CARTESIAN_POINT('Ctrl Pts',(18.480607001194,6.27673412013774,39.2936871704458));
#41199=CARTESIAN_POINT('Ctrl Pts',(18.5588089938116,6.28468095471903,39.3824177556844));
#41200=CARTESIAN_POINT('Ctrl Pts',(18.5649275232683,6.28529451259804,39.3892609554051));
#41201=CARTESIAN_POINT('Ctrl Pts',(18.5741235995761,6.28620420562221,39.3993996196901));
#41202=CARTESIAN_POINT('Ctrl Pts',(18.5771641208377,6.28650297740116,39.4027282690302));
#41203=CARTESIAN_POINT('Ctrl Pts',(18.5826248340687,6.28703594744584,39.4086645300142));
#41204=CARTESIAN_POINT('Ctrl Pts',(18.5850405876477,6.28727046961003,39.4112761246983));
#41205=CARTESIAN_POINT('Ctrl Pts',(18.5902976961603,6.28777810565677,39.4169279733381));
#41206=CARTESIAN_POINT('Ctrl Pts',(18.5931416609419,6.28805101677287,39.4199657143436));
#41207=CARTESIAN_POINT('Ctrl Pts',(18.6011491802895,6.28881473758255,39.4284635542596));
#41208=CARTESIAN_POINT('Ctrl Pts',(18.6063349122859,6.2893038935846,39.4339027920374));
#41209=CARTESIAN_POINT('Ctrl Pts',(18.6375738094868,6.29221925231093,39.4662877640944));
#41210=CARTESIAN_POINT('Ctrl Pts',(18.6643779831421,6.29459144546651,39.4925019413635));
#41211=CARTESIAN_POINT('Ctrl Pts',(18.8118854198438,6.30708656797443,39.6285814363745));
#41212=CARTESIAN_POINT('Ctrl Pts',(18.9454059379836,6.31652146295659,39.7235822546358));
#41213=CARTESIAN_POINT('Ctrl Pts',(19.1602762438589,6.33132737354187,39.8386453368161));
#41214=CARTESIAN_POINT('Ctrl Pts',(19.2335471627387,6.33630939637897,39.8721656899719));
#41215=CARTESIAN_POINT('Ctrl Pts',(19.3210007377107,6.34229448586038,39.9057343108539));
#41216=CARTESIAN_POINT('Ctrl Pts',(19.3333578820995,6.34314091934746,39.9103327518375));
#41217=CARTESIAN_POINT('Ctrl Pts',(19.353478882323,6.34452081226978,39.9175863965942));
#41218=CARTESIAN_POINT('Ctrl Pts',(19.3612143839237,6.3450517035695,39.9203194219588));
#41219=CARTESIAN_POINT('Ctrl Pts',(19.3750038410649,6.34599888200213,39.9250926465547));
#41220=CARTESIAN_POINT('Ctrl Pts',(19.3810509771349,6.34641452366576,39.9271522850192));
#41221=CARTESIAN_POINT('Ctrl Pts',(19.3938014044893,6.3472915317714,39.9314244861788));
#41222=CARTESIAN_POINT('Ctrl Pts',(19.4005068201136,6.34775310989018,39.9336303637375));
#41223=CARTESIAN_POINT('Ctrl Pts',(19.4182545319478,6.34897583634393,39.9393610638052));
#41224=CARTESIAN_POINT('Ctrl Pts',(19.4293166143379,6.34973901202268,39.942823208032));
#41225=CARTESIAN_POINT('Ctrl Pts',(19.4809164504446,6.35330431016608,39.9584634588844));
#41226=CARTESIAN_POINT('Ctrl Pts',(19.5218140549906,6.35614598200241,39.9694041526698));
#41227=CARTESIAN_POINT('Ctrl Pts',(19.7257394025522,6.37040474666933,40.0168275346694));
#41228=CARTESIAN_POINT('Ctrl Pts',(19.8926510531193,6.38244064369203,40.0333661841339));
#41229=CARTESIAN_POINT('Ctrl Pts',(20.084132292508,6.39601778788669,40.0274513122304));
#41230=CARTESIAN_POINT('Ctrl Pts',(20.1086859465943,6.39775255875644,40.0262227895227));
#41231=CARTESIAN_POINT('Ctrl Pts',(20.1839352872724,6.40303891500762,40.021014248904));
#41232=CARTESIAN_POINT('Ctrl Pts',(20.234507149808,6.40654984343746,40.0154987229859));
#41233=CARTESIAN_POINT('Ctrl Pts',(20.2925005129333,6.41048567206385,40.0068420287788));
#41234=CARTESIAN_POINT('Ctrl Pts',(20.3001876062294,6.41100551834678,40.0056469974378));
#41235=CARTESIAN_POINT('Ctrl Pts',(20.3124524482004,6.41183175378452,40.0036642551742));
#41236=CARTESIAN_POINT('Ctrl Pts',(20.3170348469129,6.4121397408633,40.0029064705798));
#41237=CARTESIAN_POINT('Ctrl Pts',(20.3251441379302,6.41268345948663,40.0015353430346));
#41238=CARTESIAN_POINT('Ctrl Pts',(20.3286721138405,6.41291956321877,40.0009287239807));
#41239=CARTESIAN_POINT('Ctrl Pts',(20.3361617800509,6.41341983947269,39.9996194362067));
#41240=CARTESIAN_POINT('Ctrl Pts',(20.3401229617851,6.4136838653726,39.9989141940544));
#41241=CARTESIAN_POINT('Ctrl Pts',(20.3508590523441,6.41439800407227,39.9969680863164));
#41242=CARTESIAN_POINT('Ctrl Pts',(20.3576296493254,6.41484679211334,39.995703308153));
#41243=CARTESIAN_POINT('Ctrl Pts',(20.3920031054282,6.41711788613702,39.9890914799765));
#41244=CARTESIAN_POINT('Ctrl Pts',(20.4194951326837,6.41891021558487,39.9831773919318));
#41245=CARTESIAN_POINT('Ctrl Pts',(20.500634210205,6.42415471412786,39.9638574839136));
#41246=CARTESIAN_POINT('Ctrl Pts',(20.5538475661347,6.42753519603736,39.9487436672612));
#41247=CARTESIAN_POINT('Ctrl Pts',(20.7260955463525,6.43849555357931,39.8917144899666));
#41248=CARTESIAN_POINT('Ctrl Pts',(20.8416699216903,6.44589826019209,39.8404160061377));
#41249=CARTESIAN_POINT('Ctrl Pts',(20.9730659132591,6.45510858215605,39.7659246609078));
#41250=CARTESIAN_POINT('Ctrl Pts',(20.9944812377571,6.45663603130124,39.7532299446848));
#41251=CARTESIAN_POINT('Ctrl Pts',(21.0588621673574,6.46131908710018,39.7133621661541));
#41252=CARTESIAN_POINT('Ctrl Pts',(21.1010019702986,6.4645112798347,39.6849039496161));
#41253=CARTESIAN_POINT('Ctrl Pts',(21.152216244641,6.46858039504897,39.6472886020495));
#41254=CARTESIAN_POINT('Ctrl Pts',(21.1623912665049,6.46939854483727,39.6396593205907));
#41255=CARTESIAN_POINT('Ctrl Pts',(21.1783522365477,6.47069778003746,39.6274433089104));
#41256=CARTESIAN_POINT('Ctrl Pts',(21.1841886830538,6.47117627572589,39.6229229185147));
#41257=CARTESIAN_POINT('Ctrl Pts',(21.1949934417558,6.47206852959698,39.6144548516959));
#41258=CARTESIAN_POINT('Ctrl Pts',(21.1999685155384,6.47248193837844,39.6105159329763));
#41259=CARTESIAN_POINT('Ctrl Pts',(21.2109515732944,6.47340035410799,39.6017318053974));
#41260=CARTESIAN_POINT('Ctrl Pts',(21.2169500703856,6.47390582053495,39.596874961873));
#41261=CARTESIAN_POINT('Ctrl Pts',(21.2342373659457,6.47537390118965,39.582705245994));
#41262=CARTESIAN_POINT('Ctrl Pts',(21.2454493413206,6.47634022362391,39.573299915237));
#41263=CARTESIAN_POINT('Ctrl Pts',(21.3350452538048,6.48417929660206,39.4963874547551));
#41264=CARTESIAN_POINT('Ctrl Pts',(21.4079773607664,6.49130657952638,39.4228140938249));
#41265=CARTESIAN_POINT('Ctrl Pts',(21.5691750418778,6.50894102404585,39.2316918563823));
#41266=CARTESIAN_POINT('Ctrl Pts',(21.6506117544955,6.51958108201855,39.1092161832616));
#41267=CARTESIAN_POINT('Ctrl Pts',(21.7316093264231,6.53186055955177,38.9509090444608));
#41268=CARTESIAN_POINT('Ctrl Pts',(21.7451527554998,6.5339891562698,38.9227753002168));
#41269=CARTESIAN_POINT('Ctrl Pts',(21.7610493532698,6.53657473306921,38.887592713206));
#41270=CARTESIAN_POINT('Ctrl Pts',(21.764051843853,6.53706723884324,38.8808445447603));
#41271=CARTESIAN_POINT('Ctrl Pts',(21.7686919029858,6.53783475536267,38.870252531614));
#41272=CARTESIAN_POINT('Ctrl Pts',(21.7703558274569,6.53811131081077,38.8664204167139));
#41273=CARTESIAN_POINT('Ctrl Pts',(21.7734130145284,6.53862186502006,38.8593164573071));
#41274=CARTESIAN_POINT('Ctrl Pts',(21.7748096683001,6.53885606130442,38.8560461917807));
#41275=CARTESIAN_POINT('Ctrl Pts',(21.7779479273725,6.53938448183763,38.8486413370029));
#41276=CARTESIAN_POINT('Ctrl Pts',(21.7796841538721,6.53967838069398,38.84450453147));
#41277=CARTESIAN_POINT('Ctrl Pts',(21.784886732932,6.5405638858627,38.8319864529696));
#41278=CARTESIAN_POINT('Ctrl Pts',(21.7883084868077,6.54115288848041,38.8235866088795));
#41279=CARTESIAN_POINT('Ctrl Pts',(21.8282370117301,6.54810932172744,38.7235551423908));
#41280=CARTESIAN_POINT('Ctrl Pts',(21.8577290836442,6.554095747652,38.6292636440085));
#41281=CARTESIAN_POINT('Ctrl Pts',(21.9182577004232,6.57026759237785,38.366548313251));
#41282=CARTESIAN_POINT('Ctrl Pts',(21.9343237842355,6.58031252440966,38.1956380298044));
#41283=CARTESIAN_POINT('Ctrl Pts',(21.9268808664875,6.59243998359089,38.0047181805862));
#41284=CARTESIAN_POINT('Ctrl Pts',(21.9257806745749,6.59372798174598,37.984599637778));
#41285=CARTESIAN_POINT('Ctrl Pts',(21.9237961428244,6.59554796944844,37.9564148556313));
#41286=CARTESIAN_POINT('Ctrl Pts',(21.9231756988274,6.59607177819576,37.9483308832298));
#41287=CARTESIAN_POINT('Ctrl Pts',(21.9220093075626,6.59698454629142,37.9342938969484));
#41288=CARTESIAN_POINT('Ctrl Pts',(21.9214866114551,6.597372778139,37.9283390212939));
#41289=CARTESIAN_POINT('Ctrl Pts',(21.9203386528133,6.59818436631446,37.9159235338434));
#41290=CARTESIAN_POINT('Ctrl Pts',(21.9197084451105,6.59860787199287,37.9094634656307));
#41291=CARTESIAN_POINT('Ctrl Pts',(21.9181393054785,6.59961292899109,37.894177404606));
#41292=CARTESIAN_POINT('Ctrl Pts',(21.9171720459524,6.60019535717728,37.8853545300361));
#41293=CARTESIAN_POINT('Ctrl Pts',(21.9137434073348,6.60214409576965,37.8559545081229));
#41294=CARTESIAN_POINT('Ctrl Pts',(21.9110114139541,6.60351880772404,37.8354109784664));
#41295=CARTESIAN_POINT('Ctrl Pts',(21.8944252373989,6.61102023562796,37.7244065303495));
#41296=CARTESIAN_POINT('Ctrl Pts',(21.8744802719041,6.61733593801558,37.6349873096741));
#41297=CARTESIAN_POINT('Ctrl Pts',(21.8290520563024,6.62850910535385,37.4830633363604));
#41298=CARTESIAN_POINT('Ctrl Pts',(21.8064962470292,6.63329635554364,37.4198434506485));
#41299=CARTESIAN_POINT('Ctrl Pts',(21.7382113517549,6.64596207811006,37.2559849758262));
#41300=CARTESIAN_POINT('Ctrl Pts',(21.6870465986893,6.65382287075045,37.1578642603265));
#41301=CARTESIAN_POINT('Ctrl Pts',(21.6228529276574,6.66185894270065,37.0569398439116));
#41302=CARTESIAN_POINT('Ctrl Pts',(21.6178921769758,6.66246990713955,37.0492616758687));
#41303=CARTESIAN_POINT('Ctrl Pts',(21.610407764078,6.66337651834278,37.0378561088854));
#41304=CARTESIAN_POINT('Ctrl Pts',(21.6079254190054,6.66367477616622,37.034101946727));
#41305=CARTESIAN_POINT('Ctrl Pts',(21.6034576768009,6.66420719412797,37.0273963043614));
#41306=CARTESIAN_POINT('Ctrl Pts',(21.6014772412968,6.66444167530487,37.0244416075902));
#41307=CARTESIAN_POINT('Ctrl Pts',(21.597159029628,6.66494964071831,37.0180374525871));
#41308=CARTESIAN_POINT('Ctrl Pts',(21.5948182518101,6.66522291994315,37.014590093821));
#41309=CARTESIAN_POINT('Ctrl Pts',(21.5882098491243,6.66598871408783,37.0049251615507));
#41310=CARTESIAN_POINT('Ctrl Pts',(21.5839168519323,6.66647956085422,36.998724903855));
#41311=CARTESIAN_POINT('Ctrl Pts',(21.5578019877073,6.66942681066192,36.9614765330277));
#41312=CARTESIAN_POINT('Ctrl Pts',(21.5351025064472,6.67182781979418,36.9310502671716));
#41313=CARTESIAN_POINT('Ctrl Pts',(21.4068722995287,6.68467074625443,36.7693549997406));
#41314=CARTESIAN_POINT('Ctrl Pts',(21.2853906179317,6.69438597509941,36.6516602986869));
#41315=CARTESIAN_POINT('Ctrl Pts',(21.0898457991599,6.70922243218139,36.5064436146901));
#41316=CARTESIAN_POINT('Ctrl Pts',(21.026977675166,6.71388326505895,36.4652215265284));
#41317=CARTESIAN_POINT('Ctrl Pts',(20.9505947929873,6.71951462871796,36.421285808312));
#41318=CARTESIAN_POINT('Ctrl Pts',(20.9392528776285,6.72034993335725,36.4149137065468));
#41319=CARTESIAN_POINT('Ctrl Pts',(20.9207011621815,6.72171522934197,36.4047364900179));
#41320=CARTESIAN_POINT('Ctrl Pts',(20.9135300398068,6.72224274214559,36.4008614355108));
#41321=CARTESIAN_POINT('Ctrl Pts',(20.9007008892524,6.72318614104143,36.394033647902));
#41322=CARTESIAN_POINT('Ctrl Pts',(20.8950523276208,6.72360140062074,36.3910633084924));
#41323=CARTESIAN_POINT('Ctrl Pts',(20.8830996229841,6.72447993502907,36.3848534030222));
#41324=CARTESIAN_POINT('Ctrl Pts',(20.8767921698609,6.72494343330415,36.3816204488361));
#41325=CARTESIAN_POINT('Ctrl Pts',(20.8600067989423,6.72617669585088,36.3731334000601));
#41326=CARTESIAN_POINT('Ctrl Pts',(20.8494986980836,6.72694855056616,36.3679399837416));
#41327=CARTESIAN_POINT('Ctrl Pts',(20.7995298994961,6.7306185211545,36.3438080121611));
#41328=CARTESIAN_POINT('Ctrl Pts',(20.7594822495647,6.73355907401936,36.3261216090152));
#41329=CARTESIAN_POINT('Ctrl Pts',(20.5649423056006,6.7478520140779,36.2480018109363));
#41330=CARTESIAN_POINT('Ctrl Pts',(20.4037004351795,6.75980643622934,36.2063089830673));
#41331=CARTESIAN_POINT('Ctrl Pts',(20.2097082455715,6.77365943589982,36.1820725319764));
#41332=CARTESIAN_POINT('Ctrl Pts',(20.1801774725054,6.77575146542181,36.1790732646532));
#41333=CARTESIAN_POINT('Ctrl Pts',(20.105119644705,6.78101002760199,36.1731963022452));
#41334=CARTESIAN_POINT('Ctrl Pts',(20.0595346626624,6.78414930483095,36.1712493620381));
#41335=CARTESIAN_POINT('Ctrl Pts',(20.0063538130482,6.78771748109636,36.1708656267592));
#41336=CARTESIAN_POINT('Ctrl Pts',(19.9987876208153,6.78822290733504,36.1708555430706));
#41337=CARTESIAN_POINT('Ctrl Pts',(19.9866394294548,6.78903062921709,36.1709108244885));
#41338=CARTESIAN_POINT('Ctrl Pts',(19.9820574745272,6.78933441461749,36.1709479999817));
#41339=CARTESIAN_POINT('Ctrl Pts',(19.973904007766,6.78987340278675,36.1710432056767));
#41340=CARTESIAN_POINT('Ctrl Pts',(19.9703324782879,6.79010895503195,36.1710948301874));
#41341=CARTESIAN_POINT('Ctrl Pts',(19.9627011060732,6.7906110873571,36.1712263385148));
#41342=CARTESIAN_POINT('Ctrl Pts',(19.9586413729366,6.79087750527097,36.1713091202974));
#41343=CARTESIAN_POINT('Ctrl Pts',(19.9475285786086,6.79160491737153,36.1715708248523));
#41344=CARTESIAN_POINT('Ctrl Pts',(19.940476103195,6.7920645018859,36.1717756242876));
#41345=CARTESIAN_POINT('Ctrl Pts',(19.9031192317641,6.7944888001296,36.1730655966357));
#41346=CARTESIAN_POINT('Ctrl Pts',(19.8728404986087,6.79641849654678,36.1748265562644));
#41347=CARTESIAN_POINT('Ctrl Pts',(19.6900069828533,6.80792484381989,36.1897927338462));
#41348=CARTESIAN_POINT('Ctrl Pts',(19.5394462013061,6.81682141895203,36.2204072326804));
#41349=CARTESIAN_POINT('Ctrl Pts',(19.3941039843085,6.82605087843334,36.2684889912782));
#41350=CARTESIAN_POINT('Origin',(20.,-1.3495818343519,38.1));
#41351=CARTESIAN_POINT('',(19.3941040087786,7.78970911166913,36.2684889831831));
#41352=CARTESIAN_POINT('',(19.3941039249488,7.61899517246903,36.2684890109154));
#41353=CARTESIAN_POINT('',(19.3941040087494,-1.3495818343519,36.2684889831927));
#41354=CARTESIAN_POINT('Ctrl Pts',(19.3941040087786,7.78970911166913,36.2684889831831));
#41355=CARTESIAN_POINT('Ctrl Pts',(19.4230126969859,7.78774471398743,36.258925481716));
#41356=CARTESIAN_POINT('Ctrl Pts',(19.4521461268376,7.78581628133123,36.2500469832411));
#41357=CARTESIAN_POINT('Ctrl Pts',(19.6276793992675,7.77443388166182,36.2010638067059));
#41358=CARTESIAN_POINT('Ctrl Pts',(19.778196168021,7.76561309781924,36.1776592354544));
#41359=CARTESIAN_POINT('Ctrl Pts',(19.993800511059,7.75259056793529,36.1698209562425));
#41360=CARTESIAN_POINT('Ctrl Pts',(20.0577593062877,7.7486852247433,36.1706756581785));
#41361=CARTESIAN_POINT('Ctrl Pts',(20.1465170279916,7.74312723625945,36.176279399263));
#41362=CARTESIAN_POINT('Ctrl Pts',(20.1714460431282,7.74155115483903,36.178340728086));
#41363=CARTESIAN_POINT('Ctrl Pts',(20.2147597009781,7.73878222709422,36.1827717548401));
#41364=CARTESIAN_POINT('Ctrl Pts',(20.2331636391685,7.73759608322611,36.1849228337826));
#41365=CARTESIAN_POINT('Ctrl Pts',(20.2600533771323,7.7358477247745,36.1884590911738));
#41366=CARTESIAN_POINT('Ctrl Pts',(20.2685658146254,7.73529199963571,36.1896364732427));
#41367=CARTESIAN_POINT('Ctrl Pts',(20.2834466841576,7.73431645791239,36.1917961186455));
#41368=CARTESIAN_POINT('Ctrl Pts',(20.2898186365916,7.73389742750038,36.192753494751));
#41369=CARTESIAN_POINT('Ctrl Pts',(20.3021631373224,7.73308304861369,36.1946715273263));
#41370=CARTESIAN_POINT('Ctrl Pts',(20.3081362057648,7.7326878239966,36.1956283903512));
#41371=CARTESIAN_POINT('Ctrl Pts',(20.3223785646891,7.73174258593293,36.1979787224022));
#41372=CARTESIAN_POINT('Ctrl Pts',(20.3306434076751,7.73119176444531,36.1993980394044));
#41373=CARTESIAN_POINT('Ctrl Pts',(20.3603236649083,7.72920524485176,36.2046944670424));
#41374=CARTESIAN_POINT('Ctrl Pts',(20.3816816932292,7.72775988479655,36.2088799016885));
#41375=CARTESIAN_POINT('Ctrl Pts',(20.551998112266,7.71610235860834,36.245258706986));
#41376=CARTESIAN_POINT('Ctrl Pts',(20.6967076181939,7.70532324178521,36.2946335874514));
#41377=CARTESIAN_POINT('Ctrl Pts',(20.9078023955057,7.68861802501816,36.3958510862184));
#41378=CARTESIAN_POINT('Ctrl Pts',(20.979216010006,7.68278709749047,36.43585866317));
#41379=CARTESIAN_POINT('Ctrl Pts',(21.0778848972642,7.67464421960516,36.4996925540394));
#41380=CARTESIAN_POINT('Ctrl Pts',(21.1073482681718,7.67220138205543,36.5199367143199));
#41381=CARTESIAN_POINT('Ctrl Pts',(21.1422253643214,7.66931145066091,36.5453557538087));
#41382=CARTESIAN_POINT('Ctrl Pts',(21.1481913287944,7.66881717619672,36.5497567313529));
#41383=CARTESIAN_POINT('Ctrl Pts',(21.1574485520769,7.66805051947128,36.5566683640855));
#41384=CARTESIAN_POINT('Ctrl Pts',(21.1607572718816,7.66777656013919,36.5591553466708));
#41385=CARTESIAN_POINT('Ctrl Pts',(21.1668968388472,7.66726835928274,36.5638011203408));
#41386=CARTESIAN_POINT('Ctrl Pts',(21.1697296882758,7.66703393558903,36.565957077828));
#41387=CARTESIAN_POINT('Ctrl Pts',(21.1761607081506,7.66650188554795,36.5708796171302));
#41388=CARTESIAN_POINT('Ctrl Pts',(21.1797550877829,7.66620460378654,36.573651058704));
#41389=CARTESIAN_POINT('Ctrl Pts',(21.1907105251123,7.66529866200773,36.5821600527802));
#41390=CARTESIAN_POINT('Ctrl Pts',(21.1980398904273,7.66469278567903,36.5879384637449));
#41391=CARTESIAN_POINT('Ctrl Pts',(21.2686271188624,7.65885664728795,36.6444243296691));
#41392=CARTESIAN_POINT('Ctrl Pts',(21.328679728693,7.65388148180971,36.69902570664));
#41393=CARTESIAN_POINT('Ctrl Pts',(21.4991950218246,7.63909506227624,36.8749222947905));
#41394=CARTESIAN_POINT('Ctrl Pts',(21.5978002372821,7.62953592665228,37.0066406178803));
#41395=CARTESIAN_POINT('Ctrl Pts',(21.6979262792275,7.61685468145044,37.1834131199225));
#41396=CARTESIAN_POINT('Ctrl Pts',(21.7162338915729,7.61437157300214,37.2181689227193));
#41397=CARTESIAN_POINT('Ctrl Pts',(21.7384256352827,7.61112611704723,37.2636110058272));
#41398=CARTESIAN_POINT('Ctrl Pts',(21.7432947640213,7.61039796083964,37.2738077730408));
#41399=CARTESIAN_POINT('Ctrl Pts',(21.7510323788957,7.60921408339267,37.2903846047971));
#41400=CARTESIAN_POINT('Ctrl Pts',(21.7539562839535,7.60876026708288,37.2967386278816));
#41401=CARTESIAN_POINT('Ctrl Pts',(21.7594912811617,7.60788861732658,37.308941209074));
#41402=CARTESIAN_POINT('Ctrl Pts',(21.762107932661,7.60747098043067,37.3147871554894));
#41403=CARTESIAN_POINT('Ctrl Pts',(21.7680054797587,7.60651680382135,37.3281410020875));
#41404=CARTESIAN_POINT('Ctrl Pts',(21.7712677350643,7.60597964080494,37.335656951136));
#41405=CARTESIAN_POINT('Ctrl Pts',(21.7797567241083,7.60455665716292,37.355561054979));
#41406=CARTESIAN_POINT('Ctrl Pts',(21.7849019178352,7.60366811498294,37.3679832870108));
#41407=CARTESIAN_POINT('Ctrl Pts',(21.8232800470759,7.59683475678498,37.4634518742567));
#41408=CARTESIAN_POINT('Ctrl Pts',(21.850825779465,7.59070178190031,37.5486531220211));
#41409=CARTESIAN_POINT('Ctrl Pts',(21.9113620256374,7.57306914979581,37.7926417097495));
#41410=CARTESIAN_POINT('Ctrl Pts',(21.93041106278,7.56127227350689,37.954110541793));
#41411=CARTESIAN_POINT('Ctrl Pts',(21.9288120879362,7.54802517561317,38.1462245611227));
#41412=CARTESIAN_POINT('Ctrl Pts',(21.9278532836705,7.54597075764192,38.1763855181439));
#41413=CARTESIAN_POINT('Ctrl Pts',(21.9257983507026,7.54348046433386,38.2135468536062));
#41414=CARTESIAN_POINT('Ctrl Pts',(21.925370899014,7.54301109256027,38.2205781097167));
#41415=CARTESIAN_POINT('Ctrl Pts',(21.9246365057137,7.54227460081027,38.2316561641678));
#41416=CARTESIAN_POINT('Ctrl Pts',(21.924355297013,7.54200609495356,38.2357045183563));
#41417=CARTESIAN_POINT('Ctrl Pts',(21.9238025165188,7.54150256630001,38.243315025211));
#41418=CARTESIAN_POINT('Ctrl Pts',(21.9235338278765,7.54126739423347,38.2468772694404));
#41419=CARTESIAN_POINT('Ctrl Pts',(21.9228976054047,7.54073157685276,38.2550109285403));
#41420=CARTESIAN_POINT('Ctrl Pts',(21.9225236649204,7.54043129075335,38.2595817900932));
#41421=CARTESIAN_POINT('Ctrl Pts',(21.9214884661334,7.53963703787592,38.2717034716854));
#41422=CARTESIAN_POINT('Ctrl Pts',(21.9207989927734,7.53914459266156,38.2792518942869));
#41423=CARTESIAN_POINT('Ctrl Pts',(21.9156354300128,7.53569593464765,38.3323277917265));
#41424=CARTESIAN_POINT('Ctrl Pts',(21.9095872325823,7.53282036885576,38.3776916909528));
#41425=CARTESIAN_POINT('Ctrl Pts',(21.8969598457538,7.52816053162149,38.4520916390105));
#41426=CARTESIAN_POINT('Ctrl Pts',(21.891312511511,7.52634787714815,38.4812640697539));
#41427=CARTESIAN_POINT('Ctrl Pts',(21.8496300210549,7.51447880651155,38.6727632104032));
#41428=CARTESIAN_POINT('Ctrl Pts',(21.7934138616941,7.50480974887611,38.8299701959233));
#41429=CARTESIAN_POINT('Ctrl Pts',(21.6980519299293,7.49177164635131,39.0165329025731));
#41430=CARTESIAN_POINT('Ctrl Pts',(21.6770801214077,7.48904318534393,39.0543661448218));
#41431=CARTESIAN_POINT('Ctrl Pts',(21.6488557882827,7.48552071744568,39.1014756354968));
#41432=CARTESIAN_POINT('Ctrl Pts',(21.6427649132515,7.48476868932577,39.1114357562944));
#41433=CARTESIAN_POINT('Ctrl Pts',(21.6328370844093,7.48355548590444,39.1273440043834));
#41434=CARTESIAN_POINT('Ctrl Pts',(21.6290570830942,7.48309639493977,39.1333274724774));
#41435=CARTESIAN_POINT('Ctrl Pts',(21.6218049030694,7.48222087314776,39.1446684502722));
#41436=CARTESIAN_POINT('Ctrl Pts',(21.6183388804184,7.48180467344617,39.1500298001021));
#41437=CARTESIAN_POINT('Ctrl Pts',(21.6103768379123,7.48085359794733,39.1622126639468));
#41438=CARTESIAN_POINT('Ctrl Pts',(21.6058639924296,7.48031810175956,39.1690229828651));
#41439=CARTESIAN_POINT('Ctrl Pts',(21.5940187761205,7.47892161695727,39.1866542935384));
#41440=CARTESIAN_POINT('Ctrl Pts',(21.586619541847,7.4780581357376,39.1974296458053));
#41441=CARTESIAN_POINT('Ctrl Pts',(21.5350728529737,7.47210153402634,39.2708849824906));
#41442=CARTESIAN_POINT('Ctrl Pts',(21.4873381480004,7.46687179953347,39.3309520066939));
#41443=CARTESIAN_POINT('Ctrl Pts',(21.3247116535933,7.44989620428154,39.5122839007502));
#41444=CARTESIAN_POINT('Ctrl Pts',(21.1976178620949,7.43773581989172,39.6215487755451));
#41445=CARTESIAN_POINT('Ctrl Pts',(21.0264369449429,7.42352657459739,39.7338297968724));
#41446=CARTESIAN_POINT('Ctrl Pts',(20.9942104714587,7.42093818392172,39.7536379934182));
#41447=CARTESIAN_POINT('Ctrl Pts',(20.9548884581443,7.41790026069237,39.7762420311942));
#41448=CARTESIAN_POINT('Ctrl Pts',(20.9483348721752,7.41739786522942,39.7799584189666));
#41449=CARTESIAN_POINT('Ctrl Pts',(20.9381243182724,7.41662139101009,39.7856697986326));
#41450=CARTESIAN_POINT('Ctrl Pts',(20.9344824664119,7.41634567060427,39.7876914490923));
#41451=CARTESIAN_POINT('Ctrl Pts',(20.9277183437048,7.41583588100278,39.7914177146214));
#41452=CARTESIAN_POINT('Ctrl Pts',(20.9245979323305,7.41560161920572,39.7931254751081));
#41453=CARTESIAN_POINT('Ctrl Pts',(20.9175168784157,7.41507206632435,39.7969754298185));
#41454=CARTESIAN_POINT('Ctrl Pts',(20.9135534560911,7.41477710665685,39.7991123904749));
#41455=CARTESIAN_POINT('Ctrl Pts',(20.9015118714846,7.41388522189775,39.8055505439311));
#41456=CARTESIAN_POINT('Ctrl Pts',(20.8934104074271,7.41329095603541,39.8098082244071));
#41457=CARTESIAN_POINT('Ctrl Pts',(20.7875959009987,7.40560014134168,39.8644610173593));
#41458=CARTESIAN_POINT('Ctrl Pts',(20.6857626506532,7.39897702969677,39.9064791998961));
#41459=CARTESIAN_POINT('Ctrl Pts',(20.5004882688963,7.38735285650232,39.9649833880569));
#41460=CARTESIAN_POINT('Ctrl Pts',(20.4185096237902,7.38234690261566,39.9850731475136));
#41461=CARTESIAN_POINT('Ctrl Pts',(20.2593509724105,7.37254537929997,40.0131796453236));
#41462=CARTESIAN_POINT('Ctrl Pts',(20.1824884283243,7.3677761810364,40.0220341285599));
#41463=CARTESIAN_POINT('Ctrl Pts',(20.0863681876826,7.36165585469403,40.0272889954938));
#41464=CARTESIAN_POINT('Ctrl Pts',(20.0674149459046,7.36044174228542,40.0280449995559));
#41465=CARTESIAN_POINT('Ctrl Pts',(20.0398913045798,7.3586667876857,40.0287365319039));
#41466=CARTESIAN_POINT('Ctrl Pts',(20.0313272267653,7.35811284442608,40.0288946385582));
#41467=CARTESIAN_POINT('Ctrl Pts',(20.0163238336893,7.35713936671488,40.0290716812621));
#41468=CARTESIAN_POINT('Ctrl Pts',(20.0098849012368,7.35672060823672,40.0291154206134));
#41469=CARTESIAN_POINT('Ctrl Pts',(19.9973887161276,7.35590597034463,40.0291377421304));
#41470=CARTESIAN_POINT('Ctrl Pts',(19.9913315388288,7.35551021109596,40.0291200334071));
#41471=CARTESIAN_POINT('Ctrl Pts',(19.9768585878334,7.35456242449169,40.0290095555435));
#41472=CARTESIAN_POINT('Ctrl Pts',(19.9684431981106,7.35400957913339,40.0288902391794));
#41473=CARTESIAN_POINT('Ctrl Pts',(19.9380761385364,7.35200815222015,40.0282609071548));
#41474=CARTESIAN_POINT('Ctrl Pts',(19.9161334800788,7.35054971827324,40.0274311998574));
#41475=CARTESIAN_POINT('Ctrl Pts',(19.7456109979168,7.3391161381636,40.0180660080172));
#41476=CARTESIAN_POINT('Ctrl Pts',(19.5984827814038,7.32860336248275,39.9927382953995));
#41477=CARTESIAN_POINT('Ctrl Pts',(19.3460420923254,7.30982728066361,39.9185049272692));
#41478=CARTESIAN_POINT('Ctrl Pts',(19.2393999249786,7.30166031560354,39.8765456286366));
#41479=CARTESIAN_POINT('Ctrl Pts',(19.1267825489578,7.29316669671472,39.8202228854585));
#41480=CARTESIAN_POINT('Ctrl Pts',(19.1165166563092,7.29239384012503,39.814973087192));
#41481=CARTESIAN_POINT('Ctrl Pts',(19.1019149817705,7.29129722365943,39.807340129858));
#41482=CARTESIAN_POINT('Ctrl Pts',(19.0975405844668,7.29096904076219,39.8050319714454));
#41483=CARTESIAN_POINT('Ctrl Pts',(19.0899867307905,7.29040298210571,39.8010089522017));
#41484=CARTESIAN_POINT('Ctrl Pts',(19.0868031436998,7.29016461995074,39.7993019473119));
#41485=CARTESIAN_POINT('Ctrl Pts',(19.0801769267375,7.28966894987765,39.795725042058));
#41486=CARTESIAN_POINT('Ctrl Pts',(19.0767351891742,7.28941174175044,39.7938535928878));
#41487=CARTESIAN_POINT('Ctrl Pts',(19.0676755382886,7.28873528887928,39.7888915793258));
#41488=CARTESIAN_POINT('Ctrl Pts',(19.0620672317395,7.28831713989765,39.7857834361775));
#41489=CARTESIAN_POINT('Ctrl Pts',(19.0386555577091,7.28657368165367,39.7726556032465));
#41490=CARTESIAN_POINT('Ctrl Pts',(19.0209956565235,7.28526363540196,39.7623809672485));
#41491=CARTESIAN_POINT('Ctrl Pts',(18.8495753242944,7.27256392490519,39.6589681490693));
#41492=CARTESIAN_POINT('Ctrl Pts',(18.7093634829027,7.26223916762675,39.5450382152355));
#41493=CARTESIAN_POINT('Ctrl Pts',(18.5348842806202,7.24668935585623,39.3573091193895));
#41494=CARTESIAN_POINT('Ctrl Pts',(18.4862063126742,7.24196969904699,39.2982557971383));
#41495=CARTESIAN_POINT('Ctrl Pts',(18.4300544974328,7.2359089241463,39.2212356234614));
#41496=CARTESIAN_POINT('Ctrl Pts',(18.4191690306801,7.23470170576816,39.2058352547844));
#41497=CARTESIAN_POINT('Ctrl Pts',(18.4036816765768,7.23293500594798,39.1832282286636));
#41498=CARTESIAN_POINT('Ctrl Pts',(18.3988989299972,7.23238233227348,39.1761463398843));
#41499=CARTESIAN_POINT('Ctrl Pts',(18.390596921988,7.2314103227781,39.163675566912));
#41500=CARTESIAN_POINT('Ctrl Pts',(18.3870572560425,7.23099175567487,39.1583003742815));
#41501=CARTESIAN_POINT('Ctrl Pts',(18.3802354280521,7.23017692355542,39.1478272990366));
#41502=CARTESIAN_POINT('Ctrl Pts',(18.3769502672998,7.2297807760512,39.1427314519655));
#41503=CARTESIAN_POINT('Ctrl Pts',(18.3691505209555,7.2288311428582,39.1305065444558));
#41504=CARTESIAN_POINT('Ctrl Pts',(18.3646586127115,7.22827683193276,39.1233632320293));
#41505=CARTESIAN_POINT('Ctrl Pts',(18.3485719635192,7.22626443299498,39.0974048525123));
#41506=CARTESIAN_POINT('Ctrl Pts',(18.3372542684254,7.22479635076791,39.078420953867));
#41507=CARTESIAN_POINT('Ctrl Pts',(18.2538315067474,7.21356262649922,38.9328614891025));
#41508=CARTESIAN_POINT('Ctrl Pts',(18.1959591830902,7.20328439919121,38.7987014536748));
#41509=CARTESIAN_POINT('Ctrl Pts',(18.128606725356,7.18670973272714,38.5763850893056));
#41510=CARTESIAN_POINT('Ctrl Pts',(18.1090930374798,7.1805169530177,38.4918266803268));
#41511=CARTESIAN_POINT('Ctrl Pts',(18.089468470469,7.17194250095033,38.3697704880633));
#41512=CARTESIAN_POINT('Ctrl Pts',(18.0846531340135,7.16941577907992,38.3331387204966));
#41513=CARTESIAN_POINT('Ctrl Pts',(18.0801304978588,7.16644044969123,38.2889435349048));
#41514=CARTESIAN_POINT('Ctrl Pts',(18.0794119457004,7.16594142321738,38.2814940627911));
#41515=CARTESIAN_POINT('Ctrl Pts',(18.0783619472562,7.16516902052696,38.269902944553));
#41516=CARTESIAN_POINT('Ctrl Pts',(18.0780005072943,7.1648940295849,38.2657641914529));
#41517=CARTESIAN_POINT('Ctrl Pts',(18.0773543193479,7.16438490233174,38.2580784772877));
#41518=CARTESIAN_POINT('Ctrl Pts',(18.0770660172333,7.16415057773019,38.2545319273491));
#41519=CARTESIAN_POINT('Ctrl Pts',(18.0764339646257,7.1636200097953,38.2464809591786));
#41520=CARTESIAN_POINT('Ctrl Pts',(18.0760962226889,7.16332410325244,38.2419761265905));
#41521=CARTESIAN_POINT('Ctrl Pts',(18.0752621293534,7.16255961258323,38.230300977487));
#41522=CARTESIAN_POINT('Ctrl Pts',(18.0747900144612,7.16209233758744,38.2231289199796));
#41523=CARTESIAN_POINT('Ctrl Pts',(18.0720535910561,7.15914553965016,38.1776853798842));
#41524=CARTESIAN_POINT('Ctrl Pts',(18.0708903152333,7.15672246204862,38.1393531677313));
#41525=CARTESIAN_POINT('Ctrl Pts',(18.0707754377414,7.1430649112224,37.9196737203836));
#41526=CARTESIAN_POINT('Ctrl Pts',(18.0962469105642,7.1326570053055,37.7392203046852));
#41527=CARTESIAN_POINT('Ctrl Pts',(18.1638473325454,7.11769897865133,37.5050411594644));
#41528=CARTESIAN_POINT('Ctrl Pts',(18.1840397598923,7.11380488429277,37.445997082769));
#41529=CARTESIAN_POINT('Ctrl Pts',(18.2116104883321,7.10902623318341,37.3765652001304));
#41530=CARTESIAN_POINT('Ctrl Pts',(18.2162764396768,7.1082330330214,37.3651359281783));
#41531=CARTESIAN_POINT('Ctrl Pts',(18.2241265677736,7.10692306561753,37.3464223365102));
#41532=CARTESIAN_POINT('Ctrl Pts',(18.2272466940099,7.10640845094331,37.3391114042222));
#41533=CARTESIAN_POINT('Ctrl Pts',(18.2329449077133,7.10547925514718,37.325984933877));
#41534=CARTESIAN_POINT('Ctrl Pts',(18.23550675901,7.10506522834411,37.3201624382943));
#41535=CARTESIAN_POINT('Ctrl Pts',(18.2410339823489,7.10417977470255,37.3077670154533));
#41536=CARTESIAN_POINT('Ctrl Pts',(18.2440074969725,7.10370807562761,37.3011978467766));
#41537=CARTESIAN_POINT('Ctrl Pts',(18.2521436981349,7.10242973736881,37.2834881081571));
#41538=CARTESIAN_POINT('Ctrl Pts',(18.2573759618329,7.10162072896155,37.27238005624));
#41539=CARTESIAN_POINT('Ctrl Pts',(18.2847069418369,7.09745972558659,37.2157650187585));
#41540=CARTESIAN_POINT('Ctrl Pts',(18.3084816677062,7.0940502655181,37.1710938129257));
#41541=CARTESIAN_POINT('Ctrl Pts',(18.4255917714032,7.07813408772557,36.9704873588428));
#41542=CARTESIAN_POINT('Ctrl Pts',(18.5389110605227,7.06491952083453,36.8273021522816));
#41543=CARTESIAN_POINT('Ctrl Pts',(18.7076702204365,7.04859360054267,36.6668036412418));
#41544=CARTESIAN_POINT('Ctrl Pts',(18.7461954943087,7.0450547075126,36.632981468767));
#41545=CARTESIAN_POINT('Ctrl Pts',(18.7920828898353,7.04109136945516,36.5958259546593));
#41546=CARTESIAN_POINT('Ctrl Pts',(18.7981699951251,7.04057052010409,36.5909579369317));
#41547=CARTESIAN_POINT('Ctrl Pts',(18.8079347495209,7.03974299810826,36.5832453699829));
#41548=CARTESIAN_POINT('Ctrl Pts',(18.8115933892912,7.0394347198947,36.5803770540618));
#41549=CARTESIAN_POINT('Ctrl Pts',(18.8180879950552,7.03889067085551,36.5753231857247));
#41550=CARTESIAN_POINT('Ctrl Pts',(18.820919720074,7.03865452627345,36.5731322684188));
#41551=CARTESIAN_POINT('Ctrl Pts',(18.826944673017,7.03815436717077,36.5684974942798));
#41552=CARTESIAN_POINT('Ctrl Pts',(18.8301394429978,7.03789049823434,36.5660557366406));
#41553=CARTESIAN_POINT('Ctrl Pts',(18.8388183851344,7.0371772311926,36.5594653198336));
#41554=CARTESIAN_POINT('Ctrl Pts',(18.8443172075076,7.03672915234368,36.5553359167372));
#41555=CARTESIAN_POINT('Ctrl Pts',(18.8722988427606,7.03446772340112,36.5345558563376));
#41556=CARTESIAN_POINT('Ctrl Pts',(18.8951212230816,7.032684045757,36.5183652906138));
#41557=CARTESIAN_POINT('Ctrl Pts',(18.9637202267152,7.02747385495932,36.4719099168097));
#41558=CARTESIAN_POINT('Ctrl Pts',(19.0104468233388,7.02411792483307,36.4430936893475));
#41559=CARTESIAN_POINT('Ctrl Pts',(19.165318497745,7.01339605634237,36.3564768397933));
#41560=CARTESIAN_POINT('Ctrl Pts',(19.2777463335862,7.00619900177139,36.3069821443026));
#41561=CARTESIAN_POINT('Ctrl Pts',(19.394104010982,6.99874099840483,36.2684889824541));
#41562=CARTESIAN_POINT('',(18.0708706407966,6.98311453081294,38.1007530932072));
#41563=CARTESIAN_POINT('Ctrl Pts',(19.3941039843085,6.82605087843334,36.2684889912782));
#41564=CARTESIAN_POINT('Ctrl Pts',(19.3858528029974,6.82657484143018,36.2712186270038));
#41565=CARTESIAN_POINT('Ctrl Pts',(19.3776184331728,6.82709973804903,36.2740045622803));
#41566=CARTESIAN_POINT('Ctrl Pts',(19.2849251791949,6.83303300897787,36.3060656240963));
#41567=CARTESIAN_POINT('Ctrl Pts',(19.2025922685194,6.83854103777915,36.3411167380629));
#41568=CARTESIAN_POINT('Ctrl Pts',(19.1110112470517,6.84510809905579,36.3878602602958));
#41569=CARTESIAN_POINT('Ctrl Pts',(19.0990949656175,6.84597139340104,36.3941003559776));
#41570=CARTESIAN_POINT('Ctrl Pts',(19.0800254104803,6.84736764354507,36.4043418767981));
#41571=CARTESIAN_POINT('Ctrl Pts',(19.0728305429145,6.8478978580011,36.4082652363379));
#41572=CARTESIAN_POINT('Ctrl Pts',(19.060214048235,6.84883374352925,36.4152496673183));
#41573=CARTESIAN_POINT('Ctrl Pts',(19.0547817974993,6.8492387238008,36.4182913847059));
#41574=CARTESIAN_POINT('Ctrl Pts',(19.0434579570639,6.85008720746342,36.4247042196473));
#41575=CARTESIAN_POINT('Ctrl Pts',(19.0375692551277,6.85053088187969,36.4280802378942));
#41576=CARTESIAN_POINT('Ctrl Pts',(19.0255918218128,6.85143834971552,36.4350311981593));
#41577=CARTESIAN_POINT('Ctrl Pts',(19.0195046599771,6.85190222782742,36.43860862685));
#41578=CARTESIAN_POINT('Ctrl Pts',(19.0046459956348,6.85304121002375,36.4474511739059));
#41579=CARTESIAN_POINT('Ctrl Pts',(18.9958965524585,6.85371762520485,36.4527527579495));
#41580=CARTESIAN_POINT('Ctrl Pts',(18.9719116545613,6.85558793663787,36.4675481155321));
#41581=CARTESIAN_POINT('Ctrl Pts',(18.9567662206135,6.85678699571189,36.47718514733));
#41582=CARTESIAN_POINT('Ctrl Pts',(18.8305710747376,6.86693285706205,36.5599797255668));
#41583=CARTESIAN_POINT('Ctrl Pts',(18.7272441820305,6.87629880461213,36.6442159180892));
#41584=CARTESIAN_POINT('Ctrl Pts',(18.5488978627026,6.89432033860499,36.8232134784334));
#41585=CARTESIAN_POINT('Ctrl Pts',(18.4724541005455,6.90290581454265,36.9157322605341));
#41586=CARTESIAN_POINT('Ctrl Pts',(18.3968573039755,6.91201507984912,37.0268319732218));
#41587=CARTESIAN_POINT('Ctrl Pts',(18.3887734687498,6.91299822987586,37.0390074392153));
#41588=CARTESIAN_POINT('Ctrl Pts',(18.3777786216145,6.91434690562991,37.0559828397409));
#41589=CARTESIAN_POINT('Ctrl Pts',(18.3747492691931,6.91471974381913,37.0607050008008));
#41590=CARTESIAN_POINT('Ctrl Pts',(18.3699338963258,6.91531431801821,37.0682837583883));
#41591=CARTESIAN_POINT('Ctrl Pts',(18.3681347126011,6.91553690649327,37.0711318890301));
#41592=CARTESIAN_POINT('Ctrl Pts',(18.3643995069793,6.91599990077081,37.077079212767));
#41593=CARTESIAN_POINT('Ctrl Pts',(18.3624648219408,6.91624021331643,37.0801792066211));
#41594=CARTESIAN_POINT('Ctrl Pts',(18.3578078552176,6.91681992784397,37.0876886004259));
#41595=CARTESIAN_POINT('Ctrl Pts',(18.3550944831485,6.91715875069488,37.0921035508282));
#41596=CARTESIAN_POINT('Ctrl Pts',(18.3456651142437,6.91834011585873,37.1075856579283));
#41597=CARTESIAN_POINT('Ctrl Pts',(18.3390425719821,6.91917683939054,37.1187097346776));
#41598=CARTESIAN_POINT('Ctrl Pts',(18.3001090547877,6.9241437771133,37.185631064587));
#41599=CARTESIAN_POINT('Ctrl Pts',(18.2704965689311,6.9281241885141,37.2429588914674));
#41600=CARTESIAN_POINT('Ctrl Pts',(18.1696011057843,6.94292279780581,37.4649113805477));
#41601=CARTESIAN_POINT('Ctrl Pts',(18.118518246039,6.95330957281582,37.637694948239));
#41602=CARTESIAN_POINT('Ctrl Pts',(18.0868252863435,6.96673918983442,37.8499060277107));
#41603=CARTESIAN_POINT('Ctrl Pts',(18.0825762337671,6.96897078751891,37.8848945998393));
#41604=CARTESIAN_POINT('Ctrl Pts',(18.0782348999335,6.97195645029124,37.9312137384344));
#41605=CARTESIAN_POINT('Ctrl Pts',(18.0772804609192,6.97268365675433,37.9424580463212));
#41606=CARTESIAN_POINT('Ctrl Pts',(18.0758945872619,6.97386636712201,37.9606809615308));
#41607=CARTESIAN_POINT('Ctrl Pts',(18.075402333959,6.97431997309735,37.9676547864593));
#41608=CARTESIAN_POINT('Ctrl Pts',(18.0745479911337,6.97517517715424,37.9807733015578));
#41609=CARTESIAN_POINT('Ctrl Pts',(18.0741773809398,6.97557650453005,37.9869173642128));
#41610=CARTESIAN_POINT('Ctrl Pts',(18.0734923732556,6.97638407949335,37.9992558201496));
#41611=CARTESIAN_POINT('Ctrl Pts',(18.073178432564,6.97679033638118,38.0054501643088));
#41612=CARTESIAN_POINT('Ctrl Pts',(18.0725289063486,6.97772140725912,38.0196170787916));
#41613=CARTESIAN_POINT('Ctrl Pts',(18.072212906941,6.97824682371792,38.0275903909346));
#41614=CARTESIAN_POINT('Ctrl Pts',(18.071220412909,6.98020917223027,38.0572884063515));
#41615=CARTESIAN_POINT('Ctrl Pts',(18.0708616452603,6.98165587447813,38.0790212731587));
#41616=CARTESIAN_POINT('Ctrl Pts',(18.0708701476231,6.98311378152447,38.1007546975382));
#41617=CARTESIAN_POINT('Ctrl Pts',(18.0708701470186,6.98311367775493,38.1007531506166));
#41618=CARTESIAN_POINT('Ctrl Pts',(18.0709451226708,6.99599621466959,38.2927967682577));
#41619=CARTESIAN_POINT('Ctrl Pts',(18.0996985916395,7.00983650789902,38.4837380098122));
#41620=CARTESIAN_POINT('Ctrl Pts',(18.1775359073487,7.02858094791619,38.7367556225892));
#41621=CARTESIAN_POINT('Ctrl Pts',(18.2028404352395,7.03366187836658,38.8050199547983));
#41622=CARTESIAN_POINT('Ctrl Pts',(18.2354352276877,7.03913218367775,38.8796986002796));
#41623=CARTESIAN_POINT('Ctrl Pts',(18.2389811590489,7.03971525543524,38.887674673867));
#41624=CARTESIAN_POINT('Ctrl Pts',(18.2444029712373,7.04058864085328,38.8996506370724));
#41625=CARTESIAN_POINT('Ctrl Pts',(18.2462385951028,7.04088129764717,38.9036684667384));
#41626=CARTESIAN_POINT('Ctrl Pts',(18.2494314268578,7.04138508451765,38.9105939324495));
#41627=CARTESIAN_POINT('Ctrl Pts',(18.2507820980219,7.04159660737534,38.9135045079869));
#41628=CARTESIAN_POINT('Ctrl Pts',(18.253872949792,7.04207703553061,38.9201217276398));
#41629=CARTESIAN_POINT('Ctrl Pts',(18.2556176703331,7.04234565868894,38.9238262027469));
#41630=CARTESIAN_POINT('Ctrl Pts',(18.2603876043567,7.04307320154476,38.9338708645408));
#41631=CARTESIAN_POINT('Ctrl Pts',(18.263435711834,7.04353074276029,38.9402002038676));
#41632=CARTESIAN_POINT('Ctrl Pts',(18.2783620745301,7.04573665027384,38.9707662782485));
#41633=CARTESIAN_POINT('Ctrl Pts',(18.2907141940179,7.04745771292089,38.9947699535155));
#41634=CARTESIAN_POINT('Ctrl Pts',(18.4017574022293,7.06213277724415,39.1998606076852));
#41635=CARTESIAN_POINT('Ctrl Pts',(18.5283992585239,7.07383150893857,39.364313140902));
#41636=CARTESIAN_POINT('Ctrl Pts',(18.7040178810975,7.08872703666962,39.5293984731066));
#41637=CARTESIAN_POINT('Ctrl Pts',(18.7299694634229,7.09089665352579,39.5525053762315));
#41638=CARTESIAN_POINT('Ctrl Pts',(18.769034327419,7.09412821904715,39.585440534307));
#41639=CARTESIAN_POINT('Ctrl Pts',(18.7816722336872,7.09516857750915,39.5958233506788));
#41640=CARTESIAN_POINT('Ctrl Pts',(18.801927124806,7.09682895698293,39.612037007154));
#41641=CARTESIAN_POINT('Ctrl Pts',(18.8094583841522,7.09744481993309,39.6179740382746));
#41642=CARTESIAN_POINT('Ctrl Pts',(18.8236245114228,7.09860064406508,39.6289711861119));
#41643=CARTESIAN_POINT('Ctrl Pts',(18.8302485728027,7.09914005916544,39.6340449058181));
#41644=CARTESIAN_POINT('Ctrl Pts',(18.8419404748374,7.10009044353685,39.6428805934953));
#41645=CARTESIAN_POINT('Ctrl Pts',(18.8469942857584,7.1005006888193,39.6466609877271));
#41646=CARTESIAN_POINT('Ctrl Pts',(18.8568340599231,7.10129840730382,39.6539463890965));
#41647=CARTESIAN_POINT('Ctrl Pts',(18.8616178239336,7.10168576380203,39.6574542582801));
#41648=CARTESIAN_POINT('Ctrl Pts',(18.8740318279235,7.10268980871408,39.6664695286179));
#41649=CARTESIAN_POINT('Ctrl Pts',(18.881686250106,7.10330777787923,39.6719432114814));
#41650=CARTESIAN_POINT('Ctrl Pts',(18.9076056374896,7.10539680513369,39.6901930538897));
#41651=CARTESIAN_POINT('Ctrl Pts',(18.9260513321061,7.10687763623885,39.7027082018218));
#41652=CARTESIAN_POINT('Ctrl Pts',(19.0620143709475,7.11775512283747,39.7915561260047));
#41653=CARTESIAN_POINT('Ctrl Pts',(19.1873009218152,7.12762216127692,39.8551881107461));
#41654=CARTESIAN_POINT('Ctrl Pts',(19.3576475400654,7.14061115860368,39.9195304164095));
#41655=CARTESIAN_POINT('Ctrl Pts',(19.3974247670469,7.14361211671348,39.9330877674157));
#41656=CARTESIAN_POINT('Ctrl Pts',(19.4936432251052,7.15076111878538,39.9624114271104));
#41657=CARTESIAN_POINT('Ctrl Pts',(19.5504261981082,7.15489197747742,39.976927782616));
#41658=CARTESIAN_POINT('Ctrl Pts',(19.6363569591627,7.16093783703543,39.9947711799202));
#41659=CARTESIAN_POINT('Ctrl Pts',(19.6650613478746,7.16292352358157,40.0000553709158));
#41660=CARTESIAN_POINT('Ctrl Pts',(19.7007583214694,7.16534230290854,40.0057926326559));
#41661=CARTESIAN_POINT('Ctrl Pts',(19.7076462975802,7.16580669843896,40.0068614153111));
#41662=CARTESIAN_POINT('Ctrl Pts',(19.7185372774929,7.16653715221506,40.0084909295829));
#41663=CARTESIAN_POINT('Ctrl Pts',(19.7225364264193,7.16680455936949,40.009076441252));
#41664=CARTESIAN_POINT('Ctrl Pts',(19.7300770239457,7.16730719778903,40.0101562578836));
#41665=CARTESIAN_POINT('Ctrl Pts',(19.733617964495,7.16754257157321,40.0106532793601));
#41666=CARTESIAN_POINT('Ctrl Pts',(19.7417303601146,7.16808034151931,40.0117689792453));
#41667=CARTESIAN_POINT('Ctrl Pts',(19.7463026649192,7.16838236883808,40.0123811074555));
#41668=CARTESIAN_POINT('Ctrl Pts',(19.758484353295,7.16918429667777,40.0139675022851));
#41669=CARTESIAN_POINT('Ctrl Pts',(19.7660975214228,7.16968262842431,40.0149128028862));
#41670=CARTESIAN_POINT('Ctrl Pts',(19.821492170406,7.17328920535012,40.0214556697545));
#41671=CARTESIAN_POINT('Ctrl Pts',(19.8694670976077,7.17630816033769,40.0253100999269));
#41672=CARTESIAN_POINT('Ctrl Pts',(19.931403883757,7.18012862032513,40.0279599789975));
#41673=CARTESIAN_POINT('Ctrl Pts',(19.9452737255619,7.18097918049418,40.0284035254081));
#41674=CARTESIAN_POINT('Ctrl Pts',(20.0763372416713,7.18897930323712,40.0311796406608));
#41675=CARTESIAN_POINT('Ctrl Pts',(20.1935132412684,7.1958648121822,40.0229761317434));
#41676=CARTESIAN_POINT('Ctrl Pts',(20.3755218295595,7.20697510283853,39.9934194593316));
#41677=CARTESIAN_POINT('Ctrl Pts',(20.4412072872112,7.21106939490562,39.9791990006346));
#41678=CARTESIAN_POINT('Ctrl Pts',(20.5437210434686,7.21770155986098,39.9513338088674));
#41679=CARTESIAN_POINT('Ctrl Pts',(20.581105888455,7.22017225540584,39.9399415907366));
#41680=CARTESIAN_POINT('Ctrl Pts',(20.6288020949996,7.22340365428764,39.923808573504));
#41681=CARTESIAN_POINT('Ctrl Pts',(20.6394549708123,7.22413053792766,39.920100854069));
#41682=CARTESIAN_POINT('Ctrl Pts',(20.6566557872662,7.22531285188686,39.9139444851462));
#41683=CARTESIAN_POINT('Ctrl Pts',(20.6632241124896,7.22576638665549,39.9115532541511));
#41684=CARTESIAN_POINT('Ctrl Pts',(20.6757868369142,7.22663783912198,39.9069022514233));
#41685=CARTESIAN_POINT('Ctrl Pts',(20.6817832705229,7.22705556215035,39.9046482110165));
#41686=CARTESIAN_POINT('Ctrl Pts',(20.6954316454362,7.22801041352389,39.8994400966851));
#41687=CARTESIAN_POINT('Ctrl Pts',(20.7030761551102,7.22854816829931,39.8964670193599));
#41688=CARTESIAN_POINT('Ctrl Pts',(20.7232293359044,7.2299737510969,39.8884807746029));
#41689=CARTESIAN_POINT('Ctrl Pts',(20.7357046576024,7.23086431665249,39.8833852064625));
#41690=CARTESIAN_POINT('Ctrl Pts',(20.830525979133,7.23769649664952,39.8434910170851));
#41691=CARTESIAN_POINT('Ctrl Pts',(20.9104048294238,7.24382600958484,39.8031421497736));
#41692=CARTESIAN_POINT('Ctrl Pts',(21.126345242012,7.26145560671731,39.6745231123822));
#41693=CARTESIAN_POINT('Ctrl Pts',(21.2544989827452,7.27325312490255,39.5744509597995));
#41694=CARTESIAN_POINT('Ctrl Pts',(21.3898939094768,7.28649995315475,39.4381506157628));
#41695=CARTESIAN_POINT('Ctrl Pts',(21.4106454898574,7.28855364428785,39.4162567006065));
#41696=CARTESIAN_POINT('Ctrl Pts',(21.4356004539932,7.29104318179648,39.3886595753161));
#41697=CARTESIAN_POINT('Ctrl Pts',(21.4402958797064,7.29151250106591,39.3834095009929));
#41698=CARTESIAN_POINT('Ctrl Pts',(21.4476510550319,7.29224892866684,39.3750942891025));
#41699=CARTESIAN_POINT('Ctrl Pts',(21.4503300093345,7.29251742248839,39.3720463387847));
#41700=CARTESIAN_POINT('Ctrl Pts',(21.4553493182554,7.29302094048996,39.3662992067547));
#41701=CARTESIAN_POINT('Ctrl Pts',(21.4576917654595,7.29325611387016,39.3636020086775));
#41702=CARTESIAN_POINT('Ctrl Pts',(21.4630244268615,7.29379194932174,39.3574271818331));
#41703=CARTESIAN_POINT('Ctrl Pts',(21.4660097391147,7.29409225208356,39.353945388403));
#41704=CARTESIAN_POINT('Ctrl Pts',(21.4738963060659,7.29488657974326,39.3446805615358));
#41705=CARTESIAN_POINT('Ctrl Pts',(21.4787759994876,7.29537908261486,39.3388791584424));
#41706=CARTESIAN_POINT('Ctrl Pts',(21.5130216006856,7.29884399537533,39.297674382362));
#41707=CARTESIAN_POINT('Ctrl Pts',(21.5411499254214,7.30173484522444,39.2612562076873));
#41708=CARTESIAN_POINT('Ctrl Pts',(21.5851969229477,7.30640260330273,39.1998043172763));
#41709=CARTESIAN_POINT('Ctrl Pts',(21.6018867570773,7.30820849952043,39.1753500662346));
#41710=CARTESIAN_POINT('Ctrl Pts',(21.7087264647854,7.32008957529816,39.0107959576731));
#41711=CARTESIAN_POINT('Ctrl Pts',(21.7809613327102,7.32977717791028,38.8599164126599));
#41712=CARTESIAN_POINT('Ctrl Pts',(21.8462808818332,7.34281454240508,38.6609151748142));
#41713=CARTESIAN_POINT('Ctrl Pts',(21.8582840242908,7.34551865650919,38.6197681966811));
#41714=CARTESIAN_POINT('Ctrl Pts',(21.8717921112903,7.3490136989711,38.5669821409585));
#41715=CARTESIAN_POINT('Ctrl Pts',(21.8745754704882,7.34976345918943,38.5556806158579));
#41716=CARTESIAN_POINT('Ctrl Pts',(21.8788847448866,7.35097387502627,38.5374753150206));
#41717=CARTESIAN_POINT('Ctrl Pts',(21.8804753007679,7.35143246362559,38.5305870142263));
#41718=CARTESIAN_POINT('Ctrl Pts',(21.8834304582037,7.35230759950435,38.5174602323339));
#41719=CARTESIAN_POINT('Ctrl Pts',(21.8848020185533,7.35272391888372,38.5112234011923));
#41720=CARTESIAN_POINT('Ctrl Pts',(21.887860698522,7.35367607038993,38.4969779880783));
#41721=CARTESIAN_POINT('Ctrl Pts',(21.889527861157,7.35421252807334,38.4889652921254));
#41722=CARTESIAN_POINT('Ctrl Pts',(21.8937345861478,7.35561316221726,38.4680814945215));
#41723=CARTESIAN_POINT('Ctrl Pts',(21.8961938929825,7.35647985571269,38.4551948411967));
#41724=CARTESIAN_POINT('Ctrl Pts',(21.9124042379086,7.36254472456089,38.3652822091085));
#41725=CARTESIAN_POINT('Ctrl Pts',(21.9215876540301,7.36788540887421,38.287517058924));
#41726=CARTESIAN_POINT('Ctrl Pts',(21.9354059469477,7.38487899077248,38.044280527458));
#41727=CARTESIAN_POINT('Ctrl Pts',(21.9235109431242,7.39692556273527,37.8786416431793));
#41728=CARTESIAN_POINT('Ctrl Pts',(21.8831495853239,7.41101825561416,37.6796311612153));
#41729=CARTESIAN_POINT('Ctrl Pts',(21.8745792757848,7.41359709236386,37.6429274420165));
#41730=CARTESIAN_POINT('Ctrl Pts',(21.8630132651908,7.41662532754928,37.5992198355335));
#41731=CARTESIAN_POINT('Ctrl Pts',(21.8610453548205,7.41712720679983,37.5919553254992));
#41732=CARTESIAN_POINT('Ctrl Pts',(21.8579227787256,7.41790305680837,37.5806900338326));
#41733=CARTESIAN_POINT('Ctrl Pts',(21.8567976164936,7.41817866508047,37.5766812588244));
#41734=CARTESIAN_POINT('Ctrl Pts',(21.8546870762952,7.41868835174971,37.5692542410238));
#41735=CARTESIAN_POINT('Ctrl Pts',(21.8537052306787,7.41892262209014,37.5658351099622));
#41736=CARTESIAN_POINT('Ctrl Pts',(21.8514585354851,7.4194523266521,37.5580921270005));
#41737=CARTESIAN_POINT('Ctrl Pts',(21.8501879969507,7.41974742864587,37.5537699858152));
#41738=CARTESIAN_POINT('Ctrl Pts',(21.8462873501272,7.42064017400587,37.5406704584045));
#41739=CARTESIAN_POINT('Ctrl Pts',(21.8436097897944,7.42123515059807,37.5319071674792));
#41740=CARTESIAN_POINT('Ctrl Pts',(21.808117864894,7.42890006571124,37.4186411624404));
#41741=CARTESIAN_POINT('Ctrl Pts',(21.7665180241971,7.43550018066607,37.3170813538788));
#41742=CARTESIAN_POINT('Ctrl Pts',(21.6783718978196,7.4470564462287,37.1452250043875));
#41743=CARTESIAN_POINT('Ctrl Pts',(21.6354378095822,7.4520184438928,37.0734181698498));
#41744=CARTESIAN_POINT('Ctrl Pts',(21.5435486302553,7.46182775610449,36.9402049872904));
#41745=CARTESIAN_POINT('Ctrl Pts',(21.4952393446977,7.46665292326438,36.8785565830981));
#41746=CARTESIAN_POINT('Ctrl Pts',(21.4306574021558,7.47284053338721,36.8057332562141));
#41747=CARTESIAN_POINT('Ctrl Pts',(21.417779815532,7.47406239039933,36.7916394382466));
#41748=CARTESIAN_POINT('Ctrl Pts',(21.3988092978767,7.47584661267469,36.7714862229735));
#41749=CARTESIAN_POINT('Ctrl Pts',(21.3928814395482,7.47640197587688,36.7652724626271));
#41750=CARTESIAN_POINT('Ctrl Pts',(21.3824342476616,7.47737709711229,36.7544667916662));
#41751=CARTESIAN_POINT('Ctrl Pts',(21.3779329992399,7.4777960710417,36.7498575216788));
#41752=CARTESIAN_POINT('Ctrl Pts',(21.3691596018897,7.47861049875699,36.7409631520696));
#41753=CARTESIAN_POINT('Ctrl Pts',(21.3648902094779,7.4790058294298,36.7366754296384));
#41754=CARTESIAN_POINT('Ctrl Pts',(21.3546515772088,7.47995157623165,36.7264891388185));
#41755=CARTESIAN_POINT('Ctrl Pts',(21.3486639215867,7.48050280239419,36.7206093358758));
#41756=CARTESIAN_POINT('Ctrl Pts',(21.326982973375,7.48249228792233,36.6995950315257));
#41757=CARTESIAN_POINT('Ctrl Pts',(21.3110722399557,7.48394024694469,36.6846882311464));
#41758=CARTESIAN_POINT('Ctrl Pts',(21.1824184618211,7.49555857838946,36.5681834691844));
#41759=CARTESIAN_POINT('Ctrl Pts',(21.0583168501463,7.5062906466541,36.4799619870505));
#41760=CARTESIAN_POINT('Ctrl Pts',(20.8530483154411,7.52298307926174,36.3677727958251));
#41761=CARTESIAN_POINT('Ctrl Pts',(20.778450239649,7.52884716119518,36.3329913917537));
#41762=CARTESIAN_POINT('Ctrl Pts',(20.6684626299568,7.53702977321516,36.2900316223206));
#41763=CARTESIAN_POINT('Ctrl Pts',(20.6347091761776,7.53948047198674,36.2779208355744));
#41764=CARTESIAN_POINT('Ctrl Pts',(20.5935839753904,7.54237841826551,36.2644467648996));
#41765=CARTESIAN_POINT('Ctrl Pts',(20.5865192814805,7.54287314567127,36.2621771707859));
#41766=CARTESIAN_POINT('Ctrl Pts',(20.5754921552711,7.54364034976065,36.2587046732253));
#41767=CARTESIAN_POINT('Ctrl Pts',(20.5715387422013,7.5439144070902,36.2574736994701));
#41768=CARTESIAN_POINT('Ctrl Pts',(20.5641791091952,7.54442269467029,36.2552080979581));
#41769=CARTESIAN_POINT('Ctrl Pts',(20.5607740206233,7.54465710767688,36.2541701792394));
#41770=CARTESIAN_POINT('Ctrl Pts',(20.5530228441907,7.54518901183027,36.2518309407373));
#41771=CARTESIAN_POINT('Ctrl Pts',(20.5486750336585,7.54548615914995,36.2505355244583));
#41772=CARTESIAN_POINT('Ctrl Pts',(20.5353790266784,7.54639128627431,36.2466250347177));
#41773=CARTESIAN_POINT('Ctrl Pts',(20.5264162470188,7.54699648967387,36.2440594278164));
#41774=CARTESIAN_POINT('Ctrl Pts',(20.4403978630993,7.55276072658779,36.2201098276846));
#41775=CARTESIAN_POINT('Ctrl Pts',(20.3620909182083,7.55767164189551,36.2034687248536));
#41776=CARTESIAN_POINT('Ctrl Pts',(20.1202135927457,7.57243785141414,36.1676018583233));
#41777=CARTESIAN_POINT('Ctrl Pts',(19.9550508868086,7.58202967028628,36.1643882268082));
#41778=CARTESIAN_POINT('Ctrl Pts',(19.7520416458881,7.59477220980439,36.1864605562292));
#41779=CARTESIAN_POINT('Ctrl Pts',(19.7127445987153,7.59727992024078,36.1919642210437));
#41780=CARTESIAN_POINT('Ctrl Pts',(19.6624717017945,7.60055322058162,36.2005933094492));
#41781=CARTESIAN_POINT('Ctrl Pts',(19.6513135329234,7.60128387631829,36.2026099855445));
#41782=CARTESIAN_POINT('Ctrl Pts',(19.6332937046177,7.60247082253156,36.2060311263591));
#41783=CARTESIAN_POINT('Ctrl Pts',(19.6264206683724,7.60292518959078,36.2073748172886));
#41784=CARTESIAN_POINT('Ctrl Pts',(19.6132785022379,7.60379722409308,36.2100185104325));
#41785=CARTESIAN_POINT('Ctrl Pts',(19.6070082179981,7.60421469129771,36.2113123589736));
#41786=CARTESIAN_POINT('Ctrl Pts',(19.5927455496838,7.60516754715848,36.2143295046778));
#41787=CARTESIAN_POINT('Ctrl Pts',(19.5847574899224,7.60570355301937,36.2160724380727));
#41788=CARTESIAN_POINT('Ctrl Pts',(19.5637203264854,7.6071214662114,36.2208028827239));
#41789=CARTESIAN_POINT('Ctrl Pts',(19.5506910091764,7.60800606408194,36.2238754906501));
#41790=CARTESIAN_POINT('Ctrl Pts',(19.4892970214218,7.61220539181532,36.2390297946192));
#41791=CARTESIAN_POINT('Ctrl Pts',(19.4413979263548,7.61557396157359,36.2528433227398));
#41792=CARTESIAN_POINT('Ctrl Pts',(19.3941039249488,7.61899517246903,36.2684890109154));
#41793=CARTESIAN_POINT('Origin',(20.,-1.3495818343519,38.1));
#41794=CARTESIAN_POINT('',(19.3941041019635,8.58595480644739,36.2684889523559));
#41795=CARTESIAN_POINT('',(19.3941040078119,8.41575742730426,36.2684889835028));
#41796=CARTESIAN_POINT('',(19.3941040087494,-1.3495818343519,36.2684889831927));
#41797=CARTESIAN_POINT('',(18.0708707679468,7.94955926345013,38.0982625861522));
#41798=CARTESIAN_POINT('Ctrl Pts',(19.3941041019635,8.58595480644739,36.2684889523559));
#41799=CARTESIAN_POINT('Ctrl Pts',(19.5043238617899,8.57774700749365,36.232026327439));
#41800=CARTESIAN_POINT('Ctrl Pts',(19.6176380959992,8.56937247835458,36.2055779375375));
#41801=CARTESIAN_POINT('Ctrl Pts',(19.7850254076397,8.55751279271299,36.1821568103993));
#41802=CARTESIAN_POINT('Ctrl Pts',(19.837658427954,8.5538586227368,36.1769859789215));
#41803=CARTESIAN_POINT('Ctrl Pts',(19.899036483125,8.5497314476424,36.1734946084228));
#41804=CARTESIAN_POINT('Ctrl Pts',(19.9076340194586,8.54915639541592,36.1730632631204));
#41805=CARTESIAN_POINT('Ctrl Pts',(19.9206797789185,8.54828875176964,36.1724962623643));
#41806=CARTESIAN_POINT('Ctrl Pts',(19.925125919035,8.5479939174509,36.1723184316234));
#41807=CARTESIAN_POINT('Ctrl Pts',(19.9331241524775,8.54746514442149,36.172026243011));
#41808=CARTESIAN_POINT('Ctrl Pts',(19.9366759626202,8.54723090377612,36.1719063161892));
#41809=CARTESIAN_POINT('Ctrl Pts',(19.9444328203213,8.54672059747401,36.1716658636416));
#41810=CARTESIAN_POINT('Ctrl Pts',(19.948637926966,8.54644475234078,36.1715492769608));
#41811=CARTESIAN_POINT('Ctrl Pts',(19.9605663728216,8.5456644564136,36.1712576052149));
#41812=CARTESIAN_POINT('Ctrl Pts',(19.9682905379219,8.54516177653989,36.1711151534359));
#41813=CARTESIAN_POINT('Ctrl Pts',(20.017461461831,8.54197711599725,36.1705037738062));
#41814=CARTESIAN_POINT('Ctrl Pts',(20.0589169041221,8.53936141876005,36.1713242933359));
#41815=CARTESIAN_POINT('Ctrl Pts',(20.2079179135493,8.53010681927217,36.1790830263577));
#41816=CARTESIAN_POINT('Ctrl Pts',(20.3148688809859,8.52373175893408,36.1936911955294));
#41817=CARTESIAN_POINT('Ctrl Pts',(20.5473984682729,8.50948737417836,36.2455666793631));
#41818=CARTESIAN_POINT('Ctrl Pts',(20.671519263033,8.50160823850721,36.2868196307428));
#41819=CARTESIAN_POINT('Ctrl Pts',(20.8030862588113,8.49240019764376,36.345923366389));
#41820=CARTESIAN_POINT('Ctrl Pts',(20.8155927443807,8.49151624699186,36.3517034475761));
#41821=CARTESIAN_POINT('Ctrl Pts',(20.8355243352645,8.49009305184941,36.3611755747837));
#41822=CARTESIAN_POINT('Ctrl Pts',(20.8429895623312,8.48955672380164,36.36478246585));
#41823=CARTESIAN_POINT('Ctrl Pts',(20.8561929276389,8.48860220064429,36.3712671020124));
#41824=CARTESIAN_POINT('Ctrl Pts',(20.8619404243843,8.48818467592202,36.3741255940601));
#41825=CARTESIAN_POINT('Ctrl Pts',(20.8738790821723,8.48731313620537,36.3801377433142));
#41826=CARTESIAN_POINT('Ctrl Pts',(20.8800676765594,8.48685895650295,36.383296264702));
#41827=CARTESIAN_POINT('Ctrl Pts',(20.8960886652151,8.48567684880896,36.3915824196914));
#41828=CARTESIAN_POINT('Ctrl Pts',(20.9058940384917,8.48494712963843,36.3967614650363));
#41829=CARTESIAN_POINT('Ctrl Pts',(20.9484084422549,8.48175550116334,36.4196878792799));
#41830=CARTESIAN_POINT('Ctrl Pts',(20.9806428129817,8.47926346246601,36.4382940256709));
#41831=CARTESIAN_POINT('Ctrl Pts',(21.0655832083181,8.47249507451684,36.4906552785584));
#41832=CARTESIAN_POINT('Ctrl Pts',(21.1172150874565,8.46816320792328,36.526060000138));
#41833=CARTESIAN_POINT('Ctrl Pts',(21.2768268029229,8.4540822400479,36.6473234756515));
#41834=CARTESIAN_POINT('Ctrl Pts',(21.3773552268127,8.44409944195503,36.7422645013639));
#41835=CARTESIAN_POINT('Ctrl Pts',(21.4982057141647,8.43108015010229,36.8837576728504));
#41836=CARTESIAN_POINT('Ctrl Pts',(21.5281279916781,8.42775725084318,36.9215724488586));
#41837=CARTESIAN_POINT('Ctrl Pts',(21.5611384527053,8.42400694206373,36.9666650110812));
#41838=CARTESIAN_POINT('Ctrl Pts',(21.5656352515864,8.42349412976692,36.9728852190596));
#41839=CARTESIAN_POINT('Ctrl Pts',(21.5727758183025,8.42267691897157,36.9828876186431));
#41840=CARTESIAN_POINT('Ctrl Pts',(21.5754432915877,8.42237097572814,36.9866526672662));
#41841=CARTESIAN_POINT('Ctrl Pts',(21.580153945673,8.42182956483748,36.9933524268374));
#41842=CARTESIAN_POINT('Ctrl Pts',(21.5822025049234,8.42159373604685,36.9962832893163));
#41843=CARTESIAN_POINT('Ctrl Pts',(21.5865488342371,8.42109258842567,37.002538527402));
#41844=CARTESIAN_POINT('Ctrl Pts',(21.5888443081796,8.42082742366053,37.0058644268811));
#41845=CARTESIAN_POINT('Ctrl Pts',(21.5950689002712,8.42010697281708,37.0149441013281));
#41846=CARTESIAN_POINT('Ctrl Pts',(21.5989773733471,8.41965305159049,37.0207120574181));
#41847=CARTESIAN_POINT('Ctrl Pts',(21.6190712611747,8.41731061792136,37.0507144936513));
#41848=CARTESIAN_POINT('Ctrl Pts',(21.6347382666792,8.41545437735998,37.0752937763059));
#41849=CARTESIAN_POINT('Ctrl Pts',(21.6801363133684,8.40995273702522,37.1502099358469));
#41850=CARTESIAN_POINT('Ctrl Pts',(21.7081441322808,8.40638759226898,37.2015547359169));
#41851=CARTESIAN_POINT('Ctrl Pts',(21.776756512613,8.39695350711334,37.3421837899237));
#41852=CARTESIAN_POINT('Ctrl Pts',(21.8129586838587,8.39116609073237,37.4334189104684));
#41853=CARTESIAN_POINT('Ctrl Pts',(21.8704881540301,8.37947960255212,37.6183672151824));
#41854=CARTESIAN_POINT('Ctrl Pts',(21.892066264344,8.37360205581332,37.7116990205948));
#41855=CARTESIAN_POINT('Ctrl Pts',(21.9087027030294,8.36662561413914,37.819676234784));
#41856=CARTESIAN_POINT('Ctrl Pts',(21.9106309678426,8.36575311868281,37.8331354061458));
#41857=CARTESIAN_POINT('Ctrl Pts',(21.9134987862395,8.36434486056527,37.8547800690763));
#41858=CARTESIAN_POINT('Ctrl Pts',(21.9145284757811,8.36381191662194,37.8629533138285));
#41859=CARTESIAN_POINT('Ctrl Pts',(21.9162663855726,8.36286127988631,37.877498763052));
#41860=CARTESIAN_POINT('Ctrl Pts',(21.9169952520846,8.36244423875731,37.8838684133398));
#41861=CARTESIAN_POINT('Ctrl Pts',(21.9184505209835,8.36157153711125,37.8971730385672));
#41862=CARTESIAN_POINT('Ctrl Pts',(21.9191711005266,8.36111570112041,37.9041085440699));
#41863=CARTESIAN_POINT('Ctrl Pts',(21.9209512196792,8.35992449192634,37.922195487088));
#41864=CARTESIAN_POINT('Ctrl Pts',(21.9219512473859,8.35918727559492,37.9333523869684));
#41865=CARTESIAN_POINT('Ctrl Pts',(21.9259410720916,8.35591574765227,37.9826944939233));
#41866=CARTESIAN_POINT('Ctrl Pts',(21.9278902407265,8.35334940818683,38.0209527923013));
#41867=CARTESIAN_POINT('Ctrl Pts',(21.9300777005635,8.34632041394812,38.1244639282722));
#41868=CARTESIAN_POINT('Ctrl Pts',(21.9281466273671,8.34179677456824,38.1897079067705));
#41869=CARTESIAN_POINT('Ctrl Pts',(21.9119630759648,8.32759887338222,38.3908385600846));
#41870=CARTESIAN_POINT('Ctrl Pts',(21.8865905501917,8.31771292971884,38.5253986675655));
#41871=CARTESIAN_POINT('Ctrl Pts',(21.8340415134774,8.30498030128192,38.6999379413452));
#41872=CARTESIAN_POINT('Ctrl Pts',(21.8193038167707,8.30183233295177,38.7432481670721));
#41873=CARTESIAN_POINT('Ctrl Pts',(21.800344524941,8.29825506306183,38.793079772646));
#41874=CARTESIAN_POINT('Ctrl Pts',(21.7976081074813,8.2977488385694,38.8001464677335));
#41875=CARTESIAN_POINT('Ctrl Pts',(21.793149068082,8.29694009020383,38.8114632833104));
#41876=CARTESIAN_POINT('Ctrl Pts',(21.79145284255,8.29663607067478,38.8157236183458));
#41877=CARTESIAN_POINT('Ctrl Pts',(21.7884081912497,8.29609681990817,38.8232920984344));
#41878=CARTESIAN_POINT('Ctrl Pts',(21.7870657502158,8.29586123793041,38.8266025897227));
#41879=CARTESIAN_POINT('Ctrl Pts',(21.78417854837,8.29535921432831,38.8336660922654));
#41880=CARTESIAN_POINT('Ctrl Pts',(21.7826311408557,8.29509293398203,38.8374179573399));
#41881=CARTESIAN_POINT('Ctrl Pts',(21.7783650062004,8.2943662885714,38.8476697811219));
#41882=CARTESIAN_POINT('Ctrl Pts',(21.7756224589712,8.29390732820784,38.8541598529635));
#41883=CARTESIAN_POINT('Ctrl Pts',(21.7609405293519,8.29149223060244,38.8883796567442));
#41884=CARTESIAN_POINT('Ctrl Pts',(21.7483862181402,8.28957079612882,38.9158430666385));
#41885=CARTESIAN_POINT('Ctrl Pts',(21.6644354330777,8.27751898720139,39.088642953745));
#41886=CARTESIAN_POINT('Ctrl Pts',(21.5756181452756,8.2681481117834,39.2248110979603));
#41887=CARTESIAN_POINT('Ctrl Pts',(21.4129456956631,8.25294054682854,39.4164826332059));
#41888=CARTESIAN_POINT('Ctrl Pts',(21.3504064705224,8.24742933032817,39.480558327958));
#41889=CARTESIAN_POINT('Ctrl Pts',(21.2736175760321,8.24085919584937,39.5490071091366));
#41890=CARTESIAN_POINT('Ctrl Pts',(21.2634878760538,8.23999627543739,39.5578483133369));
#41891=CARTESIAN_POINT('Ctrl Pts',(21.2470379612693,8.23860051268736,39.5719055713394));
#41892=CARTESIAN_POINT('Ctrl Pts',(21.2407753675681,8.23807040856352,39.5771886039425));
#41893=CARTESIAN_POINT('Ctrl Pts',(21.2295576066806,8.23712301863193,39.5865300773592));
#41894=CARTESIAN_POINT('Ctrl Pts',(21.2246154948986,8.23670636880961,39.5906040611266));
#41895=CARTESIAN_POINT('Ctrl Pts',(21.2142339902983,8.23583262089247,39.5990754809065));
#41896=CARTESIAN_POINT('Ctrl Pts',(21.2087907949658,8.23537533804722,39.6034680882857));
#41897=CARTESIAN_POINT('Ctrl Pts',(21.1944918067681,8.23417618426676,39.6148793901517));
#41898=CARTESIAN_POINT('Ctrl Pts',(21.1855981266558,8.2334324244053,39.6218499650206));
#41899=CARTESIAN_POINT('Ctrl Pts',(21.1455179644657,8.23008942259485,39.6526989121731));
#41900=CARTESIAN_POINT('Ctrl Pts',(21.113669740123,8.22745640142304,39.6756981461338));
#41901=CARTESIAN_POINT('Ctrl Pts',(20.9453939377219,8.21365157496461,39.7895677101796));
#41902=CARTESIAN_POINT('Ctrl Pts',(20.7985066684081,8.20187442244596,39.8637397452433));
#41903=CARTESIAN_POINT('Ctrl Pts',(20.5676366157588,8.18447987720601,39.9455089633555));
#41904=CARTESIAN_POINT('Ctrl Pts',(20.4895794820079,8.17878937098991,39.9677338732078));
#41905=CARTESIAN_POINT('Ctrl Pts',(20.4012275441371,8.17271228961747,39.9869674389053));
#41906=CARTESIAN_POINT('Ctrl Pts',(20.3920938312977,8.17208834801149,39.988886469251));
#41907=CARTESIAN_POINT('Ctrl Pts',(20.3784979744386,8.17116632810962,39.9916401454374));
#41908=CARTESIAN_POINT('Ctrl Pts',(20.374046397906,8.17086550965605,39.9925254158779));
#41909=CARTESIAN_POINT('Ctrl Pts',(20.3660976824715,8.17033032891322,39.9940770092554));
#41910=CARTESIAN_POINT('Ctrl Pts',(20.3626017936172,8.17009563135596,39.994749368672));
#41911=CARTESIAN_POINT('Ctrl Pts',(20.3550371918124,8.16958925218407,39.9961825549488));
#41912=CARTESIAN_POINT('Ctrl Pts',(20.350967894551,8.16931776459893,39.9969399640085));
#41913=CARTESIAN_POINT('Ctrl Pts',(20.3396035262588,8.16856204734921,39.9990173672848));
#41914=CARTESIAN_POINT('Ctrl Pts',(20.3323031407572,8.16807941608292,40.0003084337238));
#41915=CARTESIAN_POINT('Ctrl Pts',(20.2897666433618,8.16528284560933,40.0075783503781));
#41916=CARTESIAN_POINT('Ctrl Pts',(20.2543746645343,8.1630179222717,40.0126196157674));
#41917=CARTESIAN_POINT('Ctrl Pts',(20.137616068932,8.15568851912123,40.0259519936213));
#41918=CARTESIAN_POINT('Ctrl Pts',(20.0558569695587,8.15078011848537,40.0300547921389));
#41919=CARTESIAN_POINT('Ctrl Pts',(19.8217432050462,8.13678247125998,40.0269087340195));
#41920=CARTESIAN_POINT('Ctrl Pts',(19.6702065201761,8.12774637198454,40.0068253048993));
#41921=CARTESIAN_POINT('Ctrl Pts',(19.5015120977089,8.11671399412049,39.9637400008912));
#41922=CARTESIAN_POINT('Ctrl Pts',(19.4805018061017,8.11532323014771,39.9579931499158));
#41923=CARTESIAN_POINT('Ctrl Pts',(19.4515411756094,8.11338104506318,39.9495420634647));
#41924=CARTESIAN_POINT('Ctrl Pts',(19.443503894534,8.11283933775407,39.9471396827373));
#41925=CARTESIAN_POINT('Ctrl Pts',(19.4296974824988,8.11190402058982,39.9429145931875));
#41926=CARTESIAN_POINT('Ctrl Pts',(19.4239207403249,8.11151122886803,39.941117009981));
#41927=CARTESIAN_POINT('Ctrl Pts',(19.4120095652521,8.11069828916114,39.9373489921376));
#41928=CARTESIAN_POINT('Ctrl Pts',(19.4058763644345,8.11027802768853,39.935374941052));
#41929=CARTESIAN_POINT('Ctrl Pts',(19.3915887813023,8.10929505047052,39.9306971757378));
#41930=CARTESIAN_POINT('Ctrl Pts',(19.3834423932747,8.10873156271604,39.9279696588996));
#41931=CARTESIAN_POINT('Ctrl Pts',(19.3578325081119,8.10695042193203,39.9192044673199));
#41932=CARTESIAN_POINT('Ctrl Pts',(19.3404378154737,8.10572635532772,39.9129703985791));
#41933=CARTESIAN_POINT('Ctrl Pts',(19.2997750854902,8.10283030053294,39.8977346759945));
#41934=CARTESIAN_POINT('Ctrl Pts',(19.2765872613588,8.10115181742421,39.8885297897209));
#41935=CARTESIAN_POINT('Ctrl Pts',(19.1948651886159,8.09513808727592,39.8542393282697));
#41936=CARTESIAN_POINT('Ctrl Pts',(19.1374066323552,8.09072661572826,39.8267104481585));
#41937=CARTESIAN_POINT('Ctrl Pts',(18.9866601440702,8.07867597343489,39.7450826533235));
#41938=CARTESIAN_POINT('Ctrl Pts',(18.8963694330047,8.07092809282087,39.685923146009));
#41939=CARTESIAN_POINT('Ctrl Pts',(18.7944358694665,8.06175352749629,39.6061961412275));
#41940=CARTESIAN_POINT('Ctrl Pts',(18.7776006583842,8.06022353483445,39.5925654362329));
#41941=CARTESIAN_POINT('Ctrl Pts',(18.7192075297478,8.05487279304149,39.5436363421388));
#41942=CARTESIAN_POINT('Ctrl Pts',(18.6789156492351,8.05109995361925,39.5068591291709));
#41943=CARTESIAN_POINT('Ctrl Pts',(18.6340826937053,8.04685641959878,39.462309668044));
#41944=CARTESIAN_POINT('Ctrl Pts',(18.627974052236,8.04627720477758,39.4561572640619));
#41945=CARTESIAN_POINT('Ctrl Pts',(18.6187839150898,8.04540454477022,39.4467756313335));
#41946=CARTESIAN_POINT('Ctrl Pts',(18.6156719075951,8.04510881847644,39.4435766475875));
#41947=CARTESIAN_POINT('Ctrl Pts',(18.6101012582495,8.04457910116072,39.4378104049483));
#41948=CARTESIAN_POINT('Ctrl Pts',(18.6076385976061,8.04434480321825,39.4352471373061));
#41949=CARTESIAN_POINT('Ctrl Pts',(18.6022842959842,8.04383513139112,39.4296431754841));
#41950=CARTESIAN_POINT('Ctrl Pts',(18.5993954931506,8.0435599738941,39.4265998566203));
#41951=CARTESIAN_POINT('Ctrl Pts',(18.5934540935229,8.04299363446229,39.4202996231858));
#41952=CARTESIAN_POINT('Ctrl Pts',(18.5904028217868,8.0427025517503,39.4170414868729));
#41953=CARTESIAN_POINT('Ctrl Pts',(18.5753938953932,8.04126941148954,39.4009031044856));
#41954=CARTESIAN_POINT('Ctrl Pts',(18.5636008577102,8.04013914778588,39.3878699458196));
#41955=CARTESIAN_POINT('Ctrl Pts',(18.5025906254496,8.03425795952168,39.3185632808165));
#41956=CARTESIAN_POINT('Ctrl Pts',(18.4564920560797,8.02969456057786,39.2596193255185));
#41957=CARTESIAN_POINT('Ctrl Pts',(18.3757199594956,8.02114917717964,39.1429582792398));
#41958=CARTESIAN_POINT('Ctrl Pts',(18.3404180853368,8.01716121659139,39.0858173054875));
#41959=CARTESIAN_POINT('Ctrl Pts',(18.2915384516555,8.01107235717915,38.9966042327989));
#41960=CARTESIAN_POINT('Ctrl Pts',(18.2757308962805,8.00899469787192,38.9658152121036));
#41961=CARTESIAN_POINT('Ctrl Pts',(18.2220739328013,8.0014922378881,38.8540008388833));
#41962=CARTESIAN_POINT('Ctrl Pts',(18.1890441956011,7.99598224010357,38.770801246144));
#41963=CARTESIAN_POINT('Ctrl Pts',(18.1578234815548,7.98941345427972,38.6728079897337));
#41964=CARTESIAN_POINT('Ctrl Pts',(18.1538762281101,7.98855056705286,38.6599556432484));
#41965=CARTESIAN_POINT('Ctrl Pts',(18.1477402884673,7.98715484762477,38.6392064968878));
#41966=CARTESIAN_POINT('Ctrl Pts',(18.1454669677096,7.98662475336065,38.6313350298936));
#41967=CARTESIAN_POINT('Ctrl Pts',(18.1415060026377,7.98567737467784,38.6172848736708));
#41968=CARTESIAN_POINT('Ctrl Pts',(18.1397988466497,7.98526072619015,38.6111117746514));
#41969=CARTESIAN_POINT('Ctrl Pts',(18.1362917067912,7.98438697452295,38.5981795655669));
#41970=CARTESIAN_POINT('Ctrl Pts',(18.1344976828263,7.98392968656042,38.5914189497571));
#41971=CARTESIAN_POINT('Ctrl Pts',(18.1309354455492,7.98300025366973,38.5776943280537));
#41972=CARTESIAN_POINT('Ctrl Pts',(18.1291692933754,7.98252805065453,38.5707299061581));
#41973=CARTESIAN_POINT('Ctrl Pts',(18.1249100047128,7.98136049873711,38.5535317092141));
#41974=CARTESIAN_POINT('Ctrl Pts',(18.1224617233113,7.98066373097216,38.543287168561));
#41975=CARTESIAN_POINT('Ctrl Pts',(18.1120907649617,7.97759554651792,38.4982632812398));
#41976=CARTESIAN_POINT('Ctrl Pts',(18.1050501308199,7.9751965587917,38.4632900088296));
#41977=CARTESIAN_POINT('Ctrl Pts',(18.0801736801999,7.96524177593111,38.3191745791166));
#41978=CARTESIAN_POINT('Ctrl Pts',(18.0707712265503,7.95744052614099,38.2088079959635));
#41979=CARTESIAN_POINT('Ctrl Pts',(18.0708707823177,7.94955924721526,38.0982626501526));
#41980=CARTESIAN_POINT('Ctrl Pts',(18.070870782374,7.94955924275848,38.0982625876404));
#41981=CARTESIAN_POINT('Ctrl Pts',(18.0709815859836,7.94078785002418,37.9752322203734));
#41982=CARTESIAN_POINT('Ctrl Pts',(18.0828614324957,7.93195349740318,37.852480327936));
#41983=CARTESIAN_POINT('Ctrl Pts',(18.1083340720369,7.92290448633068,37.7215163541891));
#41984=CARTESIAN_POINT('Ctrl Pts',(18.1103936426356,7.92220566482815,37.7113643372776));
#41985=CARTESIAN_POINT('Ctrl Pts',(18.1137385923834,7.92112046666037,37.695531997144));
#41986=CARTESIAN_POINT('Ctrl Pts',(18.1149680546044,7.9207312744099,37.6898402382882));
#41987=CARTESIAN_POINT('Ctrl Pts',(18.1173347732318,7.92000005993563,37.6791190339692));
#41988=CARTESIAN_POINT('Ctrl Pts',(18.1184664562775,7.91965774266281,37.6740884258275));
#41989=CARTESIAN_POINT('Ctrl Pts',(18.1204335044086,7.91907509552119,37.665505278738));
#41990=CARTESIAN_POINT('Ctrl Pts',(18.1212588003677,7.91883420057298,37.6619504824603));
#41991=CARTESIAN_POINT('Ctrl Pts',(18.1228667344757,7.91837165805236,37.6551127672726));
#41992=CARTESIAN_POINT('Ctrl Pts',(18.1236479023097,7.91814992555382,37.6518295499347));
#41993=CARTESIAN_POINT('Ctrl Pts',(18.1257579088503,7.91755883881139,37.6430634973561));
#41994=CARTESIAN_POINT('Ctrl Pts',(18.1271022020726,7.9171903587158,37.6375843599501));
#41995=CARTESIAN_POINT('Ctrl Pts',(18.1320638058245,7.91585894591206,37.6177382214434));
#41996=CARTESIAN_POINT('Ctrl Pts',(18.1358226627571,7.91490371288157,37.6034066692696));
#41997=CARTESIAN_POINT('Ctrl Pts',(18.1677708597934,7.90719006023246,37.4870747125593));
#41998=CARTESIAN_POINT('Ctrl Pts',(18.204148434913,7.90083385062824,37.3874943423854));
#41999=CARTESIAN_POINT('Ctrl Pts',(18.2747788486434,7.89075936218746,37.2345059042281));
#42000=CARTESIAN_POINT('Ctrl Pts',(18.3037960780335,7.88703051799953,37.1789353164767));
#42001=CARTESIAN_POINT('Ctrl Pts',(18.3703464451564,7.87910091362658,37.0653339632387));
#42002=CARTESIAN_POINT('Ctrl Pts',(18.4083945412223,7.87489590375913,37.0077109572764));
#42003=CARTESIAN_POINT('Ctrl Pts',(18.4722980810083,7.86818748609389,36.9213801304051));
#42004=CARTESIAN_POINT('Ctrl Pts',(18.496066448591,7.86575820966751,36.8911983184067));
#42005=CARTESIAN_POINT('Ctrl Pts',(18.526062526012,7.86275908758027,36.8553634287931));
#42006=CARTESIAN_POINT('Ctrl Pts',(18.5314476544807,7.8622231558329,36.8490140382238));
#42007=CARTESIAN_POINT('Ctrl Pts',(18.5419589338391,7.86118172943429,36.8367820114995));
#42008=CARTESIAN_POINT('Ctrl Pts',(18.5470800139676,7.86067644661945,36.8308952177528));
#42009=CARTESIAN_POINT('Ctrl Pts',(18.5564334103579,7.85975726225025,36.8202740986713));
#42010=CARTESIAN_POINT('Ctrl Pts',(18.5606536791342,7.85934386276858,36.8155292730992));
#42011=CARTESIAN_POINT('Ctrl Pts',(18.5697858202491,7.85845212863475,36.8053635766621));
#42012=CARTESIAN_POINT('Ctrl Pts',(18.5747052401864,7.85797348184289,36.7999496495272));
#42013=CARTESIAN_POINT('Ctrl Pts',(18.5880636521978,7.85667827707741,36.7854153878082));
#42014=CARTESIAN_POINT('Ctrl Pts',(18.5965600490139,7.85585929943949,36.7763485184464));
#42015=CARTESIAN_POINT('Ctrl Pts',(18.6378971595286,7.85189707292522,36.7330813624471));
#42016=CARTESIAN_POINT('Ctrl Pts',(18.6719011617202,7.8487039128033,36.7000201709512));
#42017=CARTESIAN_POINT('Ctrl Pts',(18.7301387446341,7.84333611582928,36.6474299537151));
#42018=CARTESIAN_POINT('Ctrl Pts',(18.7536898745625,7.84119086968474,36.6271733793763));
#42019=CARTESIAN_POINT('Ctrl Pts',(18.9079821399129,7.82730307682844,36.5008163217202));
#42020=CARTESIAN_POINT('Ctrl Pts',(19.0516332880843,7.81503465768568,36.4116623921454));
#42021=CARTESIAN_POINT('Ctrl Pts',(19.2395528954832,7.80071797318077,36.3266700539577));
#42022=CARTESIAN_POINT('Ctrl Pts',(19.2745400062806,7.79812364025917,36.3120718235531));
#42023=CARTESIAN_POINT('Ctrl Pts',(19.3168457914446,7.79508904265377,36.2958665195112));
#42024=CARTESIAN_POINT('Ctrl Pts',(19.3237696483125,7.7945956247834,36.2932598958635));
#42025=CARTESIAN_POINT('Ctrl Pts',(19.3346679505942,7.79382422757316,36.2892284396604));
#42026=CARTESIAN_POINT('Ctrl Pts',(19.3386322802388,7.79354471350728,36.2877767466987));
#42027=CARTESIAN_POINT('Ctrl Pts',(19.3459416611282,7.7930313897028,36.2851273131224));
#42028=CARTESIAN_POINT('Ctrl Pts',(19.3492852351804,7.79279736515268,36.2839258067258));
#42029=CARTESIAN_POINT('Ctrl Pts',(19.3568065837667,7.79227268620333,36.2812464644663));
#42030=CARTESIAN_POINT('Ctrl Pts',(19.3609861317343,7.79198233695981,36.2797737858068));
#42031=CARTESIAN_POINT('Ctrl Pts',(19.3716916238459,7.79124163933946,36.2760430852694));
#42032=CARTESIAN_POINT('Ctrl Pts',(19.378224752771,7.7907924682265,36.2738056544388));
#42033=CARTESIAN_POINT('Ctrl Pts',(19.3878786242408,7.79013273249309,36.2705572605874));
#42034=CARTESIAN_POINT('Ctrl Pts',(19.39099001264,7.78992071334236,36.2695191477629));
#42035=CARTESIAN_POINT('Ctrl Pts',(19.3941040087786,7.78970911166913,36.2684889831831));
#42036=CARTESIAN_POINT('Ctrl Pts',(19.3941039249488,7.61899517246903,36.2684890109154));
#42037=CARTESIAN_POINT('Ctrl Pts',(19.3586316938068,7.62156120579377,36.2802238493905));
#42038=CARTESIAN_POINT('Ctrl Pts',(19.3234998481385,7.62415666268337,36.2929893809385));
#42039=CARTESIAN_POINT('Ctrl Pts',(19.2536533155114,7.62942160838414,36.3206925556468));
#42040=CARTESIAN_POINT('Ctrl Pts',(19.2189711935278,7.63208971719421,36.3356411464752));
#42041=CARTESIAN_POINT('Ctrl Pts',(19.1080276902565,7.64078330005079,36.3873721080101));
#42042=CARTESIAN_POINT('Ctrl Pts',(19.0337426739678,7.64685795126209,36.428157996141));
#42043=CARTESIAN_POINT('Ctrl Pts',(18.9093149896807,7.6572940756148,36.5075457740809));
#42044=CARTESIAN_POINT('Ctrl Pts',(18.8579360495256,7.66168780432595,36.5439807747048));
#42045=CARTESIAN_POINT('Ctrl Pts',(18.7983702275426,7.66680670373622,36.5907644504401));
#42046=CARTESIAN_POINT('Ctrl Pts',(18.7883928458919,7.66766497629147,36.5987624506049));
#42047=CARTESIAN_POINT('Ctrl Pts',(18.7745043179933,7.66886002723209,36.6101243409625));
#42048=CARTESIAN_POINT('Ctrl Pts',(18.7705262813082,7.66920235989128,36.613405394005));
#42049=CARTESIAN_POINT('Ctrl Pts',(18.7637554521478,7.66978502475229,36.6190356883718));
#42050=CARTESIAN_POINT('Ctrl Pts',(18.7609560986321,7.67002592212201,36.6213769629307));
#42051=CARTESIAN_POINT('Ctrl Pts',(18.7555808061493,7.67048846268244,36.625898641239));
#42052=CARTESIAN_POINT('Ctrl Pts',(18.7530039367423,7.67071019083023,36.6280778673513));
#42053=CARTESIAN_POINT('Ctrl Pts',(18.7461349381336,7.6713012526505,36.6339178785816));
#42054=CARTESIAN_POINT('Ctrl Pts',(18.7418530840003,7.67166971230568,36.6375907823627));
#42055=CARTESIAN_POINT('Ctrl Pts',(18.7263862548942,7.67300097523286,36.6509761846395));
#42056=CARTESIAN_POINT('Ctrl Pts',(18.7152967846964,7.67395608107763,36.6607989473222));
#42057=CARTESIAN_POINT('Ctrl Pts',(18.6251393306581,7.68173694111128,36.7425306317676));
#42058=CARTESIAN_POINT('Ctrl Pts',(18.5520481770638,7.68815230300334,36.8207788541916));
#42059=CARTESIAN_POINT('Ctrl Pts',(18.4159511999036,7.70128268318915,36.9931833118541));
#42060=CARTESIAN_POINT('Ctrl Pts',(18.3539904536605,7.70797585021229,37.0876244435952));
#42061=CARTESIAN_POINT('Ctrl Pts',(18.2750831872183,7.71827010430045,37.2344837131553));
#42062=CARTESIAN_POINT('Ctrl Pts',(18.2515430873667,7.72165710710516,37.2830825954596));
#42063=CARTESIAN_POINT('Ctrl Pts',(18.2250909000193,7.72591730070476,37.344091871434));
#42064=CARTESIAN_POINT('Ctrl Pts',(18.2202209540419,7.72672333120259,37.3556305032966));
#42065=CARTESIAN_POINT('Ctrl Pts',(18.2127042285737,7.72800289084248,37.3739358428489));
#42066=CARTESIAN_POINT('Ctrl Pts',(18.2099826763191,7.72847390568883,37.3806716233918));
#42067=CARTESIAN_POINT('Ctrl Pts',(18.2049519463818,7.72935933247641,37.3933279221979));
#42068=CARTESIAN_POINT('Ctrl Pts',(18.202633844324,7.72977343937215,37.3992448065409));
#42069=CARTESIAN_POINT('Ctrl Pts',(18.1975102418428,7.73070263018082,37.4125153275659));
#42070=CARTESIAN_POINT('Ctrl Pts',(18.1947204374632,7.73121822794328,37.4198748636532));
#42071=CARTESIAN_POINT('Ctrl Pts',(18.1877595115763,7.73252968738326,37.4385824735616));
#42072=CARTESIAN_POINT('Ctrl Pts',(18.1836499420549,7.73332756563794,37.4499529340829));
#42073=CARTESIAN_POINT('Ctrl Pts',(18.1603220784099,7.73799863950985,37.5164457983572));
#42074=CARTESIAN_POINT('Ctrl Pts',(18.1435087566353,7.7419496297835,37.5723738041094));
#42075=CARTESIAN_POINT('Ctrl Pts',(18.0903790690229,7.75694828596013,37.783385047107));
#42076=CARTESIAN_POINT('Ctrl Pts',(18.0707712491718,7.76846792857911,37.9420078297301));
#42077=CARTESIAN_POINT('Ctrl Pts',(18.0708800060321,7.78078995297317,38.1166703550642));
#42078=CARTESIAN_POINT('Ctrl Pts',(18.071075702115,7.78187746815421,38.1321391168821));
#42079=CARTESIAN_POINT('Ctrl Pts',(18.072653583882,7.78635212033722,38.1960623733451));
#42080=CARTESIAN_POINT('Ctrl Pts',(18.0756758369737,7.78969441522575,38.2444631726518));
#42081=CARTESIAN_POINT('Ctrl Pts',(18.0812865879851,7.79346390897368,38.3003508899143));
#42082=CARTESIAN_POINT('Ctrl Pts',(18.0821001007524,7.79397747374924,38.3079942735344));
#42083=CARTESIAN_POINT('Ctrl Pts',(18.0834754118244,7.79479565010707,38.32022120739));
#42084=CARTESIAN_POINT('Ctrl Pts',(18.0840080104782,7.79510181208791,38.3248078611891));
#42085=CARTESIAN_POINT('Ctrl Pts',(18.0849823240584,7.79564346882633,38.3329434414558));
#42086=CARTESIAN_POINT('Ctrl Pts',(18.0854174451735,7.79587932591216,38.3364931027698));
#42087=CARTESIAN_POINT('Ctrl Pts',(18.0863650356692,7.79638037569987,38.3440493696792));
#42088=CARTESIAN_POINT('Ctrl Pts',(18.0868802171628,7.79664541514752,38.3480555760486));
#42089=CARTESIAN_POINT('Ctrl Pts',(18.0883171843531,7.79736517283325,38.358959051455));
#42090=CARTESIAN_POINT('Ctrl Pts',(18.0892637228852,7.7978185306423,38.3658530814156));
#42091=CARTESIAN_POINT('Ctrl Pts',(18.094351515473,7.80015301513959,38.4014780511042));
#42092=CARTESIAN_POINT('Ctrl Pts',(18.0991038068631,7.80200213014189,38.4301197436843));
#42093=CARTESIAN_POINT('Ctrl Pts',(18.1342044229316,7.81386158498889,38.6156323398797));
#42094=CARTESIAN_POINT('Ctrl Pts',(18.1832979986906,7.82311917516696,38.768338216969));
#42095=CARTESIAN_POINT('Ctrl Pts',(18.2897698010846,7.83837582605186,38.9973617608906));
#42096=CARTESIAN_POINT('Ctrl Pts',(18.3348804051058,7.84408195910548,39.0785288867973));
#42097=CARTESIAN_POINT('Ctrl Pts',(18.3930550783681,7.85086812418052,39.1674519173422));
#42098=CARTESIAN_POINT('Ctrl Pts',(18.4005801785246,7.85173631361516,39.1786944872048));
#42099=CARTESIAN_POINT('Ctrl Pts',(18.4128654067826,7.85313895276415,39.1966375303944));
#42100=CARTESIAN_POINT('Ctrl Pts',(18.4175512824989,7.85367062009236,39.2033884824034));
#42101=CARTESIAN_POINT('Ctrl Pts',(18.425967735118,7.85461979460738,39.2153501928541));
#42102=CARTESIAN_POINT('Ctrl Pts',(18.4296814340584,7.85503665717784,39.2205727211558));
#42103=CARTESIAN_POINT('Ctrl Pts',(18.4374957954657,7.85590981789656,39.2314468272025));
#42104=CARTESIAN_POINT('Ctrl Pts',(18.4416012516541,7.85636629565479,39.2370948293684));
#42105=CARTESIAN_POINT('Ctrl Pts',(18.4523983592904,7.85756103300159,39.2517804366233));
#42106=CARTESIAN_POINT('Ctrl Pts',(18.4591384530764,7.85830115601384,39.2607819333021));
#42107=CARTESIAN_POINT('Ctrl Pts',(18.4894422001682,7.8616042419708,39.3005240140847));
#42108=CARTESIAN_POINT('Ctrl Pts',(18.5138483705593,7.86419999990527,39.3306078757362));
#42109=CARTESIAN_POINT('Ctrl Pts',(18.5824484584771,7.87133338803641,39.4101476780712));
#42110=CARTESIAN_POINT('Ctrl Pts',(18.6283107099915,7.87593427760172,39.4580891900262));
#42111=CARTESIAN_POINT('Ctrl Pts',(18.7186366342435,7.88467530151629,39.5432592612499));
#42112=CARTESIAN_POINT('Ctrl Pts',(18.7624900067744,7.88879468224539,39.5810327149036));
#42113=CARTESIAN_POINT('Ctrl Pts',(18.8969708433063,7.90099844007742,39.6867205179527));
#42114=CARTESIAN_POINT('Ctrl Pts',(18.99196122443,7.90909339899043,39.7487019663138));
#42115=CARTESIAN_POINT('Ctrl Pts',(19.1048612870469,7.91776954821747,39.8089431905946));
#42116=CARTESIAN_POINT('Ctrl Pts',(19.117955106181,7.91876205689514,39.8157380283094));
#42117=CARTESIAN_POINT('Ctrl Pts',(19.1361541024514,7.92012138055456,39.8249187044733));
#42118=CARTESIAN_POINT('Ctrl Pts',(19.1411933111216,7.9204956565443,39.8274331665379));
#42119=CARTESIAN_POINT('Ctrl Pts',(19.1492681495525,7.92109193924984,39.8314182776021));
#42120=CARTESIAN_POINT('Ctrl Pts',(19.1522967017462,7.92131480723831,39.8329030705573));
#42121=CARTESIAN_POINT('Ctrl Pts',(19.1586114276241,7.92177786740126,39.8359784433282));
#42122=CARTESIAN_POINT('Ctrl Pts',(19.1618982350409,7.92201796843548,39.8375676439365));
#42123=CARTESIAN_POINT('Ctrl Pts',(19.1698452839241,7.92259632252402,39.8413823171334));
#42124=CARTESIAN_POINT('Ctrl Pts',(19.1745100335469,7.92293400319681,39.843598446847));
#42125=CARTESIAN_POINT('Ctrl Pts',(19.1907991679223,7.92410710027106,39.851257066921));
#42126=CARTESIAN_POINT('Ctrl Pts',(19.2024692353943,7.92493680597711,39.8566024029281));
#42127=CARTESIAN_POINT('Ctrl Pts',(19.2721028443825,7.92982910343991,39.8876602255865));
#42128=CARTESIAN_POINT('Ctrl Pts',(19.3312582818133,7.9337467355615,39.9106213284525));
#42129=CARTESIAN_POINT('Ctrl Pts',(19.47148912599,7.94272248606554,39.9572383341591));
#42130=CARTESIAN_POINT('Ctrl Pts',(19.5531966324928,7.94772282703611,39.9785701205641));
#42131=CARTESIAN_POINT('Ctrl Pts',(19.6731237878737,7.95503154128503,40.0016099584103));
#42132=CARTESIAN_POINT('Ctrl Pts',(19.7104075910097,7.957298930454,40.0076437328257));
#42133=CARTESIAN_POINT('Ctrl Pts',(19.8341072206104,7.96485470963064,40.0239524149944));
#42134=CARTESIAN_POINT('Ctrl Pts',(19.9210308904941,7.97022248919688,40.0294751262779));
#42135=CARTESIAN_POINT('Ctrl Pts',(20.0214033533959,7.97663386841754,40.0290576662761));
#42136=CARTESIAN_POINT('Ctrl Pts',(20.0347820945742,7.97749266036616,40.0288628190695));
#42137=CARTESIAN_POINT('Ctrl Pts',(20.0563289978584,7.97888303197086,40.0283247694685));
#42138=CARTESIAN_POINT('Ctrl Pts',(20.0644990494948,7.97941190778711,40.0280687855412));
#42139=CARTESIAN_POINT('Ctrl Pts',(20.0790647209291,7.98035789671796,40.0275197312065));
#42140=CARTESIAN_POINT('Ctrl Pts',(20.0854610112012,7.98077438061481,40.0272467299766));
#42141=CARTESIAN_POINT('Ctrl Pts',(20.0988519696126,7.98164859907185,40.0266083938286));
#42142=CARTESIAN_POINT('Ctrl Pts',(20.1058462318858,7.98210652246107,40.0262367943975));
#42143=CARTESIAN_POINT('Ctrl Pts',(20.1241621666118,7.98330919578944,40.0251636254735));
#42144=CARTESIAN_POINT('Ctrl Pts',(20.1354798124313,7.9840558550888,40.0244002805033));
#42145=CARTESIAN_POINT('Ctrl Pts',(20.1863934508014,7.98743107601014,40.0205149351695));
#42146=CARTESIAN_POINT('Ctrl Pts',(20.2258915623011,7.99009422285054,40.016270529701));
#42147=CARTESIAN_POINT('Ctrl Pts',(20.428295209575,8.00398280930177,39.9881760861714));
#42148=CARTESIAN_POINT('Ctrl Pts',(20.5877741696179,8.01581788385942,39.944762637889));
#42149=CARTESIAN_POINT('Ctrl Pts',(20.8135054934771,8.03317028334888,39.8510356739615));
#42150=CARTESIAN_POINT('Ctrl Pts',(20.8852804194693,8.03877112835411,39.8158667835322));
#42151=CARTESIAN_POINT('Ctrl Pts',(20.9627759903949,8.04476476583556,39.7717331820617));
#42152=CARTESIAN_POINT('Ctrl Pts',(20.970842355216,8.04538791678101,39.7670616573996));
#42153=CARTESIAN_POINT('Ctrl Pts',(20.9827837220664,8.04630899831782,39.7600299066897));
#42154=CARTESIAN_POINT('Ctrl Pts',(20.986684622988,8.04660966112339,39.7577142670757));
#42155=CARTESIAN_POINT('Ctrl Pts',(20.993631982281,8.04714467256645,39.7535569879711));
#42156=CARTESIAN_POINT('Ctrl Pts',(20.9966815374143,8.04737935561046,39.7517206611203));
#42157=CARTESIAN_POINT('Ctrl Pts',(21.0032674203887,8.04788582565731,39.7477300100116));
#42158=CARTESIAN_POINT('Ctrl Pts',(21.0068018924797,8.04815741798161,39.7455727430906));
#42159=CARTESIAN_POINT('Ctrl Pts',(21.0166512489848,8.04891372522387,39.7395175708778));
#42160=CARTESIAN_POINT('Ctrl Pts',(21.0229507122316,8.04939683769124,39.7355945316549));
#42161=CARTESIAN_POINT('Ctrl Pts',(21.0595614304736,8.05220195870442,39.7125006690888));
#42162=CARTESIAN_POINT('Ctrl Pts',(21.0893582392945,8.05447460043281,39.692522482486));
#42163=CARTESIAN_POINT('Ctrl Pts',(21.1856139593697,8.06184216656047,39.6240180700438));
#42164=CARTESIAN_POINT('Ctrl Pts',(21.2495304216564,8.06677915040896,39.5720691320599));
#42165=CARTESIAN_POINT('Ctrl Pts',(21.4212818959306,8.08076508786182,39.4132039033355));
#42166=CARTESIAN_POINT('Ctrl Pts',(21.5200776652444,8.08976415563604,39.2974574445647));
#42167=CARTESIAN_POINT('Ctrl Pts',(21.6164070899917,8.10075490971927,39.1532075792018));
#42168=CARTESIAN_POINT('Ctrl Pts',(21.6282086252709,8.10214726928203,39.1348694105022));
#42169=CARTESIAN_POINT('Ctrl Pts',(21.6441179568364,8.10409132906229,39.1092022282616));
#42170=CARTESIAN_POINT('Ctrl Pts',(21.6484928544548,8.10463329051996,39.1020400684056));
#42171=CARTESIAN_POINT('Ctrl Pts',(21.6559413258108,8.10556892853469,39.0896653460847));
#42172=CARTESIAN_POINT('Ctrl Pts',(21.6590373902036,8.1059617856487,39.0844664079044));
#42173=CARTESIAN_POINT('Ctrl Pts',(21.6653792077322,8.10677475001872,39.073702293791));
#42174=CARTESIAN_POINT('Ctrl Pts',(21.6686216409256,8.10719497027218,39.0681352592644));
#42175=CARTESIAN_POINT('Ctrl Pts',(21.6761207125708,8.10817765932373,39.0551102831739));
#42176=CARTESIAN_POINT('Ctrl Pts',(21.6803555339772,8.10874089877448,39.0476400010277));
#42177=CARTESIAN_POINT('Ctrl Pts',(21.6938420896868,8.11056186847124,39.0234748735027));
#42178=CARTESIAN_POINT('Ctrl Pts',(21.7028957352163,8.1118265626218,39.0066713503215));
#42179=CARTESIAN_POINT('Ctrl Pts',(21.7477794305653,8.11831976181454,38.920322950688));
#42180=CARTESIAN_POINT('Ctrl Pts',(21.7796001965999,8.12368480579476,38.8487877032886));
#42181=CARTESIAN_POINT('Ctrl Pts',(21.8362631412043,8.13501029869256,38.6972180849379));
#42182=CARTESIAN_POINT('Ctrl Pts',(21.8604150401814,8.14097504914594,38.6170938619879));
#42183=CARTESIAN_POINT('Ctrl Pts',(21.9040327012736,8.15475497030959,38.4289423079409));
#42184=CARTESIAN_POINT('Ctrl Pts',(21.9196403105624,8.16254911679998,38.3202963550283));
#42185=CARTESIAN_POINT('Ctrl Pts',(21.9264663620621,8.17052696431,38.2017539819836));
#42186=CARTESIAN_POINT('Ctrl Pts',(21.9269279537935,8.17113941799179,38.192602300432));
#42187=CARTESIAN_POINT('Ctrl Pts',(21.9275192005714,8.17204779903873,38.1789467100881));
#42188=CARTESIAN_POINT('Ctrl Pts',(21.9276983061123,8.17234635213509,38.1744452365181));
#42189=CARTESIAN_POINT('Ctrl Pts',(21.927990618872,8.17287908712782,38.1663881387808));
#42190=CARTESIAN_POINT('Ctrl Pts',(21.9281097611104,8.17311359170593,38.162832803767));
#42191=CARTESIAN_POINT('Ctrl Pts',(21.9283470078961,8.17362136722873,38.1551154215447));
#42192=CARTESIAN_POINT('Ctrl Pts',(21.9284614727892,8.17389443445415,38.1509533250296));
#42193=CARTESIAN_POINT('Ctrl Pts',(21.928745006828,8.17465903431459,38.1392669975236));
#42194=CARTESIAN_POINT('Ctrl Pts',(21.9288835238361,8.17514890713363,38.1317419985071));
#42195=CARTESIAN_POINT('Ctrl Pts',(21.9294509794553,8.17807772840586,38.0865405224694));
#42196=CARTESIAN_POINT('Ctrl Pts',(21.9288201015081,8.18046208516254,38.0488559683224));
#42197=CARTESIAN_POINT('Ctrl Pts',(21.9194747838983,8.19310159733426,37.8460238356851));
#42198=CARTESIAN_POINT('Ctrl Pts',(21.8906565594837,8.202652775606,37.682488463203));
#42199=CARTESIAN_POINT('Ctrl Pts',(21.8179856199345,8.21747001524946,37.4499270471553));
#42200=CARTESIAN_POINT('Ctrl Pts',(21.7901244959107,8.22231803728569,37.3767306128295));
#42201=CARTESIAN_POINT('Ctrl Pts',(21.7524950502558,8.22815578990775,37.2934792233196));
#42202=CARTESIAN_POINT('Ctrl Pts',(21.7469699397382,8.22899804480771,37.2815803763392));
#42203=CARTESIAN_POINT('Ctrl Pts',(21.7378016523831,8.23037245836208,37.2623515319013));
#42204=CARTESIAN_POINT('Ctrl Pts',(21.7342323682332,8.23090208269006,37.254986610337));
#42205=CARTESIAN_POINT('Ctrl Pts',(21.7277948721757,8.23184784116408,37.2419159621177));
#42206=CARTESIAN_POINT('Ctrl Pts',(21.7249449730744,8.23226333695332,37.2362013112899));
#42207=CARTESIAN_POINT('Ctrl Pts',(21.7188803620385,8.23314090484524,37.2241901820371));
#42208=CARTESIAN_POINT('Ctrl Pts',(21.7156593130333,8.2336031929943,37.2178970266403));
#42209=CARTESIAN_POINT('Ctrl Pts',(21.7070437825133,8.23482981514142,37.2012900603284));
#42210=CARTESIAN_POINT('Ctrl Pts',(21.7015904915591,8.23559619972432,37.1910072497079));
#42211=CARTESIAN_POINT('Ctrl Pts',(21.6756244452469,8.23919979743906,37.1430978116501));
#42212=CARTESIAN_POINT('Ctrl Pts',(21.6539560314363,8.24207760377928,37.1061146783885));
#42213=CARTESIAN_POINT('Ctrl Pts',(21.5421081887488,8.25634853445262,36.9290155501603));
#42214=CARTESIAN_POINT('Ctrl Pts',(21.4352743836774,8.26835428211553,36.8002800804146));
#42215=CARTESIAN_POINT('Ctrl Pts',(21.2915027350888,8.28226363717272,36.6666660701462));
#42216=CARTESIAN_POINT('Ctrl Pts',(21.2692718390209,8.28435854278109,36.6469430187106));
#42217=CARTESIAN_POINT('Ctrl Pts',(21.2115692145182,8.28964055618312,36.5980849692795));
#42218=CARTESIAN_POINT('Ctrl Pts',(21.1754944732726,8.29279999932842,36.5696855723567));
#42219=CARTESIAN_POINT('Ctrl Pts',(21.1323217570056,8.29638805205321,36.538126961166));
#42220=CARTESIAN_POINT('Ctrl Pts',(21.1261792834721,8.29689414749572,36.5336921832167));
#42221=CARTESIAN_POINT('Ctrl Pts',(21.1162776361748,8.29770272955752,36.5266316967654));
#42222=CARTESIAN_POINT('Ctrl Pts',(21.1125350248994,8.29800671088129,36.5239830590709));
#42223=CARTESIAN_POINT('Ctrl Pts',(21.1058597288791,8.29854591831643,36.5192945949083));
#42224=CARTESIAN_POINT('Ctrl Pts',(21.1029307831459,8.29878149496404,36.51724954398));
#42225=CARTESIAN_POINT('Ctrl Pts',(21.0966618492847,8.29928353469675,36.5128982961346));
#42226=CARTESIAN_POINT('Ctrl Pts',(21.0933202644203,8.29954983636275,36.5105945041466));
#42227=CARTESIAN_POINT('Ctrl Pts',(21.0841569342351,8.30027660235733,36.5043195932789));
#42228=CARTESIAN_POINT('Ctrl Pts',(21.0783205894319,8.30073566119903,36.5003697525375));
#42229=CARTESIAN_POINT('Ctrl Pts',(21.0473497758358,8.30315221743393,36.4796562858718));
#42230=CARTESIAN_POINT('Ctrl Pts',(21.0218441318058,8.30507496225765,36.46345176615));
#42231=CARTESIAN_POINT('Ctrl Pts',(20.857311029446,8.31712672377891,36.3642660455556));
#42232=CARTESIAN_POINT('Ctrl Pts',(20.7086709131394,8.32649664374638,36.2984583172808));
#42233=CARTESIAN_POINT('Ctrl Pts',(20.4678683178965,8.34170282012976,36.2263297539923));
#42234=CARTESIAN_POINT('Ctrl Pts',(20.3805252277703,8.34721367131673,36.2066594666256));
#42235=CARTESIAN_POINT('Ctrl Pts',(20.2788501727,8.35378340003351,36.1910825296478));
#42236=CARTESIAN_POINT('Ctrl Pts',(20.2655394972315,8.35464630896633,36.1891854909047));
#42237=CARTESIAN_POINT('Ctrl Pts',(20.2440873889443,8.35604205597547,36.1863566075999));
#42238=CARTESIAN_POINT('Ctrl Pts',(20.2359577965741,8.35657215592866,36.1853372094417));
#42239=CARTESIAN_POINT('Ctrl Pts',(20.2214620496584,8.35751954013853,36.1836132594661));
#42240=CARTESIAN_POINT('Ctrl Pts',(20.2150983777735,8.35793618842828,36.1828885621943));
#42241=CARTESIAN_POINT('Ctrl Pts',(20.2017777893657,8.35880993490592,36.1814387671002));
#42242=CARTESIAN_POINT('Ctrl Pts',(20.1948203139704,8.35926721785211,36.1807197901899));
#42243=CARTESIAN_POINT('Ctrl Pts',(20.1766129680696,8.36046637585641,36.1789382872848));
#42244=CARTESIAN_POINT('Ctrl Pts',(20.1653575338497,8.36121013987433,36.177936754066));
#42245=CARTESIAN_POINT('Ctrl Pts',(20.1174891358582,8.36438422576868,36.1741008876191));
#42246=CARTESIAN_POINT('Ctrl Pts',(20.080810120225,8.36684368675126,36.1722135749258));
#42247=CARTESIAN_POINT('Ctrl Pts',(19.981685618553,8.37356887418159,36.1699469091807));
#42248=CARTESIAN_POINT('Ctrl Pts',(19.9192430039199,8.37789058335963,36.1715505362774));
#42249=CARTESIAN_POINT('Ctrl Pts',(19.6994584290954,8.39337083360433,36.1878881812139));
#42250=CARTESIAN_POINT('Ctrl Pts',(19.5440037610217,8.40486352406218,36.2188995139984));
#42251=CARTESIAN_POINT('Ctrl Pts',(19.3941040078119,8.41575742730426,36.2684889835028));
#42252=CARTESIAN_POINT('Origin',(20.,-1.3495818343519,38.1));
#42253=CARTESIAN_POINT('',(19.3941040511559,9.38044738890627,36.2684889691639));
#42254=CARTESIAN_POINT('',(19.3941038390373,9.20793124499895,36.2684890393365));
#42255=CARTESIAN_POINT('',(19.3941040087494,-1.3495818343519,36.2684889831927));
#42256=CARTESIAN_POINT('Ctrl Pts',(19.3941040511559,9.38044738890628,36.2684889691639));
#42257=CARTESIAN_POINT('Ctrl Pts',(19.4244038591954,9.37846238576415,36.2584652616171));
#42258=CARTESIAN_POINT('Ctrl Pts',(19.4549533095265,9.37645671543785,36.2491931539581));
#42259=CARTESIAN_POINT('Ctrl Pts',(19.5040072665787,9.37322083091372,36.2356251480271));
#42260=CARTESIAN_POINT('Ctrl Pts',(19.5223628701376,9.37200664483843,36.2308383933716));
#42261=CARTESIAN_POINT('Ctrl Pts',(19.5491051150438,9.37023160205265,36.2242842080849));
#42262=CARTESIAN_POINT('Ctrl Pts',(19.5574380363418,9.36967764525106,36.2223006540568));
#42263=CARTESIAN_POINT('Ctrl Pts',(19.5720576898282,9.36870415186853,36.2189233405878));
#42264=CARTESIAN_POINT('Ctrl Pts',(19.5783387501935,9.36828539133833,36.2175054294475));
#42265=CARTESIAN_POINT('Ctrl Pts',(19.590541821096,9.36747075547413,36.2148147979837));
#42266=CARTESIAN_POINT('Ctrl Pts',(19.5964629656583,9.36707500033364,36.2135384693337));
#42267=CARTESIAN_POINT('Ctrl Pts',(19.610625294456,9.36612723328662,36.2105554453514));
#42268=CARTESIAN_POINT('Ctrl Pts',(19.6188717728155,9.36557440345402,36.2088747643098));
#42269=CARTESIAN_POINT('Ctrl Pts',(19.648670885457,9.3635730919338,36.2030043548024));
#42270=CARTESIAN_POINT('Ctrl Pts',(19.6702829845787,9.36211475933806,36.1991288189235));
#42271=CARTESIAN_POINT('Ctrl Pts',(19.8388999266286,9.35067924359567,36.1718540324525));
#42272=CARTESIAN_POINT('Ctrl Pts',(19.9880738755674,9.34016418351602,36.165176695416));
#42273=CARTESIAN_POINT('Ctrl Pts',(20.2206175186628,9.32352888107175,36.1816720874378));
#42274=CARTESIAN_POINT('Ctrl Pts',(20.3042592883843,9.31750923899284,36.1931486498103));
#42275=CARTESIAN_POINT('Ctrl Pts',(20.4225175357811,9.30914071088895,36.2173570928217));
#42276=CARTESIAN_POINT('Ctrl Pts',(20.457938823403,9.30665359955468,36.2256580252604));
#42277=CARTESIAN_POINT('Ctrl Pts',(20.5003102661593,9.3037185581774,36.2368607913251));
#42278=CARTESIAN_POINT('Ctrl Pts',(20.5075027295189,9.30322175072343,36.2388070875614));
#42279=CARTESIAN_POINT('Ctrl Pts',(20.5186808416477,9.30245203076062,36.2419015253712));
#42280=CARTESIAN_POINT('Ctrl Pts',(20.5226742729832,9.30217752115653,36.2430209042437));
#42281=CARTESIAN_POINT('Ctrl Pts',(20.5300879647477,9.30166882767936,36.2451248092114));
#42282=CARTESIAN_POINT('Ctrl Pts',(20.5335090794663,9.30143445836815,36.2461059128876));
#42283=CARTESIAN_POINT('Ctrl Pts',(20.5412759195961,9.30090320582331,36.2483565592067));
#42284=CARTESIAN_POINT('Ctrl Pts',(20.545619896105,9.30060666298822,36.2496319331079));
#42285=CARTESIAN_POINT('Ctrl Pts',(20.5588495816369,9.29970520746404,36.2535667548162));
#42286=CARTESIAN_POINT('Ctrl Pts',(20.5677207967211,9.29910303843171,36.2562750505778));
#42287=CARTESIAN_POINT('Ctrl Pts',(20.6473669768653,9.29371462932592,36.2812196266964));
#42288=CARTESIAN_POINT('Ctrl Pts',(20.7168330279982,9.2891415070555,36.3074601151395));
#42289=CARTESIAN_POINT('Ctrl Pts',(20.9367400680525,9.27456410133199,36.405365234781));
#42290=CARTESIAN_POINT('Ctrl Pts',(21.0794427766388,9.26488110398889,36.4924947714893));
#42291=CARTESIAN_POINT('Ctrl Pts',(21.2426534575564,9.2518435705921,36.6237887336634));
#42292=CARTESIAN_POINT('Ctrl Pts',(21.2752090120273,9.24913342488915,36.6518187763585));
#42293=CARTESIAN_POINT('Ctrl Pts',(21.3153687305914,9.24563158594843,36.6888007450324));
#42294=CARTESIAN_POINT('Ctrl Pts',(21.3238653920219,9.24488126087871,36.6967684977933));
#42295=CARTESIAN_POINT('Ctrl Pts',(21.3374035244911,9.2436701501548,36.7096963006409));
#42296=CARTESIAN_POINT('Ctrl Pts',(21.3424908719135,9.24321143582419,36.7146080625331));
#42297=CARTESIAN_POINT('Ctrl Pts',(21.3521203777699,9.24233620254087,36.724008061369));
#42298=CARTESIAN_POINT('Ctrl Pts',(21.3566674914402,9.2419199122914,36.7284911056837));
#42299=CARTESIAN_POINT('Ctrl Pts',(21.366989178197,9.24096802738791,36.7387689145601));
#42300=CARTESIAN_POINT('Ctrl Pts',(21.3727492850227,9.24043180846375,36.7445779704189));
#42301=CARTESIAN_POINT('Ctrl Pts',(21.3876417101336,9.2390322069458,36.7597892553047));
#42302=CARTESIAN_POINT('Ctrl Pts',(21.3967153372187,9.2381663134145,36.769248104141));
#42303=CARTESIAN_POINT('Ctrl Pts',(21.4590011949815,9.23212919639442,36.8355171112266));
#42304=CARTESIAN_POINT('Ctrl Pts',(21.5088220041314,9.2268169889976,36.895402637748));
#42305=CARTESIAN_POINT('Ctrl Pts',(21.6530198036651,9.20982806213482,37.0917562660446));
#42306=CARTESIAN_POINT('Ctrl Pts',(21.7335086258486,9.19775235637622,37.2374626824317));
#42307=CARTESIAN_POINT('Ctrl Pts',(21.8082255479244,9.1836298125289,37.426735314335));
#42308=CARTESIAN_POINT('Ctrl Pts',(21.8210432808862,9.1810485131656,37.4622172763466));
#42309=CARTESIAN_POINT('Ctrl Pts',(21.8351623376683,9.17801777970067,37.5052072430586));
#42310=CARTESIAN_POINT('Ctrl Pts',(21.8374694895923,9.17751576643795,37.5123733253891));
#42311=CARTESIAN_POINT('Ctrl Pts',(21.8409875851325,9.17673975402923,37.5235239747351));
#42312=CARTESIAN_POINT('Ctrl Pts',(21.8422276448457,9.1764641162977,37.5274991688242));
#42313=CARTESIAN_POINT('Ctrl Pts',(21.8445031930614,9.1759544020594,37.5348777280876));
#42314=CARTESIAN_POINT('Ctrl Pts',(21.8455421306458,9.17572013343907,37.5382799133167));
#42315=CARTESIAN_POINT('Ctrl Pts',(21.8478753063466,9.17519046685254,37.5459966619202));
#42316=CARTESIAN_POINT('Ctrl Pts',(21.8491638452499,9.17489540090658,37.5503128882292));
#42317=CARTESIAN_POINT('Ctrl Pts',(21.8530268222574,9.17400287539873,37.5634200345114));
#42318=CARTESIAN_POINT('Ctrl Pts',(21.8555538227229,9.17340808067707,37.5722249699103));
#42319=CARTESIAN_POINT('Ctrl Pts',(21.8875096341518,9.1657370155284,37.6866371891619));
#42320=CARTESIAN_POINT('Ctrl Pts',(21.9079514847886,9.15913142827709,37.7945658202078));
#42321=CARTESIAN_POINT('Ctrl Pts',(21.9276361675249,9.14755927770369,37.9869735489237));
#42322=CARTESIAN_POINT('Ctrl Pts',(21.9307253218687,9.14258709039382,38.0707517429598));
#42323=CARTESIAN_POINT('Ctrl Pts',(21.926157940346,9.1327796939752,38.2324680106435));
#42324=CARTESIAN_POINT('Ctrl Pts',(21.9192241078182,9.12796760679228,38.3102591182425));
#42325=CARTESIAN_POINT('Ctrl Pts',(21.9047600020269,9.12179572070304,38.4062601017254));
#42326=CARTESIAN_POINT('Ctrl Pts',(21.9016409252653,9.120575668573,38.4250656321996));
#42327=CARTESIAN_POINT('Ctrl Pts',(21.8967141269301,9.11879360499452,38.4522665745052));
#42328=CARTESIAN_POINT('Ctrl Pts',(21.8951281530765,9.11823857150069,38.4607013977202));
#42329=CARTESIAN_POINT('Ctrl Pts',(21.8922533776101,9.1172638313924,38.4754480103079));
#42330=CARTESIAN_POINT('Ctrl Pts',(21.8909891383856,9.11684490698925,38.4817644959315));
#42331=CARTESIAN_POINT('Ctrl Pts',(21.8884757795538,9.11603042943014,38.4940030679972));
#42332=CARTESIAN_POINT('Ctrl Pts',(21.8872303786607,9.11563499870301,38.4999258481425));
#42333=CARTESIAN_POINT('Ctrl Pts',(21.8841904883848,9.11468877732292,38.5140522670446));
#42334=CARTESIAN_POINT('Ctrl Pts',(21.882370275238,9.11413717478833,38.5222501859118));
#42335=CARTESIAN_POINT('Ctrl Pts',(21.8756240450917,9.11214493212019,38.5517232489689));
#42336=CARTESIAN_POINT('Ctrl Pts',(21.8703905377779,9.11069455722079,38.5729255989421));
#42337=CARTESIAN_POINT('Ctrl Pts',(21.826096309839,9.09911620725388,38.7401202359833));
#42338=CARTESIAN_POINT('Ctrl Pts',(21.7703692472354,9.08843182462655,38.8811254707893));
#42339=CARTESIAN_POINT('Ctrl Pts',(21.6596033282708,9.07175209988574,39.0869626119126));
#42340=CARTESIAN_POINT('Ctrl Pts',(21.6157816893467,9.0658541105387,39.1571800352473));
#42341=CARTESIAN_POINT('Ctrl Pts',(21.5466253219692,9.05763089955311,39.2535970458031));
#42342=CARTESIAN_POINT('Ctrl Pts',(21.5248487100224,9.0551721954122,39.2822321471084));
#42343=CARTESIAN_POINT('Ctrl Pts',(21.497623200754,9.05226608806357,39.316027328985));
#42344=CARTESIAN_POINT('Ctrl Pts',(21.4929304428478,9.05177089933937,39.3217841108422));
#42345=CARTESIAN_POINT('Ctrl Pts',(21.4855688499592,9.05100313685232,39.3307091068223));
#42346=CARTESIAN_POINT('Ctrl Pts',(21.4829229222756,9.05072897880338,39.3338959927707));
#42347=CARTESIAN_POINT('Ctrl Pts',(21.4779840634496,9.05022060045816,39.3398057654878));
#42348=CARTESIAN_POINT('Ctrl Pts',(21.4756938816787,9.04998619681082,39.3425308027766));
#42349=CARTESIAN_POINT('Ctrl Pts',(21.4704690700792,9.04945443661566,39.3487128704998));
#42350=CARTESIAN_POINT('Ctrl Pts',(21.4675297905048,9.04915742313382,39.3521658971675));
#42351=CARTESIAN_POINT('Ctrl Pts',(21.4585175207047,9.04825311159094,39.3626780705615));
#42352=CARTESIAN_POINT('Ctrl Pts',(21.4524054609673,9.04764858263776,39.3697037660274));
#42353=CARTESIAN_POINT('Ctrl Pts',(21.3940139908399,9.04195253499656,39.4358502518299));
#42354=CARTESIAN_POINT('Ctrl Pts',(21.3381967541865,9.03710260876241,39.4917627707013));
#42355=CARTESIAN_POINT('Ctrl Pts',(21.1960911101685,9.02563331058928,39.6176317108342));
#42356=CARTESIAN_POINT('Ctrl Pts',(21.10689339749,9.01910525917784,39.6838647883179));
#42357=CARTESIAN_POINT('Ctrl Pts',(20.943689398834,9.00749882551336,39.7844962620863));
#42358=CARTESIAN_POINT('Ctrl Pts',(20.8722891876929,9.00252171477326,39.8225523536512));
#42359=CARTESIAN_POINT('Ctrl Pts',(20.7810406904025,8.99615139195069,39.8640564463471));
#42360=CARTESIAN_POINT('Ctrl Pts',(20.7632432124232,8.99490872858356,39.8718294108));
#42361=CARTESIAN_POINT('Ctrl Pts',(20.7373561356301,8.9930996289828,39.8826730662276));
#42362=CARTESIAN_POINT('Ctrl Pts',(20.7293580857635,8.99254047558438,39.8859602768648));
#42363=CARTESIAN_POINT('Ctrl Pts',(20.7153542311147,8.99156095217925,39.8916061259698));
#42364=CARTESIAN_POINT('Ctrl Pts',(20.7093581465315,8.99114138802137,39.8939886300791));
#42365=CARTESIAN_POINT('Ctrl Pts',(20.6977312563621,8.99032746428574,39.8985410934219));
#42366=CARTESIAN_POINT('Ctrl Pts',(20.6921019921489,8.98993323556966,39.9007148030457));
#42367=CARTESIAN_POINT('Ctrl Pts',(20.6786789094188,8.98899276374748,39.905825812679));
#42368=CARTESIAN_POINT('Ctrl Pts',(20.6708761364911,8.9884457311628,39.9087391004906));
#42369=CARTESIAN_POINT('Ctrl Pts',(20.6429493512222,8.98648648253201,39.9189604366463));
#42370=CARTESIAN_POINT('Ctrl Pts',(20.6227234672199,8.98506494653042,39.9259836689474));
#42371=CARTESIAN_POINT('Ctrl Pts',(20.4526192343711,8.97308376293558,39.9818957594698));
#42372=CARTESIAN_POINT('Ctrl Pts',(20.2974113932982,8.96191218739062,40.0125696590943));
#42373=CARTESIAN_POINT('Ctrl Pts',(20.0623679540216,8.94509792303987,40.0297018606919));
#42374=CARTESIAN_POINT('Ctrl Pts',(19.9842165924889,8.9395385470095,40.0306453615445));
#42375=CARTESIAN_POINT('Ctrl Pts',(19.8714624720214,8.93172264803946,40.0251575319472));
#42376=CARTESIAN_POINT('Ctrl Pts',(19.8367555490695,8.92934560012076,40.0225256929755));
#42377=CARTESIAN_POINT('Ctrl Pts',(19.7948191062741,8.92652285876029,40.0182016234981));
#42378=CARTESIAN_POINT('Ctrl Pts',(19.7875061362813,8.92603245473581,40.0174052857218));
#42379=CARTESIAN_POINT('Ctrl Pts',(19.7760980460962,8.92527048055544,40.0160969444762));
#42380=CARTESIAN_POINT('Ctrl Pts',(19.7719998068556,8.92499736372034,40.015613608824));
#42381=CARTESIAN_POINT('Ctrl Pts',(19.7643674621382,8.92448991011912,40.0146886296104));
#42382=CARTESIAN_POINT('Ctrl Pts',(19.760833063402,8.92425539620444,40.0142503540567));
#42383=CARTESIAN_POINT('Ctrl Pts',(19.7527794119199,8.92372209355355,40.013229024536));
#42384=CARTESIAN_POINT('Ctrl Pts',(19.748261004609,8.92342365594821,40.0126397462013));
#42385=CARTESIAN_POINT('Ctrl Pts',(19.7364926377775,8.92264826019279,40.0110625221561));
#42386=CARTESIAN_POINT('Ctrl Pts',(19.7292460535279,8.92217267375755,40.0100493182461));
#42387=CARTESIAN_POINT('Ctrl Pts',(19.681701635306,8.91906367903118,40.0031257283683));
#42388=CARTESIAN_POINT('Ctrl Pts',(19.6415905066323,8.91649406947823,39.9959811663601));
#42389=CARTESIAN_POINT('Ctrl Pts',(19.5921586802583,8.91336033079535,39.9855513124973));
#42390=CARTESIAN_POINT('Ctrl Pts',(19.5826002870814,8.91275592212322,39.9834584623849));
#42391=CARTESIAN_POINT('Ctrl Pts',(19.4397828752035,8.90374282818457,39.9510473811516));
#42392=CARTESIAN_POINT('Ctrl Pts',(19.3100921994943,8.89576331158421,39.9067240423076));
#42393=CARTESIAN_POINT('Ctrl Pts',(19.1297083245816,8.88374270018395,39.822792157683));
#42394=CARTESIAN_POINT('Ctrl Pts',(19.0745576891679,8.8799343561846,39.7938051795173));
#42395=CARTESIAN_POINT('Ctrl Pts',(18.9889509952811,8.87372177197631,39.7433800751516));
#42396=CARTESIAN_POINT('Ctrl Pts',(18.9575450559463,8.87137413994948,39.7236396039021));
#42397=CARTESIAN_POINT('Ctrl Pts',(18.9175255030823,8.868282332471,39.696845076736));
#42398=CARTESIAN_POINT('Ctrl Pts',(18.9083752869649,8.86756840773729,39.6906038831658));
#42399=CARTESIAN_POINT('Ctrl Pts',(18.8935758024318,8.86640200055295,39.6803215771954));
#42400=CARTESIAN_POINT('Ctrl Pts',(18.8878936333849,8.86595131912475,39.6763280811934));
#42401=CARTESIAN_POINT('Ctrl Pts',(18.8770006502491,8.86508177814535,39.668584149672));
#42402=CARTESIAN_POINT('Ctrl Pts',(18.8717867424945,8.86466309383263,39.6648382082713));
#42403=CARTESIAN_POINT('Ctrl Pts',(18.8598775001756,8.86370100407859,39.6561915326735));
#42404=CARTESIAN_POINT('Ctrl Pts',(18.8531949277063,8.86315693883525,39.6512735166657));
#42405=CARTESIAN_POINT('Ctrl Pts',(18.8354836532283,8.86170357276788,39.6380619777819));
#42406=CARTESIAN_POINT('Ctrl Pts',(18.8245120238657,8.86079136091972,39.6296930968732));
#42407=CARTESIAN_POINT('Ctrl Pts',(18.7298754388197,8.85281728693721,39.5558873317374));
#42408=CARTESIAN_POINT('Ctrl Pts',(18.6516716104444,8.84548606823654,39.4837731137147));
#42409=CARTESIAN_POINT('Ctrl Pts',(18.568921918506,8.83685000721198,39.3937607319565));
#42410=CARTESIAN_POINT('Ctrl Pts',(18.5581840611404,8.83571065882233,39.381783169043));
#42411=CARTESIAN_POINT('Ctrl Pts',(18.4991291495343,8.82934148227517,39.3142291477083));
#42412=CARTESIAN_POINT('Ctrl Pts',(18.4538760987799,8.82406482873878,39.2560564159517));
#42413=CARTESIAN_POINT('Ctrl Pts',(18.369825225448,8.81355272452002,39.1342169669674));
#42414=CARTESIAN_POINT('Ctrl Pts',(18.331161947731,8.80832711214604,39.07059594045));
#42415=CARTESIAN_POINT('Ctrl Pts',(18.2897378853471,8.80234892868185,38.9926028038602));
#42416=CARTESIAN_POINT('Ctrl Pts',(18.2833423872953,8.80141363314989,38.9802402708871));
#42417=CARTESIAN_POINT('Ctrl Pts',(18.2746817378842,8.80013077599138,38.9630457105301));
#42418=CARTESIAN_POINT('Ctrl Pts',(18.2723021807264,8.7997765373723,38.9582722476042));
#42419=CARTESIAN_POINT('Ctrl Pts',(18.2683126910433,8.79917969634672,38.9501853857593));
#42420=CARTESIAN_POINT('Ctrl Pts',(18.2666924084319,8.79893646156411,38.9468771575315));
#42421=CARTESIAN_POINT('Ctrl Pts',(18.2636225012257,8.79847403793311,38.9405634256781));
#42422=CARTESIAN_POINT('Ctrl Pts',(18.2621711889263,8.79825474225271,38.9375587828101));
#42423=CARTESIAN_POINT('Ctrl Pts',(18.2583735829543,8.79767907212881,38.9296442562446));
#42424=CARTESIAN_POINT('Ctrl Pts',(18.2560402339743,8.79732348947124,38.9247281398847));
#42425=CARTESIAN_POINT('Ctrl Pts',(18.2479539520215,8.79608436302568,38.9075034345863));
#42426=CARTESIAN_POINT('Ctrl Pts',(18.2423101114116,8.79520719849086,38.8951436548102));
#42427=CARTESIAN_POINT('Ctrl Pts',(18.1799165613098,8.78535596336925,38.7545930070958));
#42428=CARTESIAN_POINT('Ctrl Pts',(18.1371632352496,8.77710197449362,38.6206219757629));
#42429=CARTESIAN_POINT('Ctrl Pts',(18.0837672653261,8.76102929922204,38.3571566361323));
#42430=CARTESIAN_POINT('Ctrl Pts',(18.0708933042763,8.75326579097362,38.2289117854329));
#42431=CARTESIAN_POINT('Ctrl Pts',(18.0708670590945,8.74402192427518,38.0839284960393));
#42432=CARTESIAN_POINT('Ctrl Pts',(18.0710737457995,8.7429687848692,38.0675088299204));
#42433=CARTESIAN_POINT('Ctrl Pts',(18.0716948983203,8.74138762033962,38.0430148267056));
#42434=CARTESIAN_POINT('Ctrl Pts',(18.0719505535161,8.74086452035167,38.0349369245966));
#42435=CARTESIAN_POINT('Ctrl Pts',(18.0724986235123,8.73992602230705,38.0204913121164));
#42436=CARTESIAN_POINT('Ctrl Pts',(18.0727718557725,8.73951122603781,38.0141229583419));
#42437=CARTESIAN_POINT('Ctrl Pts',(18.0734174500292,8.73863052621088,38.0006368505826));
#42438=CARTESIAN_POINT('Ctrl Pts',(18.0737977061702,8.73816438323541,37.9935195873927));
#42439=CARTESIAN_POINT('Ctrl Pts',(18.0749181598952,8.73691660500432,37.9745245250183));
#42440=CARTESIAN_POINT('Ctrl Pts',(18.0757288334513,8.73613279111056,37.9626513458907));
#42441=CARTESIAN_POINT('Ctrl Pts',(18.0801953071342,8.73231274178848,37.9050787814133));
#42442=CARTESIAN_POINT('Ctrl Pts',(18.0853692480883,8.72922973673812,37.8595154430513));
#42443=CARTESIAN_POINT('Ctrl Pts',(18.1164982500365,8.71488274826938,37.6517283940498));
#42444=CARTESIAN_POINT('Ctrl Pts',(18.1614846170246,8.70304011542222,37.4930642508039));
#42445=CARTESIAN_POINT('Ctrl Pts',(18.2367485133002,8.68947005300853,37.3169070974939));
#42446=CARTESIAN_POINT('Ctrl Pts',(18.2480259964632,8.68754241184183,37.2919916546102));
#42447=CARTESIAN_POINT('Ctrl Pts',(18.2621790961266,8.68525000917455,37.2624137719484));
#42448=CARTESIAN_POINT('Ctrl Pts',(18.2645492727808,8.68487011077749,37.2575138234003));
#42449=CARTESIAN_POINT('Ctrl Pts',(18.2853959830184,8.6815637120522,37.2148779769429));
#42450=CARTESIAN_POINT('Ctrl Pts',(18.3050817046749,8.67867815729521,37.177741619172));
#42451=CARTESIAN_POINT('Ctrl Pts',(18.3296354828288,8.67536458103033,37.1348681721982));
#42452=CARTESIAN_POINT('Ctrl Pts',(18.3333414428768,8.67487152678297,37.1284824636091));
#42453=CARTESIAN_POINT('Ctrl Pts',(18.3394038990088,8.67407649207481,37.1181730850818));
#42454=CARTESIAN_POINT('Ctrl Pts',(18.3417378144184,8.67377313033206,37.1142363232365));
#42455=CARTESIAN_POINT('Ctrl Pts',(18.3459137970119,8.67323517877215,37.1072492322241));
#42456=CARTESIAN_POINT('Ctrl Pts',(18.3477503243465,8.67300023958734,37.1041956698814));
#42457=CARTESIAN_POINT('Ctrl Pts',(18.3517249614256,8.67249531340159,37.0976283767873));
#42458=CARTESIAN_POINT('Ctrl Pts',(18.3538658461293,8.6722255099855,37.0941163973641));
#42459=CARTESIAN_POINT('Ctrl Pts',(18.3598344350876,8.67147922719108,37.0843954122656));
#42460=CARTESIAN_POINT('Ctrl Pts',(18.3636861953476,8.6710042821337,37.0782011470955));
#42461=CARTESIAN_POINT('Ctrl Pts',(18.3855916359656,8.66833952165047,37.0434151242131));
#42462=CARTESIAN_POINT('Ctrl Pts',(18.4043607577609,8.66619348035324,37.0152780484829));
#42463=CARTESIAN_POINT('Ctrl Pts',(18.4667417501141,8.65943280195774,36.9268878564747));
#42464=CARTESIAN_POINT('Ctrl Pts',(18.5131034263716,8.65494784971253,36.8686538359602));
#42465=CARTESIAN_POINT('Ctrl Pts',(18.671523798129,8.64072457814127,36.6917017671893));
#42466=CARTESIAN_POINT('Ctrl Pts',(18.7952931434053,8.63110109067927,36.5844709369568));
#42467=CARTESIAN_POINT('Ctrl Pts',(18.9485086637306,8.61942861651755,36.4824873374328));
#42468=CARTESIAN_POINT('Ctrl Pts',(18.9661315180916,8.6180904710202,36.4711669356563));
#42469=CARTESIAN_POINT('Ctrl Pts',(18.9909491234143,8.61621042931289,36.4557898621723));
#42470=CARTESIAN_POINT('Ctrl Pts',(18.9979913069591,8.61567744333818,36.4514887854548));
#42471=CARTESIAN_POINT('Ctrl Pts',(19.0102136088123,8.61475313843034,36.4441311554727));
#42472=CARTESIAN_POINT('Ctrl Pts',(19.0153808667649,8.61436259313252,36.4410533789283));
#42473=CARTESIAN_POINT('Ctrl Pts',(19.0261318314719,8.61355044918303,36.4347177000761));
#42474=CARTESIAN_POINT('Ctrl Pts',(19.0317176833372,8.61312871997651,36.4314636049375));
#42475=CARTESIAN_POINT('Ctrl Pts',(19.0448791960044,8.61213552361083,36.4238845798414));
#42476=CARTESIAN_POINT('Ctrl Pts',(19.0524679949931,8.61156323599834,36.4195828651214));
#42477=CARTESIAN_POINT('Ctrl Pts',(19.0774180298089,8.60968276691568,36.405662669337));
#42478=CARTESIAN_POINT('Ctrl Pts',(19.0948980847875,8.60836696962201,36.396260889952));
#42479=CARTESIAN_POINT('Ctrl Pts',(19.1873279636243,8.601415661773,36.3483706546545));
#42480=CARTESIAN_POINT('Ctrl Pts',(19.2645848629636,8.59562094572606,36.3145582251576));
#42481=CARTESIAN_POINT('Ctrl Pts',(19.3604890961541,8.58845997117052,36.2798671695252));
#42482=CARTESIAN_POINT('Ctrl Pts',(19.3772604491198,8.5872091125392,36.2740611274072));
#42483=CARTESIAN_POINT('Ctrl Pts',(19.3941041019635,8.5859548064474,36.2684889523559));
#42484=CARTESIAN_POINT('',(18.0708705926165,8.57277459783182,38.0983183026454));
#42485=CARTESIAN_POINT('Ctrl Pts',(19.3941040078119,8.41575742730426,36.2684889835028));
#42486=CARTESIAN_POINT('Ctrl Pts',(19.3848991309847,8.41642638796206,36.2715341183276));
#42487=CARTESIAN_POINT('Ctrl Pts',(19.375715186781,8.41709286238427,36.274649315926));
#42488=CARTESIAN_POINT('Ctrl Pts',(19.3456867897387,8.4192679999204,36.2850882128645));
#42489=CARTESIAN_POINT('Ctrl Pts',(19.324945616991,8.42076405854974,36.2927002862353));
#42490=CARTESIAN_POINT('Ctrl Pts',(19.2981774761885,8.42268247904916,36.3030494338562));
#42491=CARTESIAN_POINT('Ctrl Pts',(19.292028396551,8.42312231425697,36.3054631784397));
#42492=CARTESIAN_POINT('Ctrl Pts',(19.2822123156983,8.42382293322785,36.3093746665292));
#42493=CARTESIAN_POINT('Ctrl Pts',(19.2785373869231,8.42408488937646,36.3108521740117));
#42494=CARTESIAN_POINT('Ctrl Pts',(19.2715337944116,8.42458343306352,36.3136930603939));
#42495=CARTESIAN_POINT('Ctrl Pts',(19.2682044333705,8.42482012882439,36.3150544142676));
#42496=CARTESIAN_POINT('Ctrl Pts',(19.2604867172502,8.42536814024514,36.3182353608926));
#42497=CARTESIAN_POINT('Ctrl Pts',(19.2561012544136,8.42567903862751,36.3200618600532));
#42498=CARTESIAN_POINT('Ctrl Pts',(19.242108999303,8.42666952907365,36.3259502331411));
#42499=CARTESIAN_POINT('Ctrl Pts',(19.232528182215,8.42734553221231,36.33007390978));
#42500=CARTESIAN_POINT('Ctrl Pts',(19.2098593523128,8.42894082442971,36.3400494795614));
#42501=CARTESIAN_POINT('Ctrl Pts',(19.1968020205997,8.42985638625897,36.3459700372146));
#42502=CARTESIAN_POINT('Ctrl Pts',(19.1501614706936,8.43311898507669,36.3677482185352));
#42503=CARTESIAN_POINT('Ctrl Pts',(19.1169699950115,8.43542625216121,36.3844300878864));
#42504=CARTESIAN_POINT('Ctrl Pts',(18.9892696182184,8.44432445756877,36.4533005999203));
#42505=CARTESIAN_POINT('Ctrl Pts',(18.8987238035524,8.45068962835837,36.5124269462432));
#42506=CARTESIAN_POINT('Ctrl Pts',(18.7224411708371,8.46409296921966,36.6499139954033));
#42507=CARTESIAN_POINT('Ctrl Pts',(18.6378743550572,8.47112546962341,36.7290462520064));
#42508=CARTESIAN_POINT('Ctrl Pts',(18.5516755013798,8.47938786456374,36.8256018110458));
#42509=CARTESIAN_POINT('Ctrl Pts',(18.5425584861293,8.48027690314834,36.8360384440502));
#42510=CARTESIAN_POINT('Ctrl Pts',(18.5281526999225,8.48170672774657,36.852892461833));
#42511=CARTESIAN_POINT('Ctrl Pts',(18.5227914972279,8.48224455341234,36.8592475177218));
#42512=CARTESIAN_POINT('Ctrl Pts',(18.5133620365193,8.48320080127514,36.8705727459033));
#42513=CARTESIAN_POINT('Ctrl Pts',(18.5092771777996,8.48361854477857,36.8755289822587));
#42514=CARTESIAN_POINT('Ctrl Pts',(18.5008317449632,8.48448959551847,36.8858808843018));
#42515=CARTESIAN_POINT('Ctrl Pts',(18.4964753806189,8.48494306278867,36.8912798500816));
#42516=CARTESIAN_POINT('Ctrl Pts',(18.4852616353359,8.48612125631757,36.9053317865503));
#42517=CARTESIAN_POINT('Ctrl Pts',(18.4784493250547,8.48684775159144,36.914020241056));
#42518=CARTESIAN_POINT('Ctrl Pts',(18.4497742969285,8.48995243895945,36.9512462462982));
#42519=CARTESIAN_POINT('Ctrl Pts',(18.4286382113707,8.49235857879415,36.9803318556644));
#42520=CARTESIAN_POINT('Ctrl Pts',(18.360446956283,8.50053748306687,37.0799071250089));
#42521=CARTESIAN_POINT('Ctrl Pts',(18.3172305370408,8.50644268603515,37.1528952376087));
#42522=CARTESIAN_POINT('Ctrl Pts',(18.2475280489201,8.51736527376308,37.2905409566783));
#42523=CARTESIAN_POINT('Ctrl Pts',(18.2194811459851,8.52234319012644,37.3542560202293));
#42524=CARTESIAN_POINT('Ctrl Pts',(18.1616715418693,8.53401414430814,37.5075640687818));
#42525=CARTESIAN_POINT('Ctrl Pts',(18.1349134168957,8.54067530251925,37.5981152197207));
#42526=CARTESIAN_POINT('Ctrl Pts',(18.1128933647926,8.54764374833379,37.6994267760442));
#42527=CARTESIAN_POINT('Ctrl Pts',(18.1109698776412,8.54827023232164,37.7085979485047));
#42528=CARTESIAN_POINT('Ctrl Pts',(18.1082125335167,8.54919526664416,37.7222389572455));
#42529=CARTESIAN_POINT('Ctrl Pts',(18.1073275641157,8.54949658276279,37.7266981445789));
#42530=CARTESIAN_POINT('Ctrl Pts',(18.1057775955158,8.55003230303361,37.7346553451855));
#42531=CARTESIAN_POINT('Ctrl Pts',(18.1051065111721,8.55026704521818,37.7381521021605));
#42532=CARTESIAN_POINT('Ctrl Pts',(18.1036771975485,8.55077312865774,37.7457127228023));
#42533=CARTESIAN_POINT('Ctrl Pts',(18.1029223498069,8.5510442779673,37.749777162634));
#42534=CARTESIAN_POINT('Ctrl Pts',(18.101395415165,8.55160094695933,37.7581486674295));
#42535=CARTESIAN_POINT('Ctrl Pts',(18.1006249048359,8.55188637835711,37.7624560000345));
#42536=CARTESIAN_POINT('Ctrl Pts',(18.0986976260184,8.5526121835612,37.7734455202549));
#42537=CARTESIAN_POINT('Ctrl Pts',(18.0975614133501,8.55305146036004,37.7801313194813));
#42538=CARTESIAN_POINT('Ctrl Pts',(18.0795216856533,8.560220281871,37.8897796796842));
#42539=CARTESIAN_POINT('Ctrl Pts',(18.070961640832,8.5665249751136,37.9939540363477));
#42540=CARTESIAN_POINT('Ctrl Pts',(18.0708707318637,8.57277491926653,38.0983196072232));
#42541=CARTESIAN_POINT('Ctrl Pts',(18.0708707330131,8.5727748402797,38.0983182882505));
#42542=CARTESIAN_POINT('Ctrl Pts',(18.070749004497,8.58113704941933,38.2379557992846));
#42543=CARTESIAN_POINT('Ctrl Pts',(18.0857878098588,8.58938279054467,38.3771880622356));
#42544=CARTESIAN_POINT('Ctrl Pts',(18.1230963197836,8.60024268730473,38.5471660746574));
#42545=CARTESIAN_POINT('Ctrl Pts',(18.1313644004084,8.60241260062862,38.580547285625));
#42546=CARTESIAN_POINT('Ctrl Pts',(18.1432112590839,8.60525678639379,38.623431275503));
#42547=CARTESIAN_POINT('Ctrl Pts',(18.1459793066124,8.60590534179989,38.6331528775391));
#42548=CARTESIAN_POINT('Ctrl Pts',(18.1513784890223,8.60714109316598,38.6515645933021));
#42549=CARTESIAN_POINT('Ctrl Pts',(18.1539948320585,8.60772780255918,38.6602587855167));
#42550=CARTESIAN_POINT('Ctrl Pts',(18.1585975142864,8.60873975400798,38.6751713239731));
#42551=CARTESIAN_POINT('Ctrl Pts',(18.1605542390729,8.60916402911885,38.6813987075839));
#42552=CARTESIAN_POINT('Ctrl Pts',(18.1643503649932,8.60997604842752,38.6932690791636));
#42553=CARTESIAN_POINT('Ctrl Pts',(18.1661842795609,8.61036360949216,38.6989137541779));
#42554=CARTESIAN_POINT('Ctrl Pts',(18.1709985031265,8.61136898667718,38.7135022040483));
#42555=CARTESIAN_POINT('Ctrl Pts',(18.1740183477367,8.61198809041072,38.7224326712289));
#42556=CARTESIAN_POINT('Ctrl Pts',(18.1844393840789,8.61408659738454,38.7525217759866));
#42557=CARTESIAN_POINT('Ctrl Pts',(18.1921436279316,8.61557590037894,38.7735727760014));
#42558=CARTESIAN_POINT('Ctrl Pts',(18.2475914471912,8.62589226262562,38.9172683532188));
#42559=CARTESIAN_POINT('Ctrl Pts',(18.3074018082523,8.63512920963893,39.0348597902583));
#42560=CARTESIAN_POINT('Ctrl Pts',(18.4173860652214,8.64959396410313,39.2054285540465));
#42561=CARTESIAN_POINT('Ctrl Pts',(18.4593751358328,8.6547045979383,39.263234528087));
#42562=CARTESIAN_POINT('Ctrl Pts',(18.531987846301,8.66281453450918,39.3523499195233));
#42563=CARTESIAN_POINT('Ctrl Pts',(18.5606412034207,8.66585735539084,39.3851796683715));
#42564=CARTESIAN_POINT('Ctrl Pts',(18.606682020665,8.67047890652087,39.4344577644889));
#42565=CARTESIAN_POINT('Ctrl Pts',(18.6233040037462,8.67209731613394,39.4515993414355));
#42566=CARTESIAN_POINT('Ctrl Pts',(18.6448687868715,8.67412940367131,39.4730275006471));
#42567=CARTESIAN_POINT('Ctrl Pts',(18.6495201242178,8.67456381686548,39.4776027113989));
#42568=CARTESIAN_POINT('Ctrl Pts',(18.6566110345848,8.67522007655582,39.4845071394238));
#42569=CARTESIAN_POINT('Ctrl Pts',(18.6590335932596,8.67544323160539,39.4868536433027));
#42570=CARTESIAN_POINT('Ctrl Pts',(18.6640220310874,8.67590056600051,39.4916601807315));
#42571=CARTESIAN_POINT('Ctrl Pts',(18.666588528428,8.67613468040881,39.4941194496579));
#42572=CARTESIAN_POINT('Ctrl Pts',(18.6723927952703,8.67666150327284,39.4996505224452));
#42573=CARTESIAN_POINT('Ctrl Pts',(18.675634428608,8.67695389491405,39.5027181859993));
#42574=CARTESIAN_POINT('Ctrl Pts',(18.685204629784,8.67781184124905,39.5117120316583));
#42575=CARTESIAN_POINT('Ctrl Pts',(18.6915626391734,8.67837507944434,39.5176069291249));
#42576=CARTESIAN_POINT('Ctrl Pts',(18.7381991707946,8.68245954925458,39.5602654245514));
#42577=CARTESIAN_POINT('Ctrl Pts',(18.7799849334239,8.6858662967866,39.5953531080771));
#42578=CARTESIAN_POINT('Ctrl Pts',(18.924186096177,8.69702459548907,39.7063646310801));
#42579=CARTESIAN_POINT('Ctrl Pts',(19.0326252067003,8.70448789627749,39.7739093515283));
#42580=CARTESIAN_POINT('Ctrl Pts',(19.2052572280039,8.71609845039306,39.8590208122445));
#42581=CARTESIAN_POINT('Ctrl Pts',(19.2649876174564,8.72006756913927,39.8848041988912));
#42582=CARTESIAN_POINT('Ctrl Pts',(19.3616063094172,8.72650973299399,39.9208372077941));
#42583=CARTESIAN_POINT('Ctrl Pts',(19.3976949994992,8.72892018185757,39.933091109892));
#42584=CARTESIAN_POINT('Ctrl Pts',(19.4448736679951,8.73208747244164,39.947566999168));
#42585=CARTESIAN_POINT('Ctrl Pts',(19.455654753367,8.73281230352817,39.9507720833908));
#42586=CARTESIAN_POINT('Ctrl Pts',(19.4731736494373,8.73399209720041,39.9558139225065));
#42587=CARTESIAN_POINT('Ctrl Pts',(19.4798945945483,8.73444517933215,39.9577087187482));
#42588=CARTESIAN_POINT('Ctrl Pts',(19.4928027209772,8.73531631965207,39.9612722911868));
#42589=CARTESIAN_POINT('Ctrl Pts',(19.4989882309744,8.73573418621684,39.9629468128287));
#42590=CARTESIAN_POINT('Ctrl Pts',(19.5131238880677,8.73669014368657,39.9666980810024));
#42591=CARTESIAN_POINT('Ctrl Pts',(19.5210791477153,8.73722886613063,39.9687549030615));
#42592=CARTESIAN_POINT('Ctrl Pts',(19.5421631522625,8.738658698237,39.9740626745617));
#42593=CARTESIAN_POINT('Ctrl Pts',(19.5553131721715,8.73955257163661,39.977226437254));
#42594=CARTESIAN_POINT('Ctrl Pts',(19.6587672497156,8.74660249150382,40.0009684417915));
#42595=CARTESIAN_POINT('Ctrl Pts',(19.750400094876,8.75296084105432,40.0151543159398));
#42596=CARTESIAN_POINT('Ctrl Pts',(20.0020530997806,8.77069677533662,40.0357444041683));
#42597=CARTESIAN_POINT('Ctrl Pts',(20.1624136223143,8.78233862110124,40.0289194047978));
#42598=CARTESIAN_POINT('Ctrl Pts',(20.3487489584781,8.79535381899516,39.9975672075715));
#42599=CARTESIAN_POINT('Ctrl Pts',(20.3772972232622,8.79733122699818,39.9920978235376));
#42600=CARTESIAN_POINT('Ctrl Pts',(20.4125182631042,8.79974137504841,39.984521078921));
#42601=CARTESIAN_POINT('Ctrl Pts',(20.4193158669378,8.80020515829813,39.9830202393171));
#42602=CARTESIAN_POINT('Ctrl Pts',(20.4300452655318,8.80093486901602,39.9805903184399));
#42603=CARTESIAN_POINT('Ctrl Pts',(20.4339824389206,8.80120214087178,39.9796856438431));
#42604=CARTESIAN_POINT('Ctrl Pts',(20.4413995565228,8.80170467110893,39.9779568091657));
#42605=CARTESIAN_POINT('Ctrl Pts',(20.4448800093189,8.80194007117429,39.9771353502433));
#42606=CARTESIAN_POINT('Ctrl Pts',(20.4528482502636,8.8024780878774,39.9752312738602));
#42607=CARTESIAN_POINT('Ctrl Pts',(20.4573344491471,8.80278033446005,39.9741422227101));
#42608=CARTESIAN_POINT('Ctrl Pts',(20.4692763458322,8.8035832302941,39.9711978239821));
#42609=CARTESIAN_POINT('Ctrl Pts',(20.4767250351528,8.80408230476811,39.9693140000673));
#42610=CARTESIAN_POINT('Ctrl Pts',(20.5310041663886,8.80770780715442,39.9552408946917));
#42611=CARTESIAN_POINT('Ctrl Pts',(20.5773769612004,8.81074388346939,39.9413367275625));
#42612=CARTESIAN_POINT('Ctrl Pts',(20.6340067761872,8.81443064499459,39.922006804528));
#42613=CARTESIAN_POINT('Ctrl Pts',(20.6447987662835,8.8151322727096,39.9182155942086));
#42614=CARTESIAN_POINT('Ctrl Pts',(20.7563313686681,8.82237940952885,39.8779164275811));
#42615=CARTESIAN_POINT('Ctrl Pts',(20.853901503815,8.82869497554362,39.8331700404347));
#42616=CARTESIAN_POINT('Ctrl Pts',(21.0449215969719,8.84185653653094,39.7255001694213));
#42617=CARTESIAN_POINT('Ctrl Pts',(21.1375897259241,8.84869277879936,39.662048752801));
#42618=CARTESIAN_POINT('Ctrl Pts',(21.2356696326248,8.85679948852639,39.5815136467512));
#42619=CARTESIAN_POINT('Ctrl Pts',(21.2470125584576,8.85775110702672,39.5719788673308));
#42620=CARTESIAN_POINT('Ctrl Pts',(21.2641238536013,8.85920891731446,39.5572555037967));
#42621=CARTESIAN_POINT('Ctrl Pts',(21.269972799541,8.85971126396723,39.5521610813264));
#42622=CARTESIAN_POINT('Ctrl Pts',(21.2805076733181,8.86062351311857,39.5428728977643));
#42623=CARTESIAN_POINT('Ctrl Pts',(21.2852041432915,8.86103291211857,39.5386912139283));
#42624=CARTESIAN_POINT('Ctrl Pts',(21.2953299090283,8.86192155003038,39.5295861987027));
#42625=CARTESIAN_POINT('Ctrl Pts',(21.3007517448856,8.86240112493821,39.5246547541177));
#42626=CARTESIAN_POINT('Ctrl Pts',(21.315334154858,8.86370126720918,39.5112386482854));
#42627=CARTESIAN_POINT('Ctrl Pts',(21.3244405434089,8.86452428553332,39.5026958672255));
#42628=CARTESIAN_POINT('Ctrl Pts',(21.3682107678858,8.86853518513463,39.4608284049176));
#42629=CARTESIAN_POINT('Ctrl Pts',(21.401700680364,8.87177446489907,39.4263065874626));
#42630=CARTESIAN_POINT('Ctrl Pts',(21.4538512339425,8.87710966042895,39.368365788667));
#42631=CARTESIAN_POINT('Ctrl Pts',(21.4733191800944,8.87917330927737,39.345698852864));
#42632=CARTESIAN_POINT('Ctrl Pts',(21.5715215036719,8.88996168302534,39.2258363954545));
#42633=CARTESIAN_POINT('Ctrl Pts',(21.6411886795515,8.89895774966858,39.1216076880706));
#42634=CARTESIAN_POINT('Ctrl Pts',(21.7261395517637,8.91171898264758,38.9631239835298));
#42635=CARTESIAN_POINT('Ctrl Pts',(21.7499435467515,8.9155720030314,38.9137808153142));
#42636=CARTESIAN_POINT('Ctrl Pts',(21.7826749066873,8.92126245519379,38.8378301643255));
#42637=CARTESIAN_POINT('Ctrl Pts',(21.7931745007223,8.92316197395149,38.8119329925777));
#42638=CARTESIAN_POINT('Ctrl Pts',(21.8055519995158,8.92549072161026,38.7793907413106));
#42639=CARTESIAN_POINT('Ctrl Pts',(21.8079612661913,8.92594860121751,38.772953093317));
#42640=CARTESIAN_POINT('Ctrl Pts',(21.8117251102374,8.92667114522577,38.762729842947));
#42641=CARTESIAN_POINT('Ctrl Pts',(21.8131023217205,8.9269371107392,38.7589527232692));
#42642=CARTESIAN_POINT('Ctrl Pts',(21.8156837402881,8.92743861232784,38.7518035993506));
#42643=CARTESIAN_POINT('Ctrl Pts',(21.8168903529345,8.92767428198447,38.7484325890233));
#42644=CARTESIAN_POINT('Ctrl Pts',(21.8196424737847,8.92821475154627,38.7406757740149));
#42645=CARTESIAN_POINT('Ctrl Pts',(21.8211815148747,8.92851916939472,38.7362877264286));
#42646=CARTESIAN_POINT('Ctrl Pts',(21.8252589615289,8.92933167171634,38.7245262917952));
#42647=CARTESIAN_POINT('Ctrl Pts',(21.8277685837473,8.92983812124188,38.7171429129602));
#42648=CARTESIAN_POINT('Ctrl Pts',(21.8464626821652,8.93366122788981,38.6610299493216));
#42649=CARTESIAN_POINT('Ctrl Pts',(21.8607422232866,8.93687605393367,38.6116820031645));
#42650=CARTESIAN_POINT('Ctrl Pts',(21.9032979656997,8.94780253537605,38.4390849951399));
#42651=CARTESIAN_POINT('Ctrl Pts',(21.9214243829713,8.95520991517982,38.3136682034745));
#42652=CARTESIAN_POINT('Ctrl Pts',(21.9313172375979,8.96836514029637,38.0954661817475));
#42653=CARTESIAN_POINT('Ctrl Pts',(21.9289038780743,8.9739946166648,38.0033896555581));
#42654=CARTESIAN_POINT('Ctrl Pts',(21.9179053219143,8.98115052821193,37.8911613108213));
#42655=CARTESIAN_POINT('Ctrl Pts',(21.9155444275347,8.9824789906151,37.8705138026597));
#42656=CARTESIAN_POINT('Ctrl Pts',(21.9116985871941,8.98439030799835,37.8410984296478));
#42657=CARTESIAN_POINT('Ctrl Pts',(21.9104858170327,8.98496466461387,37.8322959656726));
#42658=CARTESIAN_POINT('Ctrl Pts',(21.9082817397875,8.98596199478974,37.8170768460204));
#42659=CARTESIAN_POINT('Ctrl Pts',(21.9073187629761,8.98638407430636,37.8106561834941));
#42660=CARTESIAN_POINT('Ctrl Pts',(21.9054072741554,8.98719659460326,37.7983356435837));
#42661=CARTESIAN_POINT('Ctrl Pts',(21.9044637230924,8.98758687487998,37.7924350630936));
#42662=CARTESIAN_POINT('Ctrl Pts',(21.9019246921422,8.98860972958084,37.7770167898633));
#42663=CARTESIAN_POINT('Ctrl Pts',(21.9002851971068,8.9892436824687,37.7675066127627));
#42664=CARTESIAN_POINT('Ctrl Pts',(21.8943600199353,8.99144719419011,37.7346127670919));
#42665=CARTESIAN_POINT('Ctrl Pts',(21.8897136488818,8.99302804768908,37.71129708652));
#42666=CARTESIAN_POINT('Ctrl Pts',(21.8836364454197,8.99493685725024,37.6834927496696));
#42667=CARTESIAN_POINT('Ctrl Pts',(21.8826184102268,8.99525188702551,37.6789151286036));
#42668=CARTESIAN_POINT('Ctrl Pts',(21.8328060834032,9.01044251524392,37.4587244877102));
#42669=CARTESIAN_POINT('Ctrl Pts',(21.7473247955972,9.02662360429059,37.253110031045));
#42670=CARTESIAN_POINT('Ctrl Pts',(21.6068857344155,9.04486668649835,37.0317503188578));
#42671=CARTESIAN_POINT('Ctrl Pts',(21.583709448555,9.04769209480757,36.997682387957));
#42672=CARTESIAN_POINT('Ctrl Pts',(21.5549181370492,9.05096919408511,36.9581455331121));
#42673=CARTESIAN_POINT('Ctrl Pts',(21.5503407009979,9.05148363503288,36.9519382628826));
#42674=CARTESIAN_POINT('Ctrl Pts',(21.543210800634,9.05227465113135,36.9423901113885));
#42675=CARTESIAN_POINT('Ctrl Pts',(21.5406844993102,9.05255296574694,36.9390299298318));
#42676=CARTESIAN_POINT('Ctrl Pts',(21.5360021763646,9.05306515595803,36.9328442682106));
#42677=CARTESIAN_POINT('Ctrl Pts',(21.5338493456925,9.05329923938201,36.9300165073158));
#42678=CARTESIAN_POINT('Ctrl Pts',(21.5289814439366,9.05382538694573,36.9236590074866));
#42679=CARTESIAN_POINT('Ctrl Pts',(21.5262619649147,9.05411713792295,36.920132718477));
#42680=CARTESIAN_POINT('Ctrl Pts',(21.5182400788114,9.05497146061535,36.9098050610497));
#42681=CARTESIAN_POINT('Ctrl Pts',(21.5129041607175,9.05553174500311,36.9030296842318));
#42682=CARTESIAN_POINT('Ctrl Pts',(21.4742794605666,9.05953245837888,36.8546562166427));
#42683=CARTESIAN_POINT('Ctrl Pts',(21.4393220807361,9.06286367324542,36.8144129055365));
#42684=CARTESIAN_POINT('Ctrl Pts',(21.3876762214856,9.06748088874049,36.7597094537792));
#42685=CARTESIAN_POINT('Ctrl Pts',(21.3723411088095,9.06881691676788,36.7440118093443));
#42686=CARTESIAN_POINT('Ctrl Pts',(21.2380857010789,9.08025248628564,36.6111935025206));
#42687=CARTESIAN_POINT('Ctrl Pts',(21.1047047731269,9.08995843329927,36.5097078479521));
#42688=CARTESIAN_POINT('Ctrl Pts',(20.9230890044272,9.10299529583187,36.4055229008584));
#42689=CARTESIAN_POINT('Ctrl Pts',(20.8855679655936,9.10567556289841,36.3856152986424));
#42690=CARTESIAN_POINT('Ctrl Pts',(20.8369982689855,9.10914373137084,36.3618656246571));
#42691=CARTESIAN_POINT('Ctrl Pts',(20.8265282337326,9.10989125050262,36.3568625188116));
#42692=CARTESIAN_POINT('Ctrl Pts',(20.8096149755404,9.11109891262312,36.3489671570532));
#42693=CARTESIAN_POINT('Ctrl Pts',(20.8031997872061,9.11155700565227,36.3460152436993));
#42694=CARTESIAN_POINT('Ctrl Pts',(20.7909512363762,9.11243176533418,36.3404604293796));
#42695=CARTESIAN_POINT('Ctrl Pts',(20.7851208590442,9.11284820728739,36.3378511430763));
#42696=CARTESIAN_POINT('Ctrl Pts',(20.7717775677259,9.11380144044364,36.3319589474194));
#42697=CARTESIAN_POINT('Ctrl Pts',(20.764256508982,9.11433886238197,36.328694898489));
#42698=CARTESIAN_POINT('Ctrl Pts',(20.7446029372759,9.11574365899821,36.3203139600039));
#42699=CARTESIAN_POINT('Ctrl Pts',(20.7324386048686,9.11661357532109,36.3152732392011));
#42700=CARTESIAN_POINT('Ctrl Pts',(20.6461070447136,9.12279157365804,36.2805299582289));
#42701=CARTESIAN_POINT('Ctrl Pts',(20.5702189862095,9.12824847194836,36.2553393763607));
#42702=CARTESIAN_POINT('Ctrl Pts',(20.3346190373906,9.14526108929534,36.193062999274));
#42703=CARTESIAN_POINT('Ctrl Pts',(20.1715716519762,9.15718905139255,36.1715458474117));
#42704=CARTESIAN_POINT('Ctrl Pts',(19.9702403675266,9.17116011690922,36.1707343852393));
#42705=CARTESIAN_POINT('Ctrl Pts',(19.932705896441,9.17372881788065,36.1716786030518));
#42706=CARTESIAN_POINT('Ctrl Pts',(19.8877131282004,9.17674677200587,36.1741259814492));
#42707=CARTESIAN_POINT('Ctrl Pts',(19.8802085451391,9.17724810198117,36.174578204958));
#42708=CARTESIAN_POINT('Ctrl Pts',(19.8685538603466,9.17802328825103,36.1753489172515));
#42709=CARTESIAN_POINT('Ctrl Pts',(19.8644019241899,9.17829877766179,36.1756369779577));
#42710=CARTESIAN_POINT('Ctrl Pts',(19.8567027268409,9.1788083561495,36.1761961886969));
#42711=CARTESIAN_POINT('Ctrl Pts',(19.8531553137936,9.17904263646819,36.1764637119729));
#42712=CARTESIAN_POINT('Ctrl Pts',(19.8451149639858,9.17957250526819,36.177092436318));
#42713=CARTESIAN_POINT('Ctrl Pts',(19.8406225489198,9.17986776065101,36.1774595707885));
#42714=CARTESIAN_POINT('Ctrl Pts',(19.8269897691844,9.18076143135048,36.1786217983355));
#42715=CARTESIAN_POINT('Ctrl Pts',(19.8178535894194,9.18135717177682,36.1794663692121));
#42716=CARTESIAN_POINT('Ctrl Pts',(19.7409610406316,9.18634704018642,36.1871281474852));
#42717=CARTESIAN_POINT('Ctrl Pts',(19.6735951110742,9.19056193509964,36.1974643286947));
#42718=CARTESIAN_POINT('Ctrl Pts',(19.5349075608324,9.19916953874482,36.2263296784686));
#42719=CARTESIAN_POINT('Ctrl Pts',(19.4638576286326,9.20354104659619,36.2454132542409));
#42720=CARTESIAN_POINT('Ctrl Pts',(19.3941038390373,9.20793124499895,36.2684890393365));
#42721=CARTESIAN_POINT('Origin',(20.,-1.3495818343519,38.1));
#42722=CARTESIAN_POINT('',(19.394104010895,10.1712205940279,36.2684889824829));
#42723=CARTESIAN_POINT('',(19.3941040084883,9.99997597504684,36.2684889832791));
#42724=CARTESIAN_POINT('',(19.3941040087494,-1.3495818343519,36.2684889831927));
#42725=CARTESIAN_POINT('',(18.0708705563808,9.53609590521103,38.1014651490007));
#42726=CARTESIAN_POINT('Ctrl Pts',(19.394104010895,10.1712205940279,36.2684889824829));
#42727=CARTESIAN_POINT('Ctrl Pts',(19.4649959241567,10.1665882905303,36.2450366933651));
#42728=CARTESIAN_POINT('Ctrl Pts',(19.5372003889732,10.162104549311,36.2257166576543));
#42729=CARTESIAN_POINT('Ctrl Pts',(19.76068220923,10.1484606807009,36.1796277861682));
#42730=CARTESIAN_POINT('Ctrl Pts',(19.9141540621807,10.1393618920268,36.1666798877873));
#42731=CARTESIAN_POINT('Ctrl Pts',(20.0892165160705,10.1282613971371,36.1728119526785));
#42732=CARTESIAN_POINT('Ctrl Pts',(20.1108860438118,10.1268758742603,36.1739372851868));
#42733=CARTESIAN_POINT('Ctrl Pts',(20.140886959719,10.1249398545048,36.1760032303887));
#42734=CARTESIAN_POINT('Ctrl Pts',(20.1492386658252,10.1243989897188,36.1766330246421));
#42735=CARTESIAN_POINT('Ctrl Pts',(20.1636122185678,10.1234647382788,36.1778111020717));
#42736=CARTESIAN_POINT('Ctrl Pts',(20.1696361243812,10.1230721654309,36.1783333532301));
#42737=CARTESIAN_POINT('Ctrl Pts',(20.1820756803133,10.1222593131199,36.1794707651238));
#42738=CARTESIAN_POINT('Ctrl Pts',(20.188490894217,10.1218389185514,36.1800897738471));
#42739=CARTESIAN_POINT('Ctrl Pts',(20.2034619842848,10.1208549953831,36.1816101041192));
#42740=CARTESIAN_POINT('Ctrl Pts',(20.2120151179916,10.1202906902932,36.182536530369));
#42741=CARTESIAN_POINT('Ctrl Pts',(20.2396113324032,10.1184627843337,36.1857124920675));
#42742=CARTESIAN_POINT('Ctrl Pts',(20.2586266572917,10.1171921451402,36.1881886963173));
#42743=CARTESIAN_POINT('Ctrl Pts',(20.3556989931151,10.1106465368118,36.2023042936129));
#42744=CARTESIAN_POINT('Ctrl Pts',(20.4330159749597,10.1052325321538,36.2184407885767));
#42745=CARTESIAN_POINT('Ctrl Pts',(20.6119589365952,10.0922429472052,36.2674017054927));
#42746=CARTESIAN_POINT('Ctrl Pts',(20.7122841736996,10.0845917594271,36.3040158994054));
#42747=CARTESIAN_POINT('Ctrl Pts',(20.8865847804673,10.0709400513689,36.3845402034327));
#42748=CARTESIAN_POINT('Ctrl Pts',(20.9616535051949,10.0649328293062,36.4254669184944));
#42749=CARTESIAN_POINT('Ctrl Pts',(21.0416775986849,10.0585623095673,36.4762580101657));
#42750=CARTESIAN_POINT('Ctrl Pts',(21.049548402247,10.0579361551078,36.4813343677029));
#42751=CARTESIAN_POINT('Ctrl Pts',(21.0611836815631,10.0570115109919,36.4889592155716));
#42752=CARTESIAN_POINT('Ctrl Pts',(21.0649764788323,10.0567102588818,36.491463921545));
#42753=CARTESIAN_POINT('Ctrl Pts',(21.0717245704979,10.0561746075507,36.4959545895044));
#42754=CARTESIAN_POINT('Ctrl Pts',(21.0746832454251,10.0559398706551,36.4979353456665));
#42755=CARTESIAN_POINT('Ctrl Pts',(21.0810658284941,10.0554337477318,36.5022339576626));
#42756=CARTESIAN_POINT('Ctrl Pts',(21.0844877666132,10.0551625539207,36.5045546275588));
#42757=CARTESIAN_POINT('Ctrl Pts',(21.0940071958797,10.0544084847684,36.5110552361693));
#42758=CARTESIAN_POINT('Ctrl Pts',(21.1000882410997,10.0539271965464,36.5152593040997));
#42759=CARTESIAN_POINT('Ctrl Pts',(21.1351424913628,10.0511542661278,36.5397927082321));
#42760=CARTESIAN_POINT('Ctrl Pts',(21.1635781421165,10.0489106765686,36.5608828635199));
#42761=CARTESIAN_POINT('Ctrl Pts',(21.254653703138,10.0416859268719,36.6323996499693));
#42762=CARTESIAN_POINT('Ctrl Pts',(21.3147274912008,10.0368557999983,36.6859630531611));
#42763=CARTESIAN_POINT('Ctrl Pts',(21.4798171190979,10.0228199523344,36.8528060026792));
#42764=CARTESIAN_POINT('Ctrl Pts',(21.574782938254,10.0136768967401,36.9750982186026));
#42765=CARTESIAN_POINT('Ctrl Pts',(21.665304317528,10.0025277986846,37.1259503912495));
#42766=CARTESIAN_POINT('Ctrl Pts',(21.6761284926041,10.0011455352919,37.1446967357882));
#42767=CARTESIAN_POINT('Ctrl Pts',(21.6906959371529,9.99921335317547,37.1709360547496));
#42768=CARTESIAN_POINT('Ctrl Pts',(21.694709578797,9.99867301591924,37.1782776957265));
#42769=CARTESIAN_POINT('Ctrl Pts',(21.7015401442436,9.99773943156566,37.1909674215174));
#42770=CARTESIAN_POINT('Ctrl Pts',(21.7043799496864,9.99734699556814,37.1963031056026));
#42771=CARTESIAN_POINT('Ctrl Pts',(21.7101964736796,9.99653419687392,37.2073566598612));
#42772=CARTESIAN_POINT('Ctrl Pts',(21.7131696978256,9.99611371805557,37.2130762738291));
#42773=CARTESIAN_POINT('Ctrl Pts',(21.7200474771764,9.99512919826382,37.2264707324197));
#42774=CARTESIAN_POINT('Ctrl Pts',(21.7239293983343,9.99456437797395,37.234156982723));
#42775=CARTESIAN_POINT('Ctrl Pts',(21.7363085378277,9.99273310979356,37.2590811197142));
#42776=CARTESIAN_POINT('Ctrl Pts',(21.744599440101,9.9914595873496,37.2764196152406));
#42777=CARTESIAN_POINT('Ctrl Pts',(21.7857473129233,9.98488847437703,37.3658813017795));
#42778=CARTESIAN_POINT('Ctrl Pts',(21.8143921259442,9.9794506243686,37.4398469568211));
#42779=CARTESIAN_POINT('Ctrl Pts',(21.871046628862,9.96635915464611,37.6179963340078));
#42780=CARTESIAN_POINT('Ctrl Pts',(21.8950333370717,9.9586272905294,37.7231856738415));
#42781=CARTESIAN_POINT('Ctrl Pts',(21.9218704451539,9.94500781825628,37.9129166339437));
#42782=CARTESIAN_POINT('Ctrl Pts',(21.9281908260042,9.93910823600938,37.9967051917086));
#42783=CARTESIAN_POINT('Ctrl Pts',(21.9291267891915,9.93283719732254,38.090003750186));
#42784=CARTESIAN_POINT('Ctrl Pts',(21.9291525841898,9.93221167669767,38.0993601865164));
#42785=CARTESIAN_POINT('Ctrl Pts',(21.9290897784271,9.93128778414922,38.1132599052371));
#42786=CARTESIAN_POINT('Ctrl Pts',(21.9290532000281,9.93098665616662,38.1178031129038));
#42787=CARTESIAN_POINT('Ctrl Pts',(21.9289593299774,9.93045113961431,38.125906295107));
#42788=CARTESIAN_POINT('Ctrl Pts',(21.9289082332758,9.93021641405884,38.1294662714569));
#42789=CARTESIAN_POINT('Ctrl Pts',(21.9287764747286,9.92971021815369,38.1371614432153));
#42790=CARTESIAN_POINT('Ctrl Pts',(21.9286923706892,9.92943894053822,38.1412965176261));
#42791=CARTESIAN_POINT('Ctrl Pts',(21.928420731219,9.92868440134286,38.1528278205568));
#42792=CARTESIAN_POINT('Ctrl Pts',(21.928203942358,9.92820273009551,38.1602233859235));
#42793=CARTESIAN_POINT('Ctrl Pts',(21.9267005859875,9.92542308482274,38.2030877432137));
#42794=CARTESIAN_POINT('Ctrl Pts',(21.9244778427498,9.92317343600712,38.2385194939745));
#42795=CARTESIAN_POINT('Ctrl Pts',(21.9139970829203,9.9159190829748,38.3543312259466));
#42796=CARTESIAN_POINT('Ctrl Pts',(21.9016680714019,9.91106683073614,38.4342602797698));
#42797=CARTESIAN_POINT('Ctrl Pts',(21.8514305530821,9.8970416194577,38.6633715767694));
#42798=CARTESIAN_POINT('Ctrl Pts',(21.8006685042045,9.88792855439208,38.8090622710938));
#42799=CARTESIAN_POINT('Ctrl Pts',(21.7236352340713,9.87681237690304,38.9666569228625));
#42800=CARTESIAN_POINT('Ctrl Pts',(21.7137864337047,9.87542788984801,38.9859732735747));
#42801=CARTESIAN_POINT('Ctrl Pts',(21.6996860759464,9.87349308937315,39.0125129610778));
#42802=CARTESIAN_POINT('Ctrl Pts',(21.6957096331897,9.87295239194218,39.0198812408094));
#42803=CARTESIAN_POINT('Ctrl Pts',(21.6887795088047,9.87201835214705,39.0325250021952));
#42804=CARTESIAN_POINT('Ctrl Pts',(21.6858487375998,9.87162582273017,39.0378129566343));
#42805=CARTESIAN_POINT('Ctrl Pts',(21.6797422326439,9.87081298752134,39.0487097197133));
#42806=CARTESIAN_POINT('Ctrl Pts',(21.6765631534016,9.87039256630184,39.0543165572153));
#42807=CARTESIAN_POINT('Ctrl Pts',(21.6690740264862,9.8694084542222,39.0673719594894));
#42808=CARTESIAN_POINT('Ctrl Pts',(21.6647421442592,9.86884398597719,39.0748077774518));
#42809=CARTESIAN_POINT('Ctrl Pts',(21.6505906530725,9.86701501570477,39.098729828786));
#42810=CARTESIAN_POINT('Ctrl Pts',(21.6405750284971,9.86574346389546,39.1150981754499));
#42811=CARTESIAN_POINT('Ctrl Pts',(21.5880704421911,9.85918978854265,39.198098248913));
#42812=CARTESIAN_POINT('Ctrl Pts',(21.5417655895339,9.85376824297744,39.2622149037894));
#42813=CARTESIAN_POINT('Ctrl Pts',(21.42382340675,9.84074482274933,39.4060304183565));
#42814=CARTESIAN_POINT('Ctrl Pts',(21.3492198441774,9.83306642434861,39.4829648354101));
#42815=CARTESIAN_POINT('Ctrl Pts',(21.2046549156477,9.81942393050644,39.6091589882342));
#42816=CARTESIAN_POINT('Ctrl Pts',(21.1370525263523,9.81345144494535,39.660727217085));
#42817=CARTESIAN_POINT('Ctrl Pts',(21.0584688699067,9.80711368956272,39.7128464562181));
#42818=CARTESIAN_POINT('Ctrl Pts',(21.0506364875694,9.80648836383973,39.7179595234547));
#42819=CARTESIAN_POINT('Ctrl Pts',(21.0389451591874,9.80556470241084,39.7254710546045));
#42820=CARTESIAN_POINT('Ctrl Pts',(21.0351145726499,9.8052636126109,39.7279130860375));
#42821=CARTESIAN_POINT('Ctrl Pts',(21.0282664923011,9.80472813750468,39.7322448509045));
#42822=CARTESIAN_POINT('Ctrl Pts',(21.0252523671354,9.80449341542469,39.7341397788733));
#42823=CARTESIAN_POINT('Ctrl Pts',(21.0187251106484,9.80398719701102,39.738218182836));
#42824=CARTESIAN_POINT('Ctrl Pts',(21.0152102056271,9.80371589357096,39.7403987030064));
#42825=CARTESIAN_POINT('Ctrl Pts',(21.0053871895073,9.80296120951313,39.7464488821565));
#42826=CARTESIAN_POINT('Ctrl Pts',(20.9990637013461,9.80247942021881,39.750293624587));
#42827=CARTESIAN_POINT('Ctrl Pts',(20.9622601544136,9.79969770111211,39.7723814697535));
#42828=CARTESIAN_POINT('Ctrl Pts',(20.931300738835,9.79744618085657,39.7898176548111));
#42829=CARTESIAN_POINT('Ctrl Pts',(20.8283090852643,9.79018266543246,39.8441309247444));
#42830=CARTESIAN_POINT('Ctrl Pts',(20.7544333834276,9.78532356272082,39.8773353883116));
#42831=CARTESIAN_POINT('Ctrl Pts',(20.5349197014824,9.77130161209216,39.9598364114961));
#42832=CARTESIAN_POINT('Ctrl Pts',(20.3852352351913,9.76219781349318,39.9965015465132));
#42833=CARTESIAN_POINT('Ctrl Pts',(20.2112602955656,9.75109181437335,40.0176501751828));
#42834=CARTESIAN_POINT('Ctrl Pts',(20.1896847583094,9.74970665333064,40.0199043567324));
#42835=CARTESIAN_POINT('Ctrl Pts',(20.1597337905059,9.74777105946612,40.0225238114789));
#42836=CARTESIAN_POINT('Ctrl Pts',(20.1513865601794,9.74723025310996,40.0231991044382));
#42837=CARTESIAN_POINT('Ctrl Pts',(20.1370056597,9.74629607556473,40.0242683190484));
#42838=CARTESIAN_POINT('Ctrl Pts',(20.1309739989704,9.7459035178819,40.0246882668881));
#42839=CARTESIAN_POINT('Ctrl Pts',(20.1185088804897,9.74509067155156,40.0254972714536));
#42840=CARTESIAN_POINT('Ctrl Pts',(20.1120752556066,9.74467026768632,40.0258824555316));
#42841=CARTESIAN_POINT('Ctrl Pts',(20.0970487562776,9.74368627860025,40.0267065488306));
#42842=CARTESIAN_POINT('Ctrl Pts',(20.088454690224,9.74312191657721,40.0271202220249));
#42843=CARTESIAN_POINT('Ctrl Pts',(20.0606945402361,9.74129363927183,40.0282703670021));
#42844=CARTESIAN_POINT('Ctrl Pts',(20.0415206558564,9.74002268166886,40.0287784802007));
#42845=CARTESIAN_POINT('Ctrl Pts',(19.9433922951502,9.73347425938291,40.0299150673486));
#42846=CARTESIAN_POINT('Ctrl Pts',(19.8644702952461,9.72805762442425,40.025981678958));
#42847=CARTESIAN_POINT('Ctrl Pts',(19.6715366108952,9.71446481865499,40.0044484717718));
#42848=CARTESIAN_POINT('Ctrl Pts',(19.5584321425053,9.70618045046398,39.9814427942617));
#42849=CARTESIAN_POINT('Ctrl Pts',(19.3743846412666,9.69255631185649,39.9264886965181));
#42850=CARTESIAN_POINT('Ctrl Pts',(19.3020750178764,9.68717013762186,39.900099752653));
#42851=CARTESIAN_POINT('Ctrl Pts',(19.2230007051749,9.68137649435539,39.8657579258365));
#42852=CARTESIAN_POINT('Ctrl Pts',(19.2145015485332,9.68075509840767,39.8619935153268));
#42853=CARTESIAN_POINT('Ctrl Pts',(19.2019000544553,9.67983609853562,39.8563028115702));
#42854=CARTESIAN_POINT('Ctrl Pts',(19.1977769132116,9.67953578000136,39.8544233266439));
#42855=CARTESIAN_POINT('Ctrl Pts',(19.1904268798643,9.67900114077,39.8510415725895));
#42856=CARTESIAN_POINT('Ctrl Pts',(19.187197496407,9.6787664875804,39.8495448884342));
#42857=CARTESIAN_POINT('Ctrl Pts',(19.1802922818348,9.67826528684794,39.8463213640352));
#42858=CARTESIAN_POINT('Ctrl Pts',(19.1766177657984,9.67799890569718,39.8445918568131));
#42859=CARTESIAN_POINT('Ctrl Pts',(19.1665166372142,9.67726745677584,39.8397984735528));
#42860=CARTESIAN_POINT('Ctrl Pts',(19.1601014013035,9.67680383459057,39.8367105666686));
#42861=CARTESIAN_POINT('Ctrl Pts',(19.145729251475,9.67576692357286,39.8296944191807));
#42862=CARTESIAN_POINT('Ctrl Pts',(19.1377819946491,9.67519476332585,39.8257466250005));
#42863=CARTESIAN_POINT('Ctrl Pts',(19.113111069951,9.6734215000712,39.8132783914431));
#42864=CARTESIAN_POINT('Ctrl Pts',(19.0964838071241,9.67223058286875,39.8045683814513));
#42865=CARTESIAN_POINT('Ctrl Pts',(19.0311115708399,9.66755458028526,39.7690984584579));
#42866=CARTESIAN_POINT('Ctrl Pts',(18.9834029641842,9.66415558504402,39.7404773307421));
#42867=CARTESIAN_POINT('Ctrl Pts',(18.8350421150492,9.65341823802039,39.6425116137417));
#42868=CARTESIAN_POINT('Ctrl Pts',(18.7397166904998,9.64624241909166,39.5656587266026));
#42869=CARTESIAN_POINT('Ctrl Pts',(18.5976202782277,9.63415376555496,39.4269188401294));
#42870=CARTESIAN_POINT('Ctrl Pts',(18.5461681174707,9.62941539700512,39.3703358775547));
#42871=CARTESIAN_POINT('Ctrl Pts',(18.4900115667643,9.62369811854916,39.300686521365));
#42872=CARTESIAN_POINT('Ctrl Pts',(18.4819161749414,9.62285942838922,39.2904346591537));
#42873=CARTESIAN_POINT('Ctrl Pts',(18.4689295119072,9.62148968983956,39.2736406700217));
#42874=CARTESIAN_POINT('Ctrl Pts',(18.463974490419,9.62096114708986,39.2671481878404));
#42875=CARTESIAN_POINT('Ctrl Pts',(18.4552201706204,9.62001659735412,39.2555252439903));
#42876=CARTESIAN_POINT('Ctrl Pts',(18.4514048077431,9.61960122265204,39.2504069886976));
#42877=CARTESIAN_POINT('Ctrl Pts',(18.4434124302717,9.61872316185317,39.2395735189644));
#42878=CARTESIAN_POINT('Ctrl Pts',(18.4392413367565,9.61826025593173,39.2338540736025));
#42879=CARTESIAN_POINT('Ctrl Pts',(18.4282709743024,9.61703024767821,39.2186361680782));
#42880=CARTESIAN_POINT('Ctrl Pts',(18.4215264220232,9.61626107448402,39.209098805445));
#42881=CARTESIAN_POINT('Ctrl Pts',(18.3901798509238,9.61262382905547,39.1639070112198));
#42882=CARTESIAN_POINT('Ctrl Pts',(18.3666983929922,9.60971423449023,39.1274942298399));
#42883=CARTESIAN_POINT('Ctrl Pts',(18.281337322627,9.59838122471123,38.9847951859685));
#42884=CARTESIAN_POINT('Ctrl Pts',(18.2284540414812,9.58966000280737,38.8734860773268));
#42885=CARTESIAN_POINT('Ctrl Pts',(18.1688032042414,9.57717917568953,38.7090662829805));
#42886=CARTESIAN_POINT('Ctrl Pts',(18.1530600684469,9.57347048292888,38.6595145964407));
#42887=CARTESIAN_POINT('Ctrl Pts',(18.1340470662796,9.56838523903191,38.5900648133828));
#42888=CARTESIAN_POINT('Ctrl Pts',(18.1290585436424,9.56697651259576,38.5706612157791));
#42889=CARTESIAN_POINT('Ctrl Pts',(18.1134947759365,9.56232566692103,38.5059605850597));
#42890=CARTESIAN_POINT('Ctrl Pts',(18.1042545185894,9.55912236775163,38.4603551557423));
#42891=CARTESIAN_POINT('Ctrl Pts',(18.0954319979138,9.55549068614111,38.4069545475228));
#42892=CARTESIAN_POINT('Ctrl Pts',(18.0942369457064,9.55498272859598,38.3994454113471));
#42893=CARTESIAN_POINT('Ctrl Pts',(18.0923912445439,9.55417175310109,38.3873890902728));
#42894=CARTESIAN_POINT('Ctrl Pts',(18.0917123988027,9.55386722664874,38.3828463987725));
#42895=CARTESIAN_POINT('Ctrl Pts',(18.0905342963766,9.55332740788027,38.3747654478461));
#42896=CARTESIAN_POINT('Ctrl Pts',(18.0900286387866,9.55309176208119,38.371228178464));
#42897=CARTESIAN_POINT('Ctrl Pts',(18.0890687704878,9.55263666535322,38.3643777142746));
#42898=CARTESIAN_POINT('Ctrl Pts',(18.0886133485044,9.55241714493617,38.3610647594689));
#42899=CARTESIAN_POINT('Ctrl Pts',(18.0876307925645,9.55193545172768,38.3537767714693));
#42900=CARTESIAN_POINT('Ctrl Pts',(18.0871074311142,9.55167348782868,38.3498012327642));
#42901=CARTESIAN_POINT('Ctrl Pts',(18.0858454067869,9.55102810372736,38.3399781018139));
#42902=CARTESIAN_POINT('Ctrl Pts',(18.0851211340462,9.55064545435456,38.3341286546547));
#42903=CARTESIAN_POINT('Ctrl Pts',(18.0819461242232,9.54890974689848,38.3074855708987));
#42904=CARTESIAN_POINT('Ctrl Pts',(18.0798070880588,9.54757262754034,38.2866552908564));
#42905=CARTESIAN_POINT('Ctrl Pts',(18.0732936774698,9.54278424126604,38.2111472711882));
#42906=CARTESIAN_POINT('Ctrl Pts',(18.0709122189169,9.53941792722163,38.1563212933755));
#42907=CARTESIAN_POINT('Ctrl Pts',(18.0708705563808,9.53609590521103,38.1014651490007));
#42908=CARTESIAN_POINT('Ctrl Pts',(18.0708705582293,9.53609605247733,38.1014675807908));
#42909=CARTESIAN_POINT('Ctrl Pts',(18.0707475123805,9.52630106866043,37.9397242743709));
#42910=CARTESIAN_POINT('Ctrl Pts',(18.0909647819437,9.51688673489116,37.7786045611159));
#42911=CARTESIAN_POINT('Ctrl Pts',(18.1387402813931,9.50492507849212,37.5918503987071));
#42912=CARTESIAN_POINT('Ctrl Pts',(18.1471466991239,9.5029825872267,37.5620053481951));
#42913=CARTESIAN_POINT('Ctrl Pts',(18.1627822011627,9.49961511887058,37.5112186986139));
#42914=CARTESIAN_POINT('Ctrl Pts',(18.1696596305332,9.49820123441122,37.4901748373821));
#42915=CARTESIAN_POINT('Ctrl Pts',(18.1798769836897,9.49618870302921,37.4606426614083));
#42916=CARTESIAN_POINT('Ctrl Pts',(18.182917448527,9.49559985736207,37.4520520102845));
#42917=CARTESIAN_POINT('Ctrl Pts',(18.1882422042667,9.49458536469453,37.4373395004886));
#42918=CARTESIAN_POINT('Ctrl Pts',(18.1904969612513,9.49416069736462,37.4312070581813));
#42919=CARTESIAN_POINT('Ctrl Pts',(18.1948570029757,9.49334871223282,37.4195321702686));
#42920=CARTESIAN_POINT('Ctrl Pts',(18.1969567735783,9.49296158136236,37.4139877338231));
#42921=CARTESIAN_POINT('Ctrl Pts',(18.2024485930958,9.49195901337829,37.3996860044953));
#42922=CARTESIAN_POINT('Ctrl Pts',(18.2058790596842,9.49134230311789,37.3909437264771));
#42923=CARTESIAN_POINT('Ctrl Pts',(18.2176324755155,9.48926062737823,37.3616225052364));
#42924=CARTESIAN_POINT('Ctrl Pts',(18.2262464957679,9.48778597762043,37.3411628937835));
#42925=CARTESIAN_POINT('Ctrl Pts',(18.2930318561073,9.47671270814131,37.1898914672849));
#42926=CARTESIAN_POINT('Ctrl Pts',(18.3652402756797,9.46662090537987,37.0657933018514));
#42927=CARTESIAN_POINT('Ctrl Pts',(18.4920805803653,9.45142940711717,36.8947627891727));
#42928=CARTESIAN_POINT('Ctrl Pts',(18.5366881514936,9.4464400254975,36.8409778397677));
#42929=CARTESIAN_POINT('Ctrl Pts',(18.6092341047012,9.43894035552907,36.7625843765442));
#42930=CARTESIAN_POINT('Ctrl Pts',(18.635130367261,9.43636976574947,36.736166593274));
#42931=CARTESIAN_POINT('Ctrl Pts',(18.6720680551765,9.43286530381482,36.700591676009));
#42932=CARTESIAN_POINT('Ctrl Pts',(18.6824746359163,9.43189497741125,36.6907896361231));
#42933=CARTESIAN_POINT('Ctrl Pts',(18.7006119355222,9.43023429457237,36.674082535878));
#42934=CARTESIAN_POINT('Ctrl Pts',(18.708290979118,9.42954037513509,36.6671225545748));
#42935=CARTESIAN_POINT('Ctrl Pts',(18.7195805289102,9.42853398414788,36.6570546723713));
#42936=CARTESIAN_POINT('Ctrl Pts',(18.7231468886364,9.42821804744576,36.6538978688645));
#42937=CARTESIAN_POINT('Ctrl Pts',(18.7294285157419,9.42766509479738,36.6483789710895));
#42938=CARTESIAN_POINT('Ctrl Pts',(18.7321387537609,9.42742766441651,36.6460112210384));
#42939=CARTESIAN_POINT('Ctrl Pts',(18.7378414247173,9.42693049692422,36.641057256056));
#42940=CARTESIAN_POINT('Ctrl Pts',(18.7408351894679,9.42667087667347,36.6384726551028));
#42941=CARTESIAN_POINT('Ctrl Pts',(18.7488307319795,9.42598110222339,36.631612682091));
#42942=CARTESIAN_POINT('Ctrl Pts',(18.7538465256499,9.42555212272525,36.6273536154028));
#42943=CARTESIAN_POINT('Ctrl Pts',(18.7756221401123,9.4237053146275,36.6090541832584));
#42944=CARTESIAN_POINT('Ctrl Pts',(18.7925989584449,9.42230508157986,36.595272983099));
#42945=CARTESIAN_POINT('Ctrl Pts',(18.8136722356079,9.42060963220974,36.5787527779028));
#42946=CARTESIAN_POINT('Ctrl Pts',(18.8175488059204,9.42029947658223,36.5757376046465));
#42947=CARTESIAN_POINT('Ctrl Pts',(18.9576493762786,9.40915092542419,36.467624339207));
#42948=CARTESIAN_POINT('Ctrl Pts',(19.10732627959,9.39923735809111,36.3811939480628));
#42949=CARTESIAN_POINT('Ctrl Pts',(19.3084769628542,9.38604804867732,36.2985010871314));
#42950=CARTESIAN_POINT('Ctrl Pts',(19.3510383571465,9.38326871166235,36.2827358555299));
#42951=CARTESIAN_POINT('Ctrl Pts',(19.3941040511559,9.38044738890628,36.2684889691639));
#42952=CARTESIAN_POINT('Ctrl Pts',(19.3941038390373,9.20793124499895,36.2684890393365));
#42953=CARTESIAN_POINT('Ctrl Pts',(19.3501240934884,9.21069926390922,36.2830383156228));
#42954=CARTESIAN_POINT('Ctrl Pts',(19.3066595720485,9.21347421489961,36.2991746145473));
#42955=CARTESIAN_POINT('Ctrl Pts',(19.1874942354977,9.22127174790429,36.3483746531975));
#42956=CARTESIAN_POINT('Ctrl Pts',(19.1133014513578,9.22634940605603,36.3847390173774));
#42957=CARTESIAN_POINT('Ctrl Pts',(19.0246292538217,9.23284067912221,36.4354940588227));
#42958=CARTESIAN_POINT('Ctrl Pts',(19.0077381266876,9.23409693255132,36.4455077968246));
#42959=CARTESIAN_POINT('Ctrl Pts',(18.9836003409766,9.23592226083478,36.4603202351066));
#42960=CARTESIAN_POINT('Ctrl Pts',(18.9762282732511,9.23648386650944,36.4649130158542));
#42961=CARTESIAN_POINT('Ctrl Pts',(18.9634291409999,9.23746624533909,36.473007338139));
#42962=CARTESIAN_POINT('Ctrl Pts',(18.9579881373336,9.23788619852095,36.4764866665614));
#42963=CARTESIAN_POINT('Ctrl Pts',(18.9475059377085,9.23869982769704,36.4832640611803));
#42964=CARTESIAN_POINT('Ctrl Pts',(18.9424625107784,9.23909336789468,36.4865585524908));
#42965=CARTESIAN_POINT('Ctrl Pts',(18.9305160291075,9.24003053190812,36.4944423689675));
#42966=CARTESIAN_POINT('Ctrl Pts',(18.9236270063268,9.24057493237622,36.4990526412667));
#42967=CARTESIAN_POINT('Ctrl Pts',(18.8992506127762,9.24251561461815,36.5155942732559));
#42968=CARTESIAN_POINT('Ctrl Pts',(18.8819307013555,9.24392098794825,36.5277685591875));
#42969=CARTESIAN_POINT('Ctrl Pts',(18.734951916477,9.25608158223776,36.634737886082));
#42970=CARTESIAN_POINT('Ctrl Pts',(18.6174246854991,9.2674751429148,36.7450813449964));
#42971=CARTESIAN_POINT('Ctrl Pts',(18.4664009631485,9.28435420803083,36.9272248224959));
#42972=CARTESIAN_POINT('Ctrl Pts',(18.4213554586576,9.28976502358068,36.9885997210177));
#42973=CARTESIAN_POINT('Ctrl Pts',(18.361442343916,9.29740085717466,37.0812529312707));
#42974=CARTESIAN_POINT('Ctrl Pts',(18.3436038389566,9.29974083650397,37.110520896351));
#42975=CARTESIAN_POINT('Ctrl Pts',(18.3229101943336,9.3025256340672,37.1466029348882));
#42976=CARTESIAN_POINT('Ctrl Pts',(18.3193032091774,9.30301379832689,37.1529759867949));
#42977=CARTESIAN_POINT('Ctrl Pts',(18.3137239805373,9.30377306130415,37.162966002833));
#42978=CARTESIAN_POINT('Ctrl Pts',(18.3117269318189,9.30404568923033,37.1665689239666));
#42979=CARTESIAN_POINT('Ctrl Pts',(18.3080243513598,9.3045527124166,37.1732995886816));
#42980=CARTESIAN_POINT('Ctrl Pts',(18.3063159597765,9.30478728190548,37.1764256282661));
#42981=CARTESIAN_POINT('Ctrl Pts',(18.3024370637711,9.30532132677222,37.1835702462792));
#42982=CARTESIAN_POINT('Ctrl Pts',(18.300272167248,9.30562044715279,37.187591806487));
#42983=CARTESIAN_POINT('Ctrl Pts',(18.2946596981478,9.30639879380033,37.198106955948));
#42984=CARTESIAN_POINT('Ctrl Pts',(18.2912348885162,9.30687663117823,37.2046127061479));
#42985=CARTESIAN_POINT('Ctrl Pts',(18.2687690375852,9.31003148454768,37.247887103816));
#42986=CARTESIAN_POINT('Ctrl Pts',(18.2508772262192,9.31264253692699,37.2852441209302));
#42987=CARTESIAN_POINT('Ctrl Pts',(18.2278590751154,9.31618594056925,37.3375650386193));
#42988=CARTESIAN_POINT('Ctrl Pts',(18.2216943925456,9.31715562636448,37.3520563409197));
#42989=CARTESIAN_POINT('Ctrl Pts',(18.1694563902217,9.32557154291674,37.4791502036097));
#42990=CARTESIAN_POINT('Ctrl Pts',(18.1339517265813,9.33270997147971,37.5958062287506));
#42991=CARTESIAN_POINT('Ctrl Pts',(18.08945911872,9.34613947268664,37.8142821471299));
#42992=CARTESIAN_POINT('Ctrl Pts',(18.0770972984977,9.35234908399952,37.9149537258496));
#42993=CARTESIAN_POINT('Ctrl Pts',(18.0720603354054,9.35975131309222,38.0306902099867));
#42994=CARTESIAN_POINT('Ctrl Pts',(18.0715915218523,9.36068798874525,38.0452650025497));
#42995=CARTESIAN_POINT('Ctrl Pts',(18.0711275585347,9.36212757092115,38.0675490479106));
#42996=CARTESIAN_POINT('Ctrl Pts',(18.0710133057468,9.36262678064356,38.0752554998596));
#42997=CARTESIAN_POINT('Ctrl Pts',(18.0708946302922,9.36349964784425,38.0886922880725));
#42998=CARTESIAN_POINT('Ctrl Pts',(18.0708695531956,9.36387265932713,38.09442238259));
#42999=CARTESIAN_POINT('Ctrl Pts',(18.0708705727147,9.36471426490537,38.1073233343368));
#43000=CARTESIAN_POINT('Ctrl Pts',(18.0709111223382,9.36518330242469,38.114494074409));
#43001=CARTESIAN_POINT('Ctrl Pts',(18.0711275066883,9.36644699301404,38.1337610907952));
#43002=CARTESIAN_POINT('Ctrl Pts',(18.0713771447937,9.36724392313439,38.1458560553616));
#43003=CARTESIAN_POINT('Ctrl Pts',(18.0731898140528,9.37123704769623,38.2061742407294));
#43004=CARTESIAN_POINT('Ctrl Pts',(18.0764477118004,9.37448529224399,38.254325489858));
#43005=CARTESIAN_POINT('Ctrl Pts',(18.091252879719,9.38414275486742,38.3947285053799));
#43006=CARTESIAN_POINT('Ctrl Pts',(18.1076646370504,9.39068615082627,38.4863206825209));
#43007=CARTESIAN_POINT('Ctrl Pts',(18.1637587715744,9.40685838216643,38.7064504052619));
#43008=CARTESIAN_POINT('Ctrl Pts',(18.2103980126566,9.41653568545989,38.8327306887193));
#43009=CARTESIAN_POINT('Ctrl Pts',(18.2759986406667,9.42658321504773,38.9657712415146));
#43010=CARTESIAN_POINT('Ctrl Pts',(18.2823592781132,9.427529290171,38.9783227814374));
#43011=CARTESIAN_POINT('Ctrl Pts',(18.291406939334,9.4288355583237,38.9957024096441));
#43012=CARTESIAN_POINT('Ctrl Pts',(18.2939780404203,9.42920249014677,39.0005898782935));
#43013=CARTESIAN_POINT('Ctrl Pts',(18.2981434198537,9.42979005366411,39.0084260966459));
#43014=CARTESIAN_POINT('Ctrl Pts',(18.2997244337548,9.43001150196547,39.0113818034794));
#43015=CARTESIAN_POINT('Ctrl Pts',(18.3030520117823,9.43047429538931,39.0175639171299));
#43016=CARTESIAN_POINT('Ctrl Pts',(18.3048000854554,9.43071553836563,39.0207894801605));
#43017=CARTESIAN_POINT('Ctrl Pts',(18.3090759026668,9.43130112875833,39.0286258138788));
#43018=CARTESIAN_POINT('Ctrl Pts',(18.3116133407053,9.43164486778196,39.033231319371));
#43019=CARTESIAN_POINT('Ctrl Pts',(18.320697231118,9.43286233329601,39.0495604582404));
#43020=CARTESIAN_POINT('Ctrl Pts',(18.327347400683,9.43372975646454,39.0612263832182));
#43021=CARTESIAN_POINT('Ctrl Pts',(18.3690521875225,9.43903129738863,39.132642518273));
#43022=CARTESIAN_POINT('Ctrl Pts',(18.4071862134468,9.44329290629607,39.1905446988378));
#43023=CARTESIAN_POINT('Ctrl Pts',(18.5308569171335,9.45588991037731,39.3579501809029));
#43024=CARTESIAN_POINT('Ctrl Pts',(18.6251696972001,9.46401018240935,39.4603906310022));
#43025=CARTESIAN_POINT('Ctrl Pts',(18.7788142338452,9.47651626133117,39.5948288697938));
#43026=CARTESIAN_POINT('Ctrl Pts',(18.8301130726918,9.48058797385536,39.6353081805357));
#43027=CARTESIAN_POINT('Ctrl Pts',(18.8935671672071,9.48556432962506,39.6803498255568));
#43028=CARTESIAN_POINT('Ctrl Pts',(18.9038426363326,9.4863683165942,39.687494317102));
#43029=CARTESIAN_POINT('Ctrl Pts',(18.92079998754,9.48769247323145,39.6990415585192));
#43030=CARTESIAN_POINT('Ctrl Pts',(18.9274411413075,9.48821040876076,39.7035036838841));
#43031=CARTESIAN_POINT('Ctrl Pts',(18.9394158032488,9.48914322348645,39.7114416663877));
#43032=CARTESIAN_POINT('Ctrl Pts',(18.9447391513668,9.48955752978617,39.7149326989978));
#43033=CARTESIAN_POINT('Ctrl Pts',(18.9561005762446,9.4904410202715,39.7223033190187));
#43034=CARTESIAN_POINT('Ctrl Pts',(18.9621432050364,9.49091046348663,39.7261756782787));
#43035=CARTESIAN_POINT('Ctrl Pts',(18.9784523136573,9.4921763857583,39.7364992818736));
#43036=CARTESIAN_POINT('Ctrl Pts',(18.9887581036584,9.4929751558104,39.7428875161686));
#43037=CARTESIAN_POINT('Ctrl Pts',(19.0406676854646,9.49699330920741,39.7743911456416));
#43038=CARTESIAN_POINT('Ctrl Pts',(19.0831465328743,9.50026553160234,39.7980233223761));
#43039=CARTESIAN_POINT('Ctrl Pts',(19.2739225980985,9.51490566946668,39.894910734128));
#43040=CARTESIAN_POINT('Ctrl Pts',(19.4303813035583,9.52684801110277,39.9505165372845));
#43041=CARTESIAN_POINT('Ctrl Pts',(19.6593145691804,9.54341439066651,40.0000587903222));
#43042=CARTESIAN_POINT('Ctrl Pts',(19.7273979016863,9.54822056535423,40.011015509051));
#43043=CARTESIAN_POINT('Ctrl Pts',(19.8050739201912,9.55346924639649,40.0192787607443));
#43044=CARTESIAN_POINT('Ctrl Pts',(19.8142261826906,9.55408398824943,40.0201862501002));
#43045=CARTESIAN_POINT('Ctrl Pts',(19.8278775622705,9.55499508778264,40.0214413284848));
#43046=CARTESIAN_POINT('Ctrl Pts',(19.8323718113926,9.55529409381009,40.0218386258454));
#43047=CARTESIAN_POINT('Ctrl Pts',(19.8404125411351,9.55582731587694,40.02252101625));
#43048=CARTESIAN_POINT('Ctrl Pts',(19.843958442719,9.55606185711737,40.0228120677918));
#43049=CARTESIAN_POINT('Ctrl Pts',(19.8516508212141,9.55656934484548,40.0234220473183));
#43050=CARTESIAN_POINT('Ctrl Pts',(19.8557975207638,9.55684208958325,40.0237373772804));
#43051=CARTESIAN_POINT('Ctrl Pts',(19.8674284938225,9.55760487386947,40.0245840195274));
#43052=CARTESIAN_POINT('Ctrl Pts',(19.8749149954767,9.55809326623989,40.0250850886677));
#43053=CARTESIAN_POINT('Ctrl Pts',(19.9196068272948,9.56099437596235,40.0278144824805));
#43054=CARTESIAN_POINT('Ctrl Pts',(19.9568703169092,9.56335369628595,40.0290080389433));
#43055=CARTESIAN_POINT('Ctrl Pts',(20.1551208361316,9.57569958374174,40.0296094488459));
#43056=CARTESIAN_POINT('Ctrl Pts',(20.3155344280209,9.58501443592247,40.0099485250386));
#43057=CARTESIAN_POINT('Ctrl Pts',(20.5519671952843,9.59980926224643,39.9503337818635));
#43058=CARTESIAN_POINT('Ctrl Pts',(20.6308837347644,9.60492930420942,39.9249345229931));
#43059=CARTESIAN_POINT('Ctrl Pts',(20.7202482928829,9.61106662166177,39.8896817176314));
#43060=CARTESIAN_POINT('Ctrl Pts',(20.7325279212618,9.61191749704039,39.8846907531358));
#43061=CARTESIAN_POINT('Ctrl Pts',(20.7523424551433,9.61330321274557,39.8763983340653));
#43062=CARTESIAN_POINT('Ctrl Pts',(20.7599095249537,9.61383544877372,39.8731744757692));
#43063=CARTESIAN_POINT('Ctrl Pts',(20.773319057722,9.61478413761193,39.8673599054797));
#43064=CARTESIAN_POINT('Ctrl Pts',(20.7791697341692,9.61519993739894,39.8647883511207));
#43065=CARTESIAN_POINT('Ctrl Pts',(20.7914454097769,9.61607636742363,39.859319866422));
#43066=CARTESIAN_POINT('Ctrl Pts',(20.7978675153779,9.61653720475634,39.8564167087384));
#43067=CARTESIAN_POINT('Ctrl Pts',(20.8147636308329,9.61775586695601,39.8486669141415));
#43068=CARTESIAN_POINT('Ctrl Pts',(20.8252101779364,9.61851569503189,39.8437614238165));
#43069=CARTESIAN_POINT('Ctrl Pts',(20.8732730865031,9.6220415266545,39.820663423926));
#43070=CARTESIAN_POINT('Ctrl Pts',(20.9103336133401,9.62484601927103,39.801346747986));
#43071=CARTESIAN_POINT('Ctrl Pts',(21.0926750039765,9.63909265958647,39.6986429059937));
#43072=CARTESIAN_POINT('Ctrl Pts',(21.2272707971901,9.65116003616743,39.5977936628705));
#43073=CARTESIAN_POINT('Ctrl Pts',(21.354481044171,9.66375609817016,39.4736918323114));
#43074=CARTESIAN_POINT('Ctrl Pts',(21.3617790717965,9.66448314261507,39.4664574318117));
#43075=CARTESIAN_POINT('Ctrl Pts',(21.3817771862801,9.66648697180734,39.4463143298881));
#43076=CARTESIAN_POINT('Ctrl Pts',(21.3943540842626,9.66776031289888,39.433284360277));
#43077=CARTESIAN_POINT('Ctrl Pts',(21.4392335800274,9.67234696863018,39.3854583964633));
#43078=CARTESIAN_POINT('Ctrl Pts',(21.4704353312311,9.6756185948558,39.3496469023362));
#43079=CARTESIAN_POINT('Ctrl Pts',(21.5050923871608,9.67931811399798,39.3067716892547));
#43080=CARTESIAN_POINT('Ctrl Pts',(21.5098630480204,9.67982888795917,39.3007974786973));
#43081=CARTESIAN_POINT('Ctrl Pts',(21.5174504235336,9.68064348096734,39.2911792382944));
#43082=CARTESIAN_POINT('Ctrl Pts',(21.5202897642299,9.68094882949931,39.287553282802));
#43083=CARTESIAN_POINT('Ctrl Pts',(21.5253099315662,9.68148957070916,39.2810948090356));
#43084=CARTESIAN_POINT('Ctrl Pts',(21.5274959004492,9.68172532131815,39.2782663579121));
#43085=CARTESIAN_POINT('Ctrl Pts',(21.5321395100343,9.68222673180104,39.2722232942386));
#43086=CARTESIAN_POINT('Ctrl Pts',(21.5345948990082,9.68249223540639,39.2690070258332));
#43087=CARTESIAN_POINT('Ctrl Pts',(21.5412649181824,9.68321456880345,39.260212861489));
#43088=CARTESIAN_POINT('Ctrl Pts',(21.5454594271367,9.68367002167998,39.2546196753557));
#43089=CARTESIAN_POINT('Ctrl Pts',(21.5671680990639,9.68603427071463,39.2253419033744));
#43090=CARTESIAN_POINT('Ctrl Pts',(21.5841696012473,9.68791007500744,39.2012797802326));
#43091=CARTESIAN_POINT('Ctrl Pts',(21.6337956154844,9.69349178594968,39.1275154347867));
#43092=CARTESIAN_POINT('Ctrl Pts',(21.6646821873011,9.69711466392501,39.0766833731836));
#43093=CARTESIAN_POINT('Ctrl Pts',(21.7391969249331,9.7064840516289,38.9402138314247));
#43094=CARTESIAN_POINT('Ctrl Pts',(21.7788617621778,9.71215736207527,38.8526064159828));
#43095=CARTESIAN_POINT('Ctrl Pts',(21.8448967637367,9.72375810818517,38.6719857594255));
#43096=CARTESIAN_POINT('Ctrl Pts',(21.8711359817914,9.72967094720642,38.5792266550017));
#43097=CARTESIAN_POINT('Ctrl Pts',(21.8930569864779,9.73668660347681,38.4715683434059));
#43098=CARTESIAN_POINT('Ctrl Pts',(21.8956312137392,9.73755995052958,38.4582039560962));
#43099=CARTESIAN_POINT('Ctrl Pts',(21.899536911396,9.7389693187787,38.436704628201));
#43100=CARTESIAN_POINT('Ctrl Pts',(21.9009580567887,9.73950251404045,38.4285862858861));
#43101=CARTESIAN_POINT('Ctrl Pts',(21.9033922207678,9.74045343780786,38.4141364703876));
#43102=CARTESIAN_POINT('Ctrl Pts',(21.904425783656,9.74087051325671,38.4078085460165));
#43103=CARTESIAN_POINT('Ctrl Pts',(21.9065171595972,9.74174312251042,38.3945903448051));
#43104=CARTESIAN_POINT('Ctrl Pts',(21.9075692079511,9.74219883097318,38.3876992628191));
#43105=CARTESIAN_POINT('Ctrl Pts',(21.9102131191753,9.74338934335397,38.3697289006122));
#43106=CARTESIAN_POINT('Ctrl Pts',(21.9117459284203,9.74412598641252,38.3586413283726));
#43107=CARTESIAN_POINT('Ctrl Pts',(21.9180861499256,9.74739134347441,38.3096393981654));
#43108=CARTESIAN_POINT('Ctrl Pts',(21.9218624632354,9.74995193652486,38.2716026716396));
#43109=CARTESIAN_POINT('Ctrl Pts',(21.9290060262769,9.75696062438339,38.1686080392972));
#43110=CARTESIAN_POINT('Ctrl Pts',(21.9302220588169,9.76146926708123,38.1035552679438));
#43111=CARTESIAN_POINT('Ctrl Pts',(21.9237787942949,9.77570506015676,37.9013131273564));
#43112=CARTESIAN_POINT('Ctrl Pts',(21.9047630966813,9.78564853995499,37.7649225774155));
#43113=CARTESIAN_POINT('Ctrl Pts',(21.8604264278452,9.798403124821,37.5877398233219));
#43114=CARTESIAN_POINT('Ctrl Pts',(21.8478764530512,9.80152241654691,37.544166973035));
#43115=CARTESIAN_POINT('Ctrl Pts',(21.8314587178022,9.80507025048261,37.4938989527412));
#43116=CARTESIAN_POINT('Ctrl Pts',(21.8290735058185,9.80557439506994,37.4867385309838));
#43117=CARTESIAN_POINT('Ctrl Pts',(21.8251745025519,9.80638046926953,37.4752588248066));
#43118=CARTESIAN_POINT('Ctrl Pts',(21.8236872847086,9.80668387918572,37.470930695861));
#43119=CARTESIAN_POINT('Ctrl Pts',(21.8210121206036,9.80722244751244,37.4632346059124));
#43120=CARTESIAN_POINT('Ctrl Pts',(21.8198302094704,9.80745795336688,37.4598646080818));
#43121=CARTESIAN_POINT('Ctrl Pts',(21.8172832850434,9.8079602648716,37.4526665968217));
#43122=CARTESIAN_POINT('Ctrl Pts',(21.8159155341989,9.80822690691791,37.4488396154719));
#43123=CARTESIAN_POINT('Ctrl Pts',(21.8121349156973,9.80895556507878,37.4383659595681));
#43124=CARTESIAN_POINT('Ctrl Pts',(21.8096975521361,9.809416163433,37.4317281019501));
#43125=CARTESIAN_POINT('Ctrl Pts',(21.7965391787765,9.81185547899812,37.3964928766794));
#43126=CARTESIAN_POINT('Ctrl Pts',(21.7851760064855,9.81379866232296,37.3681378726281));
#43127=CARTESIAN_POINT('Ctrl Pts',(21.7094715498149,9.82584996041843,37.1914984530761));
#43128=CARTESIAN_POINT('Ctrl Pts',(21.6273749496718,9.835205202887,37.0515101290951));
#43129=CARTESIAN_POINT('Ctrl Pts',(21.4742835165198,9.85038971055659,36.8525983324099));
#43130=CARTESIAN_POINT('Ctrl Pts',(21.4149537175753,9.85589457628662,36.785684336338));
#43131=CARTESIAN_POINT('Ctrl Pts',(21.3416129671817,9.86245768215677,36.7137107427696));
#43132=CARTESIAN_POINT('Ctrl Pts',(21.3319207117148,9.86332042857703,36.7043960226969));
#43133=CARTESIAN_POINT('Ctrl Pts',(21.3161661976289,9.86471596343047,36.6895687841902));
#43134=CARTESIAN_POINT('Ctrl Pts',(21.3101646724415,9.86524601509756,36.6839921603347));
#43135=CARTESIAN_POINT('Ctrl Pts',(21.2994083428786,9.86619334422087,36.6741242915941));
#43136=CARTESIAN_POINT('Ctrl Pts',(21.2946673178167,9.86660998597644,36.6698181542562));
#43137=CARTESIAN_POINT('Ctrl Pts',(21.2847036890168,9.86748375082805,36.6608586180118));
#43138=CARTESIAN_POINT('Ctrl Pts',(21.2794770520499,9.8679410588422,36.6562098639211));
#43139=CARTESIAN_POINT('Ctrl Pts',(21.2657399517664,9.86914035445502,36.6441247795574));
#43140=CARTESIAN_POINT('Ctrl Pts',(21.2571893202924,9.86988423181042,36.6367347175733));
#43141=CARTESIAN_POINT('Ctrl Pts',(21.2186190101163,9.87322854541444,36.6039871532445));
#43142=CARTESIAN_POINT('Ctrl Pts',(21.1878955283131,9.87586279354813,36.5794768789033));
#43143=CARTESIAN_POINT('Ctrl Pts',(21.0252313208048,9.8896709579344,36.4576484044795));
#43144=CARTESIAN_POINT('Ctrl Pts',(20.8820395217641,9.90145038697358,36.376513317007));
#43145=CARTESIAN_POINT('Ctrl Pts',(20.6553671038989,9.91884322396282,36.2837949765454));
#43146=CARTESIAN_POINT('Ctrl Pts',(20.57851074932,9.92453015371424,36.257872082175));
#43147=CARTESIAN_POINT('Ctrl Pts',(20.4912302176463,9.9306039082824,36.2344377463513));
#43148=CARTESIAN_POINT('Ctrl Pts',(20.4821994595275,9.93122781836522,36.2320831552781));
#43149=CARTESIAN_POINT('Ctrl Pts',(20.4687518010566,9.93214980037734,36.2286809719913));
#43150=CARTESIAN_POINT('Ctrl Pts',(20.4643478815609,9.93245061215031,36.2275833258816));
#43151=CARTESIAN_POINT('Ctrl Pts',(20.4564828062857,9.93298578506149,36.2256524661782));
#43152=CARTESIAN_POINT('Ctrl Pts',(20.453023188383,9.93322048143339,36.2248132835683));
#43153=CARTESIAN_POINT('Ctrl Pts',(20.4455359639117,9.93372686260932,36.2230190745426));
#43154=CARTESIAN_POINT('Ctrl Pts',(20.4415076097524,9.93399835336069,36.2220674343853));
#43155=CARTESIAN_POINT('Ctrl Pts',(20.4302556048344,9.93475409051943,36.2194475187775));
#43156=CARTESIAN_POINT('Ctrl Pts',(20.4230252582531,9.93523673838637,36.2178078856434));
#43157=CARTESIAN_POINT('Ctrl Pts',(20.3808815217012,9.93803361802056,36.2085060240188));
#43158=CARTESIAN_POINT('Ctrl Pts',(20.3457674428849,9.94029882119903,36.2017730735065));
#43159=CARTESIAN_POINT('Ctrl Pts',(20.2297596889918,9.94762961023454,36.1828555795166));
#43160=CARTESIAN_POINT('Ctrl Pts',(20.1482729411872,9.95253904933887,36.1748377686137));
#43161=CARTESIAN_POINT('Ctrl Pts',(19.9142629416303,9.96653750933651,36.1667641825865));
#43162=CARTESIAN_POINT('Ctrl Pts',(19.7619420073179,9.97557349499058,36.179564193676));
#43163=CARTESIAN_POINT('Ctrl Pts',(19.5913941629291,9.98660491492779,36.2145139468371));
#43164=CARTESIAN_POINT('Ctrl Pts',(19.570145896334,9.98799482265803,36.2192443605353));
#43165=CARTESIAN_POINT('Ctrl Pts',(19.540828806502,9.98993600010771,36.2262938583384));
#43166=CARTESIAN_POINT('Ctrl Pts',(19.5326877089189,9.99047756939347,36.2283076884247));
#43167=CARTESIAN_POINT('Ctrl Pts',(19.5186972911352,9.99141271124057,36.2318654077675));
#43168=CARTESIAN_POINT('Ctrl Pts',(19.5128415785039,9.99180546637457,36.2333838575541));
#43169=CARTESIAN_POINT('Ctrl Pts',(19.5007637399878,9.99261838949213,36.2365764757403));
#43170=CARTESIAN_POINT('Ctrl Pts',(19.4945426735608,9.99303867122441,36.2382543236148));
#43171=CARTESIAN_POINT('Ctrl Pts',(19.4800451010952,9.99402179834448,36.2422424008804));
#43172=CARTESIAN_POINT('Ctrl Pts',(19.4717754453974,9.99458541646026,36.24457681111));
#43173=CARTESIAN_POINT('Ctrl Pts',(19.4451575598474,9.99640885071204,36.2522830479233));
#43174=CARTESIAN_POINT('Ctrl Pts',(19.4268739802495,9.99767565715358,36.2578722657269));
#43175=CARTESIAN_POINT('Ctrl Pts',(19.4038129569931,9.9992922053214,36.2652984767808));
#43176=CARTESIAN_POINT('Ctrl Pts',(19.3989552455726,9.99963378453239,36.2668841089014));
#43177=CARTESIAN_POINT('Ctrl Pts',(19.3941040084883,9.99997597504683,36.2684889832791));
#43178=CARTESIAN_POINT('Origin',(20.,-1.3495818343519,38.1));
#43179=CARTESIAN_POINT('',(19.394104009089,10.9665681892825,36.2684889830804));
#43180=CARTESIAN_POINT('',(19.3941039816494,10.7965035432258,36.2684889921579));
#43181=CARTESIAN_POINT('',(19.3941040087494,-1.3495818343519,36.2684889831927));
#43182=CARTESIAN_POINT('Ctrl Pts',(19.394104009089,10.9665681892825,36.2684889830804));
#43183=CARTESIAN_POINT('Ctrl Pts',(19.4101221984477,10.9653651090697,36.2631898848907));
#43184=CARTESIAN_POINT('Ctrl Pts',(19.4262144753514,10.9641606506422,36.258099414377));
#43185=CARTESIAN_POINT('Ctrl Pts',(19.5196416320679,10.9571968227119,36.2298897070823));
#43186=CARTESIAN_POINT('Ctrl Pts',(19.5982993265924,10.95144387542,36.2114304642891));
#43187=CARTESIAN_POINT('Ctrl Pts',(19.7128602090028,10.9433946150564,36.1920294699323));
#43188=CARTESIAN_POINT('Ctrl Pts',(19.747993522783,10.940970414967,36.1870718960526));
#43189=CARTESIAN_POINT('Ctrl Pts',(19.7905966448415,10.9380994983931,36.1822545757917));
#43190=CARTESIAN_POINT('Ctrl Pts',(19.7979519890166,10.9376063072648,36.1814656941188));
#43191=CARTESIAN_POINT('Ctrl Pts',(19.8094263256921,10.936840960956,36.1803017594435));
#43192=CARTESIAN_POINT('Ctrl Pts',(19.8135421967924,10.9365672372366,36.1798976202932));
#43193=CARTESIAN_POINT('Ctrl Pts',(19.8212038404275,10.9360592462178,36.1791701880052));
#43194=CARTESIAN_POINT('Ctrl Pts',(19.8247491746223,10.9358247981512,36.1788434780454));
#43195=CARTESIAN_POINT('Ctrl Pts',(19.8328211111554,10.9352924017041,36.1781221628661));
#43196=CARTESIAN_POINT('Ctrl Pts',(19.8373482090237,10.9349947997234,36.1777337339283));
#43197=CARTESIAN_POINT('Ctrl Pts',(19.8512032315691,10.934086909952,36.1765942572462));
#43198=CARTESIAN_POINT('Ctrl Pts',(19.860535454784,10.9334794233235,36.1758950707573));
#43199=CARTESIAN_POINT('Ctrl Pts',(19.9538653747992,10.9274410514853,36.1695852306295));
#43200=CARTESIAN_POINT('Ctrl Pts',(20.0381517457064,10.9222854391081,36.1694099671297));
#43201=CARTESIAN_POINT('Ctrl Pts',(20.229485091364,10.9107293279815,36.1815532947513));
#43202=CARTESIAN_POINT('Ctrl Pts',(20.3360223335846,10.9043925548724,36.1973201822815));
#43203=CARTESIAN_POINT('Ctrl Pts',(20.5177879137346,10.8930812134614,36.2399706261514));
#43204=CARTESIAN_POINT('Ctrl Pts',(20.5936885372475,10.8882011082911,36.2627887092187));
#43205=CARTESIAN_POINT('Ctrl Pts',(20.6859889230014,10.8819474425503,36.2968553043621));
#43206=CARTESIAN_POINT('Ctrl Pts',(20.7039100772579,10.8807180243232,36.303775582863));
#43207=CARTESIAN_POINT('Ctrl Pts',(20.7297086820844,10.878924756756,36.3141831225778));
#43208=CARTESIAN_POINT('Ctrl Pts',(20.7376712059795,10.8783680108792,36.3174574708248));
#43209=CARTESIAN_POINT('Ctrl Pts',(20.751556551582,10.8773912850768,36.3232763697998));
#43210=CARTESIAN_POINT('Ctrl Pts',(20.7574890771275,10.8769720971749,36.3257975299611));
#43211=CARTESIAN_POINT('Ctrl Pts',(20.7689601125839,10.8761578596574,36.3307404256888));
#43212=CARTESIAN_POINT('Ctrl Pts',(20.7745001015519,10.8757629359982,36.3331585562541));
#43213=CARTESIAN_POINT('Ctrl Pts',(20.787682648531,10.8748191356231,36.3389864744886));
#43214=CARTESIAN_POINT('Ctrl Pts',(20.7953145118461,10.8742694564744,36.3424200116768));
#43215=CARTESIAN_POINT('Ctrl Pts',(20.8226145052806,10.8722912389195,36.3549163629026));
#43216=CARTESIAN_POINT('Ctrl Pts',(20.8421514404493,10.8708531435323,36.3642602696513));
#43217=CARTESIAN_POINT('Ctrl Pts',(20.9995085046073,10.859082377676,36.4428012950546));
#43218=CARTESIAN_POINT('Ctrl Pts',(21.1287088513431,10.8481674527666,36.5279558749053));
#43219=CARTESIAN_POINT('Ctrl Pts',(21.3077920852644,10.8314256446526,36.6795430326499));
#43220=CARTESIAN_POINT('Ctrl Pts',(21.3659039263688,10.8256903006591,36.7353292535059));
#43221=CARTESIAN_POINT('Ctrl Pts',(21.4443266760484,10.8176622043977,36.8206576048344));
#43222=CARTESIAN_POINT('Ctrl Pts',(21.4675684444316,10.8152422396944,36.8473868264596));
#43223=CARTESIAN_POINT('Ctrl Pts',(21.4947587965076,10.8123756463806,36.880453624013));
#43224=CARTESIAN_POINT('Ctrl Pts',(21.4994219816135,10.8118827028729,36.886191552044));
#43225=CARTESIAN_POINT('Ctrl Pts',(21.5066414173815,10.811117656114,36.8951799748754));
#43226=CARTESIAN_POINT('Ctrl Pts',(21.5092203396905,10.8108439862713,36.8984120420991));
#43227=CARTESIAN_POINT('Ctrl Pts',(21.5140006069857,10.8103360431425,36.9044426420881));
#43228=CARTESIAN_POINT('Ctrl Pts',(21.516204575146,10.8101015894098,36.907238950739));
#43229=CARTESIAN_POINT('Ctrl Pts',(21.5212042455725,10.8095691133296,36.9136185877445));
#43230=CARTESIAN_POINT('Ctrl Pts',(21.5239950305894,10.8092714377985,36.9172056984092));
#43231=CARTESIAN_POINT('Ctrl Pts',(21.5324968523229,10.8083631002682,36.9282134856119));
#43232=CARTESIAN_POINT('Ctrl Pts',(21.538166663832,10.8077552434553,36.9356660442437));
#43233=CARTESIAN_POINT('Ctrl Pts',(21.5948052835147,10.8016584044776,37.0112492462203));
#43234=CARTESIAN_POINT('Ctrl Pts',(21.6412751425566,10.7964506823689,37.0826495425283));
#43235=CARTESIAN_POINT('Ctrl Pts',(21.735116451846,10.7848847107764,37.2501004817808));
#43236=CARTESIAN_POINT('Ctrl Pts',(21.7795162811571,10.7785857480623,37.3474839734465));
#43237=CARTESIAN_POINT('Ctrl Pts',(21.842318392228,10.7673260318283,37.5223806723267));
#43238=CARTESIAN_POINT('Ctrl Pts',(21.8644182278704,10.7624580138213,37.5982793183434));
#43239=CARTESIAN_POINT('Ctrl Pts',(21.8860265091716,10.7562188817615,37.6940263644846));
#43240=CARTESIAN_POINT('Ctrl Pts',(21.8899702747218,10.7549911231532,37.7128012079479));
#43241=CARTESIAN_POINT('Ctrl Pts',(21.895276363828,10.7531998403472,37.7400776425713));
#43242=CARTESIAN_POINT('Ctrl Pts',(21.8968628948534,10.752643397293,37.7485348483117));
#43243=CARTESIAN_POINT('Ctrl Pts',(21.8995387383085,10.7516670229008,37.7633448645011));
#43244=CARTESIAN_POINT('Ctrl Pts',(21.9006528994606,10.7512478818498,37.7696930931895));
#43245=CARTESIAN_POINT('Ctrl Pts',(21.9027505178823,10.7504336029172,37.7820069516984));
#43246=CARTESIAN_POINT('Ctrl Pts',(21.9037377846146,10.7500385903706,37.7879718632807));
#43247=CARTESIAN_POINT('Ctrl Pts',(21.9060254920436,10.7490943651428,37.802208965139));
#43248=CARTESIAN_POINT('Ctrl Pts',(21.9073001355414,10.7485443483725,37.8104851195592));
#43249=CARTESIAN_POINT('Ctrl Pts',(21.9116824559747,10.746563685114,37.8402249272867));
#43250=CARTESIAN_POINT('Ctrl Pts',(21.9144819238026,10.7451234508024,37.8617316650655));
#43251=CARTESIAN_POINT('Ctrl Pts',(21.934182036087,10.7333863479548,38.0359821081059));
#43252=CARTESIAN_POINT('Ctrl Pts',(21.9331346016458,10.7225117963139,38.1901711489178));
#43253=CARTESIAN_POINT('Ctrl Pts',(21.9036523115755,10.7057808353691,38.4227819587822));
#43254=CARTESIAN_POINT('Ctrl Pts',(21.8884517802785,10.700017110856,38.5022832903641));
#43255=CARTESIAN_POINT('Ctrl Pts',(21.8594594085048,10.6919548988771,38.6149894535106));
#43256=CARTESIAN_POINT('Ctrl Pts',(21.8496646697655,10.6895281109054,38.6491306146134));
#43257=CARTESIAN_POINT('Ctrl Pts',(21.8366960718268,10.686654553144,38.6900380073314));
#43258=CARTESIAN_POINT('Ctrl Pts',(21.8344193107956,10.6861612109778,38.6970788113017));
#43259=CARTESIAN_POINT('Ctrl Pts',(21.8308068323658,10.6853956819611,38.7080345440337));
#43260=CARTESIAN_POINT('Ctrl Pts',(21.8294989711216,10.6851219253832,38.7119584786884));
#43261=CARTESIAN_POINT('Ctrl Pts',(21.8270418403205,10.6846139051402,38.7192522479804));
#43262=CARTESIAN_POINT('Ctrl Pts',(21.8258958730318,10.6843794605122,38.7226230754436));
#43263=CARTESIAN_POINT('Ctrl Pts',(21.8232663861635,10.6838471125545,38.7302879346178));
#43264=CARTESIAN_POINT('Ctrl Pts',(21.8217770285472,10.6835495553709,38.7345799041406));
#43265=CARTESIAN_POINT('Ctrl Pts',(21.8171745878246,10.6826419382544,38.7476932770316));
#43266=CARTESIAN_POINT('Ctrl Pts',(21.8140124347702,10.6820346770347,38.7564974933627));
#43267=CARTESIAN_POINT('Ctrl Pts',(21.7819261411692,10.6760286253035,38.8438314656172));
#43268=CARTESIAN_POINT('Ctrl Pts',(21.7479809352931,10.6709018280553,38.920434311437));
#43269=CARTESIAN_POINT('Ctrl Pts',(21.6591398182736,10.6593517219655,39.0901683797451));
#43270=CARTESIAN_POINT('Ctrl Pts',(21.6011902314298,10.6529946338975,39.1813734606499));
#43271=CARTESIAN_POINT('Ctrl Pts',(21.4879315141877,10.6416548915286,39.3304034939366));
#43272=CARTESIAN_POINT('Ctrl Pts',(21.4360990455532,10.6367675934128,39.3905232593883));
#43273=CARTESIAN_POINT('Ctrl Pts',(21.3672910884871,10.6305052786167,39.4610390428862));
#43274=CARTESIAN_POINT('Ctrl Pts',(21.3536593352624,10.6292748737447,39.4745975987791));
#43275=CARTESIAN_POINT('Ctrl Pts',(21.3336312942754,10.6274804263415,39.4939312393025));
#43276=CARTESIAN_POINT('Ctrl Pts',(21.3273950924013,10.626923500559,39.4998710632389));
#43277=CARTESIAN_POINT('Ctrl Pts',(21.3164218113412,10.6259465659343,39.510183579809));
#43278=CARTESIAN_POINT('Ctrl Pts',(21.3117021632281,10.6255273501476,39.5145746878275));
#43279=CARTESIAN_POINT('Ctrl Pts',(21.3025150880464,10.6247131370261,39.5230367289546));
#43280=CARTESIAN_POINT('Ctrl Pts',(21.2980503587384,10.6243182660167,39.527110490231));
#43281=CARTESIAN_POINT('Ctrl Pts',(21.2873603558262,10.6233747173829,39.5367727223787));
#43282=CARTESIAN_POINT('Ctrl Pts',(21.2811177709472,10.6228252383072,39.542341774604));
#43283=CARTESIAN_POINT('Ctrl Pts',(21.2586001023722,10.6208484670549,39.5621684220729));
#43284=CARTESIAN_POINT('Ctrl Pts',(21.2421221437597,10.6194116361054,39.5761921378147));
#43285=CARTESIAN_POINT('Ctrl Pts',(21.1061191223381,10.6076260924644,39.6880492000287));
#43286=CARTESIAN_POINT('Ctrl Pts',(20.9754966135637,10.596693051929,39.7714627285026));
#43287=CARTESIAN_POINT('Ctrl Pts',(20.764000144649,10.5799460084695,39.8732159715951));
#43288=CARTESIAN_POINT('Ctrl Pts',(20.68952872574,10.5742230431937,39.9034807689238));
#43289=CARTESIAN_POINT('Ctrl Pts',(20.5798504460772,10.5662098364682,39.9402627397112));
#43290=CARTESIAN_POINT('Ctrl Pts',(20.5460117454975,10.5637928563546,39.950585057184));
#43291=CARTESIAN_POINT('Ctrl Pts',(20.5047797483321,10.5609293100268,39.9619330251845));
#43292=CARTESIAN_POINT('Ctrl Pts',(20.4976423031163,10.5604365413324,39.9638533545048));
#43293=CARTESIAN_POINT('Ctrl Pts',(20.4864954816977,10.5596717060532,39.9667838104939));
#43294=CARTESIAN_POINT('Ctrl Pts',(20.4824936912305,10.559398074251,39.967822124174));
#43295=CARTESIAN_POINT('Ctrl Pts',(20.4750392484167,10.5588901649145,39.9697307150923));
#43296=CARTESIAN_POINT('Ctrl Pts',(20.4715875576079,10.5586557071603,39.9706042901486));
#43297=CARTESIAN_POINT('Ctrl Pts',(20.4637236426423,10.5581231747591,39.9725713878697));
#43298=CARTESIAN_POINT('Ctrl Pts',(20.4593099662564,10.557825447223,39.9736588737963));
#43299=CARTESIAN_POINT('Ctrl Pts',(20.4457887087296,10.5569167930227,39.976939727686));
#43300=CARTESIAN_POINT('Ctrl Pts',(20.4366687937879,10.5563086743926,39.9790824056728));
#43301=CARTESIAN_POINT('Ctrl Pts',(20.3438462010594,10.5501641201339,40.0001783192774));
#43302=CARTESIAN_POINT('Ctrl Pts',(20.258970984391,10.5449138835771,40.0135950256768));
#43303=CARTESIAN_POINT('Ctrl Pts',(20.0676178241381,10.5333405997367,40.0308721477843));
#43304=CARTESIAN_POINT('Ctrl Pts',(19.9611539510819,10.52707329972,40.0316652488695));
#43305=CARTESIAN_POINT('Ctrl Pts',(19.776559284865,10.5158558966257,40.01776715696));
#43306=CARTESIAN_POINT('Ctrl Pts',(19.6983975116754,10.5109970366068,40.007037072446));
#43307=CARTESIAN_POINT('Ctrl Pts',(19.6023260564581,10.5047689158753,39.9877937534686));
#43308=CARTESIAN_POINT('Ctrl Pts',(19.5835928585912,10.5035424160711,39.9837502147542));
#43309=CARTESIAN_POINT('Ctrl Pts',(19.5565439798984,10.5017526388361,39.9774885605211));
#43310=CARTESIAN_POINT('Ctrl Pts',(19.54817761001,10.5011964256424,39.9754927514179));
#43311=CARTESIAN_POINT('Ctrl Pts',(19.5335663065199,10.5002203179191,39.9719037637646));
#43312=CARTESIAN_POINT('Ctrl Pts',(19.5273154437585,10.4998012123587,39.9703351036174));
#43313=CARTESIAN_POINT('Ctrl Pts',(19.5152148392156,10.4989869016947,39.9672339093337));
#43314=CARTESIAN_POINT('Ctrl Pts',(19.5093642051856,10.4985918214537,39.9657051320434));
#43315=CARTESIAN_POINT('Ctrl Pts',(19.4954254823834,10.4976472728008,39.9619928296369));
#43316=CARTESIAN_POINT('Ctrl Pts',(19.4873442940395,10.4970969990382,39.959784090925));
#43317=CARTESIAN_POINT('Ctrl Pts',(19.4583721185383,10.495114469747,39.9516622776921));
#43318=CARTESIAN_POINT('Ctrl Pts',(19.4375675667545,10.4936726028176,39.945449442693));
#43319=CARTESIAN_POINT('Ctrl Pts',(19.2707565096495,10.48195952663,39.8925522115349));
#43320=CARTESIAN_POINT('Ctrl Pts',(19.1307107244844,10.4711139029523,39.8289758729134));
#43321=CARTESIAN_POINT('Ctrl Pts',(18.9303191309305,10.454390838242,39.7074537961304));
#43322=CARTESIAN_POINT('Ctrl Pts',(18.8636653430635,10.4486068602331,39.6610477497868));
#43323=CARTESIAN_POINT('Ctrl Pts',(18.7722694426735,10.4405203199771,39.5884508856477));
#43324=CARTESIAN_POINT('Ctrl Pts',(18.7450257115796,10.4380886791583,39.5655539196107));
#43325=CARTESIAN_POINT('Ctrl Pts',(18.7128950501272,10.4352101693812,39.5369962492712));
#43326=CARTESIAN_POINT('Ctrl Pts',(18.7073894189618,10.4347165445197,39.5320458311687));
#43327=CARTESIAN_POINT('Ctrl Pts',(18.6988519857178,10.4339506735404,39.5242799993921));
#43328=CARTESIAN_POINT('Ctrl Pts',(18.6958005822549,10.4336768554702,39.5214863880075));
#43329=CARTESIAN_POINT('Ctrl Pts',(18.6901399592686,10.4331687805018,39.5162704211527));
#43330=CARTESIAN_POINT('Ctrl Pts',(18.6875284832723,10.4329343422743,39.5138506817323));
#43331=CARTESIAN_POINT('Ctrl Pts',(18.6816007977919,10.4324020849043,39.5083276349199));
#43332=CARTESIAN_POINT('Ctrl Pts',(18.6782888441936,10.4321046114337,39.5052198423452));
#43333=CARTESIAN_POINT('Ctrl Pts',(18.6697058281325,10.4313333749276,39.4971087249236));
#43334=CARTESIAN_POINT('Ctrl Pts',(18.6644519490188,10.4308609595768,39.4920872029184));
#43335=CARTESIAN_POINT('Ctrl Pts',(18.6306125887695,10.4278151097054,39.4593765033164));
#43336=CARTESIAN_POINT('Ctrl Pts',(18.6028590413918,10.4253025551288,39.4308358381864));
#43337=CARTESIAN_POINT('Ctrl Pts',(18.5643734789911,10.4217608851881,39.388726647215));
#43338=CARTESIAN_POINT('Ctrl Pts',(18.5529116337261,10.4206983190511,39.3758429250722));
#43339=CARTESIAN_POINT('Ctrl Pts',(18.4467379163231,10.4107624873512,39.2532262218638));
#43340=CARTESIAN_POINT('Ctrl Pts',(18.3645018310395,10.4023221614154,39.133297604032));
#43341=CARTESIAN_POINT('Ctrl Pts',(18.26250708063,10.3891048820596,38.9413677905178));
#43342=CARTESIAN_POINT('Ctrl Pts',(18.2321687264354,10.3846274852405,38.8755979885223));
#43343=CARTESIAN_POINT('Ctrl Pts',(18.1988738264377,10.3788578502581,38.7912471012287));
#43344=CARTESIAN_POINT('Ctrl Pts',(18.1923920902067,10.3776848655194,38.7741154617217));
#43345=CARTESIAN_POINT('Ctrl Pts',(18.1832795541511,10.3759592146978,38.7489535494239));
#43346=CARTESIAN_POINT('Ctrl Pts',(18.1804558798099,10.3754129125147,38.740993821054));
#43347=CARTESIAN_POINT('Ctrl Pts',(18.1755776566043,10.3744482396269,38.7269504753432));
#43348=CARTESIAN_POINT('Ctrl Pts',(18.1735010295625,10.3740306013608,38.7208746209553));
#43349=CARTESIAN_POINT('Ctrl Pts',(18.1695128566551,10.37321466642,38.7090127309221));
#43350=CARTESIAN_POINT('Ctrl Pts',(18.1675983146325,10.3728164736428,38.7032277765565));
#43351=CARTESIAN_POINT('Ctrl Pts',(18.1625292646284,10.3717444361701,38.6876643787747));
#43352=CARTESIAN_POINT('Ctrl Pts',(18.1594254516339,10.3710689481996,38.6778697521407));
#43353=CARTESIAN_POINT('Ctrl Pts',(18.1486411494774,10.3686519625019,38.6428694790411));
#43354=CARTESIAN_POINT('Ctrl Pts',(18.141399301703,10.3668963917609,38.6175327940379));
#43355=CARTESIAN_POINT('Ctrl Pts',(18.0921783046155,10.3539181838387,38.4309426067896));
#43356=CARTESIAN_POINT('Ctrl Pts',(18.0707382190134,10.3420192508737,38.2650273210922));
#43357=CARTESIAN_POINT('Ctrl Pts',(18.0709448114571,10.3235080837719,38.0051127617899));
#43358=CARTESIAN_POINT('Ctrl Pts',(18.0777953065008,10.3169155061858,37.9118750950458));
#43359=CARTESIAN_POINT('Ctrl Pts',(18.0927357498699,10.3100094244671,37.8102182461063));
#43360=CARTESIAN_POINT('Ctrl Pts',(18.0941660375926,10.3093828526717,37.8009560213759));
#43361=CARTESIAN_POINT('Ctrl Pts',(18.0963903565276,10.3084577137425,37.7872164463417));
#43362=CARTESIAN_POINT('Ctrl Pts',(18.0971327831626,10.3081563799409,37.7827310568363));
#43363=CARTESIAN_POINT('Ctrl Pts',(18.0984849245516,10.3076206398733,37.7747375636249));
#43364=CARTESIAN_POINT('Ctrl Pts',(18.0990884999661,10.3073858954797,37.7712284920566));
#43365=CARTESIAN_POINT('Ctrl Pts',(18.1004138069717,10.3068798204288,37.7636490823752));
#43366=CARTESIAN_POINT('Ctrl Pts',(18.1011389051305,10.3066086816481,37.7595793958716));
#43367=CARTESIAN_POINT('Ctrl Pts',(18.1031964946426,10.3058549211039,37.7482421125009));
#43368=CARTESIAN_POINT('Ctrl Pts',(18.1045576832612,10.305373884352,37.7409796975521));
#43369=CARTESIAN_POINT('Ctrl Pts',(18.1126684131882,10.3026053508087,37.6990384020968));
#43370=CARTESIAN_POINT('Ctrl Pts',(18.1203283513335,10.3003657286172,37.6645397877283));
#43371=CARTESIAN_POINT('Ctrl Pts',(18.1484474338735,10.2931603108146,37.5525338619101));
#43372=CARTESIAN_POINT('Ctrl Pts',(18.1727897677542,10.2883446256777,37.4760841470524));
#43373=CARTESIAN_POINT('Ctrl Pts',(18.257830253717,10.2743017478785,37.2572028192219));
#43374=CARTESIAN_POINT('Ctrl Pts',(18.3309650593214,10.2651390650128,37.1203170754948));
#43375=CARTESIAN_POINT('Ctrl Pts',(18.43205268078,10.253968439844,36.97592202711));
#43376=CARTESIAN_POINT('Ctrl Pts',(18.4447497331722,10.2525876669069,36.9584192394934));
#43377=CARTESIAN_POINT('Ctrl Pts',(18.4627619310325,10.2506572404359,36.9344479325156));
#43378=CARTESIAN_POINT('Ctrl Pts',(18.4678293250616,10.2501171452686,36.9277945905451));
#43379=CARTESIAN_POINT('Ctrl Pts',(18.4766326546844,10.2491838669968,36.9163906850465));
#43380=CARTESIAN_POINT('Ctrl Pts',(18.4803479753078,10.2487914937509,36.9116243011196));
#43381=CARTESIAN_POINT('Ctrl Pts',(18.4880728240719,10.247978719375,36.9018095588278));
#43382=CARTESIAN_POINT('Ctrl Pts',(18.4920853801294,10.2475582016561,36.896763690658));
#43383=CARTESIAN_POINT('Ctrl Pts',(18.5015185889721,10.2465734069415,36.8850225403936));
#43384=CARTESIAN_POINT('Ctrl Pts',(18.5069589115971,10.246008349327,36.8783433089318));
#43385=CARTESIAN_POINT('Ctrl Pts',(18.5246928589845,10.2441755309676,36.8568662571319));
#43386=CARTESIAN_POINT('Ctrl Pts',(18.5371628319802,10.2429006789327,36.842216219887));
#43387=CARTESIAN_POINT('Ctrl Pts',(18.6022186624103,10.2363177866212,36.7680632145053));
#43388=CARTESIAN_POINT('Ctrl Pts',(18.6582166143751,10.230868919598,36.7116690968204));
#43389=CARTESIAN_POINT('Ctrl Pts',(18.7983020392575,10.2177354878623,36.5870037778571));
#43390=CARTESIAN_POINT('Ctrl Pts',(18.8849791180935,10.2099717234808,36.5220388635909));
#43391=CARTESIAN_POINT('Ctrl Pts',(19.0472648203096,10.1963669467373,36.4204820220479));
#43392=CARTESIAN_POINT('Ctrl Pts',(19.1206945061303,10.1905116870977,36.3808984207502));
#43393=CARTESIAN_POINT('Ctrl Pts',(19.2049641320491,10.1842816895442,36.3422889943194));
#43394=CARTESIAN_POINT('Ctrl Pts',(19.2134943794653,10.1836564690104,36.3384555275738));
#43395=CARTESIAN_POINT('Ctrl Pts',(19.2262090591111,10.1827329323205,36.3328523632226));
#43396=CARTESIAN_POINT('Ctrl Pts',(19.2303722533585,10.1824318631306,36.3310352397469));
#43397=CARTESIAN_POINT('Ctrl Pts',(19.2378098716662,10.1818964103936,36.3278201444038));
#43398=CARTESIAN_POINT('Ctrl Pts',(19.2410817758008,10.181661690187,36.326416519583));
#43399=CARTESIAN_POINT('Ctrl Pts',(19.2481635832264,10.1811554596123,36.323401657706));
#43400=CARTESIAN_POINT('Ctrl Pts',(19.2519747800507,10.1808841422239,36.321793617562));
#43401=CARTESIAN_POINT('Ctrl Pts',(19.2626196094516,10.1801293799193,36.3173425745007));
#43402=CARTESIAN_POINT('Ctrl Pts',(19.269464565122,10.179647526862,36.3145265838545));
#43403=CARTESIAN_POINT('Ctrl Pts',(19.309269008668,10.1768646867237,36.2984184037044));
#43404=CARTESIAN_POINT('Ctrl Pts',(19.3425769949156,10.1746121548265,36.2859986408772));
#43405=CARTESIAN_POINT('Ctrl Pts',(19.3821662717714,10.172002320136,36.2724706186907));
#43406=CARTESIAN_POINT('Ctrl Pts',(19.388130481316,10.1716109234842,36.270465130908));
#43407=CARTESIAN_POINT('Ctrl Pts',(19.394104010895,10.1712205940279,36.2684889824829));
#43408=CARTESIAN_POINT('',(18.0708706529646,10.1603463946639,38.1015872324743));
#43409=CARTESIAN_POINT('Ctrl Pts',(19.3941040084883,9.99997597504683,36.2684889832791));
#43410=CARTESIAN_POINT('Ctrl Pts',(19.3745689141501,10.001353917181,36.2749515353715));
#43411=CARTESIAN_POINT('Ctrl Pts',(19.3551388044924,10.002741792661,36.2817261061457));
#43412=CARTESIAN_POINT('Ctrl Pts',(19.2733594970616,10.0086578068466,36.3117152820464));
#43413=CARTESIAN_POINT('Ctrl Pts',(19.2121307374123,10.0132746362667,36.3378339722369));
#43414=CARTESIAN_POINT('Ctrl Pts',(19.0358651373947,10.02709199074,36.4240496327043));
#43415=CARTESIAN_POINT('Ctrl Pts',(18.925402230502,10.0364680887741,36.4926407959781));
#43416=CARTESIAN_POINT('Ctrl Pts',(18.7827972608735,10.0490802422282,36.6025047087582));
#43417=CARTESIAN_POINT('Ctrl Pts',(18.7441478628999,10.052553720299,36.6347658671016));
#43418=CARTESIAN_POINT('Ctrl Pts',(18.7010434390228,10.0564526726847,36.6737059866913));
#43419=CARTESIAN_POINT('Ctrl Pts',(18.6953172141169,10.0569711560191,36.6789420867246));
#43420=CARTESIAN_POINT('Ctrl Pts',(18.6862182997434,10.0577956435505,36.6873635576435));
#43421=CARTESIAN_POINT('Ctrl Pts',(18.682825310752,10.0581032353062,36.6905267248648));
#43422=CARTESIAN_POINT('Ctrl Pts',(18.6768347457816,10.0586465064283,36.6961520467943));
#43423=CARTESIAN_POINT('Ctrl Pts',(18.6742325725197,10.058882555847,36.6986092283909));
#43424=CARTESIAN_POINT('Ctrl Pts',(18.6692154588179,10.0593377807267,36.7033732729611));
#43425=CARTESIAN_POINT('Ctrl Pts',(18.6667996806436,10.0595570289135,36.705679155066));
#43426=CARTESIAN_POINT('Ctrl Pts',(18.6600336273952,10.0601712880575,36.7121710752141));
#43427=CARTESIAN_POINT('Ctrl Pts',(18.6556969484201,10.0605652218622,36.7163713243501));
#43428=CARTESIAN_POINT('Ctrl Pts',(18.6377605635102,10.0621958357057,36.733907373454));
#43429=CARTESIAN_POINT('Ctrl Pts',(18.6243384616431,10.0634192160852,36.7474244032099));
#43430=CARTESIAN_POINT('Ctrl Pts',(18.589107196651,10.0666464094525,36.7839719241485));
#43431=CARTESIAN_POINT('Ctrl Pts',(18.5676613484233,10.0686277545001,36.8073459006618));
#43432=CARTESIAN_POINT('Ctrl Pts',(18.4922024140083,10.0757077884832,36.8937742541364));
#43433=CARTESIAN_POINT('Ctrl Pts',(18.4416941936894,10.0806607968453,36.9597724143537));
#43434=CARTESIAN_POINT('Ctrl Pts',(18.3191210866453,10.0938444526007,37.1433622856972));
#43435=CARTESIAN_POINT('Ctrl Pts',(18.2551440376971,10.1020733732418,37.2657450940994));
#43436=CARTESIAN_POINT('Ctrl Pts',(18.1965625550607,10.1122089605306,37.4146859204018));
#43437=CARTESIAN_POINT('Ctrl Pts',(18.1887447801219,10.1136353861665,37.4356232483476));
#43438=CARTESIAN_POINT('Ctrl Pts',(18.1781527163282,10.1156798811251,37.4655682096555));
#43439=CARTESIAN_POINT('Ctrl Pts',(18.1750777719302,10.1162880674129,37.4744681639007));
#43440=CARTESIAN_POINT('Ctrl Pts',(18.1701717254134,10.1172829679357,37.4890120746376));
#43441=CARTESIAN_POINT('Ctrl Pts',(18.1683012636492,10.1176683880984,37.4946426696896));
#43442=CARTESIAN_POINT('Ctrl Pts',(18.1644269700283,10.118479760742,37.5064877063497));
#43443=CARTESIAN_POINT('Ctrl Pts',(18.1624286585595,10.1189058875832,37.5127038613825));
#43444=CARTESIAN_POINT('Ctrl Pts',(18.1577241146364,10.1199277019056,37.5275973977282));
#43445=CARTESIAN_POINT('Ctrl Pts',(18.1550475978892,10.1205243465015,37.5362839313478));
#43446=CARTESIAN_POINT('Ctrl Pts',(18.1461042189783,10.1225717540805,37.566055401157));
#43447=CARTESIAN_POINT('Ctrl Pts',(18.1401368339267,10.1240321261214,37.5872277919941));
#43448=CARTESIAN_POINT('Ctrl Pts',(18.0921219256862,10.1366439167986,37.7694651422497));
#43449=CARTESIAN_POINT('Ctrl Pts',(18.0707337620348,10.1484844051065,37.9352093928769));
#43450=CARTESIAN_POINT('Ctrl Pts',(18.0708706529646,10.1603463946639,38.1015872324743));
#43451=CARTESIAN_POINT('Ctrl Pts',(18.0708706542009,10.1603465017403,38.1015887343413));
#43452=CARTESIAN_POINT('Ctrl Pts',(18.0709352769545,10.1659409537865,38.1800572656555));
#43453=CARTESIAN_POINT('Ctrl Pts',(18.0757874956902,10.1715085483743,38.258457138053));
#43454=CARTESIAN_POINT('Ctrl Pts',(18.0882688932751,10.1785084047994,38.3595647016621));
#43455=CARTESIAN_POINT('Ctrl Pts',(18.0915567020537,10.1800992157944,38.3827259361767));
#43456=CARTESIAN_POINT('Ctrl Pts',(18.0962288215372,10.1820772059349,38.411824968796));
#43457=CARTESIAN_POINT('Ctrl Pts',(18.0972208989003,10.182483780379,38.4178226012995));
#43458=CARTESIAN_POINT('Ctrl Pts',(18.0989271214245,10.1831610969617,38.4278431935512));
#43459=CARTESIAN_POINT('Ctrl Pts',(18.0996257176339,10.1834326583439,38.4318687042855));
#43460=CARTESIAN_POINT('Ctrl Pts',(18.1009219784398,10.1839262066194,38.4391998061884));
#43461=CARTESIAN_POINT('Ctrl Pts',(18.1015154959506,10.1841484203157,38.4425061003895));
#43462=CARTESIAN_POINT('Ctrl Pts',(18.1027559310396,10.1846051704734,38.4493138676983));
#43463=CARTESIAN_POINT('Ctrl Pts',(18.1034038984834,10.1848396354185,38.4528150555175));
#43464=CARTESIAN_POINT('Ctrl Pts',(18.1049014424658,10.1853722758184,38.4607834402523));
#43465=CARTESIAN_POINT('Ctrl Pts',(18.1057571206569,10.1856701035918,38.4652494334454));
#43466=CARTESIAN_POINT('Ctrl Pts',(18.1084254388448,10.1865793708479,38.4789144258778));
#43467=CARTESIAN_POINT('Ctrl Pts',(18.1102893895482,10.1871879967715,38.4881034396852));
#43468=CARTESIAN_POINT('Ctrl Pts',(18.1309504516299,10.1936640881798,38.5862801888146));
#43469=CARTESIAN_POINT('Ctrl Pts',(18.1559541064356,10.1992096620934,38.6738589164581));
#43470=CARTESIAN_POINT('Ctrl Pts',(18.2111499087872,10.2089186431627,38.8256239490101));
#43471=CARTESIAN_POINT('Ctrl Pts',(18.238866142833,10.2131048154481,38.8905203916707));
#43472=CARTESIAN_POINT('Ctrl Pts',(18.3079943050377,10.2224704338658,39.0305919247723));
#43473=CARTESIAN_POINT('Ctrl Pts',(18.350988892506,10.2276614763969,39.104810871593));
#43474=CARTESIAN_POINT('Ctrl Pts',(18.4194779264765,10.2353391129195,39.2067388905108));
#43475=CARTESIAN_POINT('Ctrl Pts',(18.4410688657087,10.2376888348495,39.2369496149498));
#43476=CARTESIAN_POINT('Ctrl Pts',(18.4702666225165,10.2407882426062,39.275407567422));
#43477=CARTESIAN_POINT('Ctrl Pts',(18.4770932736009,10.2415076630798,39.2842391016652));
#43478=CARTESIAN_POINT('Ctrl Pts',(18.4883028606127,10.2426808143607,39.2984835483605));
#43479=CARTESIAN_POINT('Ctrl Pts',(18.4926392082281,10.2431327042832,39.3039329292968));
#43480=CARTESIAN_POINT('Ctrl Pts',(18.5010257501155,10.2440030377826,39.3143557523066));
#43481=CARTESIAN_POINT('Ctrl Pts',(18.5050714342431,10.2444212978212,39.3193327177598));
#43482=CARTESIAN_POINT('Ctrl Pts',(18.5143814029875,10.2453802416169,39.3306697786118));
#43483=CARTESIAN_POINT('Ctrl Pts',(18.5196618191517,10.2459215706908,39.3370164051179));
#43484=CARTESIAN_POINT('Ctrl Pts',(18.5337857151164,10.2473628698212,39.3537722216733));
#43485=CARTESIAN_POINT('Ctrl Pts',(18.5426991516193,10.2482656749261,39.3641215661921));
#43486=CARTESIAN_POINT('Ctrl Pts',(18.6167985122066,10.2557172217791,39.4483326449094));
#43487=CARTESIAN_POINT('Ctrl Pts',(18.6874341208788,10.2624960425208,39.5171847300134));
#43488=CARTESIAN_POINT('Ctrl Pts',(18.8890225344465,10.2809959120808,39.6856354477209));
#43489=CARTESIAN_POINT('Ctrl Pts',(19.0279625851161,10.2929654556903,39.7744114923335));
#43490=CARTESIAN_POINT('Ctrl Pts',(19.1946612522752,10.305544866414,39.8531049257387));
#43491=CARTESIAN_POINT('Ctrl Pts',(19.2129901504729,10.3069046905234,39.8614093661923));
#43492=CARTESIAN_POINT('Ctrl Pts',(19.2369631539404,10.3086501048059,39.871822085772));
#43493=CARTESIAN_POINT('Ctrl Pts',(19.2424910805725,10.3090503143815,39.8741924843253));
#43494=CARTESIAN_POINT('Ctrl Pts',(19.2511160682032,10.3096711232071,39.8778432560461));
#43495=CARTESIAN_POINT('Ctrl Pts',(19.2542054710583,10.3098927716642,39.8791414523299));
#43496=CARTESIAN_POINT('Ctrl Pts',(19.2605897641369,10.3103493023631,39.8818046411333));
#43497=CARTESIAN_POINT('Ctrl Pts',(19.2638850113652,10.3105841085867,39.8831685281676));
#43498=CARTESIAN_POINT('Ctrl Pts',(19.2714468117089,10.3111210501096,39.8862737874096));
#43499=CARTESIAN_POINT('Ctrl Pts',(19.2757158306866,10.3114228154582,39.8880090142179));
#43500=CARTESIAN_POINT('Ctrl Pts',(19.2869382103075,10.3122126197885,39.8925237835756));
#43501=CARTESIAN_POINT('Ctrl Pts',(19.2939016905105,10.3126992022664,39.8952781991548));
#43502=CARTESIAN_POINT('Ctrl Pts',(19.3418611951529,10.3160276689795,39.9139264422164));
#43503=CARTESIAN_POINT('Ctrl Pts',(19.3833777536853,10.3187950940226,39.928456595436));
#43504=CARTESIAN_POINT('Ctrl Pts',(19.4486576654791,10.3230243920946,39.9488266307077));
#43505=CARTESIAN_POINT('Ctrl Pts',(19.4720937640836,10.3245188065941,39.9556544297385));
#43506=CARTESIAN_POINT('Ctrl Pts',(19.5566027997894,10.3298422263702,39.9785443261797));
#43507=CARTESIAN_POINT('Ctrl Pts',(19.6183277357985,10.333610152752,39.992050926724));
#43508=CARTESIAN_POINT('Ctrl Pts',(19.8199092623973,10.3458174644644,40.0258925883052));
#43509=CARTESIAN_POINT('Ctrl Pts',(19.9613398283213,10.354267903439,40.0339062768754));
#43510=CARTESIAN_POINT('Ctrl Pts',(20.1214528235252,10.3644604941376,40.0253978729783));
#43511=CARTESIAN_POINT('Ctrl Pts',(20.1405194323251,10.3656835920694,40.0241003105589));
#43512=CARTESIAN_POINT('Ctrl Pts',(20.1681250332468,10.3674692989962,40.0218091325499));
#43513=CARTESIAN_POINT('Ctrl Pts',(20.1766820185255,10.3680248893364,40.0210413397855));
#43514=CARTESIAN_POINT('Ctrl Pts',(20.1916468570121,10.3690002738514,40.019597758199));
#43515=CARTESIAN_POINT('Ctrl Pts',(20.1980570312033,10.3694192826215,40.0189469721179));
#43516=CARTESIAN_POINT('Ctrl Pts',(20.2104795092473,10.3702336780429,40.0176228861435));
#43517=CARTESIAN_POINT('Ctrl Pts',(20.2164921498367,10.3706289411123,40.0169533914352));
#43518=CARTESIAN_POINT('Ctrl Pts',(20.2308335874043,10.3715743653407,40.0152881693736));
#43519=CARTESIAN_POINT('Ctrl Pts',(20.2391591782037,10.3721253352737,40.0142663870391));
#43520=CARTESIAN_POINT('Ctrl Pts',(20.2690754749539,10.3741129451991,40.0103966114978));
#43521=CARTESIAN_POINT('Ctrl Pts',(20.2906235779385,10.3755592610023,40.0072374510516));
#43522=CARTESIAN_POINT('Ctrl Pts',(20.4622960855105,10.3872039789299,39.9790918425619));
#43523=CARTESIAN_POINT('Ctrl Pts',(20.6090099300316,10.3979675922106,39.936788775574));
#43524=CARTESIAN_POINT('Ctrl Pts',(20.8246847233666,10.4146684795706,39.8458945662411));
#43525=CARTESIAN_POINT('Ctrl Pts',(20.8980724662136,10.4205102164572,39.8093040253629));
#43526=CARTESIAN_POINT('Ctrl Pts',(20.9998505664068,10.4286660521415,39.750188244022));
#43527=CARTESIAN_POINT('Ctrl Pts',(21.0302824692156,10.4311114556584,39.7313616493725));
#43528=CARTESIAN_POINT('Ctrl Pts',(21.0663707241151,10.4340040028155,39.7076227873082));
#43529=CARTESIAN_POINT('Ctrl Pts',(21.0725426584164,10.4344984246822,39.703511708031));
#43530=CARTESIAN_POINT('Ctrl Pts',(21.0821228150311,10.4352652592268,39.6970503768493));
#43531=CARTESIAN_POINT('Ctrl Pts',(21.0855473555649,10.4355392501401,39.6947246259562));
#43532=CARTESIAN_POINT('Ctrl Pts',(21.0919029331634,10.4360474784253,39.6903783243166));
#43533=CARTESIAN_POINT('Ctrl Pts',(21.0948358362845,10.4362818981583,39.6883607026794));
#43534=CARTESIAN_POINT('Ctrl Pts',(21.101494845346,10.4368138993051,39.6837525867704));
#43535=CARTESIAN_POINT('Ctrl Pts',(21.1052174003785,10.4371111363833,39.6811570603093));
#43536=CARTESIAN_POINT('Ctrl Pts',(21.116564805273,10.4380168090292,39.6731855043083));
#43537=CARTESIAN_POINT('Ctrl Pts',(21.1241599842667,10.4386224633106,39.6677671809273));
#43538=CARTESIAN_POINT('Ctrl Pts',(21.1970705839275,10.4444344089309,39.6149512053395));
#43539=CARTESIAN_POINT('Ctrl Pts',(21.2593993963351,10.4493879628641,39.5635476591145));
#43540=CARTESIAN_POINT('Ctrl Pts',(21.4381357006637,10.4641674328672,39.3962397964793));
#43541=CARTESIAN_POINT('Ctrl Pts',(21.543134905801,10.4737374464768,39.269275794489));
#43542=CARTESIAN_POINT('Ctrl Pts',(21.6518517561269,10.4864392719816,39.0972369782981));
#43543=CARTESIAN_POINT('Ctrl Pts',(21.6718783960239,10.4889307615572,39.0632850573302));
#43544=CARTESIAN_POINT('Ctrl Pts',(21.696296696039,10.4921857042504,39.0188297237604));
#43545=CARTESIAN_POINT('Ctrl Pts',(21.7016557432144,10.4929147139332,39.0088664725818));
#43546=CARTESIAN_POINT('Ctrl Pts',(21.7101871469799,10.4940996386523,38.9926653592908));
#43547=CARTESIAN_POINT('Ctrl Pts',(21.7134137897006,10.4945536424513,38.9864562620348));
#43548=CARTESIAN_POINT('Ctrl Pts',(21.7195285857133,10.4954254216499,38.9745313093857));
#43549=CARTESIAN_POINT('Ctrl Pts',(21.722422202895,10.4958429992367,38.9688183478161));
#43550=CARTESIAN_POINT('Ctrl Pts',(21.7289503409683,10.4967967200319,38.955768841088));
#43551=CARTESIAN_POINT('Ctrl Pts',(21.7325666898277,10.4973334844451,38.9484233923756));
#43552=CARTESIAN_POINT('Ctrl Pts',(21.7419892288439,10.4987547225221,38.9289730523874));
#43553=CARTESIAN_POINT('Ctrl Pts',(21.7477159212063,10.4996419070503,38.9168303608091));
#43554=CARTESIAN_POINT('Ctrl Pts',(21.7899933635443,10.506373343065,38.8247063222588));
#43555=CARTESIAN_POINT('Ctrl Pts',(21.8211584396975,10.5123991818598,38.742381064723));
#43556=CARTESIAN_POINT('Ctrl Pts',(21.857138561599,10.5211145771021,38.6233600890604));
#43557=CARTESIAN_POINT('Ctrl Pts',(21.8666890615977,10.523688419848,38.5882020001733));
#43558=CARTESIAN_POINT('Ctrl Pts',(21.8949450428071,10.5322368138504,38.4711808205938));
#43559=CARTESIAN_POINT('Ctrl Pts',(21.9093025709464,10.5382611489536,38.3883670934481));
#43560=CARTESIAN_POINT('Ctrl Pts',(21.9250212246722,10.5487312788639,38.2412000422267));
#43561=CARTESIAN_POINT('Ctrl Pts',(21.9286482703333,10.5532048026547,38.1772122271859));
#43562=CARTESIAN_POINT('Ctrl Pts',(21.9291731189973,10.5584067857043,38.1002560000262));
#43563=CARTESIAN_POINT('Ctrl Pts',(21.9291316961775,10.5592728299215,38.0873544691316));
#43564=CARTESIAN_POINT('Ctrl Pts',(21.9288923212058,10.5604767802341,38.069279497368));
#43565=CARTESIAN_POINT('Ctrl Pts',(21.9288029730921,10.5608203494869,38.0641053121799));
#43566=CARTESIAN_POINT('Ctrl Pts',(21.9286150419257,10.5614044792397,38.0552795388353));
#43567=CARTESIAN_POINT('Ctrl Pts',(21.9285269063632,10.5616456118431,38.0516277778662));
#43568=CARTESIAN_POINT('Ctrl Pts',(21.9283375052746,10.5621081078961,38.044607017854));
#43569=CARTESIAN_POINT('Ctrl Pts',(21.9282377828284,10.5623295586608,38.0412380222649));
#43570=CARTESIAN_POINT('Ctrl Pts',(21.9279482679635,10.5629188882786,38.0322533845217));
#43571=CARTESIAN_POINT('Ctrl Pts',(21.9277427681328,10.5632859024816,38.0266382272589));
#43572=CARTESIAN_POINT('Ctrl Pts',(21.9269122234895,10.5646063711641,38.0063677069782));
#43573=CARTESIAN_POINT('Ctrl Pts',(21.9261445469413,10.565552290228,37.9917182427414));
#43574=CARTESIAN_POINT('Ctrl Pts',(21.9177483415487,10.5739795171772,37.8602160388294));
#43575=CARTESIAN_POINT('Ctrl Pts',(21.899660666174,10.5809660497249,37.7442581646185));
#43576=CARTESIAN_POINT('Ctrl Pts',(21.8341767007462,10.5970418487259,37.4831959467704));
#43577=CARTESIAN_POINT('Ctrl Pts',(21.7798999241105,10.6061154329658,37.3406583943935));
#43578=CARTESIAN_POINT('Ctrl Pts',(21.7023705840695,10.6167956764077,37.1924146604005));
#43579=CARTESIAN_POINT('Ctrl Pts',(21.6951174756711,10.6177780720611,37.1789389400326));
#43580=CARTESIAN_POINT('Ctrl Pts',(21.6838992128174,10.6192733693845,37.1586776706207));
#43581=CARTESIAN_POINT('Ctrl Pts',(21.6800515434783,10.6197821118376,37.1518274972547));
#43582=CARTESIAN_POINT('Ctrl Pts',(21.6730167971142,10.6207049771654,37.1394804926256));
#43583=CARTESIAN_POINT('Ctrl Pts',(21.6698441889629,10.6211185785751,37.1339755124999));
#43584=CARTESIAN_POINT('Ctrl Pts',(21.6629808945733,10.6220078390341,37.1222014403659));
#43585=CARTESIAN_POINT('Ctrl Pts',(21.6592818360192,10.6224837949027,37.1159373672581));
#43586=CARTESIAN_POINT('Ctrl Pts',(21.6492587401756,10.6237647179186,37.0991812147398));
#43587=CARTESIAN_POINT('Ctrl Pts',(21.6428701285082,10.6245720152212,37.0887283440504));
#43588=CARTESIAN_POINT('Ctrl Pts',(21.6122953015223,10.6283937742077,37.0397570848757));
#43589=CARTESIAN_POINT('Ctrl Pts',(21.5868531354346,10.6314539741804,37.0020438452081));
#43590=CARTESIAN_POINT('Ctrl Pts',(21.4427924566792,10.6481838413501,36.8039799040044));
#43591=CARTESIAN_POINT('Ctrl Pts',(21.3012133724693,10.6627652521498,36.6618985636947));
#43592=CARTESIAN_POINT('Ctrl Pts',(21.1080101421072,10.6794219046218,36.5202944995813));
#43593=CARTESIAN_POINT('Ctrl Pts',(21.0748764638824,10.6821753743147,36.4975652643608));
#43594=CARTESIAN_POINT('Ctrl Pts',(21.034605438134,10.6853801058381,36.4717516087254));
#43595=CARTESIAN_POINT('Ctrl Pts',(21.0281316559267,10.6858910343871,36.4676561210282));
#43596=CARTESIAN_POINT('Ctrl Pts',(21.0180770680163,10.6866778124796,36.4613788666111));
#43597=CARTESIAN_POINT('Ctrl Pts',(21.0145133467516,10.686955372716,36.459170086419));
#43598=CARTESIAN_POINT('Ctrl Pts',(21.0079147765544,10.687466857538,36.4551100349873));
#43599=CARTESIAN_POINT('Ctrl Pts',(21.0048820339142,10.6877009855418,36.4532555474239));
#43600=CARTESIAN_POINT('Ctrl Pts',(20.9980266130018,10.6882280905272,36.449089526444));
#43601=CARTESIAN_POINT('Ctrl Pts',(20.994201030031,10.6885207491733,36.4467828863591));
#43602=CARTESIAN_POINT('Ctrl Pts',(20.9829106389744,10.6893802077857,36.4400286944265));
#43603=CARTESIAN_POINT('Ctrl Pts',(20.9754236323362,10.6899446790255,36.4356181916699));
#43604=CARTESIAN_POINT('Ctrl Pts',(20.9202627753361,10.6940654617186,36.4036236801353));
#43605=CARTESIAN_POINT('Ctrl Pts',(20.8714518598468,10.6975049623196,36.3780391638108));
#43606=CARTESIAN_POINT('Ctrl Pts',(20.708105074409,10.7085702856281,36.3011483558419));
#43607=CARTESIAN_POINT('Ctrl Pts',(20.5896565834821,10.715921898939,36.2589164613412));
#43608=CARTESIAN_POINT('Ctrl Pts',(20.3811804371502,10.7288782260234,36.2067905676883));
#43609=CARTESIAN_POINT('Ctrl Pts',(20.2930268834515,10.7343582265289,36.1911593004242));
#43610=CARTESIAN_POINT('Ctrl Pts',(20.1837518312159,10.7413339392909,36.1795320540584));
#43611=CARTESIAN_POINT('Ctrl Pts',(20.1633571586141,10.7426432289965,36.1776898651474));
#43612=CARTESIAN_POINT('Ctrl Pts',(20.1341286410681,10.7445317543835,36.1755182278936));
#43613=CARTESIAN_POINT('Ctrl Pts',(20.1253153848545,10.745102771396,36.1749242525069));
#43614=CARTESIAN_POINT('Ctrl Pts',(20.110026972918,10.7460961705874,36.1739993105376));
#43615=CARTESIAN_POINT('Ctrl Pts',(20.1035536010687,10.746517678233,36.1736404176326));
#43616=CARTESIAN_POINT('Ctrl Pts',(20.0910986259198,10.7473304263732,36.1730128572742));
#43617=CARTESIAN_POINT('Ctrl Pts',(20.0851173305992,10.7477215126921,36.1727393931927));
#43618=CARTESIAN_POINT('Ctrl Pts',(20.0709952597496,10.7486467621112,36.1721596031678));
#43619=CARTESIAN_POINT('Ctrl Pts',(20.0628536765095,10.7491816559649,36.17187699187));
#43620=CARTESIAN_POINT('Ctrl Pts',(20.034396681097,10.7510565473495,36.1710696189872));
#43621=CARTESIAN_POINT('Ctrl Pts',(20.0140755594527,10.7524048520605,36.170814324209));
#43622=CARTESIAN_POINT('Ctrl Pts',(19.8244742170813,10.7650773821779,36.171428123064));
#43623=CARTESIAN_POINT('Ctrl Pts',(19.6560335694318,10.7771214248263,36.1942555700715));
#43624=CARTESIAN_POINT('Ctrl Pts',(19.4596217751291,10.7916335279829,36.2477811096073));
#43625=CARTESIAN_POINT('Ctrl Pts',(19.4267191744352,10.7940772742089,36.2576993133833));
#43626=CARTESIAN_POINT('Ctrl Pts',(19.3941039816494,10.7965035432258,36.2684889921579));
#43627=CARTESIAN_POINT('Origin',(20.,-1.3495818343519,38.1));
#43628=CARTESIAN_POINT('',(19.394104009052,11.7619801941422,36.2684889830926));
#43629=CARTESIAN_POINT('',(19.3941040036879,11.589834535998,36.2684889848672));
#43630=CARTESIAN_POINT('',(19.3941040087494,-1.3495818343519,36.2684889831927));
#43631=CARTESIAN_POINT('',(18.0708700189552,11.126372316702,38.0997295667639));
#43632=CARTESIAN_POINT('Ctrl Pts',(19.3941040090521,11.7619801941421,36.2684889830926));
#43633=CARTESIAN_POINT('Ctrl Pts',(19.4044891081785,11.7612816111124,36.265053410023));
#43634=CARTESIAN_POINT('Ctrl Pts',(19.4149032568815,11.7605802509376,36.2617062224656));
#43635=CARTESIAN_POINT('Ctrl Pts',(19.4333417291731,11.7593367408316,36.2559525142545));
#43636=CARTESIAN_POINT('Ctrl Pts',(19.4413541858722,11.7587957973654,36.2535093890524));
#43637=CARTESIAN_POINT('Ctrl Pts',(19.4551775088053,11.7578614464176,36.2493926471621));
#43638=CARTESIAN_POINT('Ctrl Pts',(19.4609808468757,11.7574688531459,36.2476940121907));
#43639=CARTESIAN_POINT('Ctrl Pts',(19.4729858020327,11.756655992765,36.2442413604791));
#43640=CARTESIAN_POINT('Ctrl Pts',(19.479188407167,11.7562356107018,36.2424910831708));
#43641=CARTESIAN_POINT('Ctrl Pts',(19.4936899410176,11.7552517762315,36.2384773232609));
#43642=CARTESIAN_POINT('Ctrl Pts',(19.5019954174636,11.7546875477548,36.2362382170528));
#43643=CARTESIAN_POINT('Ctrl Pts',(19.5288566781731,11.7528601414259,36.229188951451));
#43644=CARTESIAN_POINT('Ctrl Pts',(19.5474687807113,11.7515899306252,36.2245999200712));
#43645=CARTESIAN_POINT('Ctrl Pts',(19.6429945344472,11.7450481072071,36.202551706652));
#43646=CARTESIAN_POINT('Ctrl Pts',(19.7208487991724,11.739637640203,36.1895459509694));
#43647=CARTESIAN_POINT('Ctrl Pts',(19.9051343753092,11.7266644358477,36.1702661899108));
#43648=CARTESIAN_POINT('Ctrl Pts',(20.0117272473897,11.7190265464471,36.1679720693119));
#43649=CARTESIAN_POINT('Ctrl Pts',(20.2034270806906,11.7053700045545,36.1797154639987));
#43650=CARTESIAN_POINT('Ctrl Pts',(20.2884659233915,11.6993454636034,36.1906371933352));
#43651=CARTESIAN_POINT('Ctrl Pts',(20.38169698589,11.6929589644814,36.2089850068213));
#43652=CARTESIAN_POINT('Ctrl Pts',(20.3908744169038,11.6923327222023,36.2108606477118));
#43653=CARTESIAN_POINT('Ctrl Pts',(20.4044846305104,11.6914079739603,36.2137456690271));
#43654=CARTESIAN_POINT('Ctrl Pts',(20.4089279258414,11.6911067046575,36.2147039569472));
#43655=CARTESIAN_POINT('Ctrl Pts',(20.4168456537537,11.6905710346533,36.2164408862365));
#43656=CARTESIAN_POINT('Ctrl Pts',(20.4203213485379,11.690336296182,36.2172134484282));
#43657=CARTESIAN_POINT('Ctrl Pts',(20.4278283700572,11.6898301833444,36.2189039004153));
#43658=CARTESIAN_POINT('Ctrl Pts',(20.431858882062,11.6895590011233,36.2198251259853));
#43659=CARTESIAN_POINT('Ctrl Pts',(20.4430870462426,11.688804996969,36.2224294781767));
#43660=CARTESIAN_POINT('Ctrl Pts',(20.4502781276192,11.6883237617114,36.2241410481966));
#43661=CARTESIAN_POINT('Ctrl Pts',(20.491830317535,11.6855517581262,36.2342837170584));
#43662=CARTESIAN_POINT('Ctrl Pts',(20.5259666613401,11.6833090048776,36.2436180985407));
#43663=CARTESIAN_POINT('Ctrl Pts',(20.6367183710823,11.6760883336552,36.2772032930524));
#43664=CARTESIAN_POINT('Ctrl Pts',(20.7120822538879,11.6712612540214,36.3053024932868));
#43665=CARTESIAN_POINT('Ctrl Pts',(20.9264804106436,11.6572239287648,36.4008799376506));
#43666=CARTESIAN_POINT('Ctrl Pts',(21.0594091813543,11.6480767351947,36.4804257125253));
#43667=CARTESIAN_POINT('Ctrl Pts',(21.1985418401572,11.6369230974557,36.5882102153351));
#43668=CARTESIAN_POINT('Ctrl Pts',(21.2154250937131,11.6355411459726,36.6017501285546));
#43669=CARTESIAN_POINT('Ctrl Pts',(21.2385142355628,11.6336093312208,36.6209141197064));
#43670=CARTESIAN_POINT('Ctrl Pts',(21.2449170838421,11.6330690445826,36.6262992149943));
#43671=CARTESIAN_POINT('Ctrl Pts',(21.2558848672494,11.6321355242298,36.6356461189588));
#43672=CARTESIAN_POINT('Ctrl Pts',(21.2604666215982,11.6317431013556,36.6395880775738));
#43673=CARTESIAN_POINT('Ctrl Pts',(21.2698966061139,11.630930307761,36.6477786936579));
#43674=CARTESIAN_POINT('Ctrl Pts',(21.2747422104012,11.6305098208214,36.6520302461213));
#43675=CARTESIAN_POINT('Ctrl Pts',(21.2860110471288,11.6295252436052,36.6620179748811));
#43676=CARTESIAN_POINT('Ctrl Pts',(21.2924173188268,11.6289603737401,36.6677729970963));
#43677=CARTESIAN_POINT('Ctrl Pts',(21.3129981639976,11.627128781812,36.6865121571082));
#43678=CARTESIAN_POINT('Ctrl Pts',(21.3270168934776,11.6258549817018,36.6996649758481));
#43679=CARTESIAN_POINT('Ctrl Pts',(21.3978402073543,11.619281409724,36.7681322880924));
#43680=CARTESIAN_POINT('Ctrl Pts',(21.4513851287496,11.6138412600597,36.8266944002168));
#43681=CARTESIAN_POINT('Ctrl Pts',(21.5688754656985,11.600740761414,36.9722620377601));
#43682=CARTESIAN_POINT('Ctrl Pts',(21.6294271448523,11.5930019546244,37.0616707265058));
#43683=CARTESIAN_POINT('Ctrl Pts',(21.7232099611914,11.579385560088,37.228729786257));
#43684=CARTESIAN_POINT('Ctrl Pts',(21.7594303467048,11.5734955139161,37.30440419551));
#43685=CARTESIAN_POINT('Ctrl Pts',(21.7940981209714,11.5672333016133,37.3908864627234));
#43686=CARTESIAN_POINT('Ctrl Pts',(21.7975159053477,11.5666078437841,37.3995953633059));
#43687=CARTESIAN_POINT('Ctrl Pts',(21.8024991682618,11.5656840256995,37.4125700435162));
#43688=CARTESIAN_POINT('Ctrl Pts',(21.8041130871613,11.5653829100184,37.4168168865981));
#43689=CARTESIAN_POINT('Ctrl Pts',(21.8069650112877,11.5648474068196,37.4244019829029));
#43690=CARTESIAN_POINT('Ctrl Pts',(21.8082087890132,11.5646126823845,37.4277379909748));
#43691=CARTESIAN_POINT('Ctrl Pts',(21.810877506984,11.5641064792307,37.4349569050847));
#43692=CARTESIAN_POINT('Ctrl Pts',(21.8122991947508,11.5638351932976,37.4388409473546));
#43693=CARTESIAN_POINT('Ctrl Pts',(21.8162293395495,11.5630806074456,37.449686006512));
#43694=CARTESIAN_POINT('Ctrl Pts',(21.8187102895848,11.5625988981783,37.4566570192788));
#43695=CARTESIAN_POINT('Ctrl Pts',(21.8328619682382,11.5598185851996,37.4971567951531));
#43696=CARTESIAN_POINT('Ctrl Pts',(21.8436463480084,11.5575683338466,37.5309908132421));
#43697=CARTESIAN_POINT('Ctrl Pts',(21.8759023823103,11.550311031841,37.6427629675267));
#43698=CARTESIAN_POINT('Ctrl Pts',(21.8934125656299,11.5454565748662,37.7217586844452));
#43699=CARTESIAN_POINT('Ctrl Pts',(21.9296881269651,11.5314324146581,37.9534749478192));
#43700=CARTESIAN_POINT('Ctrl Pts',(21.9352265552165,11.5223223328693,38.107601150019));
#43701=CARTESIAN_POINT('Ctrl Pts',(21.9206143802755,11.5112094319007,38.282354584335));
#43702=CARTESIAN_POINT('Ctrl Pts',(21.9184433106685,11.5098247271884,38.3039313502964));
#43703=CARTESIAN_POINT('Ctrl Pts',(21.9149304248526,11.5078896704848,38.3337822450996));
#43704=CARTESIAN_POINT('Ctrl Pts',(21.9138976713883,11.5073489378651,38.3420916561724));
#43705=CARTESIAN_POINT('Ctrl Pts',(21.9120261209,11.5064148535698,38.3563888137574));
#43706=CARTESIAN_POINT('Ctrl Pts',(21.9112132041025,11.5060223150222,38.3623798732914));
#43707=CARTESIAN_POINT('Ctrl Pts',(21.9094755146625,11.5052094762245,38.3747496283011));
#43708=CARTESIAN_POINT('Ctrl Pts',(21.9085469115264,11.5047890606146,38.3811277008114));
#43709=CARTESIAN_POINT('Ctrl Pts',(21.9063039393352,11.5038049882842,38.3960099590994));
#43710=CARTESIAN_POINT('Ctrl Pts',(21.9049646050337,11.5032405543671,38.4045101879026));
#43711=CARTESIAN_POINT('Ctrl Pts',(21.9004555137718,11.5014118080604,38.4319329832436));
#43712=CARTESIAN_POINT('Ctrl Pts',(21.8970604060537,11.5001404483009,38.4508168126058));
#43713=CARTESIAN_POINT('Ctrl Pts',(21.8782463902904,11.4935884710089,38.5471850493148));
#43714=CARTESIAN_POINT('Ctrl Pts',(21.8583617419863,11.4881685128589,38.6237105414434));
#43715=CARTESIAN_POINT('Ctrl Pts',(21.8006607427853,11.4751520921861,38.800423663352));
#43716=CARTESIAN_POINT('Ctrl Pts',(21.7590865108009,11.467479292573,38.8991147880653));
#43717=CARTESIAN_POINT('Ctrl Pts',(21.6701682482757,11.4538356887566,39.0691785123149));
#43718=CARTESIAN_POINT('Ctrl Pts',(21.6258388761496,11.4478568294055,39.1418351589144));
#43719=CARTESIAN_POINT('Ctrl Pts',(21.5714609862753,11.4415124952514,39.218990882663));
#43720=CARTESIAN_POINT('Ctrl Pts',(21.5660112163951,11.4408864935662,39.226605124111));
#43721=CARTESIAN_POINT('Ctrl Pts',(21.5578341665533,11.4399620305949,39.237855843497));
#43722=CARTESIAN_POINT('Ctrl Pts',(21.5551492258448,11.4396608083972,39.2415227100084));
#43723=CARTESIAN_POINT('Ctrl Pts',(21.5503377478702,11.4391251895512,39.2480453393494));
#43724=CARTESIAN_POINT('Ctrl Pts',(21.5482162445073,11.4388904553942,39.2509047287409));
#43725=CARTESIAN_POINT('Ctrl Pts',(21.5436138237458,11.4383843149102,39.2570721746336));
#43726=CARTESIAN_POINT('Ctrl Pts',(21.5411301890773,11.4381131009247,39.2603781259911));
#43727=CARTESIAN_POINT('Ctrl Pts',(21.5341757510771,11.4373589186249,39.2695734235797));
#43728=CARTESIAN_POINT('Ctrl Pts',(21.5296816305831,11.4368775382034,39.2754451674588));
#43729=CARTESIAN_POINT('Ctrl Pts',(21.5034662142887,11.4341029933899,39.3092916452899));
#43730=CARTESIAN_POINT('Ctrl Pts',(21.4810099799045,11.4318579470929,39.3366918632568));
#43731=CARTESIAN_POINT('Ctrl Pts',(21.405092404967,11.4246260889572,39.4242873599754));
#43732=CARTESIAN_POINT('Ctrl Pts',(21.3486145402051,11.419790650427,39.4817607124033));
#43733=CARTESIAN_POINT('Ctrl Pts',(21.1739862551003,11.4057576538502,39.638527125597));
#43734=CARTESIAN_POINT('Ctrl Pts',(21.0473504373242,11.3966220873006,39.7273783367911));
#43735=CARTESIAN_POINT('Ctrl Pts',(20.8924091828192,11.3854810264254,39.8104436489183));
#43736=CARTESIAN_POINT('Ctrl Pts',(20.8731508924725,11.3840980144002,39.8203543485665));
#43737=CARTESIAN_POINT('Ctrl Pts',(20.8462255066924,11.3821649506419,39.8336421170417));
#43738=CARTESIAN_POINT('Ctrl Pts',(20.8386966625309,11.3816244919909,39.8372968954115));
#43739=CARTESIAN_POINT('Ctrl Pts',(20.825689315217,11.3806907541416,39.8435068832587));
#43740=CARTESIAN_POINT('Ctrl Pts',(20.8202221005183,11.3802982866656,39.8460855653937));
#43741=CARTESIAN_POINT('Ctrl Pts',(20.8089000169826,11.3794854757088,39.8513608623392));
#43742=CARTESIAN_POINT('Ctrl Pts',(20.8030435785427,11.3790650163406,39.8540539093432));
#43743=CARTESIAN_POINT('Ctrl Pts',(20.7893340927644,11.3780806341408,39.8602750819948));
#43744=CARTESIAN_POINT('Ctrl Pts',(20.7814707561896,11.3775159326444,39.8637800677702));
#43745=CARTESIAN_POINT('Ctrl Pts',(20.7559879087411,11.3756854400817,39.8749348729003));
#43746=CARTESIAN_POINT('Ctrl Pts',(20.7382779897368,11.3744125828281,39.8823740028251));
#43747=CARTESIAN_POINT('Ctrl Pts',(20.6470127824749,11.3678473587451,39.9191168018251));
#43748=CARTESIAN_POINT('Ctrl Pts',(20.571824014896,11.362415015562,39.9441328264967));
#43749=CARTESIAN_POINT('Ctrl Pts',(20.3914487583912,11.3493457414456,39.9920520667622));
#43750=CARTESIAN_POINT('Ctrl Pts',(20.2854579677333,11.3416311068129,40.0109171279271));
#43751=CARTESIAN_POINT('Ctrl Pts',(20.0945721445837,11.3280042424927,40.0286513738939));
#43752=CARTESIAN_POINT('Ctrl Pts',(20.0102555688925,11.3220812178345,40.0309423476456));
#43753=CARTESIAN_POINT('Ctrl Pts',(19.9166987983089,11.3157884901401,40.0273533783619));
#43754=CARTESIAN_POINT('Ctrl Pts',(19.9073498451879,11.3151628194661,40.0269265924695));
#43755=CARTESIAN_POINT('Ctrl Pts',(19.8934667745314,11.3142387489903,40.0261915465926));
#43756=CARTESIAN_POINT('Ctrl Pts',(19.8889302145428,11.3139375916165,40.0259352808703));
#43757=CARTESIAN_POINT('Ctrl Pts',(19.8808405792688,11.3134020431568,40.0254496268523));
#43758=CARTESIAN_POINT('Ctrl Pts',(19.8772872023722,11.313167314922,40.0252264290502));
#43759=CARTESIAN_POINT('Ctrl Pts',(19.8696076763202,11.3126611363241,40.0247227077444));
#43760=CARTESIAN_POINT('Ctrl Pts',(19.865481814334,11.3123898785727,40.0244387541049));
#43761=CARTESIAN_POINT('Ctrl Pts',(19.8539788540989,11.3116354507978,40.023609913492));
#43762=CARTESIAN_POINT('Ctrl Pts',(19.8466038318823,11.3111538703452,40.0230358536065));
#43763=CARTESIAN_POINT('Ctrl Pts',(19.8038869549981,11.3083758187503,40.0194635318891));
#43764=CARTESIAN_POINT('Ctrl Pts',(19.7686272527186,11.3061276080525,40.0155332454391));
#43765=CARTESIAN_POINT('Ctrl Pts',(19.653571628061,11.2988802897344,39.9994845890002));
#43766=CARTESIAN_POINT('Ctrl Pts',(19.5744211197147,11.2940332963429,39.983331918372));
#43767=CARTESIAN_POINT('Ctrl Pts',(19.3479530451862,11.2800051697463,39.9221030454742));
#43768=CARTESIAN_POINT('Ctrl Pts',(19.2047549580786,11.2708845864594,39.8643139753325));
#43769=CARTESIAN_POINT('Ctrl Pts',(19.0509629410205,11.259760336108,39.7796847292297));
#43770=CARTESIAN_POINT('Ctrl Pts',(19.0321559719663,11.2583765918905,39.768918813538));
#43771=CARTESIAN_POINT('Ctrl Pts',(19.0057022560993,11.2563947990807,39.7531780382109));
#43772=CARTESIAN_POINT('Ctrl Pts',(18.9979028270842,11.2558060482059,39.7484619743615));
#43773=CARTESIAN_POINT('Ctrl Pts',(18.984659954302,11.2547986241385,39.740325721691));
#43774=CARTESIAN_POINT('Ctrl Pts',(18.9791996004789,11.254380963533,39.7369332375866));
#43775=CARTESIAN_POINT('Ctrl Pts',(18.9682747956089,11.2535406955188,39.7300698041833));
#43776=CARTESIAN_POINT('Ctrl Pts',(18.9628106577409,11.2531180794708,39.7265985154545));
#43777=CARTESIAN_POINT('Ctrl Pts',(18.9518390687641,11.2522647029719,39.7195506605933));
#43778=CARTESIAN_POINT('Ctrl Pts',(18.9463322036395,11.2518339187012,39.7159733454214));
#43779=CARTESIAN_POINT('Ctrl Pts',(18.9262605435618,11.2502546803487,39.7027883754893));
#43780=CARTESIAN_POINT('Ctrl Pts',(18.9118083780358,11.2490999526442,39.6930115997608));
#43781=CARTESIAN_POINT('Ctrl Pts',(18.8787194124754,11.2464142797585,39.6699667833101));
#43782=CARTESIAN_POINT('Ctrl Pts',(18.8601823536816,11.2448782670727,39.6565607969657));
#43783=CARTESIAN_POINT('Ctrl Pts',(18.7970673038197,11.239537298614,39.6091840232765));
#43784=CARTESIAN_POINT('Ctrl Pts',(18.7537372053046,11.2356736062469,39.5736049495915));
#43785=CARTESIAN_POINT('Ctrl Pts',(18.6489189000324,11.2258275129363,39.4796037696543));
#43786=CARTESIAN_POINT('Ctrl Pts',(18.5896192353827,11.2197814417717,39.4189204315053));
#43787=CARTESIAN_POINT('Ctrl Pts',(18.4628524749788,11.205873370371,39.2708373986103));
#43788=CARTESIAN_POINT('Ctrl Pts',(18.3984930156784,11.1980319791849,39.1811401381752));
#43789=CARTESIAN_POINT('Ctrl Pts',(18.3374625237523,11.1900129232928,39.0785680120811));
#43790=CARTESIAN_POINT('Ctrl Pts',(18.3328414929143,11.1894015883336,39.07067437102));
#43791=CARTESIAN_POINT('Ctrl Pts',(18.3260300727759,11.1884945362618,39.0588469662555));
#43792=CARTESIAN_POINT('Ctrl Pts',(18.3237971101384,11.1881962044461,39.0549380581947));
#43793=CARTESIAN_POINT('Ctrl Pts',(18.3198242493175,11.1876637064792,39.0479265038123));
#43794=CARTESIAN_POINT('Ctrl Pts',(18.3180792372086,11.1874292188806,39.04482684032));
#43795=CARTESIAN_POINT('Ctrl Pts',(18.3143090469007,11.1869212992067,39.0380863093922));
#43796=CARTESIAN_POINT('Ctrl Pts',(18.3122870907346,11.1866480718237,39.0344437114882));
#43797=CARTESIAN_POINT('Ctrl Pts',(18.3066401411706,11.1858825719376,39.0241924901261));
#43798=CARTESIAN_POINT('Ctrl Pts',(18.3030420068112,11.1853919655264,39.0175690405687));
#43799=CARTESIAN_POINT('Ctrl Pts',(18.2815949770577,11.1824492952118,38.977531646426));
#43800=CARTESIAN_POINT('Ctrl Pts',(18.2646932560577,11.1800524252294,38.94361637071));
#43801=CARTESIAN_POINT('Ctrl Pts',(18.1784772327418,11.1672607197251,38.7570404151906));
#43802=CARTESIAN_POINT('Ctrl Pts',(18.1282856364326,11.1575868259096,38.5963302243795));
#43803=CARTESIAN_POINT('Ctrl Pts',(18.0915188350189,11.1445451990656,38.3853170457206));
#43804=CARTESIAN_POINT('Ctrl Pts',(18.0851948544881,11.1416810364982,38.3392216197336));
#43805=CARTESIAN_POINT('Ctrl Pts',(18.0785841656132,11.1375438959706,38.2734570878014));
#43806=CARTESIAN_POINT('Ctrl Pts',(18.0769221894167,11.1363099360548,38.2539411024129));
#43807=CARTESIAN_POINT('Ctrl Pts',(18.0741336388994,11.1337702160291,38.2140135981025));
#43808=CARTESIAN_POINT('Ctrl Pts',(18.0730337813545,11.132463837611,38.1936027932038));
#43809=CARTESIAN_POINT('Ctrl Pts',(18.0719215865466,11.1305754392644,38.1643044276047));
#43810=CARTESIAN_POINT('Ctrl Pts',(18.0716459911718,11.1300015740114,38.1554277922072));
#43811=CARTESIAN_POINT('Ctrl Pts',(18.0712768607941,11.1290097742771,38.1401346046638));
#43812=CARTESIAN_POINT('Ctrl Pts',(18.0711540311399,11.1285927547571,38.1337188516865));
#43813=CARTESIAN_POINT('Ctrl Pts',(18.0709862947616,11.1278206857492,38.1218682568075));
#43814=CARTESIAN_POINT('Ctrl Pts',(18.0709323413288,11.1274659214192,38.1164335908947));
#43815=CARTESIAN_POINT('Ctrl Pts',(18.0708799375339,11.1268647404811,38.1072424114113));
#43816=CARTESIAN_POINT('Ctrl Pts',(18.0708694923661,11.1266186994183,38.1034859791869));
#43817=CARTESIAN_POINT('Ctrl Pts',(18.0708700189552,11.126372316702,38.0997295667639));
#43818=CARTESIAN_POINT('Ctrl Pts',(18.0708700189004,11.126372342366,38.099729958043));
#43819=CARTESIAN_POINT('Ctrl Pts',(18.0708709872349,11.1259186174904,38.0928123546099));
#43820=CARTESIAN_POINT('Ctrl Pts',(18.0709091639535,11.1254637368608,38.0858948654552));
#43821=CARTESIAN_POINT('Ctrl Pts',(18.0711428693587,11.1240498725853,38.0644498650811));
#43822=CARTESIAN_POINT('Ctrl Pts',(18.0714653045813,11.1230869765028,38.0499245414285));
#43823=CARTESIAN_POINT('Ctrl Pts',(18.0746986210286,11.1166533098097,37.9534163132403));
#43824=CARTESIAN_POINT('Ctrl Pts',(18.0826718787771,11.1110271372982,37.8716979530662));
#43825=CARTESIAN_POINT('Ctrl Pts',(18.1164219929695,11.0962795412273,37.6638884925326));
#43826=CARTESIAN_POINT('Ctrl Pts',(18.1496497491305,11.0870037676159,37.5394111811541));
#43827=CARTESIAN_POINT('Ctrl Pts',(18.2155494381882,11.0738309847884,37.3646981679544));
#43828=CARTESIAN_POINT('Ctrl Pts',(18.238555699285,11.0697780377839,37.3111730665822));
#43829=CARTESIAN_POINT('Ctrl Pts',(18.2693069981766,11.0650156706717,37.2477117991244));
#43830=CARTESIAN_POINT('Ctrl Pts',(18.2747691295907,11.0641916014966,37.2367086778925));
#43831=CARTESIAN_POINT('Ctrl Pts',(18.2826356033553,11.0630358269944,37.2212350531694));
#43832=CARTESIAN_POINT('Ctrl Pts',(18.2849529157069,11.062699034814,37.2167209938264));
#43833=CARTESIAN_POINT('Ctrl Pts',(18.2889605280384,11.0621229081025,37.2089895117613));
#43834=CARTESIAN_POINT('Ctrl Pts',(18.2906421501433,11.0618830393679,37.2057676438564));
#43835=CARTESIAN_POINT('Ctrl Pts',(18.2939124520734,11.0614201964878,37.1995449127445));
#43836=CARTESIAN_POINT('Ctrl Pts',(18.2954999519789,11.0611971482145,37.1965434863292));
#43837=CARTESIAN_POINT('Ctrl Pts',(18.2997957715752,11.060597895667,37.1884731673233));
#43838=CARTESIAN_POINT('Ctrl Pts',(18.3025188583325,11.0602226101327,37.1834121096186));
#43839=CARTESIAN_POINT('Ctrl Pts',(18.312674706629,11.0588394723014,37.1647372082706));
#43840=CARTESIAN_POINT('Ctrl Pts',(18.3202491977173,11.0578401215727,37.151200540538));
#43841=CARTESIAN_POINT('Ctrl Pts',(18.3999604669722,11.0476327056034,37.0126926868956));
#43842=CARTESIAN_POINT('Ctrl Pts',(18.4857501115488,11.0391669846012,36.896079869725));
#43843=CARTESIAN_POINT('Ctrl Pts',(18.65994591166,11.023811867071,36.7077399526684));
#43844=CARTESIAN_POINT('Ctrl Pts',(18.7431664487442,11.0170228411159,36.6321792125026));
#43845=CARTESIAN_POINT('Ctrl Pts',(18.8507850777767,11.0084631781482,36.5503624077049));
#43846=CARTESIAN_POINT('Ctrl Pts',(18.8693422943006,11.0069950429047,36.5367710706089));
#43847=CARTESIAN_POINT('Ctrl Pts',(18.8955221226699,11.0049323855551,36.5183069721611));
#43848=CARTESIAN_POINT('Ctrl Pts',(18.9029431750116,11.0043486335185,36.5131507525847));
#43849=CARTESIAN_POINT('Ctrl Pts',(18.915739945366,11.0033434817161,36.5043921024277));
#43850=CARTESIAN_POINT('Ctrl Pts',(18.9210981130249,11.0029230473476,36.5007641995449));
#43851=CARTESIAN_POINT('Ctrl Pts',(18.9318453578966,11.0020805670416,36.493566059421));
#43852=CARTESIAN_POINT('Ctrl Pts',(18.9372343295317,11.0016585285829,36.489995815887));
#43853=CARTESIAN_POINT('Ctrl Pts',(18.9502646693496,11.0006389694786,36.4814570228568));
#43854=CARTESIAN_POINT('Ctrl Pts',(18.9579234461513,11.0000404600824,36.476515449909));
#43855=CARTESIAN_POINT('Ctrl Pts',(18.9839090849794,10.9980120932452,36.4600087095519));
#43856=CARTESIAN_POINT('Ctrl Pts',(19.0023951585604,10.9965729802426,36.4486984842456));
#43857=CARTESIAN_POINT('Ctrl Pts',(19.139116232397,10.985953347471,36.3681829708129));
#43858=CARTESIAN_POINT('Ctrl Pts',(19.2641741872061,10.976326845162,36.3114720486756));
#43859=CARTESIAN_POINT('Ctrl Pts',(19.394104009089,10.9665681892825,36.2684889830804));
#43860=CARTESIAN_POINT('Ctrl Pts',(19.3941039816494,10.7965035432258,36.2684889921579));
#43861=CARTESIAN_POINT('Ctrl Pts',(19.3599116928284,10.7990471336171,36.2798004020081));
#43862=CARTESIAN_POINT('Ctrl Pts',(19.3260352778518,10.8015715106911,36.2920696020883));
#43863=CARTESIAN_POINT('Ctrl Pts',(19.2620765811673,10.8063228479862,36.3172823953138));
#43864=CARTESIAN_POINT('Ctrl Pts',(19.2319460337816,10.8085547174039,36.3300546763576));
#43865=CARTESIAN_POINT('Ctrl Pts',(19.1955772863557,10.8112284913409,36.3465751184865));
#43866=CARTESIAN_POINT('Ctrl Pts',(19.1890183817105,10.8117098744599,36.3495990355919));
#43867=CARTESIAN_POINT('Ctrl Pts',(19.1787653143114,10.8124609259612,36.3543961114865));
#43868=CARTESIAN_POINT('Ctrl Pts',(19.1750596392986,10.8127320711585,36.3561442873237));
#43869=CARTESIAN_POINT('Ctrl Pts',(19.1681396046576,10.8132378100208,36.3594358520478));
#43870=CARTESIAN_POINT('Ctrl Pts',(19.1649239886415,10.813472569004,36.3609763296577));
#43871=CARTESIAN_POINT('Ctrl Pts',(19.1575692678434,10.8140089580062,36.364524796596));
#43872=CARTESIAN_POINT('Ctrl Pts',(19.1534330664639,10.8143102209137,36.3665386799133));
#43873=CARTESIAN_POINT('Ctrl Pts',(19.1426065060084,10.8150978447772,36.3718580385094));
#43874=CARTESIAN_POINT('Ctrl Pts',(19.1359279745571,10.8155827622142,36.3751876096739));
#43875=CARTESIAN_POINT('Ctrl Pts',(19.0903420554511,10.8188873733811,36.3982456237854));
#43876=CARTESIAN_POINT('Ctrl Pts',(19.0520908374519,10.8216337703324,36.4192518243906));
#43877=CARTESIAN_POINT('Ctrl Pts',(18.8972017639679,10.8327800232323,36.5112832481035));
#43878=CARTESIAN_POINT('Ctrl Pts',(18.7875498857725,10.840756397621,36.5932964814711));
#43879=CARTESIAN_POINT('Ctrl Pts',(18.6211573705008,10.8544391580279,36.7477710458493));
#43880=CARTESIAN_POINT('Ctrl Pts',(18.5592650701366,10.8599805149514,36.8139167925076));
#43881=CARTESIAN_POINT('Ctrl Pts',(18.489261821023,10.8670301788138,36.9001511868764));
#43882=CARTESIAN_POINT('Ctrl Pts',(18.4765344795101,10.8683473724555,36.9163531879437));
#43883=CARTESIAN_POINT('Ctrl Pts',(18.4587116599003,10.870245297248,36.9398055252864));
#43884=CARTESIAN_POINT('Ctrl Pts',(18.4534025584471,10.8708176949897,36.9468923224708));
#43885=CARTESIAN_POINT('Ctrl Pts',(18.444288890421,10.8718127181908,36.9592337737255));
#43886=CARTESIAN_POINT('Ctrl Pts',(18.4404616605289,10.8722344610605,36.9644715743379));
#43887=CARTESIAN_POINT('Ctrl Pts',(18.4331558029089,10.8730471098984,36.9745766974896));
#43888=CARTESIAN_POINT('Ctrl Pts',(18.4296732504468,10.8734378590631,36.9794411010226));
#43889=CARTESIAN_POINT('Ctrl Pts',(18.4215135114813,10.8743614556455,36.9909513063783));
#43890=CARTESIAN_POINT('Ctrl Pts',(18.416855610414,10.8748950274869,36.9976105780742));
#43891=CARTESIAN_POINT('Ctrl Pts',(18.4007260589849,10.8767652214336,37.0209836121035));
#43892=CARTESIAN_POINT('Ctrl Pts',(18.389476227185,10.8781101097891,37.0378481144686));
#43893=CARTESIAN_POINT('Ctrl Pts',(18.2864409875565,10.8908208539611,37.1977084127085));
#43894=CARTESIAN_POINT('Ctrl Pts',(18.213677883871,10.9029127476218,37.3520403874864));
#43895=CARTESIAN_POINT('Ctrl Pts',(18.1408071899472,10.9200085100449,37.5805359071926));
#43896=CARTESIAN_POINT('Ctrl Pts',(18.123185067349,10.9249735967894,37.6483276302469));
#43897=CARTESIAN_POINT('Ctrl Pts',(18.1028112370222,10.9320638973313,37.7488868729032));
#43898=CARTESIAN_POINT('Ctrl Pts',(18.0971475691218,10.9342878673296,37.7810038130815));
#43899=CARTESIAN_POINT('Ctrl Pts',(18.0912280363286,10.9369535071018,37.820385625047));
#43900=CARTESIAN_POINT('Ctrl Pts',(18.090195650858,10.9374343794746,37.8275262213884));
#43901=CARTESIAN_POINT('Ctrl Pts',(18.0886400295997,10.9381848122368,37.8387292697301));
#43902=CARTESIAN_POINT('Ctrl Pts',(18.0880896435333,10.9384558455259,37.8427877908128));
#43903=CARTESIAN_POINT('Ctrl Pts',(18.0870842461246,10.9389614886362,37.8503831117824));
#43904=CARTESIAN_POINT('Ctrl Pts',(18.0866261206356,10.9391962630999,37.8539193824085));
#43905=CARTESIAN_POINT('Ctrl Pts',(18.0855990819622,10.9397328343895,37.8620233860938));
#43906=CARTESIAN_POINT('Ctrl Pts',(18.0850367102923,10.9400342631664,37.8665918940887));
#43907=CARTESIAN_POINT('Ctrl Pts',(18.0836044799661,10.9408226066535,37.8785805309168));
#43908=CARTESIAN_POINT('Ctrl Pts',(18.0827613532863,10.9413080735657,37.8860038635187));
#43909=CARTESIAN_POINT('Ctrl Pts',(18.0772713260349,10.9446246177656,37.9369802348705));
#43910=CARTESIAN_POINT('Ctrl Pts',(18.0740653448849,10.9473817967564,37.9806794801089));
#43911=CARTESIAN_POINT('Ctrl Pts',(18.0713816451734,10.9516208186538,38.0491571450946));
#43912=CARTESIAN_POINT('Ctrl Pts',(18.0708884270925,10.9531345312603,38.0738777395733));
#43913=CARTESIAN_POINT('Ctrl Pts',(18.0708086691379,10.9598246133687,38.1839165646558));
#43914=CARTESIAN_POINT('Ctrl Pts',(18.0764063827742,10.9648818282327,38.2691444193352));
#43915=CARTESIAN_POINT('Ctrl Pts',(18.0919149180857,10.9719379610865,38.3860354226241));
#43916=CARTESIAN_POINT('Ctrl Pts',(18.0970199238408,10.9738937876136,38.4182321512069));
#43917=CARTESIAN_POINT('Ctrl Pts',(18.1197604123069,10.981459504979,38.5413898537029));
#43918=CARTESIAN_POINT('Ctrl Pts',(18.1431215745388,10.9871594415207,38.6311544189538));
#43919=CARTESIAN_POINT('Ctrl Pts',(18.1771769418904,10.9939387332478,38.7316974012605));
#43920=CARTESIAN_POINT('Ctrl Pts',(18.1816507373773,10.9948067610656,38.7444621417286));
#43921=CARTESIAN_POINT('Ctrl Pts',(18.1890575470281,10.996209189312,38.7649041357443));
#43922=CARTESIAN_POINT('Ctrl Pts',(18.1919060863509,10.9967408087142,38.7726116812072));
#43923=CARTESIAN_POINT('Ctrl Pts',(18.1970635808618,10.9976899284244,38.7862972320725));
#43924=CARTESIAN_POINT('Ctrl Pts',(18.1993532590413,10.9981067843807,38.7922824097363));
#43925=CARTESIAN_POINT('Ctrl Pts',(18.2042001618036,10.9989799627064,38.8047653923189));
#43926=CARTESIAN_POINT('Ctrl Pts',(18.2067629266385,10.9994364648422,38.8112609321807));
#43927=CARTESIAN_POINT('Ctrl Pts',(18.2135453386114,11.0006313360473,38.8281818402969));
#43928=CARTESIAN_POINT('Ctrl Pts',(18.2178209416765,11.0013715693115,38.8385843518228));
#43929=CARTESIAN_POINT('Ctrl Pts',(18.2372307904447,11.0046758581754,38.8846583725112));
#43930=CARTESIAN_POINT('Ctrl Pts',(18.2533458893538,11.0072727381979,38.9199043233803));
#43931=CARTESIAN_POINT('Ctrl Pts',(18.299904155933,11.0144101218393,39.0141219156325));
#43932=CARTESIAN_POINT('Ctrl Pts',(18.3323441975341,11.0190139728566,39.072042860555));
#43933=CARTESIAN_POINT('Ctrl Pts',(18.4302313154363,11.0319456277407,39.2274458135195));
#43934=CARTESIAN_POINT('Ctrl Pts',(18.5016846873692,11.0404031915967,39.3208019009502));
#43935=CARTESIAN_POINT('Ctrl Pts',(18.5910050510469,11.0496996635165,39.4177580707008));
#43936=CARTESIAN_POINT('Ctrl Pts',(18.6009566592841,11.0507195119575,39.4283188042161));
#43937=CARTESIAN_POINT('Ctrl Pts',(18.6447201610558,11.0551327647021,39.4737235406742));
#43938=CARTESIAN_POINT('Ctrl Pts',(18.6797247387762,11.0584806333226,39.5073997129096));
#43939=CARTESIAN_POINT('Ctrl Pts',(18.7217047583309,11.0622556370353,39.5448401158269));
#43940=CARTESIAN_POINT('Ctrl Pts',(18.7274741424071,11.0627694157682,39.549924008961));
#43941=CARTESIAN_POINT('Ctrl Pts',(18.7367570844875,11.0635878667725,39.5580059061044));
#43942=CARTESIAN_POINT('Ctrl Pts',(18.7402512052919,11.063894091051,39.5610259618359));
#43943=CARTESIAN_POINT('Ctrl Pts',(18.7464702786413,11.0644358179942,39.5663623646954));
#43944=CARTESIAN_POINT('Ctrl Pts',(18.7491908657074,11.0646716833239,39.5686837158875));
#43945=CARTESIAN_POINT('Ctrl Pts',(18.7549974618703,11.0651727058998,39.573610378352));
#43946=CARTESIAN_POINT('Ctrl Pts',(18.7580851967673,11.0654377101211,39.5762135649659));
#43947=CARTESIAN_POINT('Ctrl Pts',(18.7665134006095,11.0661572723944,39.5832739978637));
#43948=CARTESIAN_POINT('Ctrl Pts',(18.7718699030438,11.0666104712647,39.5877121402246));
#43949=CARTESIAN_POINT('Ctrl Pts',(18.7996774226552,11.0689427160613,39.6104995863804));
#43950=CARTESIAN_POINT('Ctrl Pts',(18.8225174276069,11.0707898234213,39.6283711268983));
#43951=CARTESIAN_POINT('Ctrl Pts',(18.9736937418759,11.0826415838328,39.7412599776763));
#43952=CARTESIAN_POINT('Ctrl Pts',(19.1130142084943,11.0918940290622,39.8205543686528));
#43953=CARTESIAN_POINT('Ctrl Pts',(19.3463140040522,11.1071517443397,39.9173782876406));
#43954=CARTESIAN_POINT('Ctrl Pts',(19.4345474521585,11.1128653962314,39.9467347430041));
#43955=CARTESIAN_POINT('Ctrl Pts',(19.5376584830146,11.1196599018256,39.9729564816677));
#43956=CARTESIAN_POINT('Ctrl Pts',(19.5508070994759,11.1205282867505,39.9761533476015));
#43957=CARTESIAN_POINT('Ctrl Pts',(19.5719940909266,11.1219311810019,39.9810691233432));
#43958=CARTESIAN_POINT('Ctrl Pts',(19.5800118711664,11.1224629062973,39.9828754800037));
#43959=CARTESIAN_POINT('Ctrl Pts',(19.5943014841957,11.1234121471048,39.9859990295698));
#43960=CARTESIAN_POINT('Ctrl Pts',(19.6005688362644,11.1238290176804,39.9873363158301));
#43961=CARTESIAN_POINT('Ctrl Pts',(19.6136781788222,11.1247021571285,39.9900652783141));
#43962=CARTESIAN_POINT('Ctrl Pts',(19.6205212827763,11.125158605422,39.9914510849688));
#43963=CARTESIAN_POINT('Ctrl Pts',(19.638403194324,11.1263531809751,39.9949714292462));
#43964=CARTESIAN_POINT('Ctrl Pts',(19.6494532769682,11.1270931707262,39.9970466397704));
#43965=CARTESIAN_POINT('Ctrl Pts',(19.6986293492169,11.1303948033599,40.0058376030066));
#43966=CARTESIAN_POINT('Ctrl Pts',(19.736931932925,11.1329892056909,40.0115009979894));
#43967=CARTESIAN_POINT('Ctrl Pts',(19.841184505067,11.140117768177,40.0237230516145));
#43968=CARTESIAN_POINT('Ctrl Pts',(19.907339601263,11.1447150814766,40.0280418147694));
#43969=CARTESIAN_POINT('Ctrl Pts',(20.0598071285967,11.1554507258419,40.0301300869685));
#43970=CARTESIAN_POINT('Ctrl Pts',(20.146013525069,11.1616261459808,40.025527963186));
#43971=CARTESIAN_POINT('Ctrl Pts',(20.3238671928586,11.1743842365249,40.0040186331108));
#43972=CARTESIAN_POINT('Ctrl Pts',(20.4152018114396,11.1809448982904,39.9862101381461));
#43973=CARTESIAN_POINT('Ctrl Pts',(20.5139520413686,11.1878219477999,39.9594310143172));
#43974=CARTESIAN_POINT('Ctrl Pts',(20.5229799169806,11.1884485669499,39.9569120638768));
#43975=CARTESIAN_POINT('Ctrl Pts',(20.5363594818685,11.1893737615224,39.9530735909714));
#43976=CARTESIAN_POINT('Ctrl Pts',(20.5407252768277,11.189675104094,39.9518043642341));
#43977=CARTESIAN_POINT('Ctrl Pts',(20.5485020966611,11.190210853103,39.9495136346206));
#43978=CARTESIAN_POINT('Ctrl Pts',(20.5519148110153,11.1904455977197,39.9484981138193));
#43979=CARTESIAN_POINT('Ctrl Pts',(20.5592834200984,11.1909516656761,39.9462832121868));
#43980=CARTESIAN_POINT('Ctrl Pts',(20.5632382687285,11.1912227971804,39.9450805665424));
#43981=CARTESIAN_POINT('Ctrl Pts',(20.5742509064289,11.1919765190596,39.9416929816526));
#43982=CARTESIAN_POINT('Ctrl Pts',(20.5813001478432,11.192457524681,39.9394801669547));
#43983=CARTESIAN_POINT('Ctrl Pts',(20.6219755840167,11.1952255295468,39.9264546392231));
#43984=CARTESIAN_POINT('Ctrl Pts',(20.6553149360056,11.1974646755207,39.9147597340614));
#43985=CARTESIAN_POINT('Ctrl Pts',(20.7631601280733,11.2046677806116,39.8735692398989));
#43986=CARTESIAN_POINT('Ctrl Pts',(20.8361565848331,11.2094817392772,39.8403463852523));
#43987=CARTESIAN_POINT('Ctrl Pts',(21.0434242734331,11.223525467744,39.7299514181623));
#43988=CARTESIAN_POINT('Ctrl Pts',(21.1707074125025,11.232690505048,39.6410755166232));
#43989=CARTESIAN_POINT('Ctrl Pts',(21.3021225149627,11.2438637108733,39.5235473003117));
#43990=CARTESIAN_POINT('Ctrl Pts',(21.3179935892802,11.245244302311,39.508865784622));
#43991=CARTESIAN_POINT('Ctrl Pts',(21.3396568095881,11.2471745140905,39.4881398082503));
#43992=CARTESIAN_POINT('Ctrl Pts',(21.3456617970365,11.2477145788709,39.482319362202));
#43993=CARTESIAN_POINT('Ctrl Pts',(21.3559406019377,11.2486478180218,39.4722259878023));
#43994=CARTESIAN_POINT('Ctrl Pts',(21.3602325698061,11.2490401826862,39.4679716489181));
#43995=CARTESIAN_POINT('Ctrl Pts',(21.3690617264055,11.2498529518913,39.4591372662695));
#43996=CARTESIAN_POINT('Ctrl Pts',(21.3735960821235,11.2502734730759,39.4545545100724));
#43997=CARTESIAN_POINT('Ctrl Pts',(21.3841357955715,11.2512582978363,39.4437949519513));
#43998=CARTESIAN_POINT('Ctrl Pts',(21.3901228794296,11.2518233821822,39.4376005194008));
#43999=CARTESIAN_POINT('Ctrl Pts',(21.4093467604036,11.2536563803627,39.4174423937141));
#44000=CARTESIAN_POINT('Ctrl Pts',(21.4224158544404,11.2549313874469,39.403321082275));
#44001=CARTESIAN_POINT('Ctrl Pts',(21.4883425497027,11.2615156652357,39.329913662011));
#44002=CARTESIAN_POINT('Ctrl Pts',(21.5377068651489,11.2669658296068,39.2676068853146));
#44003=CARTESIAN_POINT('Ctrl Pts',(21.6449092802338,11.2801040036711,39.1136662776948));
#44004=CARTESIAN_POINT('Ctrl Pts',(21.6991523084523,11.2878713152156,39.0198503426908));
#44005=CARTESIAN_POINT('Ctrl Pts',(21.7807163039062,11.3014743742508,38.8466746403488));
#44006=CARTESIAN_POINT('Ctrl Pts',(21.8112817039661,11.3073246293017,38.7691304706126));
#44007=CARTESIAN_POINT('Ctrl Pts',(21.8396022811142,11.3135499887683,38.6809418629148));
#44008=CARTESIAN_POINT('Ctrl Pts',(21.8423967566412,11.3141751729334,38.6720176575357));
#44009=CARTESIAN_POINT('Ctrl Pts',(21.8464520993388,11.3150986659946,38.6587287662054));
#44010=CARTESIAN_POINT('Ctrl Pts',(21.8477625699267,11.315399727561,38.6543795410763));
#44011=CARTESIAN_POINT('Ctrl Pts',(21.8500727631516,11.3159351714369,38.646613211717));
#44012=CARTESIAN_POINT('Ctrl Pts',(21.8510783970509,11.3161698903665,38.6431979389408));
#44013=CARTESIAN_POINT('Ctrl Pts',(21.8532320217961,11.3166761234742,38.6358084931247));
#44014=CARTESIAN_POINT('Ctrl Pts',(21.8543766844103,11.3169474446457,38.6318334147317));
#44015=CARTESIAN_POINT('Ctrl Pts',(21.8575338320387,11.3177022303112,38.6207354456465));
#44016=CARTESIAN_POINT('Ctrl Pts',(21.8595181494617,11.3181841027809,38.6136045148415));
#44017=CARTESIAN_POINT('Ctrl Pts',(21.8707928830716,11.3209672994778,38.5721651308519));
#44018=CARTESIAN_POINT('Ctrl Pts',(21.8791754197273,11.3232201539496,38.5376140448056));
#44019=CARTESIAN_POINT('Ctrl Pts',(21.9035123567488,11.3304902122526,38.4236405726242));
#44020=CARTESIAN_POINT('Ctrl Pts',(21.9154221619336,11.3353542084999,38.3434392082175));
#44021=CARTESIAN_POINT('Ctrl Pts',(21.9351995619217,11.3493738448671,38.1098046220398));
#44022=CARTESIAN_POINT('Ctrl Pts',(21.9298511034609,11.3584710349114,37.9559099938192));
#44023=CARTESIAN_POINT('Ctrl Pts',(21.903003268927,11.3695697724975,37.7828375909111));
#44024=CARTESIAN_POINT('Ctrl Pts',(21.8993154298238,11.3709554096055,37.7614527020763));
#44025=CARTESIAN_POINT('Ctrl Pts',(21.8937053396126,11.3728915629396,37.7319065387209));
#44026=CARTESIAN_POINT('Ctrl Pts',(21.8920893597929,11.3734324452901,37.723688213774));
#44027=CARTESIAN_POINT('Ctrl Pts',(21.8892147116964,11.3743667182407,37.7095555209315));
#44028=CARTESIAN_POINT('Ctrl Pts',(21.8879816504018,11.3747592949414,37.7036360201898));
#44029=CARTESIAN_POINT('Ctrl Pts',(21.8853768347011,11.3755721469248,37.6914191808932));
#44030=CARTESIAN_POINT('Ctrl Pts',(21.8840013123848,11.3759925372756,37.6851227316235));
#44031=CARTESIAN_POINT('Ctrl Pts',(21.8807161018317,11.3769764361389,37.6704380012747));
#44032=CARTESIAN_POINT('Ctrl Pts',(21.8787818147337,11.377540721035,37.6620554201458));
#44033=CARTESIAN_POINT('Ctrl Pts',(21.8723555920662,11.3793685004335,37.6350325505946));
#44034=CARTESIAN_POINT('Ctrl Pts',(21.8676419222311,11.3806390319143,37.6164466962242));
#44035=CARTESIAN_POINT('Ctrl Pts',(21.8421163091833,11.3871836995057,37.5217471785182));
#44036=CARTESIAN_POINT('Ctrl Pts',(21.8169281826751,11.3925968262206,37.4469012821207));
#44037=CARTESIAN_POINT('Ctrl Pts',(21.7471137408864,11.4055823897504,37.2750791087723));
#44038=CARTESIAN_POINT('Ctrl Pts',(21.6988838838886,11.4132303232867,37.1798414076816));
#44039=CARTESIAN_POINT('Ctrl Pts',(21.5982618390742,11.4268832344703,37.0163008268001));
#44040=CARTESIAN_POINT('Ctrl Pts',(21.5486896573047,11.4328947132075,36.9465665284007));
#44041=CARTESIAN_POINT('Ctrl Pts',(21.4887286844768,11.4392691597864,36.8730863196949));
#44042=CARTESIAN_POINT('Ctrl Pts',(21.4827544218702,11.4398953350182,36.8658729368436));
#44043=CARTESIAN_POINT('Ctrl Pts',(21.4738031219805,11.440820003263,36.8552238863034));
#44044=CARTESIAN_POINT('Ctrl Pts',(21.4708662039674,11.4411212589423,36.851754901205));
#44045=CARTESIAN_POINT('Ctrl Pts',(21.4656068219443,11.441656913563,36.8455870387391));
#44046=CARTESIAN_POINT('Ctrl Pts',(21.4632891263502,11.4418916502018,36.8428841869837));
#44047=CARTESIAN_POINT('Ctrl Pts',(21.4582638696937,11.4423977690667,36.8370565580966));
#44048=CARTESIAN_POINT('Ctrl Pts',(21.45555374836,11.4426689590957,36.833934070623));
#44049=CARTESIAN_POINT('Ctrl Pts',(21.4479701350849,11.4434230091762,36.8252530872529));
#44050=CARTESIAN_POINT('Ctrl Pts',(21.4430746366408,11.4439042822326,36.8197137815917));
#44051=CARTESIAN_POINT('Ctrl Pts',(21.4145592801289,11.4466769622597,36.7878197327932));
#44052=CARTESIAN_POINT('Ctrl Pts',(21.3902478784872,11.4489203266873,36.7620888555165));
#44053=CARTESIAN_POINT('Ctrl Pts',(21.3084467601857,11.4561439833719,36.6801508956201));
#44054=CARTESIAN_POINT('Ctrl Pts',(21.2481478521524,11.4609732944377,36.6268627006417));
#44055=CARTESIAN_POINT('Ctrl Pts',(21.0629033424365,11.4750093570021,36.4827203767234));
#44056=CARTESIAN_POINT('Ctrl Pts',(20.930196871483,11.484153341171,36.4029188517528));
#44057=CARTESIAN_POINT('Ctrl Pts',(20.7696565560982,11.4953035757415,36.3309211628988));
#44058=CARTESIAN_POINT('Ctrl Pts',(20.7497579451865,11.4966858913651,36.3223965262477));
#44059=CARTESIAN_POINT('Ctrl Pts',(20.7219751478198,11.4986181341304,36.311043752855));
#44060=CARTESIAN_POINT('Ctrl Pts',(20.7142091682948,11.4991584789886,36.307929178692));
#44061=CARTESIAN_POINT('Ctrl Pts',(20.7007987249799,11.5000920722507,36.3026518872159));
#44062=CARTESIAN_POINT('Ctrl Pts',(20.6951638609284,11.5004845095124,36.3004649776839));
#44063=CARTESIAN_POINT('Ctrl Pts',(20.6834984613273,11.5012973068433,36.2960005642646));
#44064=CARTESIAN_POINT('Ctrl Pts',(20.6774666089673,11.5017177830159,36.2937267363941));
#44065=CARTESIAN_POINT('Ctrl Pts',(20.6633511235763,11.5027022896786,36.2884862713249));
#44066=CARTESIAN_POINT('Ctrl Pts',(20.6552588505572,11.5032670994319,36.2855434595881));
#44067=CARTESIAN_POINT('Ctrl Pts',(20.6290432859745,11.505098303962,36.2762082313613));
#44068=CARTESIAN_POINT('Ctrl Pts',(20.6108445736694,11.506371772622,36.2700325870075));
#44069=CARTESIAN_POINT('Ctrl Pts',(20.5171405020204,11.5129424204164,36.2397880590791));
#44070=CARTESIAN_POINT('Ctrl Pts',(20.4403054803013,11.5183798367697,36.2201194327732));
#44071=CARTESIAN_POINT('Ctrl Pts',(20.2567175885002,11.531469603815,36.1849973082169));
#44072=CARTESIAN_POINT('Ctrl Pts',(20.1494436223446,11.5392001587137,36.173655483205));
#44073=CARTESIAN_POINT('Ctrl Pts',(19.9578619823083,11.552820216672,36.1695040233845));
#44074=CARTESIAN_POINT('Ctrl Pts',(19.8738904718882,11.5587216026732,36.1731657563484));
#44075=CARTESIAN_POINT('Ctrl Pts',(19.7811148404891,11.5649943093235,36.1833050885303));
#44076=CARTESIAN_POINT('Ctrl Pts',(19.7718212357972,11.5656198405102,36.1843892470191));
#44077=CARTESIAN_POINT('Ctrl Pts',(19.7580269053695,11.5665437450826,36.1861002586328));
#44078=CARTESIAN_POINT('Ctrl Pts',(19.7535200832844,11.5668448746368,36.1866754456614));
#44079=CARTESIAN_POINT('Ctrl Pts',(19.7454852185212,11.5673803923078,36.1877297631371));
#44080=CARTESIAN_POINT('Ctrl Pts',(19.7419564392349,11.5676151174222,36.1882027423781));
#44081=CARTESIAN_POINT('Ctrl Pts',(19.7343312590901,11.5681213104353,36.1892462790511));
#44082=CARTESIAN_POINT('Ctrl Pts',(19.7302353866208,11.5683925856111,36.1898202398257));
#44083=CARTESIAN_POINT('Ctrl Pts',(19.7188178772814,11.5691471132607,36.1914576486214));
#44084=CARTESIAN_POINT('Ctrl Pts',(19.7115003684001,11.569628775475,36.1925500635598));
#44085=CARTESIAN_POINT('Ctrl Pts',(19.6691190976066,11.5724082772486,36.1991265399423));
#44086=CARTESIAN_POINT('Ctrl Pts',(19.6342031353967,11.5746577973772,36.2055356632801));
#44087=CARTESIAN_POINT('Ctrl Pts',(19.5300497104521,11.5813000772639,36.2276412771628));
#44088=CARTESIAN_POINT('Ctrl Pts',(19.4614862629894,11.5855827213597,36.2461977505825));
#44089=CARTESIAN_POINT('Ctrl Pts',(19.3941040036879,11.589834535998,36.2684889848672));
#44090=CARTESIAN_POINT('Origin',(20.,-1.3495818343519,38.1));
#44091=CARTESIAN_POINT('',(19.394104060634,12.5529621656639,36.2684889660284));
#44092=CARTESIAN_POINT('',(19.3941040087481,12.3811612414289,36.2684889831931));
#44093=CARTESIAN_POINT('',(19.3941040087494,-1.3495818343519,36.2684889831927));
#44094=CARTESIAN_POINT('Ctrl Pts',(19.394104060634,12.5529621656639,36.2684889660284));
#44095=CARTESIAN_POINT('Ctrl Pts',(19.424631338161,12.551017496247,36.2583900077636));
#44096=CARTESIAN_POINT('Ctrl Pts',(19.4554190886317,12.5490873835358,36.2490516417566));
#44097=CARTESIAN_POINT('Ctrl Pts',(19.5665534787306,12.5421885724538,36.2183585513128));
#44098=CARTESIAN_POINT('Ctrl Pts',(19.6480132246812,12.5372541669735,36.2014333502371));
#44099=CARTESIAN_POINT('Ctrl Pts',(19.8084588065227,12.5274358374843,36.1787806489044));
#44100=CARTESIAN_POINT('Ctrl Pts',(19.8872045077698,12.5225712982824,36.1725543251561));
#44101=CARTESIAN_POINT('Ctrl Pts',(19.9852778237007,12.5163363490775,36.1708308646105));
#44102=CARTESIAN_POINT('Ctrl Pts',(20.0044547571054,12.515109068506,36.1707798444788));
#44103=CARTESIAN_POINT('Ctrl Pts',(20.0322314693566,12.5133183574325,36.1711200899231));
#44104=CARTESIAN_POINT('Ctrl Pts',(20.0408332899999,12.5127620016514,36.1712830136058));
#44105=CARTESIAN_POINT('Ctrl Pts',(20.0558765706518,12.511785728515,36.1716686216731));
#44106=CARTESIAN_POINT('Ctrl Pts',(20.0623185870952,12.5113666009464,36.1718660607175));
#44107=CARTESIAN_POINT('Ctrl Pts',(20.0748020570529,12.5105523099961,36.1723112883656));
#44108=CARTESIAN_POINT('Ctrl Pts',(20.0808435802147,12.5101572717702,36.1725552067973));
#44109=CARTESIAN_POINT('Ctrl Pts',(20.0952505265848,12.5092129238402,36.1732047232552));
#44110=CARTESIAN_POINT('Ctrl Pts',(20.1036145949129,12.5086628095685,36.1736364015874));
#44111=CARTESIAN_POINT('Ctrl Pts',(20.1336354991816,12.5066814388033,36.175381894291));
#44112=CARTESIAN_POINT('Ctrl Pts',(20.1552719492921,12.5052405855515,36.177006537645));
#44113=CARTESIAN_POINT('Ctrl Pts',(20.3297576347557,12.4935125285578,36.1930722345579));
#44114=CARTESIAN_POINT('Ctrl Pts',(20.4803839460583,12.4826488744393,36.2253462457159));
#44115=CARTESIAN_POINT('Ctrl Pts',(20.702145777582,12.4659208925764,36.3013648582102));
#44116=CARTESIAN_POINT('Ctrl Pts',(20.7770073281302,12.4601495456332,36.3324145462756));
#44117=CARTESIAN_POINT('Ctrl Pts',(20.8816024639393,12.4520781759104,36.3837300966564));
#44118=CARTESIAN_POINT('Ctrl Pts',(20.9130687655454,12.4496495599521,36.4002614586026));
#44119=CARTESIAN_POINT('Ctrl Pts',(20.9505170415081,12.4467741367281,36.421275875092));
#44120=CARTESIAN_POINT('Ctrl Pts',(20.9569506217065,12.4462806879936,36.4249349726863));
#44121=CARTESIAN_POINT('Ctrl Pts',(20.9669468588086,12.445515030065,36.430696720405));
#44122=CARTESIAN_POINT('Ctrl Pts',(20.9705239955341,12.4452412503049,36.4327739079785));
#44123=CARTESIAN_POINT('Ctrl Pts',(20.9771675520344,12.4447332094362,36.4366603450079));
#44124=CARTESIAN_POINT('Ctrl Pts',(20.9802356154347,12.4444987672265,36.4384665603212));
#44125=CARTESIAN_POINT('Ctrl Pts',(20.9872068410248,12.4439664534437,36.442596656203));
#44126=CARTESIAN_POINT('Ctrl Pts',(20.9911068007277,12.443668927838,36.4449258319974));
#44127=CARTESIAN_POINT('Ctrl Pts',(21.0030106518199,12.4427615028905,36.4520923418715));
#44128=CARTESIAN_POINT('Ctrl Pts',(21.0109877718324,12.4421544005366,36.456974208624));
#44129=CARTESIAN_POINT('Ctrl Pts',(21.0877462134587,12.436319082453,36.5047198235209));
#44130=CARTESIAN_POINT('Ctrl Pts',(21.1538068961394,12.4313457027217,36.5518256552691));
#44131=CARTESIAN_POINT('Ctrl Pts',(21.3438935628083,12.416561067179,36.7063174952605));
#44132=CARTESIAN_POINT('Ctrl Pts',(21.4573750412662,12.4070019722847,36.825457705512));
#44133=CARTESIAN_POINT('Ctrl Pts',(21.577691585422,12.394320804484,36.9891560058173));
#44134=CARTESIAN_POINT('Ctrl Pts',(21.5999784543272,12.3918377277858,37.0215039523279));
#44135=CARTESIAN_POINT('Ctrl Pts',(21.6273852690981,12.3885923077777,37.0640041391241));
#44136=CARTESIAN_POINT('Ctrl Pts',(21.6334254258537,12.3878641548137,37.0735538946565));
#44137=CARTESIAN_POINT('Ctrl Pts',(21.6430680354153,12.3866802813498,37.0890999500792));
#44138=CARTESIAN_POINT('Ctrl Pts',(21.6467224401222,12.3862264657556,37.0950638413322));
#44139=CARTESIAN_POINT('Ctrl Pts',(21.6536608945825,12.3853548164983,37.1065266863398));
#44140=CARTESIAN_POINT('Ctrl Pts',(21.6569501559026,12.3849371793809,37.112022389714));
#44141=CARTESIAN_POINT('Ctrl Pts',(21.6643847076799,12.3839830010491,37.1245856089187));
#44142=CARTESIAN_POINT('Ctrl Pts',(21.6685124395976,12.3834458365236,37.1316633204786));
#44143=CARTESIAN_POINT('Ctrl Pts',(21.6792944984959,12.3820228462614,37.1504246584588));
#44144=CARTESIAN_POINT('Ctrl Pts',(21.6858718835424,12.3811342989299,37.1621517613509));
#44145=CARTESIAN_POINT('Ctrl Pts',(21.7352662021658,12.3743007321268,37.2524179093656));
#44146=CARTESIAN_POINT('Ctrl Pts',(21.772690111719,12.3681675404258,37.3337691212933));
#44147=CARTESIAN_POINT('Ctrl Pts',(21.8616425961561,12.3505340907464,37.5689035611052));
#44148=CARTESIAN_POINT('Ctrl Pts',(21.8996427433279,12.3387365851242,37.7269976866177));
#44149=CARTESIAN_POINT('Ctrl Pts',(21.9207579090756,12.3254897360622,37.9179526754323));
#44150=CARTESIAN_POINT('Ctrl Pts',(21.9233694676922,12.3234360176934,37.9480055451786));
#44151=CARTESIAN_POINT('Ctrl Pts',(21.9257203854433,12.3209464510019,37.9851385084746));
#44152=CARTESIAN_POINT('Ctrl Pts',(21.9261269214358,12.3204771289205,37.9921702664075));
#44153=CARTESIAN_POINT('Ctrl Pts',(21.9267069659523,12.3197406974457,38.0032565727329));
#44154=CARTESIAN_POINT('Ctrl Pts',(21.9269062038707,12.3194722025434,38.0073096250532));
#44155=CARTESIAN_POINT('Ctrl Pts',(21.9272567947968,12.3189686828517,38.0149319910307));
#44156=CARTESIAN_POINT('Ctrl Pts',(21.9274110203678,12.3187335088595,38.0185010548979));
#44157=CARTESIAN_POINT('Ctrl Pts',(21.9277406042984,12.3181976723973,38.0266531950203));
#44158=CARTESIAN_POINT('Ctrl Pts',(21.9279095338035,12.3178973692364,38.0312364791351));
#44159=CARTESIAN_POINT('Ctrl Pts',(21.9283143127749,12.3171030412837,38.0433967101393));
#44160=CARTESIAN_POINT('Ctrl Pts',(21.9285218529068,12.3166105385146,38.0509746114753));
#44161=CARTESIAN_POINT('Ctrl Pts',(21.9296729381394,12.3131456484107,38.1045398260795));
#44162=CARTESIAN_POINT('Ctrl Pts',(21.9290162370414,12.3102548198355,38.1505509409755));
#44163=CARTESIAN_POINT('Ctrl Pts',(21.9252342300737,12.3055870741923,38.2260634270872));
#44164=CARTESIAN_POINT('Ctrl Pts',(21.9230731362518,12.3037811699448,38.2555913479382));
#44165=CARTESIAN_POINT('Ctrl Pts',(21.9042523260376,12.2919000832757,38.4508824543671));
#44166=CARTESIAN_POINT('Ctrl Pts',(21.866861624304,12.2822124796613,38.6139298674188));
#44167=CARTESIAN_POINT('Ctrl Pts',(21.7941029216956,12.2691751064047,38.8103334752139));
#44168=CARTESIAN_POINT('Ctrl Pts',(21.7778826180906,12.2664709839502,38.8500079340842));
#44169=CARTESIAN_POINT('Ctrl Pts',(21.7555947259018,12.2629759307675,38.8997281957132));
#44170=CARTESIAN_POINT('Ctrl Pts',(21.7507377820153,12.2622261684407,38.9103056445679));
#44171=CARTESIAN_POINT('Ctrl Pts',(21.7427774143578,12.2610157491995,38.9272360123358));
#44172=CARTESIAN_POINT('Ctrl Pts',(21.7397342130453,12.2605571593158,38.9336170594816));
#44173=CARTESIAN_POINT('Ctrl Pts',(21.7338754899577,12.2596820209802,38.9457299344488));
#44174=CARTESIAN_POINT('Ctrl Pts',(21.7310664413949,12.2592657004296,38.9514648028758));
#44175=CARTESIAN_POINT('Ctrl Pts',(21.7245923831517,12.2583135462291,38.964517583625));
#44176=CARTESIAN_POINT('Ctrl Pts',(21.7209091937215,12.257777087019,38.9718262922799));
#44177=CARTESIAN_POINT('Ctrl Pts',(21.7112011893108,12.2563764488287,38.9907890659834));
#44178=CARTESIAN_POINT('Ctrl Pts',(21.7051038835884,12.2555097527991,39.002405342494));
#44179=CARTESIAN_POINT('Ctrl Pts',(21.6618192074786,12.2494448471855,39.0828639892144));
#44180=CARTESIAN_POINT('Ctrl Pts',(21.6205969476849,12.2441041267393,39.1494414574469));
#44181=CARTESIAN_POINT('Ctrl Pts',(21.4799957146038,12.2271105442328,39.3484043153222));
#44182=CARTESIAN_POINT('Ctrl Pts',(21.367576077139,12.2150640152101,39.4706310059811));
#44183=CARTESIAN_POINT('Ctrl Pts',(21.212104380237,12.200971364667,39.6012545720403));
#44184=CARTESIAN_POINT('Ctrl Pts',(21.1825489529847,12.1983925303452,39.6246444685866));
#44185=CARTESIAN_POINT('Ctrl Pts',(21.1462890874629,12.1953642966231,39.6516509038929));
#44186=CARTESIAN_POINT('Ctrl Pts',(21.140226776087,12.1948624165314,39.6561112117293));
#44187=CARTESIAN_POINT('Ctrl Pts',(21.1307702960272,12.1940865650379,39.6629838228121));
#44188=CARTESIAN_POINT('Ctrl Pts',(21.1273942414321,12.1938109561178,39.6654207478978));
#44189=CARTESIAN_POINT('Ctrl Pts',(21.1211191375286,12.1933012681254,39.6699194537262));
#44190=CARTESIAN_POINT('Ctrl Pts',(21.1182222997528,12.1930669971097,39.6719841285469));
#44191=CARTESIAN_POINT('Ctrl Pts',(21.1116439439237,12.1925372908182,39.6766453607336));
#44192=CARTESIAN_POINT('Ctrl Pts',(21.1079590384875,12.1922421877734,39.6792370378244));
#44193=CARTESIAN_POINT('Ctrl Pts',(21.0967517777663,12.1913494385396,39.6870608224347));
#44194=CARTESIAN_POINT('Ctrl Pts',(21.0892010597726,12.1907544591513,39.6922523592626));
#44195=CARTESIAN_POINT('Ctrl Pts',(20.990916712871,12.1830895996628,39.7588019625556));
#44196=CARTESIAN_POINT('Ctrl Pts',(20.8951394698338,12.1764895350745,39.812388002061));
#44197=CARTESIAN_POINT('Ctrl Pts',(20.7191759435041,12.1649334108905,39.8920137364516));
#44198=CARTESIAN_POINT('Ctrl Pts',(20.6408764782058,12.1599715022992,39.9214840577016));
#44199=CARTESIAN_POINT('Ctrl Pts',(20.4860365610512,12.1501621750001,39.9685383608472));
#44200=CARTESIAN_POINT('Ctrl Pts',(20.4098507259706,12.1453368952395,39.9867133857815));
#44201=CARTESIAN_POINT('Ctrl Pts',(20.3139728939988,12.1391491484393,40.0035041472148));
#44202=CARTESIAN_POINT('Ctrl Pts',(20.2951209627249,12.1379272745513,40.0065179234554));
#44203=CARTESIAN_POINT('Ctrl Pts',(20.2677285412972,12.1361430311735,40.0104810223676));
#44204=CARTESIAN_POINT('Ctrl Pts',(20.2592211495001,12.1355876639642,40.0116539175246));
#44205=CARTESIAN_POINT('Ctrl Pts',(20.244318346252,12.1346125371526,40.0136072245455));
#44206=CARTESIAN_POINT('Ctrl Pts',(20.2379262823542,12.1341935616724,40.0144124807987));
#44207=CARTESIAN_POINT('Ctrl Pts',(20.2255232667001,12.133379132015,40.0159119044806));
#44208=CARTESIAN_POINT('Ctrl Pts',(20.2195128395581,12.1329838009568,40.0166098406884));
#44209=CARTESIAN_POINT('Ctrl Pts',(20.2051589223262,12.1320380549513,40.0182082258476));
#44210=CARTESIAN_POINT('Ctrl Pts',(20.1968127013243,12.1314868299798,40.0190825250524));
#44211=CARTESIAN_POINT('Ctrl Pts',(20.1667635619287,12.1294973588631,40.0220322039629));
#44212=CARTESIAN_POINT('Ctrl Pts',(20.1450322157591,12.1280494132623,40.0237940298105));
#44213=CARTESIAN_POINT('Ctrl Pts',(19.9718174261623,12.1164308465449,40.0348855735713));
#44214=CARTESIAN_POINT('Ctrl Pts',(19.8197714495793,12.1056984985874,40.0266749919094));
#44215=CARTESIAN_POINT('Ctrl Pts',(19.5892858667585,12.0890059960846,39.9866944539443));
#44216=CARTESIAN_POINT('Ctrl Pts',(19.5092553432328,12.083142117305,39.9674778246224));
#44217=CARTESIAN_POINT('Ctrl Pts',(19.3964378589307,12.0749597469714,39.9326321262008));
#44218=CARTESIAN_POINT('Ctrl Pts',(19.3624834579184,12.0725090947382,39.9210987975881));
#44219=CARTESIAN_POINT('Ctrl Pts',(19.3219111637762,12.0696111949304,39.9060435057152));
#44220=CARTESIAN_POINT('Ctrl Pts',(19.3149694069985,12.0691164692555,39.9034219432513));
#44221=CARTESIAN_POINT('Ctrl Pts',(19.3041777697033,12.0683492667924,39.8992751665651));
#44222=CARTESIAN_POINT('Ctrl Pts',(19.3003174740358,12.0680752093743,39.8977775348618));
#44223=CARTESIAN_POINT('Ctrl Pts',(19.2931473423426,12.067566920968,39.89496923359));
#44224=CARTESIAN_POINT('Ctrl Pts',(19.2898363431304,12.0673325072271,39.8936618438148));
#44225=CARTESIAN_POINT('Ctrl Pts',(19.2823139189638,12.0668006005164,39.8906674250551));
#44226=CARTESIAN_POINT('Ctrl Pts',(19.2781048208173,12.0665034513812,39.8889747033924));
#44227=CARTESIAN_POINT('Ctrl Pts',(19.2652647225308,12.0655983157268,39.8837582622424));
#44228=CARTESIAN_POINT('Ctrl Pts',(19.2566531029044,12.0649931056814,39.8801867500672));
#44229=CARTESIAN_POINT('Ctrl Pts',(19.1744167535828,12.0592282961597,39.8453799145038));
#44230=CARTESIAN_POINT('Ctrl Pts',(19.1027656157187,12.0543168698859,39.809652764802));
#44231=CARTESIAN_POINT('Ctrl Pts',(18.8911396409166,12.0395505057245,39.687148659267));
#44232=CARTESIAN_POINT('Ctrl Pts',(18.7598851654615,12.0299589513158,39.5868513144517));
#44233=CARTESIAN_POINT('Ctrl Pts',(18.6147535238725,12.0172169038948,39.4432082857444));
#44234=CARTESIAN_POINT('Ctrl Pts',(18.5874272912644,12.0147093882261,39.4144406765749));
#44235=CARTESIAN_POINT('Ctrl Pts',(18.5534568132957,12.0114363070004,39.376394896038));
#44236=CARTESIAN_POINT('Ctrl Pts',(18.5459798219425,12.0107056696838,39.3678708272194));
#44237=CARTESIAN_POINT('Ctrl Pts',(18.5340070934943,12.0095187452775,39.3539762353205));
#44238=CARTESIAN_POINT('Ctrl Pts',(18.5294646242508,12.0090643814645,39.3486461897602));
#44239=CARTESIAN_POINT('Ctrl Pts',(18.5208250585105,12.0081923477016,39.3383961566038));
#44240=CARTESIAN_POINT('Ctrl Pts',(18.5167232286311,12.0077748779611,39.3334802657873));
#44241=CARTESIAN_POINT('Ctrl Pts',(18.5074390774839,12.0068220087002,39.3222402789538));
#44242=CARTESIAN_POINT('Ctrl Pts',(18.5022723654489,12.006285991922,39.3159035061034));
#44243=CARTESIAN_POINT('Ctrl Pts',(18.4887526199817,12.0048680334814,39.2991051368935));
#44244=CARTESIAN_POINT('Ctrl Pts',(18.4804680514826,12.0039834010131,39.2885892541526));
#44245=CARTESIAN_POINT('Ctrl Pts',(18.4190115001122,11.9972999632436,39.2088876454116));
#44246=CARTESIAN_POINT('Ctrl Pts',(18.3704866374972,11.9913224552735,39.1362619048918));
#44247=CARTESIAN_POINT('Ctrl Pts',(18.3082514153552,11.9825650176364,39.0278761574961));
#44248=CARTESIAN_POINT('Ctrl Pts',(18.2904205048242,11.9798977569822,38.9945977826753));
#44249=CARTESIAN_POINT('Ctrl Pts',(18.2357998863346,11.9712044731663,38.8850529727456));
#44250=CARTESIAN_POINT('Ctrl Pts',(18.2030506959797,11.9651292595463,38.806882888797));
#44251=CARTESIAN_POINT('Ctrl Pts',(18.155094989453,11.9546934980988,38.667299070028));
#44252=CARTESIAN_POINT('Ctrl Pts',(18.1375699479435,11.9503006437687,38.6068122693153));
#44253=CARTESIAN_POINT('Ctrl Pts',(18.1200789722994,11.9451826545723,38.5331315641721));
#44254=CARTESIAN_POINT('Ctrl Pts',(18.1172495789451,11.9443244667038,38.5206624487318));
#44255=CARTESIAN_POINT('Ctrl Pts',(18.1134533078516,11.9431295122151,38.5031261866552));
#44256=CARTESIAN_POINT('Ctrl Pts',(18.1123825367493,11.9427871925066,38.4980822251391));
#44257=CARTESIAN_POINT('Ctrl Pts',(18.1105884941989,11.9422045424815,38.4894612123815));
#44258=CARTESIAN_POINT('Ctrl Pts',(18.1098551299822,11.9419636470719,38.4858863115054));
#44259=CARTESIAN_POINT('Ctrl Pts',(18.108463089275,11.941501104647,38.4790014006423));
#44260=CARTESIAN_POINT('Ctrl Pts',(18.1078029519872,11.9412793727008,38.4756917330097));
#44261=CARTESIAN_POINT('Ctrl Pts',(18.1060625213008,11.9406882894039,38.4668449399428));
#44262=CARTESIAN_POINT('Ctrl Pts',(18.1049978152948,11.9403198121827,38.4613047261026));
#44263=CARTESIAN_POINT('Ctrl Pts',(18.1012253161049,11.9389884210131,38.44119897386));
#44264=CARTESIAN_POINT('Ctrl Pts',(18.0986609428953,11.9380332064153,38.4266065861845));
#44265=CARTESIAN_POINT('Ctrl Pts',(18.0794575725492,11.9304408543882,38.3094276702888));
#44266=CARTESIAN_POINT('Ctrl Pts',(18.0709629304851,11.9241914034759,38.205664609979));
#44267=CARTESIAN_POINT('Ctrl Pts',(18.0707334764535,11.9087151054445,37.9468805119815));
#44268=CARTESIAN_POINT('Ctrl Pts',(18.0892346249004,11.8995431730862,37.7926169603208));
#44269=CARTESIAN_POINT('Ctrl Pts',(18.1310982777059,11.8883624079805,37.6212349761986));
#44270=CARTESIAN_POINT('Ctrl Pts',(18.136578699205,11.8869823470234,37.6003295168955));
#44271=CARTESIAN_POINT('Ctrl Pts',(18.1446649327772,11.8850527593879,37.5714697164514));
#44272=CARTESIAN_POINT('Ctrl Pts',(18.1469731684293,11.8845127800516,37.5634331074577));
#44273=CARTESIAN_POINT('Ctrl Pts',(18.1510394411321,11.8835796482179,37.5496147483513));
#44274=CARTESIAN_POINT('Ctrl Pts',(18.152772546919,11.8831873049853,37.5438257389201));
#44275=CARTESIAN_POINT('Ctrl Pts',(18.1564108489232,11.8823745421807,37.531877509525));
#44276=CARTESIAN_POINT('Ctrl Pts',(18.1583197770217,11.8819540057961,37.5257195138662));
#44277=CARTESIAN_POINT('Ctrl Pts',(18.1628519291694,11.8809690792889,37.5113542985195));
#44278=CARTESIAN_POINT('Ctrl Pts',(18.1654993248703,11.880403907923,37.5031549071008));
#44279=CARTESIAN_POINT('Ctrl Pts',(18.174238092862,11.8785703462414,37.4766971147556));
#44280=CARTESIAN_POINT('Ctrl Pts',(18.1805476571886,11.877294856603,37.4585125448242));
#44281=CARTESIAN_POINT('Ctrl Pts',(18.2143033974603,11.8707063114775,37.365733218681));
#44282=CARTESIAN_POINT('Ctrl Pts',(18.2460652388906,11.8652521565718,37.2928011453625));
#44283=CARTESIAN_POINT('Ctrl Pts',(18.3315283322058,11.8520997518482,37.1255879821471));
#44284=CARTESIAN_POINT('Ctrl Pts',(18.3888615229535,11.8443219046793,37.0334604316663));
#44285=CARTESIAN_POINT('Ctrl Pts',(18.5032681451682,11.8307241373128,36.8800683813324));
#44286=CARTESIAN_POINT('Ctrl Pts',(18.5571726610135,11.8248889240047,36.816764996132));
#44287=CARTESIAN_POINT('Ctrl Pts',(18.6215046106875,11.8186775026742,36.7504147181015));
#44288=CARTESIAN_POINT('Ctrl Pts',(18.6280617511577,11.8180524245044,36.7437494989938));
#44289=CARTESIAN_POINT('Ctrl Pts',(18.63787602175,11.8171290566407,36.7339174788928));
#44290=CARTESIAN_POINT('Ctrl Pts',(18.6410961763068,11.8168280153476,36.730714206019));
#44291=CARTESIAN_POINT('Ctrl Pts',(18.6468605696159,11.8162925928854,36.7250203950593));
#44292=CARTESIAN_POINT('Ctrl Pts',(18.6494004113494,11.8160578752119,36.7225255051657));
#44293=CARTESIAN_POINT('Ctrl Pts',(18.6549063698593,11.8155516281636,36.7171468639056));
#44294=CARTESIAN_POINT('Ctrl Pts',(18.6578748532003,11.8152802918852,36.7142656239474));
#44295=CARTESIAN_POINT('Ctrl Pts',(18.6661811527464,11.8145254236098,36.7062551741298));
#44296=CARTESIAN_POINT('Ctrl Pts',(18.6715393290097,11.8140434841966,36.701147038862));
#44297=CARTESIAN_POINT('Ctrl Pts',(18.7028063959762,11.8112591248584,36.6716807484468));
#44298=CARTESIAN_POINT('Ctrl Pts',(18.7293573469193,11.8090052219865,36.6480100663089));
#44299=CARTESIAN_POINT('Ctrl Pts',(18.8185245643896,11.801730028319,36.5728362179607));
#44300=CARTESIAN_POINT('Ctrl Pts',(18.8837366080479,11.7968621923528,36.5245408099081));
#44301=CARTESIAN_POINT('Ctrl Pts',(19.0805520101866,11.7828443763861,36.3971553927843));
#44302=CARTESIAN_POINT('Ctrl Pts',(19.2187658255787,11.7737523780295,36.329482769854));
#44303=CARTESIAN_POINT('Ctrl Pts',(19.3736905474639,11.7633525661543,36.2753370339213));
#44304=CARTESIAN_POINT('Ctrl Pts',(19.3838832094158,11.7626677251025,36.2718702030071));
#44305=CARTESIAN_POINT('Ctrl Pts',(19.3941040090521,11.7619801941421,36.2684889830926));
#44306=CARTESIAN_POINT('',(18.070870558151,11.7455906108586,38.0995325677651));
#44307=CARTESIAN_POINT('Ctrl Pts',(19.3941040036879,11.589834535998,36.2684889848672));
#44308=CARTESIAN_POINT('Ctrl Pts',(19.3847992552261,11.5904216648079,36.2715671590049));
#44309=CARTESIAN_POINT('Ctrl Pts',(19.3755170286381,11.591008177693,36.2747165499176));
#44310=CARTESIAN_POINT('Ctrl Pts',(19.2210205634771,11.600789172277,36.3284528217096));
#44311=CARTESIAN_POINT('Ctrl Pts',(19.0823620386687,11.6099032911439,36.3961447601399));
#44312=CARTESIAN_POINT('Ctrl Pts',(18.9350060058248,11.6210204272785,36.4913358843555));
#44313=CARTESIAN_POINT('Ctrl Pts',(18.9169980559991,11.6224046295,36.5034038789726));
#44314=CARTESIAN_POINT('Ctrl Pts',(18.8923230790278,11.6243390550331,36.5205493116066));
#44315=CARTESIAN_POINT('Ctrl Pts',(18.8854795765921,11.624879666536,36.5253708815999));
#44316=CARTESIAN_POINT('Ctrl Pts',(18.8737484620666,11.625813596965,36.5337507931408));
#44317=CARTESIAN_POINT('Ctrl Pts',(18.8688457559863,11.6262061033816,36.5372878769412));
#44318=CARTESIAN_POINT('Ctrl Pts',(18.8589297763901,11.6270044827186,36.5445129267101));
#44319=CARTESIAN_POINT('Ctrl Pts',(18.8539175653154,11.6274104036865,36.5482022226558));
#44320=CARTESIAN_POINT('Ctrl Pts',(18.8422591153987,11.6283601725191,36.5568708522089));
#44321=CARTESIAN_POINT('Ctrl Pts',(18.8356270435076,11.6289047434328,36.5618689466772));
#44322=CARTESIAN_POINT('Ctrl Pts',(18.8217370010024,11.6300544300048,36.572478143461));
#44323=CARTESIAN_POINT('Ctrl Pts',(18.8144863884877,11.6306598997217,36.5780984956274));
#44324=CARTESIAN_POINT('Ctrl Pts',(18.7952251635713,11.6322827884831,36.5932501049463));
#44325=CARTESIAN_POINT('Ctrl Pts',(18.7832878346289,11.6333038008267,36.6028730392944));
#44326=CARTESIAN_POINT('Ctrl Pts',(18.6883532289436,11.6415483802967,36.6812871987918));
#44327=CARTESIAN_POINT('Ctrl Pts',(18.6111536768575,11.6490443489946,36.756771672466));
#44328=CARTESIAN_POINT('Ctrl Pts',(18.455126308962,11.6659612014356,36.9372380237683));
#44329=CARTESIAN_POINT('Ctrl Pts',(18.379865355166,11.6754146641219,37.044625346559));
#44330=CARTESIAN_POINT('Ctrl Pts',(18.3010323377094,11.6865679109604,37.1856703429942));
#44331=CARTESIAN_POINT('Ctrl Pts',(18.2866602305069,11.6886659176534,37.2128940670595));
#44332=CARTESIAN_POINT('Ctrl Pts',(18.2696696300476,11.6912195433938,37.2470325912097));
#44333=CARTESIAN_POINT('Ctrl Pts',(18.2664320088598,11.6917096828299,37.2536321048101));
#44334=CARTESIAN_POINT('Ctrl Pts',(18.2614170613492,11.6924743119621,37.2640040020269));
#44335=CARTESIAN_POINT('Ctrl Pts',(18.2596141512818,11.692750328012,37.2677638306387));
#44336=CARTESIAN_POINT('Ctrl Pts',(18.2562959571921,11.6932603869921,37.2747416049217));
#44337=CARTESIAN_POINT('Ctrl Pts',(18.2547773944911,11.6934946242704,37.277957869008));
#44338=CARTESIAN_POINT('Ctrl Pts',(18.2513589976422,11.6940237706861,37.2852500852844));
#44339=CARTESIAN_POINT('Ctrl Pts',(18.2494645183888,11.6943183505608,37.2893284837318));
#44340=CARTESIAN_POINT('Ctrl Pts',(18.2437701394599,11.6952079500471,37.3017002743868));
#44341=CARTESIAN_POINT('Ctrl Pts',(18.2400147212215,11.6958003303856,37.3100141764609));
#44342=CARTESIAN_POINT('Ctrl Pts',(18.1930086331833,11.7032925200229,37.4160773300174));
#44343=CARTESIAN_POINT('Ctrl Pts',(18.157888858645,11.7097447425299,37.5172465445072));
#44344=CARTESIAN_POINT('Ctrl Pts',(18.0912163094748,11.7258131373009,37.7772502200088));
#44345=CARTESIAN_POINT('Ctrl Pts',(18.0709092920218,11.7353493249005,37.9380723583049));
#44346=CARTESIAN_POINT('Ctrl Pts',(18.0708700569582,11.7455896548511,38.099531214715));
#44347=CARTESIAN_POINT('Ctrl Pts',(18.0708700566166,11.7455897441458,38.0995326226208));
#44348=CARTESIAN_POINT('Ctrl Pts',(18.0708667520166,11.7464548413653,38.11317256992));
#44349=CARTESIAN_POINT('Ctrl Pts',(18.0710081096649,11.7473241274613,38.1268119579521));
#44350=CARTESIAN_POINT('Ctrl Pts',(18.0715353871247,11.7489349523901,38.1519541277993));
#44351=CARTESIAN_POINT('Ctrl Pts',(18.0718796265132,11.7496751891478,38.1634571554648));
#44352=CARTESIAN_POINT('Ctrl Pts',(18.0725689054531,11.7508212029005,38.181183564671));
#44353=CARTESIAN_POINT('Ctrl Pts',(18.0728412238664,11.7512247262145,38.1874096417373));
#44354=CARTESIAN_POINT('Ctrl Pts',(18.0734409464895,11.7520266431385,38.1997510611974));
#44355=CARTESIAN_POINT('Ctrl Pts',(18.0737673119516,11.7524249999186,38.2058663824237));
#44356=CARTESIAN_POINT('Ctrl Pts',(18.074525013846,11.753276039888,38.2188976466794));
#44357=CARTESIAN_POINT('Ctrl Pts',(18.0749645050548,11.7537289712671,38.2258130112067));
#44358=CARTESIAN_POINT('Ctrl Pts',(18.0761983387331,11.7549042164061,38.243703924058));
#44359=CARTESIAN_POINT('Ctrl Pts',(18.0770493435745,11.7556282825458,38.2546751892176));
#44360=CARTESIAN_POINT('Ctrl Pts',(18.0808285555749,11.7585362761984,38.2985277515414));
#44361=CARTESIAN_POINT('Ctrl Pts',(18.0845065341355,11.7607433321031,38.3313371052114));
#44362=CARTESIAN_POINT('Ctrl Pts',(18.1139570869446,11.7752962467233,38.544488538909));
#44363=CARTESIAN_POINT('Ctrl Pts',(18.1643236778433,11.7884429296676,38.7204796349323));
#44364=CARTESIAN_POINT('Ctrl Pts',(18.2648771594039,11.8058883528737,38.9456042813956));
#44365=CARTESIAN_POINT('Ctrl Pts',(18.2941027201047,11.810392163972,39.0031135480106));
#44366=CARTESIAN_POINT('Ctrl Pts',(18.3325911986786,11.8156256440845,39.0702875809741));
#44367=CARTESIAN_POINT('Ctrl Pts',(18.3391392588077,11.8164946155136,39.081453881314));
#44368=CARTESIAN_POINT('Ctrl Pts',(18.3484654887304,11.8177019154218,39.0969970740262));
#44369=CARTESIAN_POINT('Ctrl Pts',(18.3511494779868,11.8180459483263,39.1014296605992));
#44370=CARTESIAN_POINT('Ctrl Pts',(18.3557565683414,11.8186306278153,39.1089694973281));
#44371=CARTESIAN_POINT('Ctrl Pts',(18.3576706862402,11.818871849106,39.1120821780398));
#44372=CARTESIAN_POINT('Ctrl Pts',(18.3613664922593,11.8193343304889,39.1180540915133));
#44373=CARTESIAN_POINT('Ctrl Pts',(18.3631468318724,11.8195556787752,39.1209141062608));
#44374=CARTESIAN_POINT('Ctrl Pts',(18.3679121115936,11.8201443673867,39.1285247489712));
#44375=CARTESIAN_POINT('Ctrl Pts',(18.3709103280634,11.8205108465204,39.1332670891138));
#44376=CARTESIAN_POINT('Ctrl Pts',(18.3817933735479,11.8218273590555,39.1503158985907));
#44377=CARTESIAN_POINT('Ctrl Pts',(18.3897975464905,11.8227699158798,39.1625461225048));
#44378=CARTESIAN_POINT('Ctrl Pts',(18.4645086322899,11.831347574072,39.2739198416129));
#44379=CARTESIAN_POINT('Ctrl Pts',(18.5401634634514,11.8384669156742,39.3667703310375));
#44380=CARTESIAN_POINT('Ctrl Pts',(18.7172904129973,11.8535609628362,39.5470457904174));
#44381=CARTESIAN_POINT('Ctrl Pts',(18.8202228041047,11.8615148637864,39.6321246202758));
#44382=CARTESIAN_POINT('Ctrl Pts',(18.9460385741022,11.8710507719706,39.7158682700098));
#44383=CARTESIAN_POINT('Ctrl Pts',(18.9611234552733,11.8721907190265,39.7256077155327));
#44384=CARTESIAN_POINT('Ctrl Pts',(18.9850143982375,11.873992186421,39.7405643783623));
#44385=CARTESIAN_POINT('Ctrl Pts',(18.9937300119363,11.8746485652307,39.7459246507666));
#44386=CARTESIAN_POINT('Ctrl Pts',(19.0085317430884,11.8757621527334,39.7548664943664));
#44387=CARTESIAN_POINT('Ctrl Pts',(19.0145956982148,11.876218045587,39.7584844824404));
#44388=CARTESIAN_POINT('Ctrl Pts',(19.0265289638169,11.8771146481267,39.7655157750273));
#44389=CARTESIAN_POINT('Ctrl Pts',(19.0323967051017,11.8775552609616,39.7689315494957));
#44390=CARTESIAN_POINT('Ctrl Pts',(19.0436803203662,11.8784021224858,39.7754205450068));
#44391=CARTESIAN_POINT('Ctrl Pts',(19.049093291539,11.8788081890486,39.7784986632611));
#44392=CARTESIAN_POINT('Ctrl Pts',(19.0616646422348,11.8797508713398,39.7855671086773));
#44393=CARTESIAN_POINT('Ctrl Pts',(19.0688336944745,11.8802881657033,39.7895381112748));
#44394=CARTESIAN_POINT('Ctrl Pts',(19.0878366704714,11.8817117281409,39.7999063448686));
#44395=CARTESIAN_POINT('Ctrl Pts',(19.0997124108739,11.8826007213315,39.806225589545));
#44396=CARTESIAN_POINT('Ctrl Pts',(19.1910371336369,11.8894333605902,39.8536018421503));
#44397=CARTESIAN_POINT('Ctrl Pts',(19.2731767869918,11.8955650772468,39.889207690285));
#44398=CARTESIAN_POINT('Ctrl Pts',(19.5101773075653,11.913195221869,39.9729234790555));
#44399=CARTESIAN_POINT('Ctrl Pts',(19.6690481392435,11.9249908537421,40.0074161018928));
#44400=CARTESIAN_POINT('Ctrl Pts',(19.8604279017471,11.93823842866,40.0243112014333));
#44401=CARTESIAN_POINT('Ctrl Pts',(19.8905608729884,11.9402942175166,40.026259924992));
#44402=CARTESIAN_POINT('Ctrl Pts',(19.9277686787684,11.9427859336734,40.027790142086));
#44403=CARTESIAN_POINT('Ctrl Pts',(19.9348098762534,11.9432554018865,40.0280410906511));
#44404=CARTESIAN_POINT('Ctrl Pts',(19.9459089407901,11.9439920101512,40.0283757892356));
#44405=CARTESIAN_POINT('Ctrl Pts',(19.9499658806472,11.9442605368059,40.0284853162138));
#44406=CARTESIAN_POINT('Ctrl Pts',(19.9575945057654,11.9447640816737,40.02866718035));
#44407=CARTESIAN_POINT('Ctrl Pts',(19.9611660047791,11.9449992492878,40.0287423984462));
#44408=CARTESIAN_POINT('Ctrl Pts',(19.9693225404395,11.9455350275714,40.0288915152025));
#44409=CARTESIAN_POINT('Ctrl Pts',(19.9739076425209,11.9458352792141,40.0289589870954));
#44410=CARTESIAN_POINT('Ctrl Pts',(19.9860703682847,11.9466293819463,40.0290945922662));
#44411=CARTESIAN_POINT('Ctrl Pts',(19.9936483195658,11.9471217123832,40.0291344279974));
#44412=CARTESIAN_POINT('Ctrl Pts',(20.0471633339938,11.950582577631,40.0291004054082));
#44413=CARTESIAN_POINT('Ctrl Pts',(20.0930888457495,11.9534697678043,40.0274304139056));
#44414=CARTESIAN_POINT('Ctrl Pts',(20.1684737796634,11.9581361489141,40.0219878828372));
#44415=CARTESIAN_POINT('Ctrl Pts',(20.1979806192835,11.9599441722833,40.0191729046023));
#44416=CARTESIAN_POINT('Ctrl Pts',(20.392773193643,11.9718232889834,39.9960489127812));
#44417=CARTESIAN_POINT('Ctrl Pts',(20.5548892799386,11.9815068646078,39.9550932515951));
#44418=CARTESIAN_POINT('Ctrl Pts',(20.7496614401286,11.9945443683278,39.8780309266109));
#44419=CARTESIAN_POINT('Ctrl Pts',(20.7890470022918,11.9972537473934,39.8609061990242));
#44420=CARTESIAN_POINT('Ctrl Pts',(20.8383463656397,12.000754721376,39.8374848428605));
#44421=CARTESIAN_POINT('Ctrl Pts',(20.848820764612,12.0015049735651,39.8323918459337));
#44422=CARTESIAN_POINT('Ctrl Pts',(20.8655793436303,12.0027159939214,39.8240548018818));
#44423=CARTESIAN_POINT('Ctrl Pts',(20.8718930304937,12.0031746913167,39.8208704486929));
#44424=CARTESIAN_POINT('Ctrl Pts',(20.883874503638,12.0040499101917,39.8147446438005));
#44425=CARTESIAN_POINT('Ctrl Pts',(20.8895454832324,12.0044662030703,39.8118096165303));
#44426=CARTESIAN_POINT('Ctrl Pts',(20.9024487022078,12.0054181190964,39.8050500955126));
#44427=CARTESIAN_POINT('Ctrl Pts',(20.9096713551937,12.0059543666727,39.8012076623364));
#44428=CARTESIAN_POINT('Ctrl Pts',(20.9284027540773,12.0073540943327,39.7910892113087));
#44429=CARTESIAN_POINT('Ctrl Pts',(20.9398722015289,12.0082200861068,39.7847417086385));
#44430=CARTESIAN_POINT('Ctrl Pts',(21.019743907696,12.0143146010229,39.7394690979064));
#44431=CARTESIAN_POINT('Ctrl Pts',(21.0857637819588,12.0196873930672,39.6965120296976));
#44432=CARTESIAN_POINT('Ctrl Pts',(21.2815144847728,12.0366887182697,39.5513749254521));
#44433=CARTESIAN_POINT('Ctrl Pts',(21.4008895230141,12.0487053537516,39.4365142261852));
#44434=CARTESIAN_POINT('Ctrl Pts',(21.5277583354589,12.0627673644305,39.2785219812654));
#44435=CARTESIAN_POINT('Ctrl Pts',(21.5504656490871,12.0653436603892,39.2484843598443));
#44436=CARTESIAN_POINT('Ctrl Pts',(21.576640749079,12.068369318758,39.2116668192777));
#44437=CARTESIAN_POINT('Ctrl Pts',(21.5809646172689,12.0688710605764,39.205508956213));
#44438=CARTESIAN_POINT('Ctrl Pts',(21.5876248467642,12.0696467445179,39.1959047563196));
#44439=CARTESIAN_POINT('Ctrl Pts',(21.5899862075072,12.0699223230541,39.1924759721553));
#44440=CARTESIAN_POINT('Ctrl Pts',(21.5943447108031,12.0704319826447,39.1861031972554));
#44441=CARTESIAN_POINT('Ctrl Pts',(21.59634479308,12.0706662554669,39.1831613517417));
#44442=CARTESIAN_POINT('Ctrl Pts',(21.6008596500037,12.0711960010508,39.1764809509586));
#44443=CARTESIAN_POINT('Ctrl Pts',(21.6033694674206,12.0714911413672,39.172739114952));
#44444=CARTESIAN_POINT('Ctrl Pts',(21.6109452600013,12.0723841178648,39.16135853469));
#44445=CARTESIAN_POINT('Ctrl Pts',(21.6159700153187,12.0729792852458,39.1536923115998));
#44446=CARTESIAN_POINT('Ctrl Pts',(21.6802773058293,12.0806380882972,39.0540372240027));
#44447=CARTESIAN_POINT('Ctrl Pts',(21.7316921262177,12.087232756108,38.9571864849764));
#44448=CARTESIAN_POINT('Ctrl Pts',(21.8073272938944,12.0987734127171,38.7797555959279));
#44449=CARTESIAN_POINT('Ctrl Pts',(21.8350240704192,12.1037254674551,38.7009873949841));
#44450=CARTESIAN_POINT('Ctrl Pts',(21.8787163698481,12.113536726854,38.5451132135908));
#44451=CARTESIAN_POINT('Ctrl Pts',(21.8952644423721,12.118374732858,38.4683361554826));
#44452=CARTESIAN_POINT('Ctrl Pts',(21.9099723956715,12.1245777788818,38.3718704217822));
#44453=CARTESIAN_POINT('Ctrl Pts',(21.9125728642164,12.1258014064445,38.3529289936295));
#44454=CARTESIAN_POINT('Ctrl Pts',(21.9159334081861,12.1275877469895,38.3254230916756));
#44455=CARTESIAN_POINT('Ctrl Pts',(21.9169184856031,12.1281434342293,38.3168868610455));
#44456=CARTESIAN_POINT('Ctrl Pts',(21.9185423681137,12.129118931081,38.3019387430238));
#44457=CARTESIAN_POINT('Ctrl Pts',(21.9192061444247,12.1295379547332,38.2955296594074));
#44458=CARTESIAN_POINT('Ctrl Pts',(21.9204308306483,12.1303523364546,38.2830971784982));
#44459=CARTESIAN_POINT('Ctrl Pts',(21.9209955413117,12.1307475707419,38.2770742243838));
#44460=CARTESIAN_POINT('Ctrl Pts',(21.9222755029665,12.1316928576013,38.2626953595162));
#44461=CARTESIAN_POINT('Ctrl Pts',(21.9229646078136,12.132243718411,38.2543373015887));
#44462=CARTESIAN_POINT('Ctrl Pts',(21.9252462923784,12.1342305308373,38.2242702163021));
#44463=CARTESIAN_POINT('Ctrl Pts',(21.926525863421,12.1356761481378,38.2025397724955));
#44464=CARTESIAN_POINT('Ctrl Pts',(21.933818565484,12.147331889191,38.0285616240693));
#44465=CARTESIAN_POINT('Ctrl Pts',(21.9221410062127,12.1581086987237,37.8761387541007));
#44466=CARTESIAN_POINT('Ctrl Pts',(21.8768431373976,12.1748131355117,37.6464673768813));
#44467=CARTESIAN_POINT('Ctrl Pts',(21.8559287623335,12.1806455460191,37.5673067433111));
#44468=CARTESIAN_POINT('Ctrl Pts',(21.8187435340262,12.1887902004488,37.4558012035432));
#44469=CARTESIAN_POINT('Ctrl Pts',(21.8064948763291,12.1912333889468,37.4222118367068));
#44470=CARTESIAN_POINT('Ctrl Pts',(21.7905864737342,12.1941236772767,37.382088028064));
#44471=CARTESIAN_POINT('Ctrl Pts',(21.7878142554608,12.1946179710928,37.3752119539274));
#44472=CARTESIAN_POINT('Ctrl Pts',(21.783432578722,12.1953846507579,37.3645219739979));
#44473=CARTESIAN_POINT('Ctrl Pts',(21.7818504053442,12.1956586138327,37.3606970692921));
#44474=CARTESIAN_POINT('Ctrl Pts',(21.7788845763381,12.1961668172798,37.3535920054577));
#44475=CARTESIAN_POINT('Ctrl Pts',(21.7775041648888,12.1964012398475,37.3503106147376));
#44476=CARTESIAN_POINT('Ctrl Pts',(21.774343164509,12.1969332817196,37.3428543797382));
#44477=CARTESIAN_POINT('Ctrl Pts',(21.7725569238967,12.1972305564748,37.3386819926555));
#44478=CARTESIAN_POINT('Ctrl Pts',(21.767052833198,12.1981364581636,37.3259496559369));
#44479=CARTESIAN_POINT('Ctrl Pts',(21.7632875121547,12.1987423017599,37.3174101914648));
#44480=CARTESIAN_POINT('Ctrl Pts',(21.726235959192,12.2045749421816,37.2350052037527));
#44481=CARTESIAN_POINT('Ctrl Pts',(21.6883849867663,12.2095469840815,37.1632683371349));
#44482=CARTESIAN_POINT('Ctrl Pts',(21.5606599440557,12.2243323900068,36.9542461766252));
#44483=CARTESIAN_POINT('Ctrl Pts',(21.4577192458435,12.2338930907415,36.8258472871048));
#44484=CARTESIAN_POINT('Ctrl Pts',(21.3115113143279,12.2465773107174,36.6847174203685));
#44485=CARTESIAN_POINT('Ctrl Pts',(21.282412877523,12.2490616396196,36.6582983734788));
#44486=CARTESIAN_POINT('Ctrl Pts',(21.2439340760874,12.2523084760693,36.6254497983625));
#44487=CARTESIAN_POINT('Ctrl Pts',(21.2352744164194,12.2530367556515,36.6181878020119));
#44488=CARTESIAN_POINT('Ctrl Pts',(21.2211525660466,12.254220783788,36.6065550239984));
#44489=CARTESIAN_POINT('Ctrl Pts',(21.2157294472782,12.2546746264976,36.6021370574069));
#44490=CARTESIAN_POINT('Ctrl Pts',(21.2052949967704,12.2555462931071,36.5937305858084));
#44491=CARTESIAN_POINT('Ctrl Pts',(21.2002875857202,12.2559639202724,36.5897373449361));
#44492=CARTESIAN_POINT('Ctrl Pts',(21.1888298787898,12.2569180275994,36.5806931864642));
#44493=CARTESIAN_POINT('Ctrl Pts',(21.1823671412532,12.257455130753,36.5756583013783));
#44494=CARTESIAN_POINT('Ctrl Pts',(21.1652159149453,12.2588778544036,36.5624710960687));
#44495=CARTESIAN_POINT('Ctrl Pts',(21.1544741012035,12.2597661948697,36.5543891844834));
#44496=CARTESIAN_POINT('Ctrl Pts',(21.0717093789921,12.2665914126742,36.493462931605));
#44497=CARTESIAN_POINT('Ctrl Pts',(20.9961892849935,12.2727159278967,36.4455740968745));
#44498=CARTESIAN_POINT('Ctrl Pts',(20.775446145391,12.2903171298382,36.3262031637697));
#44499=CARTESIAN_POINT('Ctrl Pts',(20.6241695646565,12.302089960567,36.267493262113));
#44500=CARTESIAN_POINT('Ctrl Pts',(20.4377021427713,12.3153467701843,36.2209329114971));
#44501=CARTESIAN_POINT('Ctrl Pts',(20.4078815416648,12.3174281133537,36.2142351164447));
#44502=CARTESIAN_POINT('Ctrl Pts',(20.3709772532854,12.3199463507237,36.2068628020227));
#44503=CARTESIAN_POINT('Ctrl Pts',(20.3640343891044,12.3204176196015,36.2055154948656));
#44504=CARTESIAN_POINT('Ctrl Pts',(20.353090116737,12.3211564118,36.2034540752868));
#44505=CARTESIAN_POINT('Ctrl Pts',(20.3490936789788,12.3214253352063,36.2027143917852));
#44506=CARTESIAN_POINT('Ctrl Pts',(20.3415812732448,12.3219292060278,36.2013484931997));
#44507=CARTESIAN_POINT('Ctrl Pts',(20.3380659445226,12.3221643052714,36.2007194183288));
#44508=CARTESIAN_POINT('Ctrl Pts',(20.3300421087723,12.3226993985278,36.1993065204055));
#44509=CARTESIAN_POINT('Ctrl Pts',(20.3255325495797,12.3229990369049,36.1985289754604));
#44510=CARTESIAN_POINT('Ctrl Pts',(20.3135798019636,12.3237904428302,36.1965118332401));
#44511=CARTESIAN_POINT('Ctrl Pts',(20.3061319442596,12.3242807061441,36.195299831885));
#44512=CARTESIAN_POINT('Ctrl Pts',(20.2539218335032,12.3276986372308,36.1871177560539));
#44513=CARTESIAN_POINT('Ctrl Pts',(20.208929297298,12.3305472098203,36.1816819669351));
#44514=CARTESIAN_POINT('Ctrl Pts',(20.0269101550315,12.3418320492146,36.1661725411715));
#44515=CARTESIAN_POINT('Ctrl Pts',(19.8891744838841,12.3498530059803,36.1691617887092));
#44516=CARTESIAN_POINT('Ctrl Pts',(19.6884441257685,12.3620623308559,36.1950849140065));
#44517=CARTESIAN_POINT('Ctrl Pts',(19.6244388164892,12.3660306662166,36.2066639799372));
#44518=CARTESIAN_POINT('Ctrl Pts',(19.5239358809418,12.3724784752898,36.2301429249375));
#44519=CARTESIAN_POINT('Ctrl Pts',(19.4869968082867,12.3748955523179,36.2399381895636));
#44520=CARTESIAN_POINT('Ctrl Pts',(19.4396464623003,12.3780661859068,36.2540119895151));
#44521=CARTESIAN_POINT('Ctrl Pts',(19.4289462750206,12.3787875034616,36.2572939852841));
#44522=CARTESIAN_POINT('Ctrl Pts',(19.4116291418237,12.3799629835065,36.2627708684501));
#44523=CARTESIAN_POINT('Ctrl Pts',(19.4049943666356,12.3804152912751,36.2649088734563));
#44524=CARTESIAN_POINT('Ctrl Pts',(19.3969483833219,12.3809662089533,36.2675498512499));
#44525=CARTESIAN_POINT('Ctrl Pts',(19.3955259198999,12.381063698177,36.2680185900266));
#44526=CARTESIAN_POINT('Ctrl Pts',(19.3941040087481,12.3811612414289,36.2684889831931));
#44527=CARTESIAN_POINT('Origin',(20.,-1.3495818343519,38.1));
#44528=CARTESIAN_POINT('',(19.3941040122263,13.3471516131145,36.2684889820425));
#44529=CARTESIAN_POINT('',(19.3941040017606,13.1771182491666,36.2684889855047));
#44530=CARTESIAN_POINT('',(19.3941040087494,-1.3495818343519,36.2684889831927));
#44531=CARTESIAN_POINT('',(18.070870312024,12.710826110243,38.0989027900441));
#44532=CARTESIAN_POINT('Ctrl Pts',(19.3941040122264,13.3471516131145,36.2684889820425));
#44533=CARTESIAN_POINT('Ctrl Pts',(19.4104866366325,13.3459230207428,36.2630693223737));
#44534=CARTESIAN_POINT('Ctrl Pts',(19.4269473258092,13.3446960253705,36.2578677037214));
#44535=CARTESIAN_POINT('Ctrl Pts',(19.4546956134867,13.3426420104863,36.2495074043374));
#44536=CARTESIAN_POINT('Ctrl Pts',(19.46594005021,13.3418135851885,36.2462309483532));
#44537=CARTESIAN_POINT('Ctrl Pts',(19.4922436281491,13.3398857010468,36.2388256864404));
#44538=CARTESIAN_POINT('Ctrl Pts',(19.5073246304984,13.3387879650191,36.2347768609654));
#44539=CARTESIAN_POINT('Ctrl Pts',(19.5693839592259,13.3343057046446,36.2189208860509));
#44540=CARTESIAN_POINT('Ctrl Pts',(19.6167541759491,13.3309658843936,36.2087008831235));
#44541=CARTESIAN_POINT('Ctrl Pts',(19.6720309607961,13.3271988364703,36.1989376852914));
#44542=CARTESIAN_POINT('Ctrl Pts',(19.6796068318972,13.3266853660904,36.1976462374905));
#44543=CARTESIAN_POINT('Ctrl Pts',(19.6917462656369,13.3258673104694,36.195651421404));
#44544=CARTESIAN_POINT('Ctrl Pts',(19.6963048919101,13.3255611755419,36.194919120885));
#44545=CARTESIAN_POINT('Ctrl Pts',(19.7043990621246,13.3250195487343,36.1936486600551));
#44546=CARTESIAN_POINT('Ctrl Pts',(19.7079335239297,13.3247836946747,36.1931039566469));
#44547=CARTESIAN_POINT('Ctrl Pts',(19.7154635278836,13.3242826312277,36.1919649191741));
#44548=CARTESIAN_POINT('Ctrl Pts',(19.7194594222162,13.3240175751984,36.1913733055976));
#44549=CARTESIAN_POINT('Ctrl Pts',(19.7303449656706,13.3232977276198,36.1897965668133));
#44550=CARTESIAN_POINT('Ctrl Pts',(19.7372382175781,13.3228442970681,36.1888361548501));
#44551=CARTESIAN_POINT('Ctrl Pts',(19.7729223355767,13.3205087975777,36.1840611323613));
#44552=CARTESIAN_POINT('Ctrl Pts',(19.801793241533,13.3186587734508,36.1808594861779));
#44553=CARTESIAN_POINT('Ctrl Pts',(19.9899276761389,13.3067958172471,36.1642875926935));
#44554=CARTESIAN_POINT('Ctrl Pts',(20.1502705285004,13.2975358824369,36.1700997341512));
#44555=CARTESIAN_POINT('Ctrl Pts',(20.3995782342778,13.2822797140152,36.2104307659568));
#44556=CARTESIAN_POINT('Ctrl Pts',(20.4898846891814,13.2765770051853,36.2318072271933));
#44557=CARTESIAN_POINT('Ctrl Pts',(20.5912028442351,13.2697946368871,36.2636436248688));
#44558=CARTESIAN_POINT('Ctrl Pts',(20.6040645742524,13.2689265351607,36.2678342010854));
#44559=CARTESIAN_POINT('Ctrl Pts',(20.6246669120749,13.26752400971,36.2747873185555));
#44560=CARTESIAN_POINT('Ctrl Pts',(20.6324359413459,13.2669923676292,36.2774647163344));
#44561=CARTESIAN_POINT('Ctrl Pts',(20.6462326667885,13.2660432210262,36.282318244735));
#44562=CARTESIAN_POINT('Ctrl Pts',(20.6522671081762,13.2656263609765,36.2844749406881));
#44563=CARTESIAN_POINT('Ctrl Pts',(20.6648542174755,13.2647531879786,36.2890444001578));
#44564=CARTESIAN_POINT('Ctrl Pts',(20.6714047442395,13.2642966953321,36.2914627506309));
#44565=CARTESIAN_POINT('Ctrl Pts',(20.6884708075529,13.2631018799049,36.2978687669469));
#44566=CARTESIAN_POINT('Ctrl Pts',(20.6989647350276,13.2623616932598,36.3019128708161));
#44567=CARTESIAN_POINT('Ctrl Pts',(20.7454497181009,13.2590579260164,36.3202954705671));
#44568=CARTESIAN_POINT('Ctrl Pts',(20.7810371849496,13.2564615338074,36.3356236103787));
#44569=CARTESIAN_POINT('Ctrl Pts',(20.8762398377979,13.2493258909702,36.3800738017463));
#44570=CARTESIAN_POINT('Ctrl Pts',(20.9348494356302,13.2447233313987,36.4112142358477));
#44571=CARTESIAN_POINT('Ctrl Pts',(21.0915521980205,13.2318601121271,36.5051335256935));
#44572=CARTESIAN_POINT('Ctrl Pts',(21.1857467305076,13.2234729694017,36.573864933976));
#44573=CARTESIAN_POINT('Ctrl Pts',(21.2848959874715,13.2141622415327,36.6609626791333));
#44574=CARTESIAN_POINT('Ctrl Pts',(21.2964955796549,13.2130650678889,36.6714044166166));
#44575=CARTESIAN_POINT('Ctrl Pts',(21.3435735045677,13.2085832189015,36.7148288044768));
#44576=CARTESIAN_POINT('Ctrl Pts',(21.3779335204569,13.2052432554018,36.7490043967403));
#44577=CARTESIAN_POINT('Ctrl Pts',(21.4162141110084,13.2014760658311,36.790061372385));
#44578=CARTESIAN_POINT('Ctrl Pts',(21.4214213368371,13.200962589925,36.7957136034056));
#44579=CARTESIAN_POINT('Ctrl Pts',(21.4297027205722,13.20014452721,36.8048112089124));
#44580=CARTESIAN_POINT('Ctrl Pts',(21.4327984623419,13.1998383906732,36.8082366930513));
#44581=CARTESIAN_POINT('Ctrl Pts',(21.438270173611,13.1992967620524,36.8143350928391));
#44582=CARTESIAN_POINT('Ctrl Pts',(21.4406510429733,13.1990609077802,36.8170035389755));
#44583=CARTESIAN_POINT('Ctrl Pts',(21.4457053862687,13.1985598450376,36.8227001880427));
#44584=CARTESIAN_POINT('Ctrl Pts',(21.4483767698581,13.1982947899194,36.8257301671977));
#44585=CARTESIAN_POINT('Ctrl Pts',(21.4556247822914,13.1975749473947,36.8340033625685));
#44586=CARTESIAN_POINT('Ctrl Pts',(21.4601826415725,13.1971215209537,36.8392630529444));
#44587=CARTESIAN_POINT('Ctrl Pts',(21.4836118063188,13.1947860794523,36.8665974015581));
#44588=CARTESIAN_POINT('Ctrl Pts',(21.5020125127447,13.1929361073085,36.8890728370711));
#44589=CARTESIAN_POINT('Ctrl Pts',(21.6183205435363,13.1810733513055,37.0378692237385));
#44590=CARTESIAN_POINT('Ctrl Pts',(21.7007243985576,13.1718135505467,37.1755369235098));
#44591=CARTESIAN_POINT('Ctrl Pts',(21.802600615668,13.1565573547744,37.406626873208));
#44592=CARTESIAN_POINT('Ctrl Pts',(21.8338269770233,13.1508544504002,37.4940210563692));
#44593=CARTESIAN_POINT('Ctrl Pts',(21.8622724628248,13.144071865199,37.5963465319282));
#44594=CARTESIAN_POINT('Ctrl Pts',(21.8657582438401,13.1432037583718,37.6094169771574));
#44595=CARTESIAN_POINT('Ctrl Pts',(21.8711401114591,13.1418012262648,37.6304845399501));
#44596=CARTESIAN_POINT('Ctrl Pts',(21.873123094322,13.1412695826714,37.6384591523824));
#44597=CARTESIAN_POINT('Ctrl Pts',(21.8765616818611,13.1403204343388,37.6526747522642));
#44598=CARTESIAN_POINT('Ctrl Pts',(21.878037261573,13.1399035740804,37.6589108190113));
#44599=CARTESIAN_POINT('Ctrl Pts',(21.8810556999298,13.139030401638,37.6719570480719));
#44600=CARTESIAN_POINT('Ctrl Pts',(21.8825927065103,13.1385739097609,37.6787684553881));
#44601=CARTESIAN_POINT('Ctrl Pts',(21.8865085594151,13.1373790985584,37.6965715824627));
#44602=CARTESIAN_POINT('Ctrl Pts',(21.8888282998934,13.1366389153929,37.7075758961327));
#44603=CARTESIAN_POINT('Ctrl Pts',(21.8987110557985,13.1333351861143,37.7565763829884));
#44604=CARTESIAN_POINT('Ctrl Pts',(21.9052242331493,13.1307388293194,37.7947726915976));
#44605=CARTESIAN_POINT('Ctrl Pts',(21.9197584446584,13.1236033125858,37.8988291196341));
#44606=CARTESIAN_POINT('Ctrl Pts',(21.925539047832,13.1190008464822,37.9649443521454));
#44607=CARTESIAN_POINT('Ctrl Pts',(21.9320502179657,13.1061423907135,38.1474533354929));
#44608=CARTESIAN_POINT('Ctrl Pts',(21.9256770709189,13.0977601445207,38.2638168473678));
#44609=CARTESIAN_POINT('Ctrl Pts',(21.9065937978554,13.0884471474128,38.3944302193596));
#44610=CARTESIAN_POINT('Ctrl Pts',(21.9041343466194,13.0873433232281,38.4099378549386));
#44611=CARTESIAN_POINT('Ctrl Pts',(21.8933188571675,13.0828566601612,38.4731358037159));
#44612=CARTESIAN_POINT('Ctrl Pts',(21.8833574585024,13.0795184403877,38.520537999419));
#44613=CARTESIAN_POINT('Ctrl Pts',(21.8697596235999,13.0757529751212,38.5749742635082));
#44614=CARTESIAN_POINT('Ctrl Pts',(21.8678528600873,13.0752395665345,38.5824181784729));
#44615=CARTESIAN_POINT('Ctrl Pts',(21.8647293369496,13.0744215902376,38.5943160638661));
#44616=CARTESIAN_POINT('Ctrl Pts',(21.863541002051,13.0741154733053,38.5987773108806));
#44617=CARTESIAN_POINT('Ctrl Pts',(21.8614037783182,13.0735738667729,38.6066866088654));
#44618=CARTESIAN_POINT('Ctrl Pts',(21.8604613041627,13.0733380150907,38.6101363367485));
#44619=CARTESIAN_POINT('Ctrl Pts',(21.8584337870053,13.072836943765,38.6174772789418));
#44620=CARTESIAN_POINT('Ctrl Pts',(21.8573461149006,13.0725718775461,38.6213677062395));
#44621=CARTESIAN_POINT('Ctrl Pts',(21.8543510806332,13.0718519734385,38.6319521344957));
#44622=CARTESIAN_POINT('Ctrl Pts',(21.8524196748341,13.0713984969087,38.6386393557295));
#44623=CARTESIAN_POINT('Ctrl Pts',(21.8422399281184,13.0690623487005,38.6731828681232));
#44624=CARTESIAN_POINT('Ctrl Pts',(21.8333987925271,13.0672117430411,38.7008624147925));
#44625=CARTESIAN_POINT('Ctrl Pts',(21.771872335493,13.055346545361,38.8794622835719));
#44626=CARTESIAN_POINT('Ctrl Pts',(21.7012229380199,13.0460851093458,39.0235506671442));
#44627=CARTESIAN_POINT('Ctrl Pts',(21.5628153516968,13.0308292464975,39.2347845284807));
#44628=CARTESIAN_POINT('Ctrl Pts',(21.5065230114638,13.0251287268431,39.3085167596184));
#44629=CARTESIAN_POINT('Ctrl Pts',(21.4361966824007,13.0183487868164,39.3880468176911));
#44630=CARTESIAN_POINT('Ctrl Pts',(21.4271303824469,13.0174807422252,39.3980848861556));
#44631=CARTESIAN_POINT('Ctrl Pts',(21.4123878709626,13.0160782913333,39.4140664294999));
#44632=CARTESIAN_POINT('Ctrl Pts',(21.4067778263824,13.0155466661956,39.4200705371096));
#44633=CARTESIAN_POINT('Ctrl Pts',(21.3967247845257,13.0145975389675,39.4306928642066));
#44634=CARTESIAN_POINT('Ctrl Pts',(21.3922967857882,13.0141806812558,39.4353251593499));
#44635=CARTESIAN_POINT('Ctrl Pts',(21.3829956941587,13.0133075020316,39.4449588197553));
#44636=CARTESIAN_POINT('Ctrl Pts',(21.3781183699987,13.0128510007657,39.4499559522515));
#44637=CARTESIAN_POINT('Ctrl Pts',(21.3653148824627,13.011656138009,39.4629322502915));
#44638=CARTESIAN_POINT('Ctrl Pts',(21.3573459742881,13.010915912381,39.4708686823296));
#44639=CARTESIAN_POINT('Ctrl Pts',(21.3216155433143,13.0076117197749,39.5058365125635));
#44640=CARTESIAN_POINT('Ctrl Pts',(21.293114415621,13.005014930777,39.5320959069014));
#44641=CARTESIAN_POINT('Ctrl Pts',(21.2137188031712,12.9978778749748,39.6009433611213));
#44642=CARTESIAN_POINT('Ctrl Pts',(21.1613899964115,12.9932742680904,39.641789877225));
#44643=CARTESIAN_POINT('Ctrl Pts',(20.9967247244561,12.97911704074,39.7571771174533));
#44644=CARTESIAN_POINT('Ctrl Pts',(20.8785927519293,12.9693661124324,39.8227214746303));
#44645=CARTESIAN_POINT('Ctrl Pts',(20.7123522386906,12.9567470631984,39.8933778168564));
#44646=CARTESIAN_POINT('Ctrl Pts',(20.6694745084918,12.9535868605786,39.9098216409358));
#44647=CARTESIAN_POINT('Ctrl Pts',(20.6188808313852,12.949998050936,39.9271799240489));
#44648=CARTESIAN_POINT('Ctrl Pts',(20.6116999432382,12.9494919221188,39.9295964424867));
#44649=CARTESIAN_POINT('Ctrl Pts',(20.6001506873117,12.9486832967249,39.9334074104137));
#44650=CARTESIAN_POINT('Ctrl Pts',(20.5957913486339,12.9483793051997,39.9348286704784));
#44651=CARTESIAN_POINT('Ctrl Pts',(20.5880267023203,12.9478400857853,39.9373295608548));
#44652=CARTESIAN_POINT('Ctrl Pts',(20.5846234186874,12.9476045073072,39.9384152895781));
#44653=CARTESIAN_POINT('Ctrl Pts',(20.5773469980773,12.9471024705249,39.9407143921046));
#44654=CARTESIAN_POINT('Ctrl Pts',(20.573473048543,12.9468361736054,39.9419249965286));
#44655=CARTESIAN_POINT('Ctrl Pts',(20.5628626993358,12.9461094360908,39.945203998203));
#44656=CARTESIAN_POINT('Ctrl Pts',(20.5561186589963,12.9456504007926,39.9472477511557));
#44657=CARTESIAN_POINT('Ctrl Pts',(20.5204076043933,12.9432342022211,39.9578565383805));
#44658=CARTESIAN_POINT('Ctrl Pts',(20.4912517458491,12.9413117792703,39.965777843303));
#44659=CARTESIAN_POINT('Ctrl Pts',(20.3047241725903,12.9292599988344,40.0117790572774));
#44660=CARTESIAN_POINT('Ctrl Pts',(20.1432575342885,12.91988983781,40.03060757333));
#44661=CARTESIAN_POINT('Ctrl Pts',(19.8918904887004,12.9046833221753,40.0281736255631));
#44662=CARTESIAN_POINT('Ctrl Pts',(19.8026391473951,12.8991723910193,40.0210899929774));
#44663=CARTESIAN_POINT('Ctrl Pts',(19.7009114083019,12.8926025723142,40.0058513434477));
#44664=CARTESIAN_POINT('Ctrl Pts',(19.687636081004,12.8917396596755,40.0037205930605));
#44665=CARTESIAN_POINT('Ctrl Pts',(19.6663086228007,12.8903439070732,40.0000683545536));
#44666=CARTESIAN_POINT('Ctrl Pts',(19.6582418672984,12.8898138052589,39.9986339990952));
#44667=CARTESIAN_POINT('Ctrl Pts',(19.643885928606,12.8888664179622,39.9959869058434));
#44668=CARTESIAN_POINT('Ctrl Pts',(19.6375931495088,12.8884497684525,39.9947941450312));
#44669=CARTESIAN_POINT('Ctrl Pts',(19.6244408518261,12.887576019657,39.992233285598));
#44670=CARTESIAN_POINT('Ctrl Pts',(19.617582612476,12.8871187356132,39.9908591752054));
#44671=CARTESIAN_POINT('Ctrl Pts',(19.5996645967671,12.8859195752531,39.9871676687298));
#44672=CARTESIAN_POINT('Ctrl Pts',(19.5886175725973,12.8851758099725,39.9847903687745));
#44673=CARTESIAN_POINT('Ctrl Pts',(19.5392666116037,12.8818327482801,39.9737155941892));
#44674=CARTESIAN_POINT('Ctrl Pts',(19.5012151413987,12.8791996711569,39.9639470665539));
#44675=CARTESIAN_POINT('Ctrl Pts',(19.3060465410578,12.8653946924124,39.9074395605454));
#44676=CARTESIAN_POINT('Ctrl Pts',(19.1550739613653,12.8536174360061,39.8419791046248));
#44677=CARTESIAN_POINT('Ctrl Pts',(18.9445484973521,12.8362234263025,39.7168288036242));
#44678=CARTESIAN_POINT('Ctrl Pts',(18.8775416623102,12.8305335302837,39.6710518013999));
#44679=CARTESIAN_POINT('Ctrl Pts',(18.8062448970758,12.8244567138134,39.6154466299317));
#44680=CARTESIAN_POINT('Ctrl Pts',(18.7989240432594,12.823832495801,39.6096510486458));
#44681=CARTESIAN_POINT('Ctrl Pts',(18.7881067434159,12.8229101480593,39.6009589929291));
#44682=CARTESIAN_POINT('Ctrl Pts',(18.7845781112529,12.8226092753919,39.598103066284));
#44683=CARTESIAN_POINT('Ctrl Pts',(18.7783002468361,12.8220740358612,39.5929852456389));
#44684=CARTESIAN_POINT('Ctrl Pts',(18.7755471708376,12.821839333429,39.5907281779216));
#44685=CARTESIAN_POINT('Ctrl Pts',(18.7727872050046,12.8216040671038,39.5884526572878));
#44686=CARTESIAN_POINT('Ctrl Pts',(18.7727741229622,12.8216029519586,39.5884418711916));
#44687=CARTESIAN_POINT('Ctrl Pts',(18.7727481362398,12.8216007367877,39.5884204446584));
#44688=CARTESIAN_POINT('Ctrl Pts',(18.7727352311704,12.8215996367288,39.588409803908));
#44689=CARTESIAN_POINT('Ctrl Pts',(18.772709594357,12.8215974513866,39.588388664761));
#44690=CARTESIAN_POINT('Ctrl Pts',(18.7726968627564,12.8215963661155,39.5883781664901));
#44691=CARTESIAN_POINT('Ctrl Pts',(18.7726715698982,12.8215942100944,39.5883573098651));
#44692=CARTESIAN_POINT('Ctrl Pts',(18.7726590086188,12.8215931393426,39.5883469515004));
#44693=CARTESIAN_POINT('Ctrl Pts',(18.7726340532885,12.8215910120948,39.5883263721413));
#44694=CARTESIAN_POINT('Ctrl Pts',(18.7726216591897,12.8215899555946,39.5883161511144));
#44695=CARTESIAN_POINT('Ctrl Pts',(18.772597035398,12.8215878566093,39.5882958441243));
#44696=CARTESIAN_POINT('Ctrl Pts',(18.7725848055628,12.821586814112,39.5882857580505));
#44697=CARTESIAN_POINT('Ctrl Pts',(18.7725605068196,12.821584742836,39.5882657181181));
#44698=CARTESIAN_POINT('Ctrl Pts',(18.7725484380574,12.8215837140697,39.5882557643864));
#44699=CARTESIAN_POINT('Ctrl Pts',(18.7725244592334,12.8215816700656,39.5882359873212));
#44700=CARTESIAN_POINT('Ctrl Pts',(18.7725125489533,12.8215806548093,39.5882261638143));
#44701=CARTESIAN_POINT('Ctrl Pts',(18.7693324349942,12.8213095755693,39.5856031662366));
#44702=CARTESIAN_POINT('Ctrl Pts',(18.7661725477835,12.8210402445904,39.5829798521973));
#44703=CARTESIAN_POINT('Ctrl Pts',(18.7574928997894,12.8203004298393,39.5757271295888));
#44704=CARTESIAN_POINT('Ctrl Pts',(18.7519905862658,12.8198314252761,39.5710768036695));
#44705=CARTESIAN_POINT('Ctrl Pts',(18.7396084035956,12.8187756285039,39.5604924241627));
#44706=CARTESIAN_POINT('Ctrl Pts',(18.7327440929185,12.8181900663589,39.5545403296896));
#44707=CARTESIAN_POINT('Ctrl Pts',(18.711354852398,12.8163636818709,39.5357272038118));
#44708=CARTESIAN_POINT('Ctrl Pts',(18.6969812629984,12.815133759565,39.522695031856));
#44709=CARTESIAN_POINT('Ctrl Pts',(18.6400319629903,12.8102384024566,39.4694732855197));
#44710=CARTESIAN_POINT('Ctrl Pts',(18.5990962053157,12.8066678079791,39.4275691225681));
#44711=CARTESIAN_POINT('Ctrl Pts',(18.4948705759095,12.7972261004701,39.3106785738321));
#44712=CARTESIAN_POINT('Ctrl Pts',(18.4352887521709,12.7914362519711,39.2326236449761));
#44713=CARTESIAN_POINT('Ctrl Pts',(18.3298943415409,12.7797563213007,39.0702639614246));
#44714=CARTESIAN_POINT('Ctrl Pts',(18.2839178012904,12.7738882745998,38.986410340952));
#44715=CARTESIAN_POINT('Ctrl Pts',(18.2387086279348,12.7669223864517,38.8871340580069));
#44716=CARTESIAN_POINT('Ctrl Pts',(18.2332062565997,12.7660501222301,38.8747045731856));
#44717=CARTESIAN_POINT('Ctrl Pts',(18.2245813657808,12.7646421657658,38.8546516249525));
#44718=CARTESIAN_POINT('Ctrl Pts',(18.2213754613741,12.7641092902842,38.8470643539315));
#44719=CARTESIAN_POINT('Ctrl Pts',(18.2157608452973,12.7631587319812,38.8335354781735));
#44720=CARTESIAN_POINT('Ctrl Pts',(18.2133329636354,12.7627417004449,38.8276019230526));
#44721=CARTESIAN_POINT('Ctrl Pts',(18.2083260997637,12.7618689743556,38.8151893596229));
#44722=CARTESIAN_POINT('Ctrl Pts',(18.2057525852766,12.7614131041079,38.8087082598088));
#44723=CARTESIAN_POINT('Ctrl Pts',(18.1991359997421,12.7602217067549,38.7917780987395));
#44724=CARTESIAN_POINT('Ctrl Pts',(18.1951487653516,12.7594843354415,38.7813076376802));
#44725=CARTESIAN_POINT('Ctrl Pts',(18.1779266227264,12.7562111336676,38.7348700279562));
#44726=CARTESIAN_POINT('Ctrl Pts',(18.1656748292056,12.7536432349123,38.6985500464781));
#44727=CARTESIAN_POINT('Ctrl Pts',(18.1354956329723,12.7466087250239,38.5994289321728));
#44728=CARTESIAN_POINT('Ctrl Pts',(18.1196630484594,12.742081010321,38.5360473017325));
#44729=CARTESIAN_POINT('Ctrl Pts',(18.0829226756844,12.728673977758,38.3490888010809));
#44730=CARTESIAN_POINT('Ctrl Pts',(18.0707990830953,12.7196304759924,38.2241384755919));
#44731=CARTESIAN_POINT('Ctrl Pts',(18.070870312024,12.710826110243,38.0989027900441));
#44732=CARTESIAN_POINT('Ctrl Pts',(18.0708703135747,12.7108259188098,38.0989000670461));
#44733=CARTESIAN_POINT('Ctrl Pts',(18.0709026179318,12.7068427740739,38.0422427098023));
#44734=CARTESIAN_POINT('Ctrl Pts',(18.0734309147293,12.7029187220878,37.9856069657395));
#44735=CARTESIAN_POINT('Ctrl Pts',(18.0789883844697,12.6987069164986,37.9230990867487));
#44736=CARTESIAN_POINT('Ctrl Pts',(18.0795557556661,12.6983000684806,37.9170424451146));
#44737=CARTESIAN_POINT('Ctrl Pts',(18.0805522371805,12.6976223674496,37.9069208747982));
#44738=CARTESIAN_POINT('Ctrl Pts',(18.0809656300099,12.6973506938101,37.9028544945266));
#44739=CARTESIAN_POINT('Ctrl Pts',(18.081742345095,12.6968570081796,37.8954482648573));
#44740=CARTESIAN_POINT('Ctrl Pts',(18.0821014724423,12.6966347689286,37.8921080055112));
#44741=CARTESIAN_POINT('Ctrl Pts',(18.0828591844516,12.6961780051474,37.8852295939745));
#44742=CARTESIAN_POINT('Ctrl Pts',(18.0832588334862,12.6959435519465,37.8816916518885));
#44743=CARTESIAN_POINT('Ctrl Pts',(18.0841909141036,12.695411083327,37.8736402033923));
#44744=CARTESIAN_POINT('Ctrl Pts',(18.0847295007692,12.6951134146856,37.8691274660265));
#44745=CARTESIAN_POINT('Ctrl Pts',(18.0861719981272,12.6943413367468,37.8573935335564));
#44746=CARTESIAN_POINT('Ctrl Pts',(18.0871008420414,12.6938682799795,37.8501753938117));
#44747=CARTESIAN_POINT('Ctrl Pts',(18.0933979240791,12.690809789562,37.8033356180808));
#44748=CARTESIAN_POINT('Ctrl Pts',(18.0999564567127,12.6882858144034,37.7638805295169));
#44749=CARTESIAN_POINT('Ctrl Pts',(18.1132876790424,12.6840327512664,37.6966726168074));
#44750=CARTESIAN_POINT('Ctrl Pts',(18.1194583621691,12.6822837523729,37.6688160082693));
#44751=CARTESIAN_POINT('Ctrl Pts',(18.1531427171125,12.6736727124743,37.5312762650907));
#44752=CARTESIAN_POINT('Ctrl Pts',(18.1896453070339,12.6670232320669,37.4240220826873));
#44753=CARTESIAN_POINT('Ctrl Pts',(18.2620148362235,12.6562241379459,37.2601719599779));
#44754=CARTESIAN_POINT('Ctrl Pts',(18.2917780902862,12.652195654333,37.2011783404125));
#44755=CARTESIAN_POINT('Ctrl Pts',(18.3436498845137,12.6456597181386,37.1102835110783));
#44756=CARTESIAN_POINT('Ctrl Pts',(18.363796244046,12.6432169203731,37.077321468207));
#44757=CARTESIAN_POINT('Ctrl Pts',(18.391061212038,12.6400171262155,37.0355824384427));
#44758=CARTESIAN_POINT('Ctrl Pts',(18.3972870732006,12.6392931221061,37.02623092131));
#44759=CARTESIAN_POINT('Ctrl Pts',(18.4075129713709,12.6381143429789,37.0111582565043));
#44760=CARTESIAN_POINT('Ctrl Pts',(18.4114630664718,12.6376614423418,37.0054034133859));
#44761=CARTESIAN_POINT('Ctrl Pts',(18.4190998393028,12.6367904247175,36.9944058995908));
#44762=CARTESIAN_POINT('Ctrl Pts',(18.4227815884265,12.6363724981213,36.9891599064275));
#44763=CARTESIAN_POINT('Ctrl Pts',(18.4312465609693,12.635416087076,36.9772253924588));
#44764=CARTESIAN_POINT('Ctrl Pts',(18.4360465188126,12.6348769690029,36.9705489488405));
#44765=CARTESIAN_POINT('Ctrl Pts',(18.4488660345377,12.6334454009973,36.9529562106468));
#44766=CARTESIAN_POINT('Ctrl Pts',(18.4569580172595,12.6325501765981,36.9420935024053));
#44767=CARTESIAN_POINT('Ctrl Pts',(18.5217824141114,12.6254428547722,36.8569593308747));
#44768=CARTESIAN_POINT('Ctrl Pts',(18.5837210048834,12.6190246081369,36.7868258367444));
#44769=CARTESIAN_POINT('Ctrl Pts',(18.7642969505792,12.6012676443994,36.6100517931978));
#44770=CARTESIAN_POINT('Ctrl Pts',(18.8914568175212,12.5896737559539,36.5131674388335));
#44771=CARTESIAN_POINT('Ctrl Pts',(19.0456515281141,12.5773851187491,36.4233576357675));
#44772=CARTESIAN_POINT('Ctrl Pts',(19.062373416056,12.5760745473963,36.41394926697));
#44773=CARTESIAN_POINT('Ctrl Pts',(19.087153945382,12.574167527684,36.4004895183066));
#44774=CARTESIAN_POINT('Ctrl Pts',(19.0951045652452,12.5735609118318,36.3962429585337));
#44775=CARTESIAN_POINT('Ctrl Pts',(19.1094789486094,12.5724739580307,36.3886943658217));
#44776=CARTESIAN_POINT('Ctrl Pts',(19.1158919938871,12.5719924936274,36.3853724153249));
#44777=CARTESIAN_POINT('Ctrl Pts',(19.125955120808,12.5712425913719,36.3802311970385));
#44778=CARTESIAN_POINT('Ctrl Pts',(19.1295924895831,12.5709726720597,36.3783873975091));
#44779=CARTESIAN_POINT('Ctrl Pts',(19.136413973045,12.5704686313622,36.3749566999036));
#44780=CARTESIAN_POINT('Ctrl Pts',(19.1395966020977,12.5702343486909,36.373367089859));
#44781=CARTESIAN_POINT('Ctrl Pts',(19.1468219535318,12.5697044507354,36.3697832223703));
#44782=CARTESIAN_POINT('Ctrl Pts',(19.1508672721363,12.5694091686982,36.3677943285923));
#44783=CARTESIAN_POINT('Ctrl Pts',(19.1631690343525,12.5685153396171,36.3617995782881));
#44784=CARTESIAN_POINT('Ctrl Pts',(19.1714472709191,12.5679194688469,36.3578383673378));
#44785=CARTESIAN_POINT('Ctrl Pts',(19.2494530179171,12.5623542043217,36.321193697273));
#44786=CARTESIAN_POINT('Ctrl Pts',(19.3210323635695,12.5576170286597,36.2926623636835));
#44787=CARTESIAN_POINT('Ctrl Pts',(19.394104060634,12.5529621656639,36.2684889660284));
#44788=CARTESIAN_POINT('Ctrl Pts',(19.3941040087481,12.3811612414289,36.2684889831931));
#44789=CARTESIAN_POINT('Ctrl Pts',(19.3894385614427,12.3814812915961,36.2700323950502));
#44790=CARTESIAN_POINT('Ctrl Pts',(19.3847790597086,12.3818019234793,36.2715936175433));
#44791=CARTESIAN_POINT('Ctrl Pts',(19.3723204967097,12.3826619093985,36.2758210252751));
#44792=CARTESIAN_POINT('Ctrl Pts',(19.3645325459949,12.383202315171,36.2785193929037));
#44793=CARTESIAN_POINT('Ctrl Pts',(19.3439298925368,12.3846395490855,36.285806008883));
#44794=CARTESIAN_POINT('Ctrl Pts',(19.3311462371627,12.3855391868955,36.2904800495199));
#44795=CARTESIAN_POINT('Ctrl Pts',(19.2282827106638,12.3928431038524,36.3293285953864));
#44796=CARTESIAN_POINT('Ctrl Pts',(19.1408430686202,12.3994670186418,36.3700667720709));
#44797=CARTESIAN_POINT('Ctrl Pts',(18.9730597772507,12.4129994089861,36.4641037847634));
#44798=CARTESIAN_POINT('Ctrl Pts',(18.8929217054918,12.4198877654547,36.5172369712706));
#44799=CARTESIAN_POINT('Ctrl Pts',(18.7555623280958,12.432249848792,36.6238625797878));
#44800=CARTESIAN_POINT('Ctrl Pts',(18.696988212218,12.437731368485,36.6753001297696));
#44801=CARTESIAN_POINT('Ctrl Pts',(18.6315663969375,12.4439710121969,36.7401710214812));
#44802=CARTESIAN_POINT('Ctrl Pts',(18.6215646358858,12.4449283571687,36.7503106456924));
#44803=CARTESIAN_POINT('Ctrl Pts',(18.607938726817,12.4462361940956,36.7644338515393));
#44804=CARTESIAN_POINT('Ctrl Pts',(18.6042178965868,12.4465937022498,36.7683229195028));
#44805=CARTESIAN_POINT('Ctrl Pts',(18.5979712220241,12.4471944603881,36.7749069827943));
#44806=CARTESIAN_POINT('Ctrl Pts',(18.5954367736909,12.4474383613948,36.7775937301403));
#44807=CARTESIAN_POINT('Ctrl Pts',(18.5906335855341,12.4479008638559,36.782714935962));
#44808=CARTESIAN_POINT('Ctrl Pts',(18.5883634114059,12.4481195778438,36.785148003643));
#44809=CARTESIAN_POINT('Ctrl Pts',(18.5824309088651,12.4486914764439,36.7915392599731));
#44810=CARTESIAN_POINT('Ctrl Pts',(18.5787788288706,12.4490438891074,36.79550698707));
#44811=CARTESIAN_POINT('Ctrl Pts',(18.5661812898456,12.4502609404076,36.8093090242261));
#44812=CARTESIAN_POINT('Ctrl Pts',(18.5573206360105,12.4511194965842,36.8192207196997));
#44813=CARTESIAN_POINT('Ctrl Pts',(18.4543801621525,12.4611351320356,36.9367957871383));
#44814=CARTESIAN_POINT('Ctrl Pts',(18.3724329171708,12.4695404467044,37.0545225461056));
#44815=CARTESIAN_POINT('Ctrl Pts',(18.2625909057656,12.4833197714927,37.257038087801));
#44816=CARTESIAN_POINT('Ctrl Pts',(18.2262052961051,12.4885794995811,37.3365698201978));
#44817=CARTESIAN_POINT('Ctrl Pts',(18.1845178086963,12.4959028971725,37.4469270980462));
#44818=CARTESIAN_POINT('Ctrl Pts',(18.1743830716012,12.4978217088382,37.4758185512877));
#44819=CARTESIAN_POINT('Ctrl Pts',(18.1581780124565,12.501151626343,37.5257918954755));
#44820=CARTESIAN_POINT('Ctrl Pts',(18.1517717770796,12.5025519740575,37.546759044586));
#44821=CARTESIAN_POINT('Ctrl Pts',(18.1432203360055,12.5045485009324,37.5765554117449));
#44822=CARTESIAN_POINT('Ctrl Pts',(18.1407778731173,12.5051350914937,37.5852981096874));
#44823=CARTESIAN_POINT('Ctrl Pts',(18.1366853734852,12.5061469017297,37.600356362579));
#44824=CARTESIAN_POINT('Ctrl Pts',(18.1350055058335,12.5065711551665,37.6066637082198));
#44825=CARTESIAN_POINT('Ctrl Pts',(18.1318592437799,12.5073831769145,37.6187226350318));
#44826=CARTESIAN_POINT('Ctrl Pts',(18.1303873184461,12.5077707623048,37.6244727066352));
#44827=CARTESIAN_POINT('Ctrl Pts',(18.1266458038984,12.5087762977336,37.6393748551344));
#44828=CARTESIAN_POINT('Ctrl Pts',(18.124416759365,12.5093955362011,37.6485368561473));
#44829=CARTESIAN_POINT('Ctrl Pts',(18.117113007349,12.5114949990487,37.6795453107317));
#44830=CARTESIAN_POINT('Ctrl Pts',(18.1123522957543,12.5129851355133,37.7014631187228));
#44831=CARTESIAN_POINT('Ctrl Pts',(18.0831797851786,12.5229959686526,37.8480474258763));
#44832=CARTESIAN_POINT('Ctrl Pts',(18.0707556558024,12.5318961291499,37.9747587684464));
#44833=CARTESIAN_POINT('Ctrl Pts',(18.0709900032668,12.550305627564,38.2332319793663));
#44834=CARTESIAN_POINT('Ctrl Pts',(18.0845508458415,12.5597741731661,38.3643680613534));
#44835=CARTESIAN_POINT('Ctrl Pts',(18.1142285855124,12.569639921465,38.5069502337397));
#44836=CARTESIAN_POINT('Ctrl Pts',(18.1172608135519,12.570590326765,38.5207558732588));
#44837=CARTESIAN_POINT('Ctrl Pts',(18.1216908215274,12.5719015529136,38.5399179443012));
#44838=CARTESIAN_POINT('Ctrl Pts',(18.1229602388603,12.5722691784662,38.5453031603507));
#44839=CARTESIAN_POINT('Ctrl Pts',(18.1250363658388,12.5728575645545,38.5539440231882));
#44840=CARTESIAN_POINT('Ctrl Pts',(18.1258284162553,12.573079145883,38.5572031066483));
#44841=CARTESIAN_POINT('Ctrl Pts',(18.1275042302377,12.5735419566209,38.5640211156387));
#44842=CARTESIAN_POINT('Ctrl Pts',(18.1283896463398,12.5737830849446,38.5675796059643));
#44843=CARTESIAN_POINT('Ctrl Pts',(18.1305671077183,12.5743679600476,38.5762255444833));
#44844=CARTESIAN_POINT('Ctrl Pts',(18.1318697928919,12.5747111020066,38.5813103352729));
#44845=CARTESIAN_POINT('Ctrl Pts',(18.1365637488479,12.5759241380805,38.599326149744));
#44846=CARTESIAN_POINT('Ctrl Pts',(18.1400687526548,12.5767877894335,38.6122275325809));
#44847=CARTESIAN_POINT('Ctrl Pts',(18.1623996749785,12.5820474968774,38.6911712786608));
#44848=CARTESIAN_POINT('Ctrl Pts',(18.184608914253,12.586273971855,38.7562131937333));
#44849=CARTESIAN_POINT('Ctrl Pts',(18.2620999292085,12.5988456686863,38.9488548275447));
#44850=CARTESIAN_POINT('Ctrl Pts',(18.3277326192903,12.606971159464,39.0717891010379));
#44851=CARTESIAN_POINT('Ctrl Pts',(18.443083646501,12.6195121011069,39.241002972756));
#44852=CARTESIAN_POINT('Ctrl Pts',(18.4829203654776,12.6236152388869,39.2934589538701));
#44853=CARTESIAN_POINT('Ctrl Pts',(18.5334425004029,12.6286263575041,39.3533590594835));
#44854=CARTESIAN_POINT('Ctrl Pts',(18.5416211679351,12.629431981433,39.3628661852549));
#44855=CARTESIAN_POINT('Ctrl Pts',(18.5551737834233,12.6307582906004,39.3783129127683));
#44856=CARTESIAN_POINT('Ctrl Pts',(18.5604931421139,12.6312767292056,39.3843000825241));
#44857=CARTESIAN_POINT('Ctrl Pts',(18.5701078089014,12.6322100947065,39.3949870324086));
#44858=CARTESIAN_POINT('Ctrl Pts',(18.5743894170783,12.6326244458917,39.3996990253569));
#44859=CARTESIAN_POINT('Ctrl Pts',(18.5835435983463,12.6335076509805,39.4096737213795));
#44860=CARTESIAN_POINT('Ctrl Pts',(18.5884223401308,12.6339767619553,39.414930607326));
#44861=CARTESIAN_POINT('Ctrl Pts',(18.6016123275189,12.6352408565748,39.4289849303291));
#44862=CARTESIAN_POINT('Ctrl Pts',(18.6099771246929,12.6360381197919,39.4377314463036));
#44863=CARTESIAN_POINT('Ctrl Pts',(18.6521413790621,12.6400357613395,39.4809973457759));
#44864=CARTESIAN_POINT('Ctrl Pts',(18.6871442238691,12.6432883316831,39.5143145122849));
#44865=CARTESIAN_POINT('Ctrl Pts',(18.7931847713054,12.6529641124202,39.6079172417125));
#44866=CARTESIAN_POINT('Ctrl Pts',(18.8673755819212,12.6595221357419,39.6644090409455));
#44867=CARTESIAN_POINT('Ctrl Pts',(19.0575521339271,12.6756921820771,39.7885767865864));
#44868=CARTESIAN_POINT('Ctrl Pts',(19.1770930177662,12.6853512204797,39.849951212422));
#44869=CARTESIAN_POINT('Ctrl Pts',(19.315133925163,12.695380620995,39.9035238691594));
#44870=CARTESIAN_POINT('Ctrl Pts',(19.3282853061669,12.6963251378596,39.9084632385829));
#44871=CARTESIAN_POINT('Ctrl Pts',(19.3466771286605,12.6976296220969,39.9151424843372));
#44872=CARTESIAN_POINT('Ctrl Pts',(19.3518724675394,12.6979963046104,39.917004049577));
#44873=CARTESIAN_POINT('Ctrl Pts',(19.3602354577664,12.6985835725821,39.919960196882));
#44874=CARTESIAN_POINT('Ctrl Pts',(19.3633980489312,12.6988049731445,39.9210688466003));
#44875=CARTESIAN_POINT('Ctrl Pts',(19.3700295089851,12.6992677607782,39.9233741256175));
#44876=CARTESIAN_POINT('Ctrl Pts',(19.3734989222998,12.6995090453215,39.9245691057));
#44877=CARTESIAN_POINT('Ctrl Pts',(19.3819513049755,12.7000948944786,39.9274534333073));
#44878=CARTESIAN_POINT('Ctrl Pts',(19.3869378651887,12.7004388494064,39.92913232457));
#44879=CARTESIAN_POINT('Ctrl Pts',(19.4046946583734,12.7016579197617,39.935029967261));
#44880=CARTESIAN_POINT('Ctrl Pts',(19.4175024266653,12.7025267098489,39.9391356752712));
#44881=CARTESIAN_POINT('Ctrl Pts',(19.5857165784426,12.713812890742,39.9911254707784));
#44882=CARTESIAN_POINT('Ctrl Pts',(19.7465542659121,12.7232610610126,40.0193147913548));
#44883=CARTESIAN_POINT('Ctrl Pts',(20.0173762349158,12.7395474937246,40.0320980399145));
#44884=CARTESIAN_POINT('Ctrl Pts',(20.1259323487551,12.7461684534555,40.0280666368807));
#44885=CARTESIAN_POINT('Ctrl Pts',(20.2472870897022,12.7539728685391,40.0132649373908));
#44886=CARTESIAN_POINT('Ctrl Pts',(20.2609894771528,12.7548596849453,40.0114439835572));
#44887=CARTESIAN_POINT('Ctrl Pts',(20.2828903948863,12.7562866140849,40.0082936201062));
#44888=CARTESIAN_POINT('Ctrl Pts',(20.2911021291783,12.7568237856814,40.0070582222107));
#44889=CARTESIAN_POINT('Ctrl Pts',(20.3056488766126,12.7577792794614,40.004773622166));
#44890=CARTESIAN_POINT('Ctrl Pts',(20.3119871479582,12.758196926578,40.003745730218));
#44891=CARTESIAN_POINT('Ctrl Pts',(20.3251669424736,12.7590681875109,40.0015407457398));
#44892=CARTESIAN_POINT('Ctrl Pts',(20.3320074694585,12.759521963393,40.0003583310249));
#44893=CARTESIAN_POINT('Ctrl Pts',(20.3497310993728,12.7607018543041,39.9971961089283));
#44894=CARTESIAN_POINT('Ctrl Pts',(20.3606036985184,12.7614297479509,39.9951595926481));
#44895=CARTESIAN_POINT('Ctrl Pts',(20.4077197198617,12.7646022452176,39.9859142952311));
#44896=CARTESIAN_POINT('Ctrl Pts',(20.4437672277241,12.7670765329702,39.9777588845758));
#44897=CARTESIAN_POINT('Ctrl Pts',(20.5395577538856,12.7737832951403,39.9531749205135));
#44898=CARTESIAN_POINT('Ctrl Pts',(20.5987770524872,12.7780700377408,39.93489634623));
#44899=CARTESIAN_POINT('Ctrl Pts',(20.7833496792119,12.7918543893037,39.8680389985579));
#44900=CARTESIAN_POINT('Ctrl Pts',(20.9045535782705,12.8015733017003,39.8092040961798));
#44901=CARTESIAN_POINT('Ctrl Pts',(21.0631221448746,12.8146714398749,39.7106071693668));
#44902=CARTESIAN_POINT('Ctrl Pts',(21.1064481018816,12.8182901088628,39.6811571253871));
#44903=CARTESIAN_POINT('Ctrl Pts',(21.1554266306209,12.8223823792018,39.6448642739442));
#44904=CARTESIAN_POINT('Ctrl Pts',(21.1622932821645,12.8229561268215,39.6397047303394));
#44905=CARTESIAN_POINT('Ctrl Pts',(21.1726614715716,12.8238221971327,39.6318052722251));
#44906=CARTESIAN_POINT('Ctrl Pts',(21.1761882635435,12.8241167508104,39.6290989139398));
#44907=CARTESIAN_POINT('Ctrl Pts',(21.182517419016,12.8246452269678,39.6242072492631));
#44908=CARTESIAN_POINT('Ctrl Pts',(21.1853231118073,12.8248794498153,39.6220263815832));
#44909=CARTESIAN_POINT('Ctrl Pts',(21.1914396551959,12.8253899574658,39.6172448152299));
#44910=CARTESIAN_POINT('Ctrl Pts',(21.1947480157991,12.8256660204348,39.6146410336762));
#44911=CARTESIAN_POINT('Ctrl Pts',(21.2041151416654,12.8264475542174,39.6072190302928));
#44912=CARTESIAN_POINT('Ctrl Pts',(21.2101535524101,12.8269512452004,39.6023750744001));
#44913=CARTESIAN_POINT('Ctrl Pts',(21.2485852930034,12.8301574626768,39.5711634456018));
#44914=CARTESIAN_POINT('Ctrl Pts',(21.2801469785742,12.8327926657436,39.5437837223654));
#44915=CARTESIAN_POINT('Ctrl Pts',(21.3859893354915,12.8417379764338,39.4457633541241));
#44916=CARTESIAN_POINT('Ctrl Pts',(21.4555188571318,12.847814938025,39.370241575832));
#44917=CARTESIAN_POINT('Ctrl Pts',(21.6022832578745,12.8620374247799,39.1828640958038));
#44918=CARTESIAN_POINT('Ctrl Pts',(21.6743581448781,12.8701994281383,39.0676899569763));
#44919=CARTESIAN_POINT('Ctrl Pts',(21.7397841383618,12.8797255810793,38.933595757464));
#44920=CARTESIAN_POINT('Ctrl Pts',(21.7456675998606,12.8806057547467,38.9212035984987));
#44921=CARTESIAN_POINT('Ctrl Pts',(21.7548867655927,12.8820240255675,38.9012386953374));
#44922=CARTESIAN_POINT('Ctrl Pts',(21.7583068480036,12.8825592386653,38.8937052549385));
#44923=CARTESIAN_POINT('Ctrl Pts',(21.7642931343387,12.8835124784087,38.8802906280256));
#44924=CARTESIAN_POINT('Ctrl Pts',(21.7668786698948,12.8839298408367,38.8744181637039));
#44925=CARTESIAN_POINT('Ctrl Pts',(21.7722060169351,12.8848017505141,38.8621527257608));
#44926=CARTESIAN_POINT('Ctrl Pts',(21.7749426392276,12.8852564659792,38.8557576127109));
#44927=CARTESIAN_POINT('Ctrl Pts',(21.7819661760717,12.8864415223991,38.839095989857));
#44928=CARTESIAN_POINT('Ctrl Pts',(21.7861989219825,12.8871736713122,38.8288070644789));
#44929=CARTESIAN_POINT('Ctrl Pts',(21.8043322603752,12.8903909790854,38.7836216998618));
#44930=CARTESIAN_POINT('Ctrl Pts',(21.8173001062669,12.8929068707238,38.7483621861104));
#44931=CARTESIAN_POINT('Ctrl Pts',(21.8493745770503,12.8997584565884,38.6526107214742));
#44932=CARTESIAN_POINT('Ctrl Pts',(21.8665395683111,12.9041513811197,38.5915217137517));
#44933=CARTESIAN_POINT('Ctrl Pts',(21.9096358826708,12.9177498686682,38.402903985855));
#44934=CARTESIAN_POINT('Ctrl Pts',(21.925708350767,12.927149540771,38.2735078487818));
#44935=CARTESIAN_POINT('Ctrl Pts',(21.9298642738757,12.9400979826412,38.0891762989428));
#44936=CARTESIAN_POINT('Ctrl Pts',(21.9287944882263,12.9438564142326,38.0348362869205));
#44937=CARTESIAN_POINT('Ctrl Pts',(21.9248958727853,12.9480858454839,37.9719630035297));
#44938=CARTESIAN_POINT('Ctrl Pts',(21.9243015311271,12.9486645697535,37.9633207486838));
#44939=CARTESIAN_POINT('Ctrl Pts',(21.9233129197937,12.9495366382826,37.9502339393603));
#44940=CARTESIAN_POINT('Ctrl Pts',(21.9229614217371,12.9498322591349,37.9457864082832));
#44941=CARTESIAN_POINT('Ctrl Pts',(21.9223021584115,12.9503618640069,37.937797648107));
#44942=CARTESIAN_POINT('Ctrl Pts',(21.9220000335551,12.9505961543609,37.9342560322098));
#44943=CARTESIAN_POINT('Ctrl Pts',(21.9213197985246,12.9511058981754,37.9265341375067));
#44944=CARTESIAN_POINT('Ctrl Pts',(21.9209378350196,12.9513811347682,37.9223542613179));
#44945=CARTESIAN_POINT('Ctrl Pts',(21.9198182318219,12.9521579846264,37.9105283160174));
#44946=CARTESIAN_POINT('Ctrl Pts',(21.9190485515986,12.9526578516448,37.9028852524798));
#44947=CARTESIAN_POINT('Ctrl Pts',(21.9139261232015,12.9557837028355,37.8548957020745));
#44948=CARTESIAN_POINT('Ctrl Pts',(21.9083465067761,12.9583461971388,37.8146870280596));
#44949=CARTESIAN_POINT('Ctrl Pts',(21.8665713713731,12.9737242171507,37.5705097206401));
#44950=CARTESIAN_POINT('Ctrl Pts',(21.7989877623501,12.9855081415591,37.3732891954765));
#44951=CARTESIAN_POINT('Ctrl Pts',(21.6831026738316,13.0008510152839,37.1564951841658));
#44952=CARTESIAN_POINT('Ctrl Pts',(21.6638661860848,13.0032934489121,37.1229713716697));
#44953=CARTESIAN_POINT('Ctrl Pts',(21.6375138706213,13.0065219768893,37.0800844765128));
#44954=CARTESIAN_POINT('Ctrl Pts',(21.6313003609931,13.0072753454439,37.070175513025));
#44955=CARTESIAN_POINT('Ctrl Pts',(21.6211804342089,13.0084901952066,37.0543582290642));
#44956=CARTESIAN_POINT('Ctrl Pts',(21.6173308484455,13.0089495818076,37.0484137515919));
#44957=CARTESIAN_POINT('Ctrl Pts',(21.6099495448155,13.0098253297987,37.0371520500439));
#44958=CARTESIAN_POINT('Ctrl Pts',(21.6064239906753,13.0102414581594,37.031830883182));
#44959=CARTESIAN_POINT('Ctrl Pts',(21.5983307158113,13.0111918987519,37.019746285706));
#44960=CARTESIAN_POINT('Ctrl Pts',(21.5937463776876,13.0117268283385,37.0129941837723));
#44961=CARTESIAN_POINT('Ctrl Pts',(21.579580719837,13.0133694814656,36.9924123659104));
#44962=CARTESIAN_POINT('Ctrl Pts',(21.5698614195101,13.0144823951787,36.978679033073));
#44963=CARTESIAN_POINT('Ctrl Pts',(21.5471102082805,13.0170563267166,36.9474073028732));
#44964=CARTESIAN_POINT('Ctrl Pts',(21.5339576680707,13.0185218493343,36.9299599455592));
#44965=CARTESIAN_POINT('Ctrl Pts',(21.4882474111427,13.0235416538979,36.8714192583834));
#44966=CARTESIAN_POINT('Ctrl Pts',(21.4543144208415,13.0271471592378,36.831433982806));
#44967=CARTESIAN_POINT('Ctrl Pts',(21.3202457637964,13.0409466648584,36.6859104386596));
#44968=CARTESIAN_POINT('Ctrl Pts',(21.2099237570059,13.0514763907563,36.5904382149351));
#44969=CARTESIAN_POINT('Ctrl Pts',(21.0752167925078,13.0629507230472,36.4981980845933));
#44970=CARTESIAN_POINT('Ctrl Pts',(21.0603644449194,13.0641981109907,36.4883276372919));
#44971=CARTESIAN_POINT('Ctrl Pts',(21.0124534846761,13.0681611002534,36.4574364310749));
#44972=CARTESIAN_POINT('Ctrl Pts',(20.9788881743543,13.0708465518793,36.4372145087747));
#44973=CARTESIAN_POINT('Ctrl Pts',(20.9384209019949,13.0739583972686,36.4144849181742));
#44974=CARTESIAN_POINT('Ctrl Pts',(20.9320941546162,13.0744413489899,36.4109779837634));
#44975=CARTESIAN_POINT('Ctrl Pts',(20.9217721718468,13.0752233190207,36.4053321406502));
#44976=CARTESIAN_POINT('Ctrl Pts',(20.9177889335841,13.075523647175,36.4031716160037));
#44977=CARTESIAN_POINT('Ctrl Pts',(20.9106633770325,13.0760582962267,36.3993391168336));
#44978=CARTESIAN_POINT('Ctrl Pts',(20.907524018441,13.0762929496728,36.3976617896364));
#44979=CARTESIAN_POINT('Ctrl Pts',(20.9007192750668,13.076799620928,36.3940502587445));
#44980=CARTESIAN_POINT('Ctrl Pts',(20.8970523027785,13.0770714426467,36.3921191789105));
#44981=CARTESIAN_POINT('Ctrl Pts',(20.8867874006271,13.0778290378445,36.386755716232));
#44982=CARTESIAN_POINT('Ctrl Pts',(20.8801757150774,13.078313200024,36.3833496032255));
#44983=CARTESIAN_POINT('Ctrl Pts',(20.8413226403807,13.0811370611157,36.3636173216586));
#44984=CARTESIAN_POINT('Ctrl Pts',(20.8086448915068,13.0834266195273,36.348160270803));
#44985=CARTESIAN_POINT('Ctrl Pts',(20.6992023602477,13.0908783770015,36.300108000189));
#44986=CARTESIAN_POINT('Ctrl Pts',(20.6207553576899,13.0958784896369,36.2715689059064));
#44987=CARTESIAN_POINT('Ctrl Pts',(20.3965826012643,13.1098365678575,36.2061135275885));
#44988=CARTESIAN_POINT('Ctrl Pts',(20.2480627250366,13.1187514936008,36.1810048645534));
#44989=CARTESIAN_POINT('Ctrl Pts',(20.0762789190967,13.1296494133157,36.1722543560187));
#44990=CARTESIAN_POINT('Ctrl Pts',(20.0544003542533,13.1310470346824,36.1715129554781));
#44991=CARTESIAN_POINT('Ctrl Pts',(20.0241100082486,13.1329972752595,36.1710023531467));
#44992=CARTESIAN_POINT('Ctrl Pts',(20.0157046954574,13.1335400731801,36.1709156127982));
#44993=CARTESIAN_POINT('Ctrl Pts',(20.001244769397,13.1344767697442,36.1708609008153));
#44994=CARTESIAN_POINT('Ctrl Pts',(19.995190330847,13.1348698446403,36.1708664952495));
#44995=CARTESIAN_POINT('Ctrl Pts',(19.9826955951752,13.1356828985425,36.1709368606554));
#44996=CARTESIAN_POINT('Ctrl Pts',(19.9762554030158,13.136102988948,36.171005383513));
#44997=CARTESIAN_POINT('Ctrl Pts',(19.9612417095771,13.1370847497069,36.171240325024));
#44998=CARTESIAN_POINT('Ctrl Pts',(19.9526687885613,13.1376471863161,36.1714316601912));
#44999=CARTESIAN_POINT('Ctrl Pts',(19.9250852006237,13.1394629379899,36.1722313150435));
#45000=CARTESIAN_POINT('Ctrl Pts',(19.9060826501282,13.1407231612337,36.1730636187345));
#45001=CARTESIAN_POINT('Ctrl Pts',(19.8095132781625,13.1471770872879,36.1787251254538));
#45002=CARTESIAN_POINT('Ctrl Pts',(19.7322862382402,13.152505474303,36.1879568699085));
#45003=CARTESIAN_POINT('Ctrl Pts',(19.5731407572556,13.1638224954935,36.2168120686515));
#45004=CARTESIAN_POINT('Ctrl Pts',(19.491519858161,13.1698182844823,36.2371924624697));
#45005=CARTESIAN_POINT('Ctrl Pts',(19.4056874079929,13.1762486944391,36.2646874199425));
#45006=CARTESIAN_POINT('Ctrl Pts',(19.3998909291043,13.1766835529467,36.2665745683422));
#45007=CARTESIAN_POINT('Ctrl Pts',(19.3941040017606,13.1771182491666,36.2684889855047));
#45008=CARTESIAN_POINT('Origin',(20.,-1.3495818343519,38.1));
#45009=CARTESIAN_POINT('',(19.3941040087558,14.1433118141013,36.2684889831906));
#45010=CARTESIAN_POINT('',(19.3941039465104,13.9716756753762,36.2684890037825));
#45011=CARTESIAN_POINT('',(19.3941040087494,-1.3495818343519,36.2684889831927));
#45012=CARTESIAN_POINT('Ctrl Pts',(19.3941040087558,14.1433118141013,36.2684889831906));
#45013=CARTESIAN_POINT('Ctrl Pts',(19.3976160935084,14.1430688068057,36.2673271239099));
#45014=CARTESIAN_POINT('Ctrl Pts',(19.4011315012555,14.1428254683569,36.2661753730009));
#45015=CARTESIAN_POINT('Ctrl Pts',(19.4244732636406,14.1412090431187,36.2586022016742));
#45016=CARTESIAN_POINT('Ctrl Pts',(19.4443985677122,14.1398258608876,36.2524925259179));
#45017=CARTESIAN_POINT('Ctrl Pts',(19.6252695505569,14.1272354607431,36.2002227601991));
#45018=CARTESIAN_POINT('Ctrl Pts',(19.7914583679699,14.1153272214476,36.1748860704946));
#45019=CARTESIAN_POINT('Ctrl Pts',(20.0299828443551,14.0983175489016,36.1697888308123));
#45020=CARTESIAN_POINT('Ctrl Pts',(20.1012163382998,14.0932624730263,36.1722109059716));
#45021=CARTESIAN_POINT('Ctrl Pts',(20.2045896030247,14.0860881045754,36.181472969214));
#45022=CARTESIAN_POINT('Ctrl Pts',(20.2369458372837,14.083866151986,36.1851997880184));
#45023=CARTESIAN_POINT('Ctrl Pts',(20.2765252366262,14.0811893805295,36.190777341895));
#45024=CARTESIAN_POINT('Ctrl Pts',(20.2838501740516,14.0806957358182,36.1918526137187));
#45025=CARTESIAN_POINT('Ctrl Pts',(20.2952841830029,14.0799280868499,36.1935983794985));
#45026=CARTESIAN_POINT('Ctrl Pts',(20.2993974853126,14.0796525212811,36.1942400376794));
#45027=CARTESIAN_POINT('Ctrl Pts',(20.3070218471814,14.079142872763,36.1954547005856));
#45028=CARTESIAN_POINT('Ctrl Pts',(20.3105333690153,14.0789085981258,36.1960240969901));
#45029=CARTESIAN_POINT('Ctrl Pts',(20.3184891109961,14.0783788320141,36.1973367230223));
#45030=CARTESIAN_POINT('Ctrl Pts',(20.3229323063404,14.0780836730877,36.1980858100528));
#45031=CARTESIAN_POINT('Ctrl Pts',(20.3364071948248,14.0771905868003,36.2004061500026));
#45032=CARTESIAN_POINT('Ctrl Pts',(20.3454305106529,14.076595329195,36.2020262472717));
#45033=CARTESIAN_POINT('Ctrl Pts',(20.4619723023775,14.0689392873396,36.2238094857254));
#45034=CARTESIAN_POINT('Ctrl Pts',(20.5676157177188,14.0623470837316,36.2530216340581));
#45035=CARTESIAN_POINT('Ctrl Pts',(20.7485112528232,14.0508043559172,36.3200439956306));
#45036=CARTESIAN_POINT('Ctrl Pts',(20.8248305511398,14.0458478009006,36.3541000587445));
#45037=CARTESIAN_POINT('Ctrl Pts',(20.9681151109353,14.0360335254723,36.4295361639827));
#45038=CARTESIAN_POINT('Ctrl Pts',(21.035227516728,14.0311972764296,36.4702766661915));
#45039=CARTESIAN_POINT('Ctrl Pts',(21.1153741593196,14.0249963414926,36.5258817016223));
#45040=CARTESIAN_POINT('Ctrl Pts',(21.130916007199,14.0237729547481,36.5370102765727));
#45041=CARTESIAN_POINT('Ctrl Pts',(21.1532003677679,14.0219869013892,36.5534731508901));
#45042=CARTESIAN_POINT('Ctrl Pts',(21.1600769619241,14.021431257288,36.5586246979634));
#45043=CARTESIAN_POINT('Ctrl Pts',(21.1720496595552,14.0204558095169,36.5677194550205));
#45044=CARTESIAN_POINT('Ctrl Pts',(21.1771608858139,14.0200367915553,36.5716426071693));
#45045=CARTESIAN_POINT('Ctrl Pts',(21.1870327449106,14.0192224012284,36.5792987087563));
#45046=CARTESIAN_POINT('Ctrl Pts',(21.1917956665112,14.0188271525539,36.5830285953364));
#45047=CARTESIAN_POINT('Ctrl Pts',(21.2031198990285,14.0178817996629,36.5919829540234));
#45048=CARTESIAN_POINT('Ctrl Pts',(21.2096647926734,14.0173308869573,36.5972278988443));
#45049=CARTESIAN_POINT('Ctrl Pts',(21.2330758015869,14.0153437010099,36.6162410399895));
#45050=CARTESIAN_POINT('Ctrl Pts',(21.2497422252132,14.01389775736,36.6302514198873));
#45051=CARTESIAN_POINT('Ctrl Pts',(21.3811355477787,14.0022403833949,36.7445561670811));
#45052=CARTESIAN_POINT('Ctrl Pts',(21.4838267992947,13.991462126117,36.8578230281235));
#45053=CARTESIAN_POINT('Ctrl Pts',(21.619498044531,13.9747577900388,37.0485938896644));
#45054=CARTESIAN_POINT('Ctrl Pts',(21.662606269588,13.9689268555469,37.1181798581264));
#45055=CARTESIAN_POINT('Ctrl Pts',(21.7180230246129,13.9607839693108,37.2218105774161));
#45056=CARTESIAN_POINT('Ctrl Pts',(21.7339981539065,13.9583411301057,37.2537904646497));
#45057=CARTESIAN_POINT('Ctrl Pts',(21.7522039706805,13.9554511970229,37.2929196073081));
#45058=CARTESIAN_POINT('Ctrl Pts',(21.7552925920212,13.9549569224629,37.2996591751505));
#45059=CARTESIAN_POINT('Ctrl Pts',(21.7600450457539,13.9541902656215,37.3101891833869));
#45060=CARTESIAN_POINT('Ctrl Pts',(21.761735618768,13.9539163062687,37.3139673674167));
#45061=CARTESIAN_POINT('Ctrl Pts',(21.7648575868329,13.9534081053938,37.3210051806488));
#45062=CARTESIAN_POINT('Ctrl Pts',(21.7662921059007,13.9531736817022,37.3242633002542));
#45063=CARTESIAN_POINT('Ctrl Pts',(21.7695350504108,13.9526416316915,37.3316843994367));
#45064=CARTESIAN_POINT('Ctrl Pts',(21.77133780582,13.9523443499583,37.3358497952535));
#45065=CARTESIAN_POINT('Ctrl Pts',(21.7768025517078,13.951438408351,37.3485997390255));
#45066=CARTESIAN_POINT('Ctrl Pts',(21.7804170278818,13.950832532164,37.3572046881782));
#45067=CARTESIAN_POINT('Ctrl Pts',(21.8148224506742,13.9449964094858,37.4408075151127));
#45068=CARTESIAN_POINT('Ctrl Pts',(21.8409234212904,13.9400212580426,37.5176601423191));
#45069=CARTESIAN_POINT('Ctrl Pts',(21.9049342675449,13.9252348430738,37.7541292447737));
#45070=CARTESIAN_POINT('Ctrl Pts',(21.9274222354392,13.9156757004248,37.9171232414008));
#45071=CARTESIAN_POINT('Ctrl Pts',(21.929423274001,13.9029944418731,38.120273014458));
#45072=CARTESIAN_POINT('Ctrl Pts',(21.9286106211337,13.9005113279489,38.1595474469649));
#45073=CARTESIAN_POINT('Ctrl Pts',(21.9260214645185,13.8972658657942,38.2100525210719));
#45074=CARTESIAN_POINT('Ctrl Pts',(21.9253438161285,13.8965377090272,38.2213318591557));
#45075=CARTESIAN_POINT('Ctrl Pts',(21.9240863394978,13.8953538308932,38.2395823709361));
#45076=CARTESIAN_POINT('Ctrl Pts',(21.9235676096224,13.8949000144599,38.2465575968564));
#45077=CARTESIAN_POINT('Ctrl Pts',(21.9225012326045,13.8940283646176,38.2599143202236));
#45078=CARTESIAN_POINT('Ctrl Pts',(21.9219597142393,13.8936107277599,38.2662962247473));
#45079=CARTESIAN_POINT('Ctrl Pts',(21.9206530422187,13.8926565514477,38.2808357831492));
#45080=CARTESIAN_POINT('Ctrl Pts',(21.9198676820002,13.8921193886916,38.2889914526473));
#45081=CARTESIAN_POINT('Ctrl Pts',(21.9176563734879,13.8906964061911,38.3105169179353));
#45082=CARTESIAN_POINT('Ctrl Pts',(21.9161425817499,13.8898078648995,38.3238770431184));
#45083=CARTESIAN_POINT('Ctrl Pts',(21.9034900731792,13.8829745426769,38.4259894071141));
#45084=CARTESIAN_POINT('Ctrl Pts',(21.8863320196529,13.8768416051837,38.5138730038096));
#45085=CARTESIAN_POINT('Ctrl Pts',(21.8211460277485,13.8592091140062,38.7566586608354));
#45086=CARTESIAN_POINT('Ctrl Pts',(21.7596220350663,13.8474123461747,38.9071557708579));
#45087=CARTESIAN_POINT('Ctrl Pts',(21.665192058352,13.8341652053685,39.0744682109062));
#45088=CARTESIAN_POINT('Ctrl Pts',(21.6497468646515,13.832110666802,39.1003941313301));
#45089=CARTESIAN_POINT('Ctrl Pts',(21.6299525628263,13.8296202482447,39.1319141535314));
#45090=CARTESIAN_POINT('Ctrl Pts',(21.62617361565,13.8291508679072,39.1378591199517));
#45091=CARTESIAN_POINT('Ctrl Pts',(21.6201664356084,13.8284143657695,39.1471961353276));
#45092=CARTESIAN_POINT('Ctrl Pts',(21.6179599648291,13.828145858025,39.1506020073663));
#45093=CARTESIAN_POINT('Ctrl Pts',(21.6137909162434,13.8276423278268,39.1569929979081));
#45094=CARTESIAN_POINT('Ctrl Pts',(21.6118308168242,13.827407156092,39.1599795928037));
#45095=CARTESIAN_POINT('Ctrl Pts',(21.6073354661182,13.8268713419989,39.1667878363475));
#45096=CARTESIAN_POINT('Ctrl Pts',(21.6047948776525,13.8265710588392,39.1706058986159));
#45097=CARTESIAN_POINT('Ctrl Pts',(21.5980193327871,13.8257768188965,39.1807100524044));
#45098=CARTESIAN_POINT('Ctrl Pts',(21.59376085241,13.8252843835983,39.1869803840118));
#45099=CARTESIAN_POINT('Ctrl Pts',(21.5635419317525,13.8218358216206,39.2309163575541));
#45100=CARTESIAN_POINT('Ctrl Pts',(21.5362835463843,13.8189603373178,39.2676766743053));
#45101=CARTESIAN_POINT('Ctrl Pts',(21.4892080064309,13.8143005540875,39.3266559071788));
#45102=CARTESIAN_POINT('Ctrl Pts',(21.4701400281522,13.8124878749912,39.3494453277702));
#45103=CARTESIAN_POINT('Ctrl Pts',(21.3409390494567,13.8006189396445,39.4968072400247));
#45104=CARTESIAN_POINT('Ctrl Pts',(21.2156288217498,13.7909500406133,39.607128204402));
#45105=CARTESIAN_POINT('Ctrl Pts',(21.0418509349754,13.7779119308769,39.7241797440317));
#45106=CARTESIAN_POINT('Ctrl Pts',(21.0051785159135,13.775183260718,39.7471274742549));
#45107=CARTESIAN_POINT('Ctrl Pts',(20.9576682450241,13.7716605572902,39.7746791927508));
#45108=CARTESIAN_POINT('Ctrl Pts',(20.9475157037163,13.7709085097926,39.7804442411589));
#45109=CARTESIAN_POINT('Ctrl Pts',(20.9311256542882,13.7696952825597,39.7895554635599));
#45110=CARTESIAN_POINT('Ctrl Pts',(20.9249208641306,13.7692361873095,39.7929601417061));
#45111=CARTESIAN_POINT('Ctrl Pts',(20.9130837988498,13.7683606622248,39.7993708514347));
#45112=CARTESIAN_POINT('Ctrl Pts',(20.9074550506823,13.7679444635435,39.8023832247121));
#45113=CARTESIAN_POINT('Ctrl Pts',(20.8945893904619,13.7669933972063,39.8091866849455));
#45114=CARTESIAN_POINT('Ctrl Pts',(20.8873431790587,13.7664579092037,39.8129598304228));
#45115=CARTESIAN_POINT('Ctrl Pts',(20.8684419560345,13.7650614596873,39.8226496946919));
#45116=CARTESIAN_POINT('Ctrl Pts',(20.8567505475633,13.7641980057753,39.8284941095206));
#45117=CARTESIAN_POINT('Ctrl Pts',(20.7760919478953,13.7582422830106,39.8677951336482));
#45118=CARTESIAN_POINT('Ctrl Pts',(20.7052521195398,13.7530134473972,39.8972298401828));
#45119=CARTESIAN_POINT('Ctrl Pts',(20.475157394538,13.7360379959209,39.9771351487719));
#45120=CARTESIAN_POINT('Ctrl Pts',(20.311035843168,13.7238766857764,40.0111933586574));
#45121=CARTESIAN_POINT('Ctrl Pts',(20.1068790790113,13.7096664930776,40.0265382302504));
#45122=CARTESIAN_POINT('Ctrl Pts',(20.0690899643947,13.7070780253914,40.0282633986948));
#45123=CARTESIAN_POINT('Ctrl Pts',(20.0237388025867,13.7040400240934,40.0289986482153));
#45124=CARTESIAN_POINT('Ctrl Pts',(20.0162051534916,13.7035376244872,40.0290766478204));
#45125=CARTESIAN_POINT('Ctrl Pts',(20.0045058264873,13.7027611452615,40.0291292347054));
#45126=CARTESIAN_POINT('Ctrl Pts',(20.0003404646575,13.7024854239596,40.0291344669476));
#45127=CARTESIAN_POINT('Ctrl Pts',(19.9926178768566,13.7019756335411,40.0291191551665));
#45128=CARTESIAN_POINT('Ctrl Pts',(19.9890607546178,13.7017413718175,40.0291022637049));
#45129=CARTESIAN_POINT('Ctrl Pts',(19.9810010089807,13.7012118201667,40.0290416972593));
#45130=CARTESIAN_POINT('Ctrl Pts',(19.9764984878256,13.7009168616498,40.0289920972794));
#45131=CARTESIAN_POINT('Ctrl Pts',(19.9628453795154,13.7000249838259,40.0287938834603));
#45132=CARTESIAN_POINT('Ctrl Pts',(19.9536954758066,13.6994307236876,40.0285959166591));
#45133=CARTESIAN_POINT('Ctrl Pts',(19.8346460323971,13.6917396764961,40.0251724227426));
#45134=CARTESIAN_POINT('Ctrl Pts',(19.7251981713305,13.6851163589902,40.0126218327514));
#45135=CARTESIAN_POINT('Ctrl Pts',(19.5347554325774,13.6734915660326,39.9740864936778));
#45136=CARTESIAN_POINT('Ctrl Pts',(19.4532950810222,13.668485206967,39.9519627307868));
#45137=CARTESIAN_POINT('Ctrl Pts',(19.300434521341,13.6586837507401,39.8994793924129));
#45138=CARTESIAN_POINT('Ctrl Pts',(19.2289057456295,13.6539150639549,39.8700083417161));
#45139=CARTESIAN_POINT('Ctrl Pts',(19.1422715753804,13.6477953524673,39.8280637265226));
#45140=CARTESIAN_POINT('Ctrl Pts',(19.125323753237,13.6465813110532,39.8195475323259));
#45141=CARTESIAN_POINT('Ctrl Pts',(19.1009088277112,13.6448064414409,39.8068248258356));
#45142=CARTESIAN_POINT('Ctrl Pts',(19.0933394854519,13.6442525112324,39.8028160880288));
#45143=CARTESIAN_POINT('Ctrl Pts',(19.0801270563051,13.6432790486247,39.795705689688));
#45144=CARTESIAN_POINT('Ctrl Pts',(19.0744722944561,13.6428602921241,39.7926259135379));
#45145=CARTESIAN_POINT('Ctrl Pts',(19.0635281858917,13.6420456522766,39.7865941387933));
#45146=CARTESIAN_POINT('Ctrl Pts',(19.0582371093959,13.641649889068,39.7836454211349));
#45147=CARTESIAN_POINT('Ctrl Pts',(19.0456275562015,13.6407020836127,39.7765400778502));
#45148=CARTESIAN_POINT('Ctrl Pts',(19.0383222721577,13.6401492232894,39.7723604091534));
#45149=CARTESIAN_POINT('Ctrl Pts',(19.0120565621523,13.6381476851336,39.7571036533601));
#45150=CARTESIAN_POINT('Ctrl Pts',(18.9932588554332,13.6366891534786,39.7457511825473));
#45151=CARTESIAN_POINT('Ctrl Pts',(18.8480624751101,13.6252131409166,39.6546444792358));
#45152=CARTESIAN_POINT('Ctrl Pts',(18.7311489735664,13.6146529975257,39.5607805287003));
#45153=CARTESIAN_POINT('Ctrl Pts',(18.5673877571369,13.5980086351894,39.394679974854));
#45154=CARTESIAN_POINT('Ctrl Pts',(18.5124682596127,13.5920240549374,39.3311884934657));
#45155=CARTESIAN_POINT('Ctrl Pts',(18.4399708836711,13.5836973552639,39.2354145052578));
#45156=CARTESIAN_POINT('Ctrl Pts',(18.4189070358755,13.5812183819914,39.2058943882269));
#45157=CARTESIAN_POINT('Ctrl Pts',(18.394534960865,13.5782916260778,39.1696167442398));
#45158=CARTESIAN_POINT('Ctrl Pts',(18.3904194147332,13.5777952799965,39.1634135204228));
#45159=CARTESIAN_POINT('Ctrl Pts',(18.3840678490589,13.577026117915,39.1537186664927));
#45160=CARTESIAN_POINT('Ctrl Pts',(18.3818070586116,13.5767517084751,39.150243471679));
#45161=CARTESIAN_POINT('Ctrl Pts',(18.3776262019851,13.5762431049307,39.1437712797646));
#45162=CARTESIAN_POINT('Ctrl Pts',(18.3757032442635,13.5760087259825,39.1407762845968));
#45163=CARTESIAN_POINT('Ctrl Pts',(18.3713519839047,13.5754773294615,39.1339577899366));
#45164=CARTESIAN_POINT('Ctrl Pts',(18.3689288550081,13.5751806530446,39.1301310560846));
#45165=CARTESIAN_POINT('Ctrl Pts',(18.3615793107461,13.5742783874152,39.1184333177141));
#45166=CARTESIAN_POINT('Ctrl Pts',(18.356696137072,13.5736755490665,39.1105351058001));
#45167=CARTESIAN_POINT('Ctrl Pts',(18.3120974267784,13.5681353738897,39.03722138046));
#45168=CARTESIAN_POINT('Ctrl Pts',(18.2762451042946,13.5634250517028,38.9695234816367));
#45169=CARTESIAN_POINT('Ctrl Pts',(18.1977738219659,13.5519773257749,38.7972999057954));
#45170=CARTESIAN_POINT('Ctrl Pts',(18.1601192794525,13.545346309984,38.6908351663647));
#45171=CARTESIAN_POINT('Ctrl Pts',(18.1170861024548,13.5349163872611,38.5239498236574));
#45172=CARTESIAN_POINT('Ctrl Pts',(18.1048832695978,13.5312631084513,38.4655542460667));
#45173=CARTESIAN_POINT('Ctrl Pts',(18.0916107487005,13.5260380016165,38.3831298721843));
#45174=CARTESIAN_POINT('Ctrl Pts',(18.0882544864497,13.5245325476312,38.3595015896524));
#45175=CARTESIAN_POINT('Ctrl Pts',(18.0831320914044,13.5218656593165,38.3179116240109));
#45176=CARTESIAN_POINT('Ctrl Pts',(18.0811780451344,13.5207100359022,38.2999758116383));
#45177=CARTESIAN_POINT('Ctrl Pts',(18.0786838709592,13.5190052402117,38.2736587327016));
#45178=CARTESIAN_POINT('Ctrl Pts',(18.0779464133546,13.5184622123355,38.2652967923427));
#45179=CARTESIAN_POINT('Ctrl Pts',(18.0767418359538,13.5175012877753,38.2505381179601));
#45180=CARTESIAN_POINT('Ctrl Pts',(18.0762519940819,13.5170841049667,38.244143326596));
#45181=CARTESIAN_POINT('Ctrl Pts',(18.0753577620025,13.5162675150875,38.2316516154254));
#45182=CARTESIAN_POINT('Ctrl Pts',(18.0749504322072,13.5158682047112,38.2255549769141));
#45183=CARTESIAN_POINT('Ctrl Pts',(18.0739305071454,13.5147893497022,38.2091155940957));
#45184=CARTESIAN_POINT('Ctrl Pts',(18.0733722663082,13.5141081239309,38.1987697973994));
#45185=CARTESIAN_POINT('Ctrl Pts',(18.0716010841214,13.5115575378631,38.1601671838289));
#45186=CARTESIAN_POINT('Ctrl Pts',(18.0709263040178,13.5096716246729,38.1318904507338));
#45187=CARTESIAN_POINT('Ctrl Pts',(18.0708705914026,13.5076665792831,38.1021211705687));
#45188=CARTESIAN_POINT('Ctrl Pts',(18.0708695284367,13.5075662293439,38.1006320175785));
#45189=CARTESIAN_POINT('Ctrl Pts',(18.0708907846761,13.5043414775085,38.0528025588322));
#45190=CARTESIAN_POINT('Ctrl Pts',(18.0725810774865,13.5011680464547,38.006481683527));
#45191=CARTESIAN_POINT('Ctrl Pts',(18.0829799114519,13.4912057006306,37.8632915999895));
#45192=CARTESIAN_POINT('Ctrl Pts',(18.0973439892374,13.4842805306195,37.766992648821));
#45193=CARTESIAN_POINT('Ctrl Pts',(18.1286691419385,13.474201116631,37.6292528833835));
#45194=CARTESIAN_POINT('Ctrl Pts',(18.1399031679281,13.4710607735314,37.5866560953272));
#45195=CARTESIAN_POINT('Ctrl Pts',(18.1724034023549,13.4630787192221,37.4785745757789));
#45196=CARTESIAN_POINT('Ctrl Pts',(18.1957363603164,13.4582783704154,37.4137684033061));
#45197=CARTESIAN_POINT('Ctrl Pts',(18.2260593482032,13.4530352735776,37.3418696283535));
#45198=CARTESIAN_POINT('Ctrl Pts',(18.2296929501473,13.4524206844592,37.3334231584612));
#45199=CARTESIAN_POINT('Ctrl Pts',(18.2351992186039,13.4515097658556,37.3208715700381));
#45200=CARTESIAN_POINT('Ctrl Pts',(18.2370260550778,13.451210789539,37.3167466700077));
#45201=CARTESIAN_POINT('Ctrl Pts',(18.2403194752569,13.4506775988557,37.3093802016011));
#45202=CARTESIAN_POINT('Ctrl Pts',(18.2417805669996,13.4504430594559,37.3061362579796));
#45203=CARTESIAN_POINT('Ctrl Pts',(18.2449691179403,13.4499355509745,37.2991089606773));
#45204=CARTESIAN_POINT('Ctrl Pts',(18.2466998357794,13.4496627837764,37.2953271541788));
#45205=CARTESIAN_POINT('Ctrl Pts',(18.2515877793142,13.4488998752378,37.284737108301));
#45206=CARTESIAN_POINT('Ctrl Pts',(18.2547725644857,13.4484113819329,37.277941559953));
#45207=CARTESIAN_POINT('Ctrl Pts',(18.2740222383722,13.4455084106901,37.2374835977458));
#45208=CARTESIAN_POINT('Ctrl Pts',(18.2910222341674,13.4431474095355,37.2042716832809));
#45209=CARTESIAN_POINT('Ctrl Pts',(18.3865858704374,13.4307822465975,37.0302137604338));
#45210=CARTESIAN_POINT('Ctrl Pts',(18.4816193707039,13.421451897999,36.8991343559337));
#45211=CARTESIAN_POINT('Ctrl Pts',(18.6482753897287,13.4066556838582,36.7211621307233));
#45212=CARTESIAN_POINT('Ctrl Pts',(18.7084850091553,13.4015534488396,36.6646116362718));
#45213=CARTESIAN_POINT('Ctrl Pts',(18.782341260351,13.3954357956097,36.6036627366104));
#45214=CARTESIAN_POINT('Ctrl Pts',(18.7926439950767,13.3945854980515,36.5953374214171));
#45215=CARTESIAN_POINT('Ctrl Pts',(18.8094797635608,13.3932005389319,36.5820172159));
#45216=CARTESIAN_POINT('Ctrl Pts',(18.8159605503241,13.3926684769468,36.5769567490174));
#45217=CARTESIAN_POINT('Ctrl Pts',(18.8275353788711,13.3917199827977,36.5680371712818));
#45218=CARTESIAN_POINT('Ctrl Pts',(18.8326166490525,13.3913042026741,36.5641616274272));
#45219=CARTESIAN_POINT('Ctrl Pts',(18.8433432649051,13.3904276956455,36.5560642996642));
#45220=CARTESIAN_POINT('Ctrl Pts',(18.8489926716681,13.3899667610494,36.5518480767304));
#45221=CARTESIAN_POINT('Ctrl Pts',(18.863957070886,13.3887475688915,36.5408071431221));
#45222=CARTESIAN_POINT('Ctrl Pts',(18.873310338234,13.3879873049897,36.5340350265729));
#45223=CARTESIAN_POINT('Ctrl Pts',(18.9168440532029,13.3844563776115,36.5031069057664));
#45224=CARTESIAN_POINT('Ctrl Pts',(18.95174183085,13.3816470890907,36.4799849659832));
#45225=CARTESIAN_POINT('Ctrl Pts',(19.1151742340503,13.3685749248996,36.3791934439524));
#45226=CARTESIAN_POINT('Ctrl Pts',(19.2516913052596,13.3578316580854,36.3156016048513));
#45227=CARTESIAN_POINT('Ctrl Pts',(19.3941040122264,13.3471516131145,36.2684889820425));
#45228=CARTESIAN_POINT('',(18.0708702075028,13.336361172809,38.0991052376092));
#45229=CARTESIAN_POINT('Ctrl Pts',(19.3941040017606,13.1771182491666,36.2684889855047));
#45230=CARTESIAN_POINT('Ctrl Pts',(19.295739838268,13.1845070632129,36.3010295777036));
#45231=CARTESIAN_POINT('Ctrl Pts',(19.2001359782007,13.1918587964505,36.3414484626243));
#45232=CARTESIAN_POINT('Ctrl Pts',(19.1000991907493,13.1994385856499,36.3935987976581));
#45233=CARTESIAN_POINT('Ctrl Pts',(19.0920034783272,13.2000510867163,36.3978928192897));
#45234=CARTESIAN_POINT('Ctrl Pts',(19.0799737026927,13.2009595240691,36.4043837506301));
#45235=CARTESIAN_POINT('Ctrl Pts',(19.0760163839233,13.201258086554,36.4065369413214));
#45236=CARTESIAN_POINT('Ctrl Pts',(19.0691686469783,13.2017741891633,36.4102939678087));
#45237=CARTESIAN_POINT('Ctrl Pts',(19.0662747790067,13.2019921284975,36.4118913852251));
#45238=CARTESIAN_POINT('Ctrl Pts',(19.0633726770854,13.2022105165394,36.413503093668));
#45239=CARTESIAN_POINT('Ctrl Pts',(19.0633603915884,13.2022114410407,36.4135099167051));
#45240=CARTESIAN_POINT('Ctrl Pts',(19.0633360823957,13.2022132703363,36.4135234177293));
#45241=CARTESIAN_POINT('Ctrl Pts',(19.0633240588882,13.2022141751166,36.4135300956046));
#45242=CARTESIAN_POINT('Ctrl Pts',(19.0633002687762,13.2022159653394,36.4135433090036));
#45243=CARTESIAN_POINT('Ctrl Pts',(19.0632885019325,13.2022168507999,36.4135498446532));
#45244=CARTESIAN_POINT('Ctrl Pts',(19.0632662162387,13.2022185278036,36.4135622230853));
#45245=CARTESIAN_POINT('Ctrl Pts',(19.0632556979489,13.2022193193052,36.4135680655243));
#45246=CARTESIAN_POINT('Ctrl Pts',(19.0632347137632,13.2022208983612,36.4135797215566));
#45247=CARTESIAN_POINT('Ctrl Pts',(19.0632242476582,13.2022216859315,36.4135855352649));
#45248=CARTESIAN_POINT('Ctrl Pts',(19.0632033681448,13.2022232571023,36.4135971336639));
#45249=CARTESIAN_POINT('Ctrl Pts',(19.0631929541759,13.202224040745,36.4136029186647));
#45250=CARTESIAN_POINT('Ctrl Pts',(19.0631721779797,13.2022256041326,36.4136144601755));
#45251=CARTESIAN_POINT('Ctrl Pts',(19.0631618156603,13.2022263838844,36.4136202167354));
#45252=CARTESIAN_POINT('Ctrl Pts',(19.0631411424176,13.2022279395163,36.4136317015526));
#45253=CARTESIAN_POINT('Ctrl Pts',(19.0631308313712,13.2022287154056,36.413637429877));
#45254=CARTESIAN_POINT('Ctrl Pts',(19.0631102607706,13.2022302633054,36.4136488581661));
#45255=CARTESIAN_POINT('Ctrl Pts',(19.063100000887,13.2022310353406,36.4136545583126));
#45256=CARTESIAN_POINT('Ctrl Pts',(19.0630795320652,13.2022325755732,36.413665930546));
#45257=CARTESIAN_POINT('Ctrl Pts',(19.063069323209,13.2022333437646,36.4136716025861));
#45258=CARTESIAN_POINT('Ctrl Pts',(19.0630489543621,13.2022348764661,36.4136829197588));
#45259=CARTESIAN_POINT('Ctrl Pts',(19.0630387954007,13.2022356408988,36.4136885643183));
#45260=CARTESIAN_POINT('Ctrl Pts',(19.0630185283358,13.2022371659333,36.4136998254191));
#45261=CARTESIAN_POINT('Ctrl Pts',(19.063008419748,13.2022379265714,36.4137054422282));
#45262=CARTESIAN_POINT('Ctrl Pts',(19.0629882517581,13.2022394441427,36.4137166487541));
#45263=CARTESIAN_POINT('Ctrl Pts',(19.0629781927242,13.202240201048,36.413722238265));
#45264=CARTESIAN_POINT('Ctrl Pts',(19.0629581244126,13.2022417111108,36.4137333898737));
#45265=CARTESIAN_POINT('Ctrl Pts',(19.0629481148217,13.2022424642917,36.4137389521444));
#45266=CARTESIAN_POINT('Ctrl Pts',(19.06292814557,13.2022439668926,36.4137500491727));
#45267=CARTESIAN_POINT('Ctrl Pts',(19.0629181855005,13.2022447163433,36.4137555841562));
#45268=CARTESIAN_POINT('Ctrl Pts',(19.0628983132665,13.2022462116361,36.4137666277322));
#45269=CARTESIAN_POINT('Ctrl Pts',(19.0628884017446,13.2022469574299,36.4137721359663));
#45270=CARTESIAN_POINT('Ctrl Pts',(19.0628686276627,13.2022484453295,36.4137831254526));
#45271=CARTESIAN_POINT('Ctrl Pts',(19.062858764783,13.2022491874593,36.4137886068813));
#45272=CARTESIAN_POINT('Ctrl Pts',(19.0592991190886,13.2025170313741,36.4157669689827));
#45273=CARTESIAN_POINT('Ctrl Pts',(19.0557555344542,13.2027834157959,36.4177510766372));
#45274=CARTESIAN_POINT('Ctrl Pts',(19.0459716788548,13.2035182838886,36.4232698627054));
#45275=CARTESIAN_POINT('Ctrl Pts',(19.0397447335202,13.2039852904599,36.4268282162327));
#45276=CARTESIAN_POINT('Ctrl Pts',(19.025819094879,13.2050284376012,36.4348892948614));
#45277=CARTESIAN_POINT('Ctrl Pts',(19.0181314375016,13.2056034476988,36.4394108788538));
#45278=CARTESIAN_POINT('Ctrl Pts',(18.9942489272227,13.2073879755422,36.4536814895117));
#45279=CARTESIAN_POINT('Ctrl Pts',(18.9781653257,13.2085871581053,36.4636156273978));
#45280=CARTESIAN_POINT('Ctrl Pts',(18.9148369702489,13.2133092053696,36.5040286632081));
#45281=CARTESIAN_POINT('Ctrl Pts',(18.8687851716678,13.2167441774213,36.5363321005163));
#45282=CARTESIAN_POINT('Ctrl Pts',(18.7777021688406,13.223680186999,36.6063562868535));
#45283=CARTESIAN_POINT('Ctrl Pts',(18.7328511649458,13.2271742182929,36.6442123598367));
#45284=CARTESIAN_POINT('Ctrl Pts',(18.596959891002,13.2382351795582,36.7699555364346));
#45285=CARTESIAN_POINT('Ctrl Pts',(18.5128104311542,13.2458354397861,36.8647666324445));
#45286=CARTESIAN_POINT('Ctrl Pts',(18.4253787922848,13.2552633350704,36.9852742463396));
#45287=CARTESIAN_POINT('Ctrl Pts',(18.412527513997,13.2566946027963,37.0036531145008));
#45288=CARTESIAN_POINT('Ctrl Pts',(18.3947323252872,13.258744823538,37.0300714264242));
#45289=CARTESIAN_POINT('Ctrl Pts',(18.3895221857977,13.2593538163374,37.0379300094492));
#45290=CARTESIAN_POINT('Ctrl Pts',(18.3811265251355,13.2603496703628,37.0507972271508));
#45291=CARTESIAN_POINT('Ctrl Pts',(18.3779060990942,13.2607352324195,37.0557829911789));
#45292=CARTESIAN_POINT('Ctrl Pts',(18.3711925172954,13.2615466017112,37.0662827528582));
#45293=CARTESIAN_POINT('Ctrl Pts',(18.3677042418526,13.2619725819766,37.0717997671009));
#45294=CARTESIAN_POINT('Ctrl Pts',(18.3594317258841,13.2629934777316,37.0850316740258));
#45295=CARTESIAN_POINT('Ctrl Pts',(18.3546738461803,13.2635893459159,37.0927627848549));
#45296=CARTESIAN_POINT('Ctrl Pts',(18.3386112457111,13.2656312718369,37.1192805219571));
#45297=CARTESIAN_POINT('Ctrl Pts',(18.3275726692109,13.2670868692993,37.1382255754771));
#45298=CARTESIAN_POINT('Ctrl Pts',(18.3018981769354,13.2706028747853,37.1840686296835));
#45299=CARTESIAN_POINT('Ctrl Pts',(18.2875754893299,13.2726737486651,37.211134321155));
#45300=CARTESIAN_POINT('Ctrl Pts',(18.234879484166,13.2807351863236,37.3167191823275));
#45301=CARTESIAN_POINT('Ctrl Pts',(18.2012177998712,13.2868703672801,37.397462659485));
#45302=CARTESIAN_POINT('Ctrl Pts',(18.1374569480367,13.3009769688883,37.585397226114));
#45303=CARTESIAN_POINT('Ctrl Pts',(18.1109190123339,13.3089738170708,37.693481761211));
#45304=CARTESIAN_POINT('Ctrl Pts',(18.0897939048198,13.3185267566863,37.8291794622294));
#45305=CARTESIAN_POINT('Ctrl Pts',(18.0862867601388,13.3203353082226,37.8551880976322));
#45306=CARTESIAN_POINT('Ctrl Pts',(18.0818866307341,13.3229758969158,37.8937440804848));
#45307=CARTESIAN_POINT('Ctrl Pts',(18.0805840081068,13.3238254920839,37.9062406881092));
#45308=CARTESIAN_POINT('Ctrl Pts',(18.0785886463918,13.3252514121523,37.927384269676));
#45309=CARTESIAN_POINT('Ctrl Pts',(18.0778319879714,13.3258308641969,37.9360246341787));
#45310=CARTESIAN_POINT('Ctrl Pts',(18.0767742064885,13.326703809504,37.9491191588825));
#45311=CARTESIAN_POINT('Ctrl Pts',(18.0764302402003,13.3269995860633,37.9535696027994));
#45312=CARTESIAN_POINT('Ctrl Pts',(18.0758552968145,13.3275157226276,37.9613604351347));
#45313=CARTESIAN_POINT('Ctrl Pts',(18.0756175671818,13.3277364529654,37.9647002564846));
#45314=CARTESIAN_POINT('Ctrl Pts',(18.0751590355586,13.3281773751392,37.9713878915008));
#45315=CARTESIAN_POINT('Ctrl Pts',(18.0749382724596,13.3283975648136,37.9747356458153));
#45316=CARTESIAN_POINT('Ctrl Pts',(18.0744692701854,13.3288835600262,37.9821420379353));
#45317=CARTESIAN_POINT('Ctrl Pts',(18.0742251264333,13.3291491406976,37.9862009325409));
#45318=CARTESIAN_POINT('Ctrl Pts',(18.0736507023885,13.3298069821556,37.9962824930422));
#45319=CARTESIAN_POINT('Ctrl Pts',(18.0733358282452,13.3301984245531,38.0023060430788));
#45320=CARTESIAN_POINT('Ctrl Pts',(18.0716108636269,13.332545666938,38.0385661124733));
#45321=CARTESIAN_POINT('Ctrl Pts',(18.0708842484705,13.3344667389137,38.0688325647746));
#45322=CARTESIAN_POINT('Ctrl Pts',(18.0708702075028,13.336361172809,38.0991052376092));
#45323=CARTESIAN_POINT('Ctrl Pts',(18.0708702086382,13.3363610198239,38.0991027929391));
#45324=CARTESIAN_POINT('Ctrl Pts',(18.0708489954218,13.3392153506683,38.1447143910078));
#45325=CARTESIAN_POINT('Ctrl Pts',(18.072445425963,13.3420078590196,38.1903161632809));
#45326=CARTESIAN_POINT('Ctrl Pts',(18.0874536075436,13.3549139772547,38.4029540689302));
#45327=CARTESIAN_POINT('Ctrl Pts',(18.1209706118427,13.3646569627379,38.5678291612205));
#45328=CARTESIAN_POINT('Ctrl Pts',(18.1889039431484,13.3776934586107,38.7657419056431));
#45329=CARTESIAN_POINT('Ctrl Pts',(18.2037154102981,13.3803262450693,38.8047286589164));
#45330=CARTESIAN_POINT('Ctrl Pts',(18.2242205707633,13.3837408668965,38.8538454629391));
#45331=CARTESIAN_POINT('Ctrl Pts',(18.2287588969273,13.3844838607765,38.8644478456376));
#45332=CARTESIAN_POINT('Ctrl Pts',(18.2362226172729,13.385685962907,38.881461162125));
#45333=CARTESIAN_POINT('Ctrl Pts',(18.2390885957778,13.3861430554713,38.8878979807245));
#45334=CARTESIAN_POINT('Ctrl Pts',(18.2446213721524,13.387017065147,38.9001432865034));
#45335=CARTESIAN_POINT('Ctrl Pts',(18.2472819041317,13.3874337640563,38.9059545153501));
#45336=CARTESIAN_POINT('Ctrl Pts',(18.2534337497153,13.3883892269867,38.9192170659335));
#45337=CARTESIAN_POINT('Ctrl Pts',(18.2569439403197,13.3889286324031,38.9266594444078));
#45338=CARTESIAN_POINT('Ctrl Pts',(18.2662375189434,13.3903420032177,38.9460414986288));
#45339=CARTESIAN_POINT('Ctrl Pts',(18.272096565465,13.3912185613104,38.9579442080747));
#45340=CARTESIAN_POINT('Ctrl Pts',(18.3155898683635,13.3976234681318,39.0440483131015));
#45341=CARTESIAN_POINT('Ctrl Pts',(18.3578614607377,13.4033136954771,39.1157963937834));
#45342=CARTESIAN_POINT('Ctrl Pts',(18.4729610116639,13.4176301007636,39.2851025333739));
#45343=CARTESIAN_POINT('Ctrl Pts',(18.5506409955429,13.4263810307947,39.3789335177755));
#45344=CARTESIAN_POINT('Ctrl Pts',(18.6726409319254,13.4385976535679,39.5008041971015));
#45345=CARTESIAN_POINT('Ctrl Pts',(18.7100724914958,13.4421716545388,39.5353474354571));
#45346=CARTESIAN_POINT('Ctrl Pts',(18.7623182600264,13.4468883800316,39.5798650344584));
#45347=CARTESIAN_POINT('Ctrl Pts',(18.775965414295,13.4480967986252,39.5911726903452));
#45348=CARTESIAN_POINT('Ctrl Pts',(18.7964000097191,13.4498692698242,39.6076346276636));
#45349=CARTESIAN_POINT('Ctrl Pts',(18.8030685016884,13.450441984569,39.6129342688132));
#45350=CARTESIAN_POINT('Ctrl Pts',(18.8151483506504,13.4514688978372,39.6224046099851));
#45351=CARTESIAN_POINT('Ctrl Pts',(18.8205471340836,13.4519241049869,39.6265910284029));
#45352=CARTESIAN_POINT('Ctrl Pts',(18.8291613906758,13.4526443508002,39.6331978681199));
#45353=CARTESIAN_POINT('Ctrl Pts',(18.8323623317358,13.4529106623808,39.6356370105848));
#45354=CARTESIAN_POINT('Ctrl Pts',(18.838319976088,13.4534038405728,39.6401473850961));
#45355=CARTESIAN_POINT('Ctrl Pts',(18.8410745720454,13.4536308836003,39.6422212222934));
#45356=CARTESIAN_POINT('Ctrl Pts',(18.8474557856805,13.4541545910222,39.6469986592832));
#45357=CARTESIAN_POINT('Ctrl Pts',(18.8510863582522,13.4544508828239,39.6496968937895));
#45358=CARTESIAN_POINT('Ctrl Pts',(18.8621743921037,13.455350819529,39.6578771155848));
#45359=CARTESIAN_POINT('Ctrl Pts',(18.8696619783147,13.4559517342549,39.6633183253148));
#45360=CARTESIAN_POINT('Ctrl Pts',(18.9375845730285,13.4613446940022,39.7119343717222));
#45361=CARTESIAN_POINT('Ctrl Pts',(19.0004346202833,13.4659230425509,39.7516448768358));
#45362=CARTESIAN_POINT('Ctrl Pts',(19.2112031354325,13.4805128720727,39.8683636805306));
#45363=CARTESIAN_POINT('Ctrl Pts',(19.3668180631527,13.4902031167279,39.9298612089557));
#45364=CARTESIAN_POINT('Ctrl Pts',(19.5699004235054,13.5032403955912,39.981060470662));
#45365=CARTESIAN_POINT('Ctrl Pts',(19.6117328526723,13.5059410613468,39.9901381772669));
#45366=CARTESIAN_POINT('Ctrl Pts',(19.6652754877856,13.5094322185521,39.9999045793668));
#45367=CARTESIAN_POINT('Ctrl Pts',(19.6767392135258,13.5101816559981,40.0018886308294));
#45368=CARTESIAN_POINT('Ctrl Pts',(19.6951955133683,13.5113916752244,40.00491121706));
#45369=CARTESIAN_POINT('Ctrl Pts',(19.7021771910167,13.5118501924461,40.0060152392362));
#45370=CARTESIAN_POINT('Ctrl Pts',(19.7154778499266,13.5127252739528,40.0080436278508));
#45371=CARTESIAN_POINT('Ctrl Pts',(19.7217956748935,13.5131416107981,40.0089750369025));
#45372=CARTESIAN_POINT('Ctrl Pts',(19.7362226364188,13.5140939171807,40.0110288005477));
#45373=CARTESIAN_POINT('Ctrl Pts',(19.7443344823529,13.5146305130166,40.0121309352835));
#45374=CARTESIAN_POINT('Ctrl Pts',(19.7654705373687,13.5160317433022,40.0148657345928));
#45375=CARTESIAN_POINT('Ctrl Pts',(19.7785046524799,13.5168988983045,40.0164171380416));
#45376=CARTESIAN_POINT('Ctrl Pts',(19.8695725422199,13.5229798873746,40.0263151719155));
#45377=CARTESIAN_POINT('Ctrl Pts',(19.9480260652365,13.5283371203793,40.0300252040865));
#45378=CARTESIAN_POINT('Ctrl Pts',(20.1916405720254,13.5453334103625,40.0266810675328));
#45379=CARTESIAN_POINT('Ctrl Pts',(20.3558082288573,13.5573630659639,40.0032129851045));
#45380=CARTESIAN_POINT('Ctrl Pts',(20.5512640292596,13.5714384224051,39.9490724026588));
#45381=CARTESIAN_POINT('Ctrl Pts',(20.5872576533532,13.5740158248595,39.937958022169));
#45382=CARTESIAN_POINT('Ctrl Pts',(20.6300274432953,13.5770426054451,39.9233662832219));
#45383=CARTESIAN_POINT('Ctrl Pts',(20.6371352066219,13.5775444071354,39.9208948116692));
#45384=CARTESIAN_POINT('Ctrl Pts',(20.6481528311048,13.5783201634238,39.9169914138822));
#45385=CARTESIAN_POINT('Ctrl Pts',(20.6520727283757,13.5785957549147,39.9155883477024));
#45386=CARTESIAN_POINT('Ctrl Pts',(20.6593334889027,13.5791054263012,39.9129629235679));
#45387=CARTESIAN_POINT('Ctrl Pts',(20.6626754850138,13.5793396980409,39.9117440254431));
#45388=CARTESIAN_POINT('Ctrl Pts',(20.6702424481523,13.5798694257478,39.9089604515167));
#45389=CARTESIAN_POINT('Ctrl Pts',(20.6744653094934,13.5801645493644,39.9073902184543));
#45390=CARTESIAN_POINT('Ctrl Pts',(20.6872613774784,13.5810574251361,39.9025810231823));
#45391=CARTESIAN_POINT('Ctrl Pts',(20.6958171925645,13.5816525093738,39.8992956924009));
#45392=CARTESIAN_POINT('Ctrl Pts',(20.8062320829659,13.5893113493639,39.8559923184681));
#45393=CARTESIAN_POINT('Ctrl Pts',(20.9045465706814,13.5959061146401,39.8074314442493));
#45394=CARTESIAN_POINT('Ctrl Pts',(21.0695968470069,13.6074468153303,39.7076262187894));
#45395=CARTESIAN_POINT('Ctrl Pts',(21.13809549857,13.6123988190635,39.6598838678357));
#45396=CARTESIAN_POINT('Ctrl Pts',(21.2646270248928,13.6222100886688,39.5589104273561));
#45397=CARTESIAN_POINT('Ctrl Pts',(21.3229159928581,13.6270481607459,39.5062689222233));
#45398=CARTESIAN_POINT('Ctrl Pts',(21.3912150425075,13.6332512862093,39.4365735256565));
#45399=CARTESIAN_POINT('Ctrl Pts',(21.4043924341608,13.6344749228778,39.4227206557487));
#45400=CARTESIAN_POINT('Ctrl Pts',(21.4231906273248,13.6362612743164,39.4023612531121));
#45401=CARTESIAN_POINT('Ctrl Pts',(21.4289775331301,13.6368169632218,39.396009105369));
#45402=CARTESIAN_POINT('Ctrl Pts',(21.4390291247481,13.6377924620046,39.3848265456323));
#45403=CARTESIAN_POINT('Ctrl Pts',(21.4433124383181,13.6382114859127,39.3800129991352));
#45404=CARTESIAN_POINT('Ctrl Pts',(21.451570231621,13.6390258673992,39.3706388214836));
#45405=CARTESIAN_POINT('Ctrl Pts',(21.4555475370432,13.6394211011919,39.3660807707246));
#45406=CARTESIAN_POINT('Ctrl Pts',(21.4649873765201,13.6403663856911,39.3551593028287));
#45407=CARTESIAN_POINT('Ctrl Pts',(21.4704299461195,13.6409172446259,39.3487788669928));
#45408=CARTESIAN_POINT('Ctrl Pts',(21.4898487450387,13.6429040433563,39.3257108476849));
#45409=CARTESIAN_POINT('Ctrl Pts',(21.5035834658426,13.6443496486619,39.3088230064279));
#45410=CARTESIAN_POINT('Ctrl Pts',(21.6111534198342,13.6560055780185,39.1718877107781));
#45411=CARTESIAN_POINT('Ctrl Pts',(21.6907333274036,13.6667826130711,39.0413615887572));
#45412=CARTESIAN_POINT('Ctrl Pts',(21.788160134289,13.6834871105829,38.8285018758172));
#45413=CARTESIAN_POINT('Ctrl Pts',(21.8174367900994,13.6893193618148,38.7520405177836));
#45414=CARTESIAN_POINT('Ctrl Pts',(21.8524067692817,13.6974638252642,38.6398233547797));
#45415=CARTESIAN_POINT('Ctrl Pts',(21.862091218629,13.6999069759091,38.6054075457684));
#45416=CARTESIAN_POINT('Ctrl Pts',(21.8726234378143,13.7027972256356,38.563550406144));
#45417=CARTESIAN_POINT('Ctrl Pts',(21.8743910659366,13.7032915172621,38.5563503645383));
#45418=CARTESIAN_POINT('Ctrl Pts',(21.8770808566796,13.7040581942789,38.5451147571212));
#45419=CARTESIAN_POINT('Ctrl Pts',(21.8780315888109,13.7043321568776,38.5410862067083));
#45420=CARTESIAN_POINT('Ctrl Pts',(21.8797758875643,13.7048403599001,38.5335871801471));
#45421=CARTESIAN_POINT('Ctrl Pts',(21.880572806567,13.7050747825164,38.5301175999407));
#45422=CARTESIAN_POINT('Ctrl Pts',(21.8823638931859,13.7056068250852,38.5222195275474));
#45423=CARTESIAN_POINT('Ctrl Pts',(21.8833520383913,13.705904100485,38.5177897274217));
#45424=CARTESIAN_POINT('Ctrl Pts',(21.8863242244484,13.7068100060923,38.5042407347854));
#45425=CARTESIAN_POINT('Ctrl Pts',(21.888257770244,13.7074158529275,38.4951104313992));
#45426=CARTESIAN_POINT('Ctrl Pts',(21.9063357556511,13.7132488512,38.4065802709513));
#45427=CARTESIAN_POINT('Ctrl Pts',(21.9175312420245,13.7182212127513,38.3262408002213));
#45428=CARTESIAN_POINT('Ctrl Pts',(21.9359972793637,13.7330067223166,38.0819784549729));
#45429=CARTESIAN_POINT('Ctrl Pts',(21.9274729233002,13.7425672628078,37.9176332779694));
#45430=CARTESIAN_POINT('Ctrl Pts',(21.8912738612039,13.7552511786532,37.7176784970078));
#45431=CARTESIAN_POINT('Ctrl Pts',(21.8830947958538,13.7577353830588,37.679238547234));
#45432=CARTESIAN_POINT('Ctrl Pts',(21.8710597075914,13.7609820785598,37.6301001714052));
#45433=CARTESIAN_POINT('Ctrl Pts',(21.8682748482875,13.7617103454296,37.6191472567324));
#45434=CARTESIAN_POINT('Ctrl Pts',(21.8636108002008,13.7628943579551,37.6014558488316));
#45435=CARTESIAN_POINT('Ctrl Pts',(21.8617908863542,13.76334819786,37.5947018913116));
#45436=CARTESIAN_POINT('Ctrl Pts',(21.8582343150544,13.7642198625127,37.5817830494051));
#45437=CARTESIAN_POINT('Ctrl Pts',(21.8565036059079,13.7646374905447,37.5756166124614));
#45438=CARTESIAN_POINT('Ctrl Pts',(21.8524891414737,13.7655916046178,37.5615822657654));
#45439=CARTESIAN_POINT('Ctrl Pts',(21.8501859207831,13.766128713682,37.553720098425));
#45440=CARTESIAN_POINT('Ctrl Pts',(21.8439713708303,13.7675514632587,37.532996604485));
#45441=CARTESIAN_POINT('Ctrl Pts',(21.8399756227077,13.7684398238992,37.5201612643735));
#45442=CARTESIAN_POINT('Ctrl Pts',(21.8084002587606,13.7752658657872,37.4223474303605));
#45443=CARTESIAN_POINT('Ctrl Pts',(21.7750855501925,13.7813912376485,37.3393479085504));
#45444=CARTESIAN_POINT('Ctrl Pts',(21.6656600888732,13.7989955722757,37.1134613562713));
#45445=CARTESIAN_POINT('Ctrl Pts',(21.5771689092334,13.8107707837113,36.9774061675487));
#45446=CARTESIAN_POINT('Ctrl Pts',(21.4530375835079,13.8240266108867,36.8306869132449));
#45447=CARTESIAN_POINT('Ctrl Pts',(21.4327743999678,13.8261052686655,36.8078577058324));
#45448=CARTESIAN_POINT('Ctrl Pts',(21.4071596873433,13.8286207206734,36.7803431704839));
#45449=CARTESIAN_POINT('Ctrl Pts',(21.4023141947713,13.8290918015148,36.7751953214397));
#45450=CARTESIAN_POINT('Ctrl Pts',(21.3946389813676,13.8298303656721,36.7671304708519));
#45451=CARTESIAN_POINT('Ctrl Pts',(21.3918282151018,13.8300992476635,36.7641956391424));
#45452=CARTESIAN_POINT('Ctrl Pts',(21.3865298172039,13.8306030843481,36.7586982526915));
#45453=CARTESIAN_POINT('Ctrl Pts',(21.3840443719918,13.8308381906166,36.7561337537022));
#45454=CARTESIAN_POINT('Ctrl Pts',(21.3783572600727,13.8313733548836,36.7502982664452));
#45455=CARTESIAN_POINT('Ctrl Pts',(21.3751510667925,13.8316730568944,36.7470317629303));
#45456=CARTESIAN_POINT('Ctrl Pts',(21.3666261457944,13.8324647425108,36.7384080929788));
#45457=CARTESIAN_POINT('Ctrl Pts',(21.3612874824639,13.832955220183,36.7330706169493));
#45458=CARTESIAN_POINT('Ctrl Pts',(21.3236529755767,13.8363770307189,36.6958836416411));
#45459=CARTESIAN_POINT('Ctrl Pts',(21.2902710545293,13.8392290685353,36.665147635996));
#45460=CARTESIAN_POINT('Ctrl Pts',(21.1516409444714,13.8505101085888,36.546260668394));
#45461=CARTESIAN_POINT('Ctrl Pts',(21.0382032601898,13.8585249811965,36.4682762356855));
#45462=CARTESIAN_POINT('Ctrl Pts',(20.860228107468,13.8707293613139,36.3720589809401));
#45463=CARTESIAN_POINT('Ctrl Pts',(20.8014920038589,13.8746994998026,36.3440438306523));
#45464=CARTESIAN_POINT('Ctrl Pts',(20.7061706074671,13.8811499531319,36.3043590128268));
#45465=CARTESIAN_POINT('Ctrl Pts',(20.6704577325247,13.8835678042471,36.2907212495012));
#45466=CARTESIAN_POINT('Ctrl Pts',(20.6237942155584,13.8867393156911,36.2744730549034));
#45467=CARTESIAN_POINT('Ctrl Pts',(20.6131915946963,13.8874607144765,36.2708843912302));
#45468=CARTESIAN_POINT('Ctrl Pts',(20.5959362441997,13.8886362942413,36.265210871696));
#45469=CARTESIAN_POINT('Ctrl Pts',(20.5893022856478,13.8890886199057,36.2630694170678));
#45470=CARTESIAN_POINT('Ctrl Pts',(20.5765446078646,13.8899592456646,36.2590274356056));
#45471=CARTESIAN_POINT('Ctrl Pts',(20.57042272428,13.8903773592552,36.2571213871565));
#45472=CARTESIAN_POINT('Ctrl Pts',(20.5564103793656,13.8913351990854,36.2528351533583));
#45473=CARTESIAN_POINT('Ctrl Pts',(20.5485139822354,13.8918755655511,36.2504749559208));
#45474=CARTESIAN_POINT('Ctrl Pts',(20.5275388463699,13.8933126264856,36.2443517213357));
#45475=CARTESIAN_POINT('Ctrl Pts',(20.5144351882301,13.8942121295448,36.2406764161148));
#45476=CARTESIAN_POINT('Ctrl Pts',(20.408346861704,13.9015098692605,36.2121281368261));
#45477=CARTESIAN_POINT('Ctrl Pts',(20.3136730499356,13.9081273104651,36.1941113959828));
#45478=CARTESIAN_POINT('Ctrl Pts',(20.1226197140805,13.9216554501872,36.1723760006934));
#45479=CARTESIAN_POINT('Ctrl Pts',(20.0265014590896,13.9285464540461,36.1686621087005));
#45480=CARTESIAN_POINT('Ctrl Pts',(19.8711016849172,13.9396015732736,36.174263250096));
#45481=CARTESIAN_POINT('Ctrl Pts',(19.8118169313951,13.943796212096,36.1791499368758));
#45482=CARTESIAN_POINT('Ctrl Pts',(19.7236330946968,13.9499230948671,36.1905415198447));
#45483=CARTESIAN_POINT('Ctrl Pts',(19.6945057189264,13.9519280547887,36.1949845586013));
#45484=CARTESIAN_POINT('Ctrl Pts',(19.6586043647402,13.9543669138082,36.2013055922326));
#45485=CARTESIAN_POINT('Ctrl Pts',(19.6517255744913,13.9548327238142,36.2025553072365));
#45486=CARTESIAN_POINT('Ctrl Pts',(19.640876391822,13.9555648940217,36.2045873367379));
#45487=CARTESIAN_POINT('Ctrl Pts',(19.6369014904076,13.9558326135998,36.2053447798912));
#45488=CARTESIAN_POINT('Ctrl Pts',(19.6294195347463,13.9563355029707,36.2067949254307));
#45489=CARTESIAN_POINT('Ctrl Pts',(19.6259120641732,13.9565708172079,36.2074848607976));
#45490=CARTESIAN_POINT('Ctrl Pts',(19.6178902793492,13.9571080224161,36.2090859547423));
#45491=CARTESIAN_POINT('Ctrl Pts',(19.6133772980862,13.9574095473211,36.210003531057));
#45492=CARTESIAN_POINT('Ctrl Pts',(19.6013814759793,13.9582092585773,36.2124872785569));
#45493=CARTESIAN_POINT('Ctrl Pts',(19.5939044932465,13.9587058898582,36.2140818031038));
#45494=CARTESIAN_POINT('Ctrl Pts',(19.5400681055324,13.962269880212,36.2258978522188));
#45495=CARTESIAN_POINT('Ctrl Pts',(19.4940861494538,13.9652503128363,36.2377840522972));
#45496=CARTESIAN_POINT('Ctrl Pts',(19.4303355821949,13.969352282064,36.256799603463));
#45497=CARTESIAN_POINT('Ctrl Pts',(19.4121731230477,13.9705174109781,36.2625114023504));
#45498=CARTESIAN_POINT('Ctrl Pts',(19.3941039465104,13.9716756753762,36.2684890037825));
#45499=CARTESIAN_POINT('Origin',(20.,-1.3495818343519,38.1));
#45500=CARTESIAN_POINT('',(19.3941040816519,14.9348319053408,36.2684889590753));
#45501=CARTESIAN_POINT('',(19.3941039945165,14.7625557686229,36.2684889879012));
#45502=CARTESIAN_POINT('',(19.3941040087494,-1.3495818343519,36.2684889831927));
#45503=CARTESIAN_POINT('',(18.0708708463018,14.2998795404039,38.1017114188227));
#45504=CARTESIAN_POINT('Ctrl Pts',(19.3941040816519,14.9348319053408,36.2684889590753));
#45505=CARTESIAN_POINT('Ctrl Pts',(19.4247862302146,14.9328999468963,36.2583387671491));
#45506=CARTESIAN_POINT('Ctrl Pts',(19.4557306857153,14.9309715206932,36.2489571730916));
#45507=CARTESIAN_POINT('Ctrl Pts',(19.6120641793806,14.9212744810258,36.2058234950179));
#45508=CARTESIAN_POINT('Ctrl Pts',(19.7403665114976,14.9134320283775,36.1840191843203));
#45509=CARTESIAN_POINT('Ctrl Pts',(19.8836306306663,14.9042650559825,36.1743336816182));
#45510=CARTESIAN_POINT('Ctrl Pts',(19.897394118544,14.9033805905104,36.1735512939181));
#45511=CARTESIAN_POINT('Ctrl Pts',(19.9194490484728,14.9019567243745,36.172534596882));
#45512=CARTESIAN_POINT('Ctrl Pts',(19.9277358358974,14.9014202445816,36.1722061253688));
#45513=CARTESIAN_POINT('Ctrl Pts',(19.9424403209514,14.9004655467306,36.1717182130495));
#45514=CARTESIAN_POINT('Ctrl Pts',(19.9488572204114,14.9000479999005,36.1715373529738));
#45515=CARTESIAN_POINT('Ctrl Pts',(19.9622199291313,14.8991765102028,36.1712274671801));
#45516=CARTESIAN_POINT('Ctrl Pts',(19.9691657609965,14.8987224031027,36.171103925894));
#45517=CARTESIAN_POINT('Ctrl Pts',(19.9871953287831,14.897540694577,36.1708806528431));
#45518=CARTESIAN_POINT('Ctrl Pts',(19.9982794010565,14.8968113042384,36.1708389268761));
#45519=CARTESIAN_POINT('Ctrl Pts',(20.0465289848394,14.8936231329239,36.171073108807));
#45520=CARTESIAN_POINT('Ctrl Pts',(20.0836796137598,14.8911343032896,36.1723274923241));
#45521=CARTESIAN_POINT('Ctrl Pts',(20.1831060922766,14.8843770745986,36.1785640923564));
#45522=CARTESIAN_POINT('Ctrl Pts',(20.2452108772903,14.880053385642,36.1854989974155));
#45523=CARTESIAN_POINT('Ctrl Pts',(20.4426830809356,14.8660038154632,36.217315832157));
#45524=CARTESIAN_POINT('Ctrl Pts',(20.5757616948277,14.8560450273797,36.2536620669921));
#45525=CARTESIAN_POINT('Ctrl Pts',(20.7218537719816,14.8450634560484,36.3109097158509));
#45526=CARTESIAN_POINT('Ctrl Pts',(20.7397616984407,14.8437171756498,36.3182397492967));
#45527=CARTESIAN_POINT('Ctrl Pts',(20.7861779411219,14.8402323024529,36.3380592175638));
#45528=CARTESIAN_POINT('Ctrl Pts',(20.814501148073,14.8381103958795,36.3509719193962));
#45529=CARTESIAN_POINT('Ctrl Pts',(20.8491387344421,14.8355318017446,36.3677874253341));
#45530=CARTESIAN_POINT('Ctrl Pts',(20.855757680072,14.8350398095165,36.3710477764029));
#45531=CARTESIAN_POINT('Ctrl Pts',(20.8660933994628,14.8342729190881,36.3762128266292));
#45532=CARTESIAN_POINT('Ctrl Pts',(20.8698228843148,14.8339964801779,36.3780917137045));
#45533=CARTESIAN_POINT('Ctrl Pts',(20.8767170161116,14.8334860324997,36.3815930408509));
#45534=CARTESIAN_POINT('Ctrl Pts',(20.87988325262,14.8332518268973,36.3832121081187));
#45535=CARTESIAN_POINT('Ctrl Pts',(20.8870358297812,14.8327232481282,36.3868945913395));
#45536=CARTESIAN_POINT('Ctrl Pts',(20.8910194489728,14.8324292011929,36.3889631660726));
#45537=CARTESIAN_POINT('Ctrl Pts',(20.9030405365733,14.8315428090705,36.3952587254979));
#45538=CARTESIAN_POINT('Ctrl Pts',(20.9110555537767,14.8309530752577,36.3995286507979));
#45539=CARTESIAN_POINT('Ctrl Pts',(21.0070918910693,14.8238984916717,36.4515650457887));
#45540=CARTESIAN_POINT('Ctrl Pts',(21.0913085345902,14.8178264372581,36.5060666434814));
#45541=CARTESIAN_POINT('Ctrl Pts',(21.3053016691491,14.8016812306791,36.6695030167515));
#45542=CARTESIAN_POINT('Ctrl Pts',(21.4255903173114,14.7917354971492,36.7893434100483));
#45543=CARTESIAN_POINT('Ctrl Pts',(21.5411240658571,14.779715441941,36.9394428385481));
#45544=CARTESIAN_POINT('Ctrl Pts',(21.5532749576368,14.7784153144304,36.9557565086986));
#45545=CARTESIAN_POINT('Ctrl Pts',(21.5699294722998,14.7765803530981,36.9788709142835));
#45546=CARTESIAN_POINT('Ctrl Pts',(21.574651670708,14.7760538710277,36.9855130833277));
#45547=CARTESIAN_POINT('Ctrl Pts',(21.5827704530443,14.7751377477546,36.9970874419509));
#45548=CARTESIAN_POINT('Ctrl Pts',(21.5861864458013,14.7747488474186,37.0020059310054));
#45549=CARTESIAN_POINT('Ctrl Pts',(21.5932526317669,14.7739371281863,37.0122819140797));
#45550=CARTESIAN_POINT('Ctrl Pts',(21.5968988255033,14.7735141655081,37.0176420543741));
#45551=CARTESIAN_POINT('Ctrl Pts',(21.6054473550095,14.7725126870356,37.0303461712138));
#45552=CARTESIAN_POINT('Ctrl Pts',(21.6103263894723,14.7719333114294,37.0377055784089));
#45553=CARTESIAN_POINT('Ctrl Pts',(21.6263412496798,14.7700053077335,37.0622258457392));
#45554=CARTESIAN_POINT('Ctrl Pts',(21.637254306052,14.7686485210301,37.0795298443927));
#45555=CARTESIAN_POINT('Ctrl Pts',(21.6943019797833,14.7613170612082,37.1732572748959));
#45556=CARTESIAN_POINT('Ctrl Pts',(21.7353588374863,14.7551629062869,37.2526294021031));
#45557=CARTESIAN_POINT('Ctrl Pts',(21.8225714392239,14.7396916739259,37.4543840959422));
#45558=CARTESIAN_POINT('Ctrl Pts',(21.8620720898699,14.7302530221989,37.5791619877419));
#45559=CARTESIAN_POINT('Ctrl Pts',(21.8989537850175,14.7175687758162,37.7563932903388));
#45560=CARTESIAN_POINT('Ctrl Pts',(21.9072958969132,14.7140837352363,37.8062068453744));
#45561=CARTESIAN_POINT('Ctrl Pts',(21.9146555585686,14.7101733922558,37.863997989214));
#45562=CARTESIAN_POINT('Ctrl Pts',(21.9155900440249,14.7096544847598,37.8717071064323));
#45563=CARTESIAN_POINT('Ctrl Pts',(21.9170085726011,14.7088294527818,37.8840318916333));
#45564=CARTESIAN_POINT('Ctrl Pts',(21.917522543215,14.7085217375214,37.8886439292698));
#45565=CARTESIAN_POINT('Ctrl Pts',(21.9184034497825,14.7079783260974,37.8968164097645));
#45566=CARTESIAN_POINT('Ctrl Pts',(21.9187771251771,14.7077422592171,37.9003760730656));
#45567=CARTESIAN_POINT('Ctrl Pts',(21.9195500481131,14.7072418690173,37.9079417372841));
#45568=CARTESIAN_POINT('Ctrl Pts',(21.9199466633966,14.7069776933006,37.911947948867));
#45569=CARTESIAN_POINT('Ctrl Pts',(21.920988827981,14.7062627265642,37.9228219483343));
#45570=CARTESIAN_POINT('Ctrl Pts',(21.921610094989,14.7058132655294,37.9296920859859));
#45571=CARTESIAN_POINT('Ctrl Pts',(21.9245876520355,14.7035329752186,37.9647118953069));
#45572=CARTESIAN_POINT('Ctrl Pts',(21.92636244644,14.7017324132734,37.9929092408048));
#45573=CARTESIAN_POINT('Ctrl Pts',(21.92979395014,14.6964551657695,38.0767799507119));
#45574=CARTESIAN_POINT('Ctrl Pts',(21.9296602259244,14.6930512297805,38.1324996970163));
#45575=CARTESIAN_POINT('Ctrl Pts',(21.921528783017,14.6823031074037,38.3102886959911));
#45576=CARTESIAN_POINT('Ctrl Pts',(21.9043416800587,14.6751212411879,38.4316285920931));
#45577=CARTESIAN_POINT('Ctrl Pts',(21.8579861900769,14.6630375971956,38.6246315107449));
#45578=CARTESIAN_POINT('Ctrl Pts',(21.8358139212696,14.6583115960219,38.6976086160165));
#45579=CARTESIAN_POINT('Ctrl Pts',(21.8048578236406,14.6526079183648,38.78132316183));
#45580=CARTESIAN_POINT('Ctrl Pts',(21.8002055461629,14.6517696567692,38.7935221643994));
#45581=CARTESIAN_POINT('Ctrl Pts',(21.7924430507267,14.6504004804363,38.8132721348784));
#45582=CARTESIAN_POINT('Ctrl Pts',(21.7894080293417,14.6498720679008,38.8208523632807));
#45583=CARTESIAN_POINT('Ctrl Pts',(21.7839146420267,14.6489276636536,38.8343240821607));
#45584=CARTESIAN_POINT('Ctrl Pts',(21.781474968644,14.6485123034955,38.8402231029507));
#45585=CARTESIAN_POINT('Ctrl Pts',(21.7762678284143,14.6476341829824,38.8526388808497));
#45586=CARTESIAN_POINT('Ctrl Pts',(21.773493680488,14.647171202346,38.8591527160272));
#45587=CARTESIAN_POINT('Ctrl Pts',(21.7660456247167,14.6459407841036,38.876377470418));
#45588=CARTESIAN_POINT('Ctrl Pts',(21.761310197324,14.6451712731735,38.8870613087939));
#45589=CARTESIAN_POINT('Ctrl Pts',(21.738542399015,14.6415299264438,38.9371942849403));
#45590=CARTESIAN_POINT('Ctrl Pts',(21.7192812124342,14.6386164542797,38.9760682310339));
#45591=CARTESIAN_POINT('Ctrl Pts',(21.6199659301158,14.624333139912,39.1606000503536));
#45592=CARTESIAN_POINT('Ctrl Pts',(21.5226309567835,14.6123567140228,39.2961352243444));
#45593=CARTESIAN_POINT('Ctrl Pts',(21.3888352432497,14.5984740266838,39.4392406559418));
#45594=CARTESIAN_POINT('Ctrl Pts',(21.3680018272237,14.5963753064603,39.4605146057124));
#45595=CARTESIAN_POINT('Ctrl Pts',(21.3139938495377,14.5911067623355,39.5131691628338));
#45596=CARTESIAN_POINT('Ctrl Pts',(21.2801797847202,14.5879641487012,39.5438723663814));
#45597=CARTESIAN_POINT('Ctrl Pts',(21.2395234397472,14.5843925091466,39.5782359439074));
#45598=CARTESIAN_POINT('Ctrl Pts',(21.2337130268103,14.5838868033292,39.5830886809741));
#45599=CARTESIAN_POINT('Ctrl Pts',(21.2243390897565,14.5830787216351,39.5908243881961));
#45600=CARTESIAN_POINT('Ctrl Pts',(21.2207936664035,14.5827748539383,39.5937290210376));
#45601=CARTESIAN_POINT('Ctrl Pts',(21.2144666982101,14.5822357731247,39.5988748964508));
#45602=CARTESIAN_POINT('Ctrl Pts',(21.2116892443056,14.5820002100893,39.6011210784958));
#45603=CARTESIAN_POINT('Ctrl Pts',(21.2057417339669,14.5814981148765,39.6059036854004));
#45604=CARTESIAN_POINT('Ctrl Pts',(21.202569910501,14.5812317445556,39.6084378176918));
#45605=CARTESIAN_POINT('Ctrl Pts',(21.1938667916878,14.5805045990922,39.6153462870569));
#45606=CARTESIAN_POINT('Ctrl Pts',(21.1883194056939,14.5800452318888,39.6197003914577));
#45607=CARTESIAN_POINT('Ctrl Pts',(21.1588290636444,14.577624149487,39.642586938216));
#45608=CARTESIAN_POINT('Ctrl Pts',(21.1344746340417,14.5756973414608,39.6605854073017));
#45609=CARTESIAN_POINT('Ctrl Pts',(20.9773153735092,14.563645680831,39.771105017111));
#45610=CARTESIAN_POINT('Ctrl Pts',(20.8337228065082,14.5542786840768,39.8471851382568));
#45611=CARTESIAN_POINT('Ctrl Pts',(20.5986659097545,14.5390768219629,39.9360654868534));
#45612=CARTESIAN_POINT('Ctrl Pts',(20.512944586633,14.5335671611212,39.9618329857692));
#45613=CARTESIAN_POINT('Ctrl Pts',(20.4126396995163,14.5269987481531,39.9845295945417));
#45614=CARTESIAN_POINT('Ctrl Pts',(20.3994962190366,14.5261358700942,39.9873595499071));
#45615=CARTESIAN_POINT('Ctrl Pts',(20.3782973146781,14.5247401626346,39.9916925823877));
#45616=CARTESIAN_POINT('Ctrl Pts',(20.3702598682514,14.5242100710944,39.993282153064));
#45617=CARTESIAN_POINT('Ctrl Pts',(20.3559217253216,14.5232626955192,39.9960230231005));
#45618=CARTESIAN_POINT('Ctrl Pts',(20.3496249242537,14.5228460474002,39.9971942413408));
#45619=CARTESIAN_POINT('Ctrl Pts',(20.3364394807328,14.5219722946969,39.9995788896028));
#45620=CARTESIAN_POINT('Ctrl Pts',(20.3295498493853,14.5215150053206,40.0007862522197));
#45621=CARTESIAN_POINT('Ctrl Pts',(20.3115127794415,14.5203158156879,40.0038461180996));
#45622=CARTESIAN_POINT('Ctrl Pts',(20.3003554931003,14.5195720262978,40.0056381665317));
#45623=CARTESIAN_POINT('Ctrl Pts',(20.2509700869346,14.5162705064993,40.0131258165526));
#45624=CARTESIAN_POINT('Ctrl Pts',(20.212593907927,14.5136801665685,40.0177694964867));
#45625=CARTESIAN_POINT('Ctrl Pts',(20.1080143770553,14.5065485483287,40.0272466049029));
#45626=CARTESIAN_POINT('Ctrl Pts',(20.0416638302314,14.5019437042671,40.0298210146939));
#45627=CARTESIAN_POINT('Ctrl Pts',(19.8280666551264,14.4869030104798,40.0270879694292));
#45628=CARTESIAN_POINT('Ctrl Pts',(19.6815220422533,14.4762138563043,40.0083499655989));
#45629=CARTESIAN_POINT('Ctrl Pts',(19.504999816808,14.4636230088017,39.9648620483704));
#45630=CARTESIAN_POINT('Ctrl Pts',(19.4716868822015,14.4612623700115,39.955699666514));
#45631=CARTESIAN_POINT('Ctrl Pts',(19.4319781748459,14.4584813264809,39.9436220286079));
#45632=CARTESIAN_POINT('Ctrl Pts',(19.4253316428006,14.4580169493766,39.9415610934912));
#45633=CARTESIAN_POINT('Ctrl Pts',(19.4144553897955,14.4572590554553,39.938124002261));
#45634=CARTESIAN_POINT('Ctrl Pts',(19.410219088809,14.4569643559199,39.9367691243071));
#45635=CARTESIAN_POINT('Ctrl Pts',(19.4026063985318,14.4564357252254,39.934305337392));
#45636=CARTESIAN_POINT('Ctrl Pts',(19.3992283725346,14.4562014928851,39.9332017450712));
#45637=CARTESIAN_POINT('Ctrl Pts',(19.3918567246019,14.4556910891093,39.9307708822247));
#45638=CARTESIAN_POINT('Ctrl Pts',(19.3878643995931,14.4554151388284,39.9294398798986));
#45639=CARTESIAN_POINT('Ctrl Pts',(19.3765485806149,14.4546342465418,39.9256261066141));
#45640=CARTESIAN_POINT('Ctrl Pts',(19.3692355115153,14.4541310797432,39.9231123164689));
#45641=CARTESIAN_POINT('Ctrl Pts',(19.3230943259983,14.4509647161153,39.9069408949773));
#45642=CARTESIAN_POINT('Ctrl Pts',(19.2846932902263,14.4483668321885,39.8920863769269));
#45643=CARTESIAN_POINT('Ctrl Pts',(19.1488116232062,14.4392097191443,39.8344590422087));
#45644=CARTESIAN_POINT('Ctrl Pts',(19.0544282360465,14.4329084162657,39.7848642589556));
#45645=CARTESIAN_POINT('Ctrl Pts',(18.8674306180326,14.4196605771262,39.6659165388674));
#45646=CARTESIAN_POINT('Ctrl Pts',(18.7759920320964,14.412723800333,39.5955293663914));
#45647=CARTESIAN_POINT('Ctrl Pts',(18.6719170038453,14.4037892782618,39.4994427201339));
#45648=CARTESIAN_POINT('Ctrl Pts',(18.6528254044976,14.4021029686193,39.4810738114305));
#45649=CARTESIAN_POINT('Ctrl Pts',(18.6269918736274,14.3997509550951,39.4551727174637));
#45650=CARTESIAN_POINT('Ctrl Pts',(18.619921237454,14.3990996853729,39.4479714433529));
#45651=CARTESIAN_POINT('Ctrl Pts',(18.6086969853665,14.3980535109125,39.4363589277012));
#45652=CARTESIAN_POINT('Ctrl Pts',(18.6045070161338,14.3976601815787,39.4319829551337));
#45653=CARTESIAN_POINT('Ctrl Pts',(18.5959069765196,14.3968470188198,39.4229160183698));
#45654=CARTESIAN_POINT('Ctrl Pts',(18.5914996431544,14.3964270758429,39.4182225735173));
#45655=CARTESIAN_POINT('Ctrl Pts',(18.582820414027,14.3955936485318,39.408886694315));
#45656=CARTESIAN_POINT('Ctrl Pts',(18.5785476311178,14.3951802094035,39.4042451912353));
#45657=CARTESIAN_POINT('Ctrl Pts',(18.5647397035229,14.3938338075739,39.3890972585624));
#45658=CARTESIAN_POINT('Ctrl Pts',(18.5552978637193,14.3928969651113,39.3785067774203));
#45659=CARTESIAN_POINT('Ctrl Pts',(18.4906990553966,14.3863725773239,39.3044198836624));
#45660=CARTESIAN_POINT('Ctrl Pts',(18.439636956027,14.3806199794427,39.237488567998));
#45661=CARTESIAN_POINT('Ctrl Pts',(18.3562149296603,14.3700746907748,39.1119085980691));
#45662=CARTESIAN_POINT('Ctrl Pts',(18.3222267444621,14.3653383569757,39.0544969018628));
#45663=CARTESIAN_POINT('Ctrl Pts',(18.2357481980994,14.3520505016559,38.889475389284));
#45664=CARTESIAN_POINT('Ctrl Pts',(18.1901888144504,14.3434730023865,38.778560681935));
#45665=CARTESIAN_POINT('Ctrl Pts',(18.1509233321687,14.3343709194131,38.6501559779213));
#45666=CARTESIAN_POINT('Ctrl Pts',(18.1468085956264,14.3333877552602,38.6361322354116));
#45667=CARTESIAN_POINT('Ctrl Pts',(18.1413352222397,14.3320390628001,38.616661664716));
#45668=CARTESIAN_POINT('Ctrl Pts',(18.1398405145446,14.3316662218134,38.6112540684305));
#45669=CARTESIAN_POINT('Ctrl Pts',(18.1374860604111,14.3310716438687,38.6025890274246));
#45670=CARTESIAN_POINT('Ctrl Pts',(18.1366112335004,14.33084905443,38.5993357697672));
#45671=CARTESIAN_POINT('Ctrl Pts',(18.1348052495487,14.3303860587598,38.5925489342785));
#45672=CARTESIAN_POINT('Ctrl Pts',(18.1338756065242,14.3301457457831,38.5890149876141));
#45673=CARTESIAN_POINT('Ctrl Pts',(18.1316519191684,14.3295660311852,38.5804631712082));
#45674=CARTESIAN_POINT('Ctrl Pts',(18.1303680286128,14.3292272086903,38.5754426391592));
#45675=CARTESIAN_POINT('Ctrl Pts',(18.1276754703403,14.3285076133287,38.5647340628571));
#45676=CARTESIAN_POINT('Ctrl Pts',(18.1262724533015,14.3281271521443,38.5590446344207));
#45677=CARTESIAN_POINT('Ctrl Pts',(18.1224390156797,14.3270718043661,38.5431890802928));
#45678=CARTESIAN_POINT('Ctrl Pts',(18.12006522082,14.3263998744108,38.5330092929739));
#45679=CARTESIAN_POINT('Ctrl Pts',(18.0867292803845,14.3166796244212,38.3846076511583));
#45680=CARTESIAN_POINT('Ctrl Pts',(18.0709965071608,14.3083550520962,38.2433903014528));
#45681=CARTESIAN_POINT('Ctrl Pts',(18.070870759842,14.299879738933,38.1017122113181));
#45682=CARTESIAN_POINT('Ctrl Pts',(18.0708707591309,14.2998796909909,38.1017114098911));
#45683=CARTESIAN_POINT('Ctrl Pts',(18.0707878522312,14.2942891859856,38.0082573955159));
#45684=CARTESIAN_POINT('Ctrl Pts',(18.0774957121742,14.2886562223612,37.9149266385927));
#45685=CARTESIAN_POINT('Ctrl Pts',(18.0959050454575,14.2806751915482,37.7883016683291));
#45686=CARTESIAN_POINT('Ctrl Pts',(18.1017851561007,14.2784985604903,37.7542925728336));
#45687=CARTESIAN_POINT('Ctrl Pts',(18.1106084993665,14.2756328702757,37.7103215921296));
#45688=CARTESIAN_POINT('Ctrl Pts',(18.1127245697726,14.2749695858103,37.7001988644041));
#45689=CARTESIAN_POINT('Ctrl Pts',(18.1164318309083,14.2738462128772,37.6831498987801));
#45690=CARTESIAN_POINT('Ctrl Pts',(18.1179801059569,14.2733874786639,37.6762144755653));
#45691=CARTESIAN_POINT('Ctrl Pts',(18.1211162326129,14.272478298117,37.6625225538848));
#45692=CARTESIAN_POINT('Ctrl Pts',(18.1227022986039,14.272027914496,37.6557657538437));
#45693=CARTESIAN_POINT('Ctrl Pts',(18.1258259926136,14.2711585653936,37.6427740335848));
#45694=CARTESIAN_POINT('Ctrl Pts',(18.1273583615969,14.2707397730916,37.6365379338302));
#45695=CARTESIAN_POINT('Ctrl Pts',(18.1309444898016,14.2697768913639,37.6222520826934));
#45696=CARTESIAN_POINT('Ctrl Pts',(18.1330191570007,14.2692321384901,37.6142077594996));
#45697=CARTESIAN_POINT('Ctrl Pts',(18.1386870477191,14.2677757338819,37.5928037452177));
#45698=CARTESIAN_POINT('Ctrl Pts',(18.1423720784214,14.2668611518366,37.5794690832454));
#45699=CARTESIAN_POINT('Ctrl Pts',(18.1766362955734,14.2586335718002,37.4604805375846));
#45700=CARTESIAN_POINT('Ctrl Pts',(18.2160503423616,14.2510306864612,37.3576009145721));
#45701=CARTESIAN_POINT('Ctrl Pts',(18.2955300035121,14.2381418447551,37.1936062870507));
#45702=CARTESIAN_POINT('Ctrl Pts',(18.3306854640465,14.2329690411936,37.1303835792582));
#45703=CARTESIAN_POINT('Ctrl Pts',(18.4143809391876,14.2218102555178,36.9979688626955));
#45704=CARTESIAN_POINT('Ctrl Pts',(18.4640924114812,14.21584385365,36.9296789884445));
#45705=CARTESIAN_POINT('Ctrl Pts',(18.5286630372816,14.2089912893424,36.8522094638793));
#45706=CARTESIAN_POINT('Ctrl Pts',(18.5393673610844,14.2078817389792,36.839696061038));
#45707=CARTESIAN_POINT('Ctrl Pts',(18.5531202473567,14.2064908289844,36.8240294994696));
#45708=CARTESIAN_POINT('Ctrl Pts',(18.556020703883,14.2061993959142,36.8207480583815));
#45709=CARTESIAN_POINT('Ctrl Pts',(18.5616824335083,14.2056342577341,36.8143864319971));
#45710=CARTESIAN_POINT('Ctrl Pts',(18.5644424865603,14.2053604675247,36.8113051972182));
#45711=CARTESIAN_POINT('Ctrl Pts',(18.5695964641611,14.2048524173568,36.8055885672839));
#45712=CARTESIAN_POINT('Ctrl Pts',(18.5719877504815,14.204617976235,36.802950946174));
#45713=CARTESIAN_POINT('Ctrl Pts',(18.5774465648602,14.204085677847,36.7969631957744));
#45714=CARTESIAN_POINT('Ctrl Pts',(18.580518626907,14.2037881664674,36.7936172760333));
#45715=CARTESIAN_POINT('Ctrl Pts',(18.5899510050457,14.2028808280875,36.7834166079093));
#45716=CARTESIAN_POINT('Ctrl Pts',(18.5963494829116,14.2022737972977,36.776597101819));
#45717=CARTESIAN_POINT('Ctrl Pts',(18.6601697575652,14.1962989662403,36.7095609610465));
#45718=CARTESIAN_POINT('Ctrl Pts',(18.7213889777377,14.1912000113379,36.6530641389772));
#45719=CARTESIAN_POINT('Ctrl Pts',(18.8594388694836,14.1804889145527,36.5412909930582));
#45720=CARTESIAN_POINT('Ctrl Pts',(18.937065336087,14.1749110020345,36.4873550260979));
#45721=CARTESIAN_POINT('Ctrl Pts',(19.0762875667289,14.1651671985223,36.4050572635616));
#45722=CARTESIAN_POINT('Ctrl Pts',(19.1359954373219,14.1610635279119,36.3738567528303));
#45723=CARTESIAN_POINT('Ctrl Pts',(19.2207523208231,14.1552446400369,36.3350677012214));
#45724=CARTESIAN_POINT('Ctrl Pts',(19.2445097757659,14.1536145492692,36.3247683557207));
#45725=CARTESIAN_POINT('Ctrl Pts',(19.2861234294359,14.1507560788408,36.3077146081867));
#45726=CARTESIAN_POINT('Ctrl Pts',(19.3038862197052,14.1495349620833,36.3007411950635));
#45727=CARTESIAN_POINT('Ctrl Pts',(19.3297689470991,14.1477529355454,36.2910206514505));
#45728=CARTESIAN_POINT('Ctrl Pts',(19.3378087207323,14.1471990261802,36.2880621827648));
#45729=CARTESIAN_POINT('Ctrl Pts',(19.3519522795343,14.1462238215299,36.2829643539803));
#45730=CARTESIAN_POINT('Ctrl Pts',(19.3580476587169,14.1458032937396,36.2808019413121));
#45731=CARTESIAN_POINT('Ctrl Pts',(19.3698278172143,14.1449900364659,36.2766893583239));
#45732=CARTESIAN_POINT('Ctrl Pts',(19.3755110700828,14.1445974497822,36.2747350189503));
#45733=CARTESIAN_POINT('Ctrl Pts',(19.3854984955816,14.1439070924976,36.2713526795806));
#45734=CARTESIAN_POINT('Ctrl Pts',(19.3897987554653,14.1436097021173,36.2699132365454));
#45735=CARTESIAN_POINT('Ctrl Pts',(19.3941040087558,14.1433118141013,36.2684889831906));
#45736=CARTESIAN_POINT('Ctrl Pts',(19.3941039465104,13.9716756753762,36.2684890037825));
#45737=CARTESIAN_POINT('Ctrl Pts',(19.2849119469309,13.9786750649394,36.3046116379105));
#45738=CARTESIAN_POINT('Ctrl Pts',(19.179127144956,13.9854371548148,36.3504403871307));
#45739=CARTESIAN_POINT('Ctrl Pts',(18.9998767884834,13.9977430294354,36.4479678007505));
#45740=CARTESIAN_POINT('Ctrl Pts',(18.9247759297133,14.0031957124574,36.4958344384174));
#45741=CARTESIAN_POINT('Ctrl Pts',(18.8368294460731,14.0101385072896,36.5608463898901));
#45742=CARTESIAN_POINT('Ctrl Pts',(18.8206024090689,14.0114442625977,36.5732449951234));
#45743=CARTESIAN_POINT('Ctrl Pts',(18.7976504505213,14.0133285833006,36.5913661899096));
#45744=CARTESIAN_POINT('Ctrl Pts',(18.7907628623517,14.0138989810789,36.5968812579279));
#45745=CARTESIAN_POINT('Ctrl Pts',(18.7788818245945,14.0148916525,36.6065292200839));
#45746=CARTESIAN_POINT('Ctrl Pts',(18.7738708813281,14.0153130552183,36.6106404223933));
#45747=CARTESIAN_POINT('Ctrl Pts',(18.7642692623827,14.0161258502759,36.6185993184577));
#45748=CARTESIAN_POINT('Ctrl Pts',(18.7596755950149,14.0165170896234,36.6224432991564));
#45749=CARTESIAN_POINT('Ctrl Pts',(18.7488698310427,14.0174430878813,36.6315714625633));
#45750=CARTESIAN_POINT('Ctrl Pts',(18.7426732333181,14.0179785804158,36.6368737349178));
#45751=CARTESIAN_POINT('Ctrl Pts',(18.721113582958,14.0198575942255,36.6555598873457));
#45752=CARTESIAN_POINT('Ctrl Pts',(18.7059295514659,14.0212094708056,36.6691473426178));
#45753=CARTESIAN_POINT('Ctrl Pts',(18.5669725708207,14.0338541316554,36.7975144060723));
#45754=CARTESIAN_POINT('Ctrl Pts',(18.4585744779452,14.0458620437653,36.9278140733033));
#45755=CARTESIAN_POINT('Ctrl Pts',(18.3634323532194,14.0585718979818,37.0785891304716));
#45756=CARTESIAN_POINT('Ctrl Pts',(18.3583941275299,14.0592525663647,37.0867063664525));
#45757=CARTESIAN_POINT('Ctrl Pts',(18.3060161409061,14.0664081486044,37.1725101315125));
#45758=CARTESIAN_POINT('Ctrl Pts',(18.2641616587065,14.0728230564806,37.2534256089593));
#45759=CARTESIAN_POINT('Ctrl Pts',(18.2246119917548,14.079539603185,37.3452676240532));
#45760=CARTESIAN_POINT('Ctrl Pts',(18.2211105494007,14.0801409671818,37.3535578593079));
#45761=CARTESIAN_POINT('Ctrl Pts',(18.215956038518,14.0810361589589,37.3660042914641));
#45762=CARTESIAN_POINT('Ctrl Pts',(18.2142592629757,14.0813325041069,37.3701420838388));
#45763=CARTESIAN_POINT('Ctrl Pts',(18.2112394801778,14.0818628783071,37.3775797632312));
#45764=CARTESIAN_POINT('Ctrl Pts',(18.2099111980462,14.0820972177378,37.3808774252267));
#45765=CARTESIAN_POINT('Ctrl Pts',(18.2070377429455,14.0826064579249,37.3880685095928));
#45766=CARTESIAN_POINT('Ctrl Pts',(18.2054961356777,14.0828811451278,37.391963289079));
#45767=CARTESIAN_POINT('Ctrl Pts',(18.2012537814394,14.0836412809253,37.4027842066803));
#45768=CARTESIAN_POINT('Ctrl Pts',(18.1985803299087,14.0841251377074,37.4097210724496));
#45769=CARTESIAN_POINT('Ctrl Pts',(18.184671742712,14.0866691850657,37.4464411810257));
#45770=CARTESIAN_POINT('Ctrl Pts',(18.1741342000889,14.0886910511325,37.4764856250123));
#45771=CARTESIAN_POINT('Ctrl Pts',(18.1025222395381,14.1032654569102,37.6980808331471));
#45772=CARTESIAN_POINT('Ctrl Pts',(18.0709770307598,14.1147043860589,37.8978838092169));
#45773=CARTESIAN_POINT('Ctrl Pts',(18.0708429566733,14.1303155216926,38.1504268368755));
#45774=CARTESIAN_POINT('Ctrl Pts',(18.072873971112,14.1335455015647,38.2018543337162));
#45775=CARTESIAN_POINT('Ctrl Pts',(18.077970987111,14.1376569892982,38.2658613695612));
#45776=CARTESIAN_POINT('Ctrl Pts',(18.0791106073354,14.1384781995256,38.278576170833));
#45777=CARTESIAN_POINT('Ctrl Pts',(18.0811093846322,14.1397812248853,38.2986354069124));
#45778=CARTESIAN_POINT('Ctrl Pts',(18.0818847343445,14.1402604246902,38.3059879699693));
#45779=CARTESIAN_POINT('Ctrl Pts',(18.083403997203,14.1411533406297,38.3196419324309));
#45780=CARTESIAN_POINT('Ctrl Pts',(18.0841367736193,14.1415667032452,38.3259444901209));
#45781=CARTESIAN_POINT('Ctrl Pts',(18.0858282114475,14.1424841983547,38.3398922429677));
#45782=CARTESIAN_POINT('Ctrl Pts',(18.0868016064441,14.1429887855927,38.3475355092181));
#45783=CARTESIAN_POINT('Ctrl Pts',(18.0897481392812,14.144451804665,38.3696158497815));
#45784=CARTESIAN_POINT('Ctrl Pts',(18.0918390585632,14.1454139053866,38.3840364055957));
#45785=CARTESIAN_POINT('Ctrl Pts',(18.1096941016752,14.1530757191918,38.4980660666897));
#45786=CARTESIAN_POINT('Ctrl Pts',(18.1330810844507,14.160016752213,38.5963071742129));
#45787=CARTESIAN_POINT('Ctrl Pts',(18.1918465668368,14.1735033709713,38.7784770602139));
#45788=CARTESIAN_POINT('Ctrl Pts',(18.2256981268137,14.179998813167,38.8626281187381));
#45789=CARTESIAN_POINT('Ctrl Pts',(18.3032684230973,14.1926079821378,39.0220416301474));
#45790=CARTESIAN_POINT('Ctrl Pts',(18.3464191710355,14.1987106665962,39.0973630188985));
#45791=CARTESIAN_POINT('Ctrl Pts',(18.3996924673201,14.2051691639591,39.1773329050062));
#45792=CARTESIAN_POINT('Ctrl Pts',(18.4049451997717,14.2057957453093,39.1850947333449));
#45793=CARTESIAN_POINT('Ctrl Pts',(18.4128298534666,14.2067208950661,39.1965647050211));
#45794=CARTESIAN_POINT('Ctrl Pts',(18.4154185587463,14.2070222302401,39.2003021782356));
#45795=CARTESIAN_POINT('Ctrl Pts',(18.4200581850617,14.2075579712121,39.2069503584316));
#45796=CARTESIAN_POINT('Ctrl Pts',(18.4221039696758,14.2077927151483,39.2098645650853));
#45797=CARTESIAN_POINT('Ctrl Pts',(18.426542281998,14.2082987874333,39.2161498348777));
#45798=CARTESIAN_POINT('Ctrl Pts',(18.4289375744055,14.2085699239158,39.2195188698347));
#45799=CARTESIAN_POINT('Ctrl Pts',(18.4356443203041,14.2093236737108,39.2288881498322));
#45800=CARTESIAN_POINT('Ctrl Pts',(18.4399795001487,14.2098047020793,39.2348714428392));
#45801=CARTESIAN_POINT('Ctrl Pts',(18.465240640136,14.2125731041899,39.269317875493));
#45802=CARTESIAN_POINT('Ctrl Pts',(18.4869124628092,14.2148126085949,39.297228914235));
#45803=CARTESIAN_POINT('Ctrl Pts',(18.5602094546646,14.2220174581278,39.3864556243148));
#45804=CARTESIAN_POINT('Ctrl Pts',(18.6148923358614,14.2268327196856,39.4451556761213));
#45805=CARTESIAN_POINT('Ctrl Pts',(18.7853430230445,14.2408758103055,39.6066765519526));
#45806=CARTESIAN_POINT('Ctrl Pts',(18.9099853077166,14.2500390747562,39.6991646343082));
#45807=CARTESIAN_POINT('Ctrl Pts',(19.0631082948539,14.2612103368516,39.7864886559279));
#45808=CARTESIAN_POINT('Ctrl Pts',(19.0820685138739,14.2625910643644,39.7968829602451));
#45809=CARTESIAN_POINT('Ctrl Pts',(19.1085988977558,14.2645214364564,39.8108525872945));
#45810=CARTESIAN_POINT('Ctrl Pts',(19.1160241157818,14.2650615233667,39.8147008873421));
#45811=CARTESIAN_POINT('Ctrl Pts',(19.1288575211868,14.2659947904957,39.8212466006609));
#45812=CARTESIAN_POINT('Ctrl Pts',(19.1342538362738,14.2663871608946,39.8239671276723));
#45813=CARTESIAN_POINT('Ctrl Pts',(19.1454330171029,14.2671999323132,39.829537334185));
#45814=CARTESIAN_POINT('Ctrl Pts',(19.1512175557214,14.267620449934,39.8323834677098));
#45815=CARTESIAN_POINT('Ctrl Pts',(19.1647647741944,14.2686052495256,39.8389648890694));
#45816=CARTESIAN_POINT('Ctrl Pts',(19.172538374529,14.2691703121474,39.8426772570269));
#45817=CARTESIAN_POINT('Ctrl Pts',(19.1977521749771,14.2710031683828,39.8545116441086));
#45818=CARTESIAN_POINT('Ctrl Pts',(19.2152886236255,14.2722780537122,39.8624246629341));
#45819=CARTESIAN_POINT('Ctrl Pts',(19.3058049725359,14.2788612522324,39.9016498477938));
#45820=CARTESIAN_POINT('Ctrl Pts',(19.3805405727024,14.2843104070488,39.9286924317987));
#45821=CARTESIAN_POINT('Ctrl Pts',(19.5604893664041,14.2974449078329,39.9815069222736));
#45822=CARTESIAN_POINT('Ctrl Pts',(19.6666304157314,14.3052094770627,40.0031815398957));
#45823=CARTESIAN_POINT('Ctrl Pts',(19.8567509171756,14.3188138762382,40.0256069441313));
#45824=CARTESIAN_POINT('Ctrl Pts',(19.9400391728748,14.3246680119929,40.0299975469649));
#45825=CARTESIAN_POINT('Ctrl Pts',(20.0327102416572,14.3308969669913,40.0288753325193));
#45826=CARTESIAN_POINT('Ctrl Pts',(20.0420603879069,14.3315221784472,40.0286941024248));
#45827=CARTESIAN_POINT('Ctrl Pts',(20.0559498356314,14.3324457038719,40.0283238332691));
#45828=CARTESIAN_POINT('Ctrl Pts',(20.0604902125199,14.3327467707857,40.028186745442));
#45829=CARTESIAN_POINT('Ctrl Pts',(20.0685883392662,14.3332822204649,40.0279136059334));
#45830=CARTESIAN_POINT('Ctrl Pts',(20.0721462277512,14.3335169398803,40.0277837417011));
#45831=CARTESIAN_POINT('Ctrl Pts',(20.0798371326405,14.3340231698315,40.027481698928));
#45832=CARTESIAN_POINT('Ctrl Pts',(20.0839699517125,14.3342944873828,40.027306077263));
#45833=CARTESIAN_POINT('Ctrl Pts',(20.0954959053672,14.3350492527391,40.0267791440044));
#45834=CARTESIAN_POINT('Ctrl Pts',(20.1028877282419,14.335531108659,40.0263985717944));
#45835=CARTESIAN_POINT('Ctrl Pts',(20.1457587995633,14.3383140142852,40.0239438639971));
#45836=CARTESIAN_POINT('Ctrl Pts',(20.1811801236259,14.3405666060866,40.0209320056448));
#45837=CARTESIAN_POINT('Ctrl Pts',(20.2969657317302,14.3478353769175,40.0078551131425));
#45838=CARTESIAN_POINT('Ctrl Pts',(20.3767858369393,14.3526984103629,39.9937091658136));
#45839=CARTESIAN_POINT('Ctrl Pts',(20.6046334064205,14.3667185025429,39.9383468707799));
#45840=CARTESIAN_POINT('Ctrl Pts',(20.7489038395766,14.3758169935013,39.8844432042381));
#45841=CARTESIAN_POINT('Ctrl Pts',(20.9045364980838,14.3869171605174,39.8040619396936));
#45842=CARTESIAN_POINT('Ctrl Pts',(20.9236452280323,14.3883027039898,39.7937806242355));
#45843=CARTESIAN_POINT('Ctrl Pts',(20.9498835484393,14.3902387471173,39.7790872371453));
#45844=CARTESIAN_POINT('Ctrl Pts',(20.9571643883838,14.3907796143533,39.7749474724691));
#45845=CARTESIAN_POINT('Ctrl Pts',(20.9696546580332,14.3917138681886,39.7677376776728));
#45846=CARTESIAN_POINT('Ctrl Pts',(20.9748770783563,14.3921064409661,39.7646903009539));
#45847=CARTESIAN_POINT('Ctrl Pts',(20.9856363184326,14.3929192914005,39.7583440966246));
#45848=CARTESIAN_POINT('Ctrl Pts',(20.9911710989411,14.3933396841547,39.7550419770992));
#45849=CARTESIAN_POINT('Ctrl Pts',(21.0040551082252,14.3943236000621,39.7472674069181));
#45850=CARTESIAN_POINT('Ctrl Pts',(21.0113911258097,14.3948878996797,39.7427734344215));
#45851=CARTESIAN_POINT('Ctrl Pts',(21.0349803188844,14.3967157750897,39.7281050269173));
#45852=CARTESIAN_POINT('Ctrl Pts',(21.0511115059862,14.3979863888938,39.717737554811));
#45853=CARTESIAN_POINT('Ctrl Pts',(21.1328290246359,14.4045317839027,39.6634796864818));
#45854=CARTESIAN_POINT('Ctrl Pts',(21.1958240152582,14.4099455905328,39.6158404885852));
#45855=CARTESIAN_POINT('Ctrl Pts',(21.3366507447113,14.422934280803,39.4950888733766));
#45856=CARTESIAN_POINT('Ctrl Pts',(21.411687329708,14.4305847476165,39.419107442892));
#45857=CARTESIAN_POINT('Ctrl Pts',(21.5348377060535,14.4442367306801,39.2717978999963));
#45858=CARTESIAN_POINT('Ctrl Pts',(21.5852127261009,14.4502449039189,39.2026972998371));
#45859=CARTESIAN_POINT('Ctrl Pts',(21.63584897827,14.4566163001405,39.1225597246511));
#45860=CARTESIAN_POINT('Ctrl Pts',(21.640794139209,14.4572424583278,39.1146057715237));
#45861=CARTESIAN_POINT('Ctrl Pts',(21.6480529394401,14.4581671063632,39.1027386119726));
#45862=CARTESIAN_POINT('Ctrl Pts',(21.6504109004741,14.4584683587056,39.0988528799499));
#45863=CARTESIAN_POINT('Ctrl Pts',(21.6545914694076,14.4590040097025,39.0919084147454));
#45864=CARTESIAN_POINT('Ctrl Pts',(21.6564193589304,14.4592387460354,39.0888529425354));
#45865=CARTESIAN_POINT('Ctrl Pts',(21.6603515949405,14.459744866858,39.082238378688));
#45866=CARTESIAN_POINT('Ctrl Pts',(21.6624529575637,14.4600160591368,39.0786775853519));
#45867=CARTESIAN_POINT('Ctrl Pts',(21.6682795415641,14.4607701218344,39.0687314267732));
#45868=CARTESIAN_POINT('Ctrl Pts',(21.6719795808526,14.461251405172,39.0623312795175));
#45869=CARTESIAN_POINT('Ctrl Pts',(21.6931803477115,14.4640242651393,39.0251678264176));
#45870=CARTESIAN_POINT('Ctrl Pts',(21.7098699129593,14.4662677919328,38.9939465651123));
#45871=CARTESIAN_POINT('Ctrl Pts',(21.7616274728153,14.4734922405503,38.8903636615829));
#45872=CARTESIAN_POINT('Ctrl Pts',(21.7930350695368,14.4783221433256,38.8162635483253));
#45873=CARTESIAN_POINT('Ctrl Pts',(21.87095410656,14.492358105124,38.5948576064915));
#45874=CARTESIAN_POINT('Ctrl Pts',(21.9045255013967,14.5015014702645,38.4436999878402));
#45875=CARTESIAN_POINT('Ctrl Pts',(21.9218681088986,14.5126509071936,38.2686240364368));
#45876=CARTESIAN_POINT('Ctrl Pts',(21.9236390787485,14.5140331464573,38.2470500881662));
#45877=CARTESIAN_POINT('Ctrl Pts',(21.9255907247164,14.5159652992896,38.2171022028006));
#45878=CARTESIAN_POINT('Ctrl Pts',(21.9260805047094,14.516505631759,38.2087494863649));
#45879=CARTESIAN_POINT('Ctrl Pts',(21.9268304787907,14.5174392093566,38.194357812878));
#45880=CARTESIAN_POINT('Ctrl Pts',(21.927116658865,14.5178316434063,38.1883202841593));
#45881=CARTESIAN_POINT('Ctrl Pts',(21.9276494046836,14.5186444394878,38.175841174625));
#45882=CARTESIAN_POINT('Ctrl Pts',(21.9278920657791,14.5190649176471,38.1693995112679));
#45883=CARTESIAN_POINT('Ctrl Pts',(21.9283834510545,14.5200494383605,38.1543504477407));
#45884=CARTESIAN_POINT('Ctrl Pts',(21.9286068373525,14.5206142602441,38.145742412877));
#45885=CARTESIAN_POINT('Ctrl Pts',(21.9291425154037,14.5224455439847,38.1179182901047));
#45886=CARTESIAN_POINT('Ctrl Pts',(21.9292252779906,14.5237190805797,38.0986994518787));
#45887=CARTESIAN_POINT('Ctrl Pts',(21.9281779893899,14.5302903299362,38.0002319835502));
#45888=CARTESIAN_POINT('Ctrl Pts',(21.9224522138208,14.5357283088537,37.9211184758602));
#45889=CARTESIAN_POINT('Ctrl Pts',(21.8975070706028,14.5488203043225,37.7358418939755));
#45890=CARTESIAN_POINT('Ctrl Pts',(21.8742202824952,14.5565525783041,37.6304897175076));
#45891=CARTESIAN_POINT('Ctrl Pts',(21.8173686545484,14.5701718826056,37.4475001091928));
#45892=CARTESIAN_POINT('Ctrl Pts',(21.7872644691981,14.5760709150314,37.3690594171895));
#45893=CARTESIAN_POINT('Ctrl Pts',(21.7482280493922,14.5823414435496,37.2843231155787));
#45894=CARTESIAN_POINT('Ctrl Pts',(21.744251464342,14.5829669593776,37.2758538174195));
#45895=CARTESIAN_POINT('Ctrl Pts',(21.738252512324,14.5838908457376,37.2633152316894));
#45896=CARTESIAN_POINT('Ctrl Pts',(21.7362772053697,14.5841919722831,37.2592237721688));
#45897=CARTESIAN_POINT('Ctrl Pts',(21.7327282001407,14.5847274866882,37.2519385534095));
#45898=CARTESIAN_POINT('Ctrl Pts',(21.7311601013199,14.5849622115285,37.2487421441923));
#45899=CARTESIAN_POINT('Ctrl Pts',(21.7277512648392,14.585468406314,37.2418419556257));
#45900=CARTESIAN_POINT('Ctrl Pts',(21.7259074671023,14.5857396835238,37.2381397572271));
#45901=CARTESIAN_POINT('Ctrl Pts',(21.7207322006901,14.5864942225824,37.2278314447371));
#45902=CARTESIAN_POINT('Ctrl Pts',(21.7173745699723,14.586975894094,37.2212384362011));
#45903=CARTESIAN_POINT('Ctrl Pts',(21.6976906043734,14.5897555591137,37.1831309449869));
#45904=CARTESIAN_POINT('Ctrl Pts',(21.6805337756067,14.5920052265549,37.1520501765005));
#45905=CARTESIAN_POINT('Ctrl Pts',(21.6215479739906,14.5992596758385,37.0518341829809));
#45906=CARTESIAN_POINT('Ctrl Pts',(21.5762314243651,14.6041120008986,36.9848470547321));
#45907=CARTESIAN_POINT('Ctrl Pts',(21.4328718209787,14.6181369482902,36.799208226113));
#45908=CARTESIAN_POINT('Ctrl Pts',(21.3247028410053,14.6272496872541,36.689206954274));
#45909=CARTESIAN_POINT('Ctrl Pts',(21.1876939987385,14.6383656561559,36.5796724922583));
#45910=CARTESIAN_POINT('Ctrl Pts',(21.1705305053323,14.6397503221424,36.5664188833777));
#45911=CARTESIAN_POINT('Ctrl Pts',(21.1464351286698,14.6416853323904,36.5484526549187));
#45912=CARTESIAN_POINT('Ctrl Pts',(21.1396900432251,14.6422260578762,36.543491320283));
#45913=CARTESIAN_POINT('Ctrl Pts',(21.1280194086006,14.6431601324464,36.535023538784));
#45914=CARTESIAN_POINT('Ctrl Pts',(21.12310924136,14.6435526684364,36.5314960181971));
#45915=CARTESIAN_POINT('Ctrl Pts',(21.1129304456644,14.644365504378,36.5242557560328));
#45916=CARTESIAN_POINT('Ctrl Pts',(21.1076596365849,14.6447859196996,36.5205462250903));
#45917=CARTESIAN_POINT('Ctrl Pts',(21.0953085661789,14.6457699955869,36.5119459231924));
#45918=CARTESIAN_POINT('Ctrl Pts',(21.0882140184412,14.6463344333748,36.5070760055687));
#45919=CARTESIAN_POINT('Ctrl Pts',(21.0651965169169,14.6481632100783,36.4915016130267));
#45920=CARTESIAN_POINT('Ctrl Pts',(21.0491467967063,14.6494345967078,36.4809874507779));
#45921=CARTESIAN_POINT('Ctrl Pts',(20.9662173885793,14.6559868226076,36.4284113999003));
#45922=CARTESIAN_POINT('Ctrl Pts',(20.8969644355208,14.6614070145264,36.3902525287703));
#45923=CARTESIAN_POINT('Ctrl Pts',(20.7505318002892,14.6727516258303,36.3209163305776));
#45924=CARTESIAN_POINT('Ctrl Pts',(20.6732765741397,14.6786763520575,36.2902669214684));
#45925=CARTESIAN_POINT('Ctrl Pts',(20.4904244559541,14.6923888466525,36.2310574632859));
#45926=CARTESIAN_POINT('Ctrl Pts',(20.3838754813475,14.7001553189174,36.2062978663796));
#45927=CARTESIAN_POINT('Ctrl Pts',(20.2667117797668,14.7081092172196,36.1893740372918));
#45928=CARTESIAN_POINT('Ctrl Pts',(20.2576212725021,14.7087225039489,36.1881270881732));
#45929=CARTESIAN_POINT('Ctrl Pts',(20.2440521357221,14.7096318748217,36.1863643427277));
#45930=CARTESIAN_POINT('Ctrl Pts',(20.2395801971605,14.7099305929198,36.1857993302979));
#45931=CARTESIAN_POINT('Ctrl Pts',(20.2315752822523,14.7104635052454,36.1848164314224));
#45932=CARTESIAN_POINT('Ctrl Pts',(20.2280431049758,14.7106980230727,36.1843926405278));
#45933=CARTESIAN_POINT('Ctrl Pts',(20.2203761786501,14.7112056932662,36.1834942689287));
#45934=CARTESIAN_POINT('Ctrl Pts',(20.2162410696391,14.7114786426324,36.1830232974927));
#45935=CARTESIAN_POINT('Ctrl Pts',(20.2046323551703,14.7122425787989,36.1817391545809));
#45936=CARTESIAN_POINT('Ctrl Pts',(20.1971553724795,14.7127319104081,36.1809562705672));
#45937=CARTESIAN_POINT('Ctrl Pts',(20.1523264217291,14.7156505593776,36.1765271864679));
#45938=CARTESIAN_POINT('Ctrl Pts',(20.1148762269242,14.718025725202,36.1739275956097));
#45939=CARTESIAN_POINT('Ctrl Pts',(19.9137778933238,14.730555823681,36.1658556994479));
#45940=CARTESIAN_POINT('Ctrl Pts',(19.7500020003764,14.7400188738409,36.1801406301291));
#45941=CARTESIAN_POINT('Ctrl Pts',(19.5237833685961,14.7540856011064,36.2293449190564));
#45942=CARTESIAN_POINT('Ctrl Pts',(19.4583997580746,14.7582666790052,36.2472188202353));
#45943=CARTESIAN_POINT('Ctrl Pts',(19.3941039945165,14.7625557686229,36.2684889879012));
#45944=CARTESIAN_POINT('Origin',(20.,-1.3495818343519,38.1));
#45945=CARTESIAN_POINT('',(19.3941040321498,15.7277949589794,36.2684889754515));
#45946=CARTESIAN_POINT('',(19.394103641706,15.5577020380306,36.2684891046172));
#45947=CARTESIAN_POINT('',(19.3941040087494,-1.3495818343519,36.2684889831927));
#45948=CARTESIAN_POINT('Ctrl Pts',(19.3941040321498,15.7277949589794,36.2684889754514));
#45949=CARTESIAN_POINT('Ctrl Pts',(19.4085375566523,15.7267271732423,36.2637141124117));
#45950=CARTESIAN_POINT('Ctrl Pts',(19.4230334395446,15.7256632891615,36.2591079108319));
#45951=CARTESIAN_POINT('Ctrl Pts',(19.4769071148735,15.7217442201161,36.2426885248953));
#45952=CARTESIAN_POINT('Ctrl Pts',(19.5166018821413,15.7189248518383,36.2319638844828));
#45953=CARTESIAN_POINT('Ctrl Pts',(19.5641139309572,15.7156538202491,36.220743416885));
#45954=CARTESIAN_POINT('Ctrl Pts',(19.5716262984956,15.7151396686082,36.2190167605359));
#45955=CARTESIAN_POINT('Ctrl Pts',(19.5832506867176,15.7143490010339,36.2164182439874));
#45956=CARTESIAN_POINT('Ctrl Pts',(19.5873554402317,15.7140707480158,36.2155147414123));
#45957=CARTESIAN_POINT('Ctrl Pts',(19.5949366572934,15.7135586149015,36.2138719881819));
#45958=CARTESIAN_POINT('Ctrl Pts',(19.5984121868959,15.7133245273396,36.2131289346317));
#45959=CARTESIAN_POINT('Ctrl Pts',(19.6062481792904,15.7127983000245,36.2114762642137));
#45960=CARTESIAN_POINT('Ctrl Pts',(19.610609740669,15.7125064738596,36.2105721437792));
#45961=CARTESIAN_POINT('Ctrl Pts',(19.6234301560033,15.7116517284729,36.2079608421738));
#45962=CARTESIAN_POINT('Ctrl Pts',(19.6318975161582,15.711091099965,36.2062952737316));
#45963=CARTESIAN_POINT('Ctrl Pts',(19.6928596581227,15.7070808757036,36.1947280832066));
#45964=CARTESIAN_POINT('Ctrl Pts',(19.7457398939406,15.7037410856224,36.1869528922951));
#45965=CARTESIAN_POINT('Ctrl Pts',(19.820884861692,15.6991044086728,36.1790757779161));
#45966=CARTESIAN_POINT('Ctrl Pts',(19.8429285271434,15.6977574653253,36.1771477692367));
#45967=CARTESIAN_POINT('Ctrl Pts',(20.0322938340505,15.6862645985766,36.1638635680227));
#45968=CARTESIAN_POINT('Ctrl Pts',(20.2003943389596,15.6765125810087,36.1739911840351));
#45969=CARTESIAN_POINT('Ctrl Pts',(20.4058318820859,15.6634760378526,36.2135837454306));
#45970=CARTESIAN_POINT('Ctrl Pts',(20.446326998144,15.660854688351,36.2227526493166));
#45971=CARTESIAN_POINT('Ctrl Pts',(20.4976360195265,15.6574529713628,36.2361240501768));
#45972=CARTESIAN_POINT('Ctrl Pts',(20.508752934047,15.6567110789579,36.2391277295259));
#45973=CARTESIAN_POINT('Ctrl Pts',(20.526623831838,15.6555103292636,36.2441283746714));
#45974=CARTESIAN_POINT('Ctrl Pts',(20.5333950480607,15.655053479349,36.2460631427992));
#45975=CARTESIAN_POINT('Ctrl Pts',(20.5462920352944,15.6541796481183,36.2498247568621));
#45976=CARTESIAN_POINT('Ctrl Pts',(20.5524196285936,15.6537628834141,36.2516450637265));
#45977=CARTESIAN_POINT('Ctrl Pts',(20.5664213173985,15.6528068645446,36.2558803506851));
#45978=CARTESIAN_POINT('Ctrl Pts',(20.5742891776747,15.6522669663381,36.2583153563502));
#45979=CARTESIAN_POINT('Ctrl Pts',(20.5948127006934,15.6508514653293,36.2648114364196));
#45980=CARTESIAN_POINT('Ctrl Pts',(20.6074422338898,15.6499732570847,36.2689529961436));
#45981=CARTESIAN_POINT('Ctrl Pts',(20.6991024338432,15.6435461946761,36.3000634787849));
#45982=CARTESIAN_POINT('Ctrl Pts',(20.776339935786,15.6378342394285,36.3320043698093));
#45983=CARTESIAN_POINT('Ctrl Pts',(20.995129069237,15.6207818377479,36.4395889702883));
#45984=CARTESIAN_POINT('Ctrl Pts',(21.1296075189399,15.6091150971267,36.5279858919304));
#45985=CARTESIAN_POINT('Ctrl Pts',(21.2799112377696,15.5954125008689,36.6561322185206));
#45986=CARTESIAN_POINT('Ctrl Pts',(21.3075229557033,15.5928667775108,36.6810880525385));
#45987=CARTESIAN_POINT('Ctrl Pts',(21.3398134502562,15.589872144931,36.7120163127197));
#45988=CARTESIAN_POINT('Ctrl Pts',(21.3451991387624,15.5893720694162,36.7172353492887));
#45989=CARTESIAN_POINT('Ctrl Pts',(21.353523299206,15.5885983987347,36.7253965943152));
#45990=CARTESIAN_POINT('Ctrl Pts',(21.3564828520732,15.5883231804795,36.7283170492948));
#45991=CARTESIAN_POINT('Ctrl Pts',(21.361957397213,15.5878138474623,36.733754317844));
#45992=CARTESIAN_POINT('Ctrl Pts',(21.3644748470554,15.5875795430648,36.736268498594));
#45993=CARTESIAN_POINT('Ctrl Pts',(21.3701696631782,15.5870492943094,36.7419874756169));
#45994=CARTESIAN_POINT('Ctrl Pts',(21.3733427429397,15.5867536850555,36.7451964593665));
#45995=CARTESIAN_POINT('Ctrl Pts',(21.3829518518804,15.5858578800712,36.7549827457934));
#45996=CARTESIAN_POINT('Ctrl Pts',(21.3893522212693,15.5852603779916,36.7615951090444));
#45997=CARTESIAN_POINT('Ctrl Pts',(21.4433928454948,15.5802056598205,36.8182310836686));
#45998=CARTESIAN_POINT('Ctrl Pts',(21.4883676390894,15.5759329086197,36.8707406531145));
#45999=CARTESIAN_POINT('Ctrl Pts',(21.5913455854817,15.5656608209672,37.0049325294973));
#46000=CARTESIAN_POINT('Ctrl Pts',(21.6459924361639,15.5597560391722,37.0889294141743));
#46001=CARTESIAN_POINT('Ctrl Pts',(21.7460259395296,15.5471979069135,37.2724676154762));
#46002=CARTESIAN_POINT('Ctrl Pts',(21.7899663028703,15.5405429194917,37.3723791449959));
#46003=CARTESIAN_POINT('Ctrl Pts',(21.8300135742332,15.5326404848229,37.4894178065164));
#46004=CARTESIAN_POINT('Ctrl Pts',(21.8346302860397,15.5316927883579,37.5034331630212));
#46005=CARTESIAN_POINT('Ctrl Pts',(21.8414238557428,15.5302397598384,37.5248820080998));
#46006=CARTESIAN_POINT('Ctrl Pts',(21.8437175513971,15.5297382337177,37.5322781412575));
#46007=CARTESIAN_POINT('Ctrl Pts',(21.8478100531924,15.5288230041019,37.5457610204101));
#46008=CARTESIAN_POINT('Ctrl Pts',(21.849623477474,15.5284097815853,37.551843244001));
#46009=CARTESIAN_POINT('Ctrl Pts',(21.8534753441479,15.5275151571575,37.5649991614076));
#46010=CARTESIAN_POINT('Ctrl Pts',(21.8555033709289,15.527033425708,37.5720757756974));
#46011=CARTESIAN_POINT('Ctrl Pts',(21.8608998997988,15.5257218073417,37.5913217531051));
#46012=CARTESIAN_POINT('Ctrl Pts',(21.8641894575628,15.5248893960787,37.6035126895597));
#46013=CARTESIAN_POINT('Ctrl Pts',(21.8798138466165,15.5207670131837,37.6637613799391));
#46014=CARTESIAN_POINT('Ctrl Pts',(21.8904101869077,15.5174221638474,37.7122464722687));
#46015=CARTESIAN_POINT('Ctrl Pts',(21.9038960606682,15.5121626743248,37.7878146213803));
#46016=CARTESIAN_POINT('Ctrl Pts',(21.9081015256913,15.5102866751858,37.8146434179864));
#46017=CARTESIAN_POINT('Ctrl Pts',(21.9285826523755,15.4996480655928,37.9661417142186));
#46018=CARTESIAN_POINT('Ctrl Pts',(21.9332049105341,15.4906061002666,38.092073840477));
#46019=CARTESIAN_POINT('Ctrl Pts',(21.921130115353,15.4765410159168,38.2898764992507));
#46020=CARTESIAN_POINT('Ctrl Pts',(21.9126419041394,15.4714549368797,38.3619106998993));
#46021=CARTESIAN_POINT('Ctrl Pts',(21.8977454429915,15.4656198606342,38.4468335251208));
#46022=CARTESIAN_POINT('Ctrl Pts',(21.8952275216262,15.4646968966408,38.4603386299913));
#46023=CARTESIAN_POINT('Ctrl Pts',(21.8915372997211,15.4634280397048,38.4790215748941));
#46024=CARTESIAN_POINT('Ctrl Pts',(21.8904876468279,15.4630756560278,38.4842228120673));
#46025=CARTESIAN_POINT('Ctrl Pts',(21.8886740509162,15.4624810332889,38.4930221559424));
#46026=CARTESIAN_POINT('Ctrl Pts',(21.8879212579673,15.4622381723908,38.4966225033613));
#46027=CARTESIAN_POINT('Ctrl Pts',(21.8864647909285,15.4617757740526,38.5034901727427));
#46028=CARTESIAN_POINT('Ctrl Pts',(21.8857629194071,15.4615561330702,38.5067578384331));
#46029=CARTESIAN_POINT('Ctrl Pts',(21.8838898304956,15.4609782428977,38.5153692213372));
#46030=CARTESIAN_POINT('Ctrl Pts',(21.8827043582617,15.4606207972262,38.5207098580398));
#46031=CARTESIAN_POINT('Ctrl Pts',(21.8784577368085,15.459368729564,38.5394637299755));
#46032=CARTESIAN_POINT('Ctrl Pts',(21.8752757469053,15.4584806637124,38.5528495755311));
#46033=CARTESIAN_POINT('Ctrl Pts',(21.8383263780269,15.4486885458102,38.7012135719824));
#46034=CARTESIAN_POINT('Ctrl Pts',(21.7901888193471,15.4404921868739,38.8322142356736));
#46035=CARTESIAN_POINT('Ctrl Pts',(21.6699312892944,15.4243070583666,39.0747706104339));
#46036=CARTESIAN_POINT('Ctrl Pts',(21.5996043498948,15.4163659961291,39.1863273948278));
#46037=CARTESIAN_POINT('Ctrl Pts',(21.5091734073059,15.4070033805869,39.3017345654883));
#46038=CARTESIAN_POINT('Ctrl Pts',(21.4997257631104,15.4060343583162,39.3135044103313));
#46039=CARTESIAN_POINT('Ctrl Pts',(21.4851790074799,15.4045553396243,39.331197353137));
#46040=CARTESIAN_POINT('Ctrl Pts',(21.4801802516527,15.4040493645198,39.3372025001138));
#46041=CARTESIAN_POINT('Ctrl Pts',(21.4710525854525,15.4031294463274,39.3480333252024));
#46042=CARTESIAN_POINT('Ctrl Pts',(21.4669360437069,15.4027160091941,39.3528693196211));
#46043=CARTESIAN_POINT('Ctrl Pts',(21.4580320360931,15.4018247835741,39.3632254468956));
#46044=CARTESIAN_POINT('Ctrl Pts',(21.4532369494356,15.4013466860645,39.3687388676496));
#46045=CARTESIAN_POINT('Ctrl Pts',(21.4402270020213,15.4000543996305,39.3835272679631));
#46046=CARTESIAN_POINT('Ctrl Pts',(21.4319540321716,15.3992378094522,39.3927504409573));
#46047=CARTESIAN_POINT('Ctrl Pts',(21.391864800589,15.3953046473618,39.4365871794421));
#46048=CARTESIAN_POINT('Ctrl Pts',(21.3588815409081,15.3921390434092,39.4701070110743));
#46049=CARTESIAN_POINT('Ctrl Pts',(21.3016145165002,15.3867517567224,39.5242020555569));
#46050=CARTESIAN_POINT('Ctrl Pts',(21.2779854429527,15.3845577169161,39.545442796018));
#46051=CARTESIAN_POINT('Ctrl Pts',(21.1260539856926,15.3706342996767,39.6753791296951));
#46052=CARTESIAN_POINT('Ctrl Pts',(20.9845409896285,15.3583824167357,39.7674795249549));
#46053=CARTESIAN_POINT('Ctrl Pts',(20.7986849251493,15.3440795812625,39.8564404798812));
#46054=CARTESIAN_POINT('Ctrl Pts',(20.7639995693595,15.3414836328523,39.8718030078));
#46055=CARTESIAN_POINT('Ctrl Pts',(20.7219002254329,15.3384380492012,39.8889828031167));
#46056=CARTESIAN_POINT('Ctrl Pts',(20.7149025360734,15.337935247864,39.8917906612813));
#46057=CARTESIAN_POINT('Ctrl Pts',(20.7040124808177,15.3371582832542,39.8960863966644));
#46058=CARTESIAN_POINT('Ctrl Pts',(20.7001315491789,15.336882475076,39.897602773721));
#46059=CARTESIAN_POINT('Ctrl Pts',(20.692928360163,15.3363726053825,39.9003903736069));
#46060=CARTESIAN_POINT('Ctrl Pts',(20.6896075276151,15.3361383507479,39.9016649710479));
#46061=CARTESIAN_POINT('Ctrl Pts',(20.6820765480582,15.335608918214,39.9045316285624));
#46062=CARTESIAN_POINT('Ctrl Pts',(20.6778643510864,15.3353140710924,39.9061181407743));
#46063=CARTESIAN_POINT('Ctrl Pts',(20.6650790809015,15.3344228645973,39.9108826490856));
#46064=CARTESIAN_POINT('Ctrl Pts',(20.6564887798748,15.3338291585201,39.9140145100043));
#46065=CARTESIAN_POINT('Ctrl Pts',(20.543948400933,15.3261133696095,39.9541404467903));
#46066=CARTESIAN_POINT('Ctrl Pts',(20.4370157988463,15.3194681944235,39.9822171622928));
#46067=CARTESIAN_POINT('Ctrl Pts',(20.2444412014136,15.3077770373346,40.0154699672662));
#46068=CARTESIAN_POINT('Ctrl Pts',(20.1597634307075,15.3027271058219,40.0243834965628));
#46069=CARTESIAN_POINT('Ctrl Pts',(19.9984614643572,15.2929326424395,40.030640553098));
#46070=CARTESIAN_POINT('Ctrl Pts',(19.9220459436619,15.2882187775183,40.0290662181722));
#46071=CARTESIAN_POINT('Ctrl Pts',(19.8271448834909,15.2821649643941,40.0214626798917));
#46072=CARTESIAN_POINT('Ctrl Pts',(19.8083828873996,15.2809585543214,40.0196824121958));
#46073=CARTESIAN_POINT('Ctrl Pts',(19.7811581236177,15.2791928226067,40.0166960578686));
#46074=CARTESIAN_POINT('Ctrl Pts',(19.7726721456242,15.2786402980827,40.0157081165657));
#46075=CARTESIAN_POINT('Ctrl Pts',(19.7578057289366,15.2776684609402,40.0138771929179));
#46076=CARTESIAN_POINT('Ctrl Pts',(19.7514223791438,15.2772499161873,40.0130585822829));
#46077=CARTESIAN_POINT('Ctrl Pts',(19.7390327888985,15.2764350607119,40.011406665313));
#46078=CARTESIAN_POINT('Ctrl Pts',(19.7330261392349,15.2760388671883,40.0105769499638));
#46079=CARTESIAN_POINT('Ctrl Pts',(19.7186676047639,15.2750890153492,40.008524531897));
#46080=CARTESIAN_POINT('Ctrl Pts',(19.7103196947321,15.2745345309396,40.0072753137343));
#46081=CARTESIAN_POINT('Ctrl Pts',(19.680128032732,15.2725208225955,40.0025545145015));
#46082=CARTESIAN_POINT('Ctrl Pts',(19.6583368888801,15.2710515874259,39.9987622299225));
#46083=CARTESIAN_POINT('Ctrl Pts',(19.493958766669,15.2598441958226,39.9672345119551));
#46084=CARTESIAN_POINT('Ctrl Pts',(19.3548743813257,15.2495966812474,39.9238530192994));
#46085=CARTESIAN_POINT('Ctrl Pts',(19.1424040560139,15.2330297591623,39.8302133311163));
#46086=CARTESIAN_POINT('Ctrl Pts',(19.0652655584608,15.2268142796279,39.7897876339777));
#46087=CARTESIAN_POINT('Ctrl Pts',(18.9595704378302,15.2182129055477,39.7249364832432));
#46088=CARTESIAN_POINT('Ctrl Pts',(18.9285864535048,15.2156810605605,39.7046761983854));
#46089=CARTESIAN_POINT('Ctrl Pts',(18.8920556801133,15.2127005252348,39.6792586905437));
#46090=CARTESIAN_POINT('Ctrl Pts',(18.8859339162135,15.2122012149464,39.6749461556205));
#46091=CARTESIAN_POINT('Ctrl Pts',(18.8764542161156,15.2114284691882,39.6681851598062));
#46092=CARTESIAN_POINT('Ctrl Pts',(18.873078901255,15.2111534167321,39.6657613681315));
#46093=CARTESIAN_POINT('Ctrl Pts',(18.8668279200554,15.2106442338538,39.661241895053));
#46094=CARTESIAN_POINT('Ctrl Pts',(18.8639502453261,15.2104099147768,39.6591491823679));
#46095=CARTESIAN_POINT('Ctrl Pts',(18.8574332007428,15.2098794334755,39.6543822122633));
#46096=CARTESIAN_POINT('Ctrl Pts',(18.8537974278094,15.209583607584,39.6517031343314));
#46097=CARTESIAN_POINT('Ctrl Pts',(18.8427684654447,15.2086864931242,39.6435163506903));
#46098=CARTESIAN_POINT('Ctrl Pts',(18.8354051862607,15.2080879097539,39.6379682953233));
#46099=CARTESIAN_POINT('Ctrl Pts',(18.7720914277111,15.2029413207942,39.5895474399158));
#46100=CARTESIAN_POINT('Ctrl Pts',(18.7184828857319,15.1985854926288,39.5436853390429));
#46101=CARTESIAN_POINT('Ctrl Pts',(18.5865458704213,15.1875141749061,39.4176581829229));
#46102=CARTESIAN_POINT('Ctrl Pts',(18.512475459151,15.1809286172461,39.3334292880801));
#46103=CARTESIAN_POINT('Ctrl Pts',(18.4080698552719,15.1702963969616,39.1915240886494));
#46104=CARTESIAN_POINT('Ctrl Pts',(18.3726224065446,15.1663742420883,39.1379342746715));
#46105=CARTESIAN_POINT('Ctrl Pts',(18.3206147686253,15.159994205808,39.050075440991));
#46106=CARTESIAN_POINT('Ctrl Pts',(18.3022805602356,15.1575970177786,39.0169113899435));
#46107=CARTESIAN_POINT('Ctrl Pts',(18.2798264055172,15.1544489441784,38.9733097338618));
#46108=CARTESIAN_POINT('Ctrl Pts',(18.2748035229787,15.1537297213717,38.9633447709798));
#46109=CARTESIAN_POINT('Ctrl Pts',(18.2667871986205,15.1525568119072,38.9470917498654));
#46110=CARTESIAN_POINT('Ctrl Pts',(18.263740804832,15.1521049646905,38.9408299784408));
#46111=CARTESIAN_POINT('Ctrl Pts',(18.2579536251644,15.1512346580685,38.9287690425657));
#46112=CARTESIAN_POINT('Ctrl Pts',(18.2552077241167,15.1508163819025,38.9229724238086));
#46113=CARTESIAN_POINT('Ctrl Pts',(18.248992974397,15.1498573231739,38.9096821232672));
#46114=CARTESIAN_POINT('Ctrl Pts',(18.2455432496341,15.1493158947734,38.9021796880832));
#46115=CARTESIAN_POINT('Ctrl Pts',(18.2365134720629,15.1478741607111,38.8822049071968));
#46116=CARTESIAN_POINT('Ctrl Pts',(18.2310176625595,15.1469710172888,38.8696952154138));
#46117=CARTESIAN_POINT('Ctrl Pts',(18.1868999874683,15.139503517502,38.7663046210797));
#46118=CARTESIAN_POINT('Ctrl Pts',(18.1551815304772,15.1327079376398,38.6726541272111));
#46119=CARTESIAN_POINT('Ctrl Pts',(18.1078542109622,15.1192276954962,38.4871920801643));
#46120=CARTESIAN_POINT('Ctrl Pts',(18.0914391766159,15.1125805430756,38.3958508109507));
#46121=CARTESIAN_POINT('Ctrl Pts',(18.0786747548679,15.103984302572,38.2756352576924));
#46122=CARTESIAN_POINT('Ctrl Pts',(18.0763116895298,15.1019851890267,38.2475188328068));
#46123=CARTESIAN_POINT('Ctrl Pts',(18.0720921829533,15.0971857104321,38.1794526580731));
#46124=CARTESIAN_POINT('Ctrl Pts',(18.0708594130487,15.0944000276961,38.1394752581004));
#46125=CARTESIAN_POINT('Ctrl Pts',(18.0708759804055,15.090145480618,38.0772988364329));
#46126=CARTESIAN_POINT('Ctrl Pts',(18.0712646576823,15.0886427997716,38.0551122559255));
#46127=CARTESIAN_POINT('Ctrl Pts',(18.0722660625258,15.0867171863381,38.0263236714397));
#46128=CARTESIAN_POINT('Ctrl Pts',(18.0725300991515,15.0862766227344,38.0197122702361));
#46129=CARTESIAN_POINT('Ctrl Pts',(18.0730066727158,15.0855751177809,38.009143077628));
#46130=CARTESIAN_POINT('Ctrl Pts',(18.0731973967014,15.0853129989548,38.0051844297204));
#46131=CARTESIAN_POINT('Ctrl Pts',(18.073584451733,15.084814340807,37.9976348441183));
#46132=CARTESIAN_POINT('Ctrl Pts',(18.0737786219787,15.0845776922221,37.9940439110168));
#46133=CARTESIAN_POINT('Ctrl Pts',(18.0742578372785,15.0840236679026,37.9856184792676));
#46134=CARTESIAN_POINT('Ctrl Pts',(18.0745510466235,15.0837067478324,37.9807844860561));
#46135=CARTESIAN_POINT('Ctrl Pts',(18.0755663250056,15.0826766821078,37.9650281339409));
#46136=CARTESIAN_POINT('Ctrl Pts',(18.0763631682835,15.0819675454294,37.9541105650493));
#46137=CARTESIAN_POINT('Ctrl Pts',(18.0784760588321,15.0802943126343,37.9282014080321));
#46138=CARTESIAN_POINT('Ctrl Pts',(18.0798746973229,15.079334306866,37.9132170629736));
#46139=CARTESIAN_POINT('Ctrl Pts',(18.0856182798852,15.0758581357153,37.858598154672));
#46140=CARTESIAN_POINT('Ctrl Pts',(18.0910165316802,15.0733876090198,37.819082286835));
#46141=CARTESIAN_POINT('Ctrl Pts',(18.1188531923818,15.0631320113997,37.6537206717427));
#46142=CARTESIAN_POINT('Ctrl Pts',(18.1525440759779,15.055648475771,37.5300979534588));
#46143=CARTESIAN_POINT('Ctrl Pts',(18.2311988342254,15.0423483810047,37.3244964157323));
#46144=CARTESIAN_POINT('Ctrl Pts',(18.27032214551,15.0366683151079,37.2407709757419));
#46145=CARTESIAN_POINT('Ctrl Pts',(18.3218691396414,15.0299110609312,37.1483687156214));
#46146=CARTESIAN_POINT('Ctrl Pts',(18.3285784148818,15.0290435529437,37.1366334260572));
#46147=CARTESIAN_POINT('Ctrl Pts',(18.3395622441858,15.0276418023127,37.1178816276831));
#46148=CARTESIAN_POINT('Ctrl Pts',(18.3437593355424,15.0271103363201,37.1108200890934));
#46149=CARTESIAN_POINT('Ctrl Pts',(18.351310421068,15.0261613910522,37.0982983027419));
#46150=CARTESIAN_POINT('Ctrl Pts',(18.354646780932,15.025744555277,37.0928275218107));
#46151=CARTESIAN_POINT('Ctrl Pts',(18.3616763252453,15.0248713174555,37.0814290056135));
#46152=CARTESIAN_POINT('Ctrl Pts',(18.3653745615516,15.0244147351359,37.0755045106534));
#46153=CARTESIAN_POINT('Ctrl Pts',(18.3751149949633,15.0232194273196,37.060087555919));
#46154=CARTESIAN_POINT('Ctrl Pts',(18.3812081469487,15.0224788351204,37.050627759859));
#46155=CARTESIAN_POINT('Ctrl Pts',(18.4086797963715,15.0191706397919,37.0087859087772));
#46156=CARTESIAN_POINT('Ctrl Pts',(18.4309483519988,15.0165701166044,36.9770018959075));
#46157=CARTESIAN_POINT('Ctrl Pts',(18.4939313233235,15.0094197570901,36.8926394066831));
#46158=CARTESIAN_POINT('Ctrl Pts',(18.5364272442127,15.0048062870758,36.8414628793917));
#46159=CARTESIAN_POINT('Ctrl Pts',(18.667701780251,14.9911668571237,36.6990320336801));
#46160=CARTESIAN_POINT('Ctrl Pts',(18.7629663621871,14.9819748753686,36.6142423313337));
#46161=CARTESIAN_POINT('Ctrl Pts',(18.9085123176894,14.969351265367,36.5084678973066));
#46162=CARTESIAN_POINT('Ctrl Pts',(18.9523992111517,14.9657084238926,36.4792429210688));
#46163=CARTESIAN_POINT('Ctrl Pts',(19.0047811865298,14.9615923819726,36.447379032057));
#46164=CARTESIAN_POINT('Ctrl Pts',(19.0121602386957,14.9610177427832,36.4429577062959));
#46165=CARTESIAN_POINT('Ctrl Pts',(19.0233997758683,14.9601505970668,36.4363250478059));
#46166=CARTESIAN_POINT('Ctrl Pts',(19.0272386228386,14.9598558514163,36.4340775382926));
#46167=CARTESIAN_POINT('Ctrl Pts',(19.0341582643769,14.9593271720334,36.4300584058574));
#46168=CARTESIAN_POINT('Ctrl Pts',(19.0372361939428,14.9590929368622,36.4282820092776));
#46169=CARTESIAN_POINT('Ctrl Pts',(19.0439692301107,14.9585825664841,36.4244208675977));
#46170=CARTESIAN_POINT('Ctrl Pts',(19.0476262452673,14.9583066522158,36.422339577254));
#46171=CARTESIAN_POINT('Ctrl Pts',(19.0580209409351,14.9575259641974,36.4164686621131));
#46172=CARTESIAN_POINT('Ctrl Pts',(19.0647747253548,14.9570229641856,36.4127074930724));
#46173=CARTESIAN_POINT('Ctrl Pts',(19.1079721456911,14.9538315073299,36.3889899951918));
#46174=CARTESIAN_POINT('Ctrl Pts',(19.1450329642464,14.9512096608562,36.3701731604945));
#46175=CARTESIAN_POINT('Ctrl Pts',(19.2514578480228,14.9439227361318,36.3203952183265));
#46176=CARTESIAN_POINT('Ctrl Pts',(19.3220578546409,14.9393684297755,36.2923231123525));
#46177=CARTESIAN_POINT('Ctrl Pts',(19.3941040816519,14.9348319053408,36.2684889590753));
#46178=CARTESIAN_POINT('',(18.0708709355256,14.9215670950978,38.101670466408));
#46179=CARTESIAN_POINT('Ctrl Pts',(19.3941039945165,14.7625557686229,36.2684889879012));
#46180=CARTESIAN_POINT('Ctrl Pts',(19.3825170814759,14.7633287170362,36.2723221422098));
#46181=CARTESIAN_POINT('Ctrl Pts',(19.3709654940846,14.7641050973507,36.2762655991737));
#46182=CARTESIAN_POINT('Ctrl Pts',(19.3470290856284,14.7657264678271,36.2846914971796));
#46183=CARTESIAN_POINT('Ctrl Pts',(19.3346527248423,14.7665718818522,36.2891910743904));
#46184=CARTESIAN_POINT('Ctrl Pts',(19.3146469097067,14.7679504381129,36.296697217088));
#46185=CARTESIAN_POINT('Ctrl Pts',(19.3069887168908,14.7684810204803,36.2996263878568));
#46186=CARTESIAN_POINT('Ctrl Pts',(19.2933980211644,14.7694278523957,36.3049242347102));
#46187=CARTESIAN_POINT('Ctrl Pts',(19.2874581362398,14.7698434582092,36.3072737380237));
#46188=CARTESIAN_POINT('Ctrl Pts',(19.2760054960788,14.7706482930595,36.3118697051008));
#46189=CARTESIAN_POINT('Ctrl Pts',(19.2704912476441,14.7710373877188,36.3141122733644));
#46190=CARTESIAN_POINT('Ctrl Pts',(19.2559313623455,14.7720689949999,36.3201122617398));
#46191=CARTESIAN_POINT('Ctrl Pts',(19.2469039046818,14.7727129604863,36.3239130754404));
#46192=CARTESIAN_POINT('Ctrl Pts',(19.2113863830722,14.7752640548029,36.3391864217279));
#46193=CARTESIAN_POINT('Ctrl Pts',(19.1851274521977,14.7771888165935,36.3511836938677));
#46194=CARTESIAN_POINT('Ctrl Pts',(19.1193430360133,14.7821124641708,36.3830428096565));
#46195=CARTESIAN_POINT('Ctrl Pts',(19.0802148840544,14.7851365946205,36.4036823668253));
#46196=CARTESIAN_POINT('Ctrl Pts',(18.9526186235064,14.7953188952831,36.4767007375094));
#46197=CARTESIAN_POINT('Ctrl Pts',(18.8676351296202,14.8026426126488,36.5347989567379));
#46198=CARTESIAN_POINT('Ctrl Pts',(18.7080612505083,14.8172795360261,36.6637143537549));
#46199=CARTESIAN_POINT('Ctrl Pts',(18.6336687812491,14.8245678760486,36.734289351721));
#46200=CARTESIAN_POINT('Ctrl Pts',(18.5553319258502,14.8325138185745,36.8214478193331));
#46201=CARTESIAN_POINT('Ctrl Pts',(18.5455668768958,14.8335095128195,36.8325672221919));
#46202=CARTESIAN_POINT('Ctrl Pts',(18.5322585460864,14.8348724550545,36.8480777271274));
#46203=CARTESIAN_POINT('Ctrl Pts',(18.5286054291828,14.8352472149661,36.8523733043125));
#46204=CARTESIAN_POINT('Ctrl Pts',(18.5227964260123,14.8358440728404,36.8592649179751));
#46205=CARTESIAN_POINT('Ctrl Pts',(18.5206284606786,14.8360670350476,36.8618506585018));
#46206=CARTESIAN_POINT('Ctrl Pts',(18.5161297155703,14.8365301187888,36.8672450136462));
#46207=CARTESIAN_POINT('Ctrl Pts',(18.5138001128867,14.836770149891,36.8700545649531));
#46208=CARTESIAN_POINT('Ctrl Pts',(18.5081971783227,14.8373480519452,36.8768509871864));
#46209=CARTESIAN_POINT('Ctrl Pts',(18.5049318057403,14.8376853527562,36.8808444470318));
#46210=CARTESIAN_POINT('Ctrl Pts',(18.4936205515567,14.8388557098299,36.89479158512));
#46211=CARTESIAN_POINT('Ctrl Pts',(18.485657522621,14.8396830909797,36.9048124630799));
#46212=CARTESIAN_POINT('Ctrl Pts',(18.4446693281657,14.8439645510968,36.9574604197185));
#46213=CARTESIAN_POINT('Ctrl Pts',(18.4133393160563,14.8473155636438,37.0013830573589));
#46214=CARTESIAN_POINT('Ctrl Pts',(18.3493137886308,14.8544785413536,37.0996068567846));
#46215=CARTESIAN_POINT('Ctrl Pts',(18.317369987036,14.858265337978,37.1543212235262));
#46216=CARTESIAN_POINT('Ctrl Pts',(18.2565596030849,14.8661437693364,37.271350940125));
#46217=CARTESIAN_POINT('Ctrl Pts',(18.2282122160191,14.8702295591531,37.3338333431942));
#46218=CARTESIAN_POINT('Ctrl Pts',(18.1716566276983,14.8796380772103,37.4785218755403));
#46219=CARTESIAN_POINT('Ctrl Pts',(18.1455556554264,14.8849926744456,37.5613834283294));
#46220=CARTESIAN_POINT('Ctrl Pts',(18.1219729855613,14.8913894558923,37.6587110420034));
#46221=CARTESIAN_POINT('Ctrl Pts',(18.1189589631229,14.8922478408553,37.6717407157426));
#46222=CARTESIAN_POINT('Ctrl Pts',(18.1143218482917,14.893637680983,37.6927810789366));
#46223=CARTESIAN_POINT('Ctrl Pts',(18.1126137308912,14.8941664356862,37.7007727347712));
#46224=CARTESIAN_POINT('Ctrl Pts',(18.1096581721152,14.8951122867157,37.7150437496867));
#46225=CARTESIAN_POINT('Ctrl Pts',(18.1083911062992,14.8955287544917,37.7213189567283));
#46226=CARTESIAN_POINT('Ctrl Pts',(18.1060070083707,14.89633411947,37.7334369229984));
#46227=CARTESIAN_POINT('Ctrl Pts',(18.1048857182964,14.8967228766726,37.7392787783969));
#46228=CARTESIAN_POINT('Ctrl Pts',(18.1025267576376,14.8975628067071,37.7518834695705));
#46229=CARTESIAN_POINT('Ctrl Pts',(18.1012981884257,14.898014261659,37.7586479047967));
#46230=CARTESIAN_POINT('Ctrl Pts',(18.0984106526094,14.899110315052,37.7750445543664));
#46231=CARTESIAN_POINT('Ctrl Pts',(18.0967886934356,14.8997560682308,37.7846830096993));
#46232=CARTESIAN_POINT('Ctrl Pts',(18.0903074014813,14.9024683268269,37.8250711259566));
#46233=CARTESIAN_POINT('Ctrl Pts',(18.0861197531659,14.9045556203006,37.8559223123455));
#46234=CARTESIAN_POINT('Ctrl Pts',(18.0747503038764,14.9115296362581,37.9581971170406));
#46235=CARTESIAN_POINT('Ctrl Pts',(18.0708085194889,14.9165097739879,38.0299123159641));
#46236=CARTESIAN_POINT('Ctrl Pts',(18.0708707248063,14.9215668540041,38.1016722710962));
#46237=CARTESIAN_POINT('Ctrl Pts',(18.0708707232653,14.9215667286563,38.101670492412));
#46238=CARTESIAN_POINT('Ctrl Pts',(18.0710017404283,14.9322293155351,38.2529726133779));
#46239=CARTESIAN_POINT('Ctrl Pts',(18.0889313147645,14.9432227578084,38.4037348986348));
#46240=CARTESIAN_POINT('Ctrl Pts',(18.1288901782916,14.9550052098152,38.5699757315882));
#46241=CARTESIAN_POINT('Ctrl Pts',(18.133777615627,14.9563491307252,38.5890227310713));
#46242=CARTESIAN_POINT('Ctrl Pts',(18.1424976031405,14.9585893130191,38.6209686453709));
#46243=CARTESIAN_POINT('Ctrl Pts',(18.1461753347472,14.9594927965574,38.6339078751857));
#46244=CARTESIAN_POINT('Ctrl Pts',(18.1514796798755,14.9607394923726,38.6518540293113));
#46245=CARTESIAN_POINT('Ctrl Pts',(18.1529917907639,14.9610889061984,38.6568939936875));
#46246=CARTESIAN_POINT('Ctrl Pts',(18.1555933817275,14.9616799838705,38.6654381028776));
#46247=CARTESIAN_POINT('Ctrl Pts',(18.1566722662579,14.9619222527361,38.6689454178969));
#46248=CARTESIAN_POINT('Ctrl Pts',(18.1587555972969,14.962384641447,38.6756499255739));
#46249=CARTESIAN_POINT('Ctrl Pts',(18.1597583721496,14.9626048594809,38.6788475955318));
#46250=CARTESIAN_POINT('Ctrl Pts',(18.1624344337767,14.9631864317609,38.6873038385007));
#46251=CARTESIAN_POINT('Ctrl Pts',(18.1641219756233,14.963546962936,38.6925579215016));
#46252=CARTESIAN_POINT('Ctrl Pts',(18.1701844730051,14.9648206826069,38.7111587070151));
#46253=CARTESIAN_POINT('Ctrl Pts',(18.174682742171,14.965727013232,38.7244651823075));
#46254=CARTESIAN_POINT('Ctrl Pts',(18.2236061562312,14.9752009919015,38.8641398535692));
#46255=CARTESIAN_POINT('Ctrl Pts',(18.2809395216915,14.9831150931849,38.9856222866736));
#46256=CARTESIAN_POINT('Ctrl Pts',(18.385668460247,14.9951847352943,39.1583483003979));
#46257=CARTESIAN_POINT('Ctrl Pts',(18.423976823261,14.9992598497402,39.2145930735379));
#46258=CARTESIAN_POINT('Ctrl Pts',(18.5075294039111,15.0076858888618,39.324321174371));
#46259=CARTESIAN_POINT('Ctrl Pts',(18.5528739008648,15.0120352672345,39.3775974322869));
#46260=CARTESIAN_POINT('Ctrl Pts',(18.610500179791,15.0173862518684,39.4382910508278));
#46261=CARTESIAN_POINT('Ctrl Pts',(18.6201010914718,15.0182722541408,39.4481882930215));
#46262=CARTESIAN_POINT('Ctrl Pts',(18.6342192964939,15.0195676649752,39.4624334529925));
#46263=CARTESIAN_POINT('Ctrl Pts',(18.6386531403675,15.0199734414555,39.4668637716116));
#46264=CARTESIAN_POINT('Ctrl Pts',(18.647670492156,15.0207966307534,39.4757865565823));
#46265=CARTESIAN_POINT('Ctrl Pts',(18.6522549829831,15.0212140841874,39.4802779120552));
#46266=CARTESIAN_POINT('Ctrl Pts',(18.6612404755007,15.0220302707643,39.4889934139346));
#46267=CARTESIAN_POINT('Ctrl Pts',(18.6656392737165,15.0224289028678,39.4932197310939));
#46268=CARTESIAN_POINT('Ctrl Pts',(18.6775253828868,15.0235036268749,39.5045318479923));
#46269=CARTESIAN_POINT('Ctrl Pts',(18.6850494838382,15.0241813769467,39.5115785341292));
#46270=CARTESIAN_POINT('Ctrl Pts',(18.7131687768133,15.026705135967,39.5374936989384));
#46271=CARTESIAN_POINT('Ctrl Pts',(18.7341156938454,15.028567253217,39.555973734906));
#46272=CARTESIAN_POINT('Ctrl Pts',(18.7573490814075,15.0306146182162,39.5755905235295));
#46273=CARTESIAN_POINT('Ctrl Pts',(18.7592457091535,15.0307816237693,39.5771856647896));
#46274=CARTESIAN_POINT('Ctrl Pts',(18.7659970004889,15.0313756470995,39.5828416004334));
#46275=CARTESIAN_POINT('Ctrl Pts',(18.7708685275807,15.0318034437056,39.5868821193089));
#46276=CARTESIAN_POINT('Ctrl Pts',(18.880176702941,15.0413839856123,39.6766397100555));
#46277=CARTESIAN_POINT('Ctrl Pts',(18.993296241773,15.0509644470984,39.7511611698253));
#46278=CARTESIAN_POINT('Ctrl Pts',(19.1858804051716,15.0664383684951,39.8508399462787));
#46279=CARTESIAN_POINT('Ctrl Pts',(19.2608342202858,15.0722704320492,39.8837788136787));
#46280=CARTESIAN_POINT('Ctrl Pts',(19.3712259614628,15.080414670461,39.9241335631306));
#46281=CARTESIAN_POINT('Ctrl Pts',(19.405132556716,15.0828577765018,39.9354708314618));
#46282=CARTESIAN_POINT('Ctrl Pts',(19.4464307297838,15.0857479807396,39.9480147676338));
#46283=CARTESIAN_POINT('Ctrl Pts',(19.4535368266165,15.0862422697861,39.9501285152242));
#46284=CARTESIAN_POINT('Ctrl Pts',(19.4646291628682,15.0870089436822,39.9533585071972));
#46285=CARTESIAN_POINT('Ctrl Pts',(19.4686070135657,15.08728290572,39.9545029480212));
#46286=CARTESIAN_POINT('Ctrl Pts',(19.4760129032362,15.087791108242,39.9566078618513));
#46287=CARTESIAN_POINT('Ctrl Pts',(19.4794398852097,15.0880255309155,39.9575716399306));
#46288=CARTESIAN_POINT('Ctrl Pts',(19.4872421104714,15.0885575743056,39.9597425904262));
#46289=CARTESIAN_POINT('Ctrl Pts',(19.4916189514371,15.088854850465,39.9609438106565));
#46290=CARTESIAN_POINT('Ctrl Pts',(19.505008422866,15.0897607606897,39.9645677759412));
#46291=CARTESIAN_POINT('Ctrl Pts',(19.5140345933868,15.0903666113415,39.9669406215983));
#46292=CARTESIAN_POINT('Ctrl Pts',(19.6015932486645,15.096200031468,39.9892804416742));
#46293=CARTESIAN_POINT('Ctrl Pts',(19.6813037663588,15.10117276984,40.0043488982309));
#46294=CARTESIAN_POINT('Ctrl Pts',(19.9243903049339,15.1159584016255,40.034603883621));
#46295=CARTESIAN_POINT('Ctrl Pts',(20.0889516302879,15.1255187532477,40.034036160001));
#46296=CARTESIAN_POINT('Ctrl Pts',(20.2904168733236,15.1382023105806,40.0075493186322));
#46297=CARTESIAN_POINT('Ctrl Pts',(20.3292050326199,15.1406863681932,40.0012390881905));
#46298=CARTESIAN_POINT('Ctrl Pts',(20.3788653726925,15.1439328975019,39.9915949096823));
#46299=CARTESIAN_POINT('Ctrl Pts',(20.3899399174842,15.1446611493818,39.9893430405516));
#46300=CARTESIAN_POINT('Ctrl Pts',(20.4078358993412,15.1458451434993,39.9855400721729));
#46301=CARTESIAN_POINT('Ctrl Pts',(20.4146699153154,15.1462989800969,39.984048922868));
#46302=CARTESIAN_POINT('Ctrl Pts',(20.4277456025235,15.1471706424426,39.9811212819063));
#46303=CARTESIAN_POINT('Ctrl Pts',(20.4339885366748,15.1475882714966,39.9796908059837));
#46304=CARTESIAN_POINT('Ctrl Pts',(20.4482007201145,15.1485423935251,39.9763597181838));
#46305=CARTESIAN_POINT('Ctrl Pts',(20.4561651747887,15.1490795095595,39.9744393848178));
#46306=CARTESIAN_POINT('Ctrl Pts',(20.4771654052179,15.1505022897096,39.9692341888015));
#46307=CARTESIAN_POINT('Ctrl Pts',(20.490179305898,15.151390674141,39.9658637434479));
#46308=CARTESIAN_POINT('Ctrl Pts',(20.5894197347014,15.158217686716,39.9390517711754));
#46309=CARTESIAN_POINT('Ctrl Pts',(20.673946386771,15.1643440675916,39.9097842745135));
#46310=CARTESIAN_POINT('Ctrl Pts',(20.9049052988862,15.1819521047212,39.8113855113679));
#46311=CARTESIAN_POINT('Ctrl Pts',(21.0451088356389,15.193730133982,39.7295515177725));
#46312=CARTESIAN_POINT('Ctrl Pts',(21.1976432290568,15.2069848038621,39.6126539078794));
#46313=CARTESIAN_POINT('Ctrl Pts',(21.2213892505422,15.2090602884132,39.5935460170333));
#46314=CARTESIAN_POINT('Ctrl Pts',(21.2500727286646,15.2115724485675,39.569323197854));
#46315=CARTESIAN_POINT('Ctrl Pts',(21.2554463438305,15.2120433068556,39.5647344360943));
#46316=CARTESIAN_POINT('Ctrl Pts',(21.2638698556542,15.2127816011059,39.557460823532));
#46317=CARTESIAN_POINT('Ctrl Pts',(21.2669366244723,15.213050434075,39.5547957432197));
#46318=CARTESIAN_POINT('Ctrl Pts',(21.2726833519682,15.2135542303858,39.5497697741118));
#46319=CARTESIAN_POINT('Ctrl Pts',(21.2753651433426,15.213789345003,39.5474111591748));
#46320=CARTESIAN_POINT('Ctrl Pts',(21.281469795115,15.2143245934729,39.5420120252132));
#46321=CARTESIAN_POINT('Ctrl Pts',(21.2848883899372,15.2146243709207,39.5389667623406));
#46322=CARTESIAN_POINT('Ctrl Pts',(21.29391801812,15.2154163881467,39.530865390543));
#46323=CARTESIAN_POINT('Ctrl Pts',(21.2995103225973,15.2159071199763,39.5257883887399));
#46324=CARTESIAN_POINT('Ctrl Pts',(21.3385239143036,15.2193333352411,39.4899494752967));
#46325=CARTESIAN_POINT('Ctrl Pts',(21.3708824305684,15.2221892972435,39.458045629051));
#46326=CARTESIAN_POINT('Ctrl Pts',(21.4228671277103,15.2268642049187,39.4030376060969));
#46327=CARTESIAN_POINT('Ctrl Pts',(21.4431278438082,15.2287101559551,39.380562387515));
#46328=CARTESIAN_POINT('Ctrl Pts',(21.5714959396856,15.2406343612329,39.231245672687));
#46329=CARTESIAN_POINT('Ctrl Pts',(21.6633022064373,15.2503255900376,39.0913338677388));
#46330=CARTESIAN_POINT('Ctrl Pts',(21.7546434489484,15.263362838157,38.9028690596031));
#46331=CARTESIAN_POINT('Ctrl Pts',(21.7720129821099,15.2660622206113,38.86376823612));
#46332=CARTESIAN_POINT('Ctrl Pts',(21.792434012896,15.2695519318515,38.8133429576412));
#46333=CARTESIAN_POINT('Ctrl Pts',(21.7967026416769,15.2703012490666,38.8025222228319));
#46334=CARTESIAN_POINT('Ctrl Pts',(21.8034072256107,15.2715111205582,38.7850656119356));
#46335=CARTESIAN_POINT('Ctrl Pts',(21.8059050662551,15.2719696111923,38.7784536856085));
#46336=CARTESIAN_POINT('Ctrl Pts',(21.8105905219428,15.272844672462,38.7658418000608));
#46337=CARTESIAN_POINT('Ctrl Pts',(21.8127847931839,15.2732610158293,38.7598444004608));
#46338=CARTESIAN_POINT('Ctrl Pts',(21.817724086413,15.2742133799803,38.7461336799947));
#46339=CARTESIAN_POINT('Ctrl Pts',(21.820449850792,15.2747500273393,38.7384135994957));
#46340=CARTESIAN_POINT('Ctrl Pts',(21.8274184041377,15.2761514799716,38.7182692731368));
#46341=CARTESIAN_POINT('Ctrl Pts',(21.8315835931396,15.2770188071101,38.7058188217716));
#46342=CARTESIAN_POINT('Ctrl Pts',(21.8597854138577,15.2831058275555,38.6185686959296));
#46343=CARTESIAN_POINT('Ctrl Pts',(21.8793568689404,15.2884692535588,38.5424139948449));
#46344=CARTESIAN_POINT('Ctrl Pts',(21.9254910035408,15.3054665577556,38.3031809285054));
#46345=CARTESIAN_POINT('Ctrl Pts',(21.9358114740606,15.3174898856621,38.1377515694563));
#46346=CARTESIAN_POINT('Ctrl Pts',(21.9224695882963,15.3315587564005,37.9354676778912));
#46347=CARTESIAN_POINT('Ctrl Pts',(21.9188920251195,15.3341356213825,37.8979750979097));
#46348=CARTESIAN_POINT('Ctrl Pts',(21.9132852138639,15.3371618568658,37.8531420124475));
#46349=CARTESIAN_POINT('Ctrl Pts',(21.9123077759905,15.3376636294777,37.8456810072378));
#46350=CARTESIAN_POINT('Ctrl Pts',(21.9107217499668,15.3384393506288,37.8341009890665));
#46351=CARTESIAN_POINT('Ctrl Pts',(21.9101434537088,15.3387149358281,37.8299780066767));
#46352=CARTESIAN_POINT('Ctrl Pts',(21.9090462781763,15.3392246014857,37.822335598849));
#46353=CARTESIAN_POINT('Ctrl Pts',(21.9085310159957,15.3394588737509,37.8188157664191));
#46354=CARTESIAN_POINT('Ctrl Pts',(21.9073410949495,15.339988610139,37.8108412147191));
#46355=CARTESIAN_POINT('Ctrl Pts',(21.9066605663013,15.3402837418653,37.8063874295647));
#46356=CARTESIAN_POINT('Ctrl Pts',(21.9045483463365,15.3411766665509,37.7928808795931));
#46357=CARTESIAN_POINT('Ctrl Pts',(21.9030677137793,15.341771791164,37.78383573498));
#46358=CARTESIAN_POINT('Ctrl Pts',(21.8830710705866,15.3494319397087,37.6669100944897));
#46359=CARTESIAN_POINT('Ctrl Pts',(21.8554673429379,15.3560278073103,37.560767298052));
#46360=CARTESIAN_POINT('Ctrl Pts',(21.7912119339226,15.367571884396,37.3788443180618));
#46361=CARTESIAN_POINT('Ctrl Pts',(21.7583458000219,15.3725261118798,37.3020492958186));
#46362=CARTESIAN_POINT('Ctrl Pts',(21.6851460026965,15.3823369386165,37.1576749837671));
#46363=CARTESIAN_POINT('Ctrl Pts',(21.6454512378319,15.3871721320615,37.089959618423));
#46364=CARTESIAN_POINT('Ctrl Pts',(21.591097417306,15.3933717965582,37.0089835692151));
#46365=CARTESIAN_POINT('Ctrl Pts',(21.580210683998,15.3945950364533,36.993274200126));
#46366=CARTESIAN_POINT('Ctrl Pts',(21.5640943762968,15.3963809132185,36.9707413237919));
#46367=CARTESIAN_POINT('Ctrl Pts',(21.5590495446857,15.3969365295344,36.9637866005684));
#46368=CARTESIAN_POINT('Ctrl Pts',(21.5501404688064,15.3979119441622,36.9516757431441));
#46369=CARTESIAN_POINT('Ctrl Pts',(21.5462965087628,15.3983309569206,36.9465047996514));
#46370=CARTESIAN_POINT('Ctrl Pts',(21.5387932639153,15.3991453486652,36.9365162455755));
#46371=CARTESIAN_POINT('Ctrl Pts',(21.5351370754279,15.3995406040156,36.931696394712));
#46372=CARTESIAN_POINT('Ctrl Pts',(21.5263577760805,15.4004859914057,36.9202352569944));
#46373=CARTESIAN_POINT('Ctrl Pts',(21.5212139386252,15.4010369320755,36.9136100731111));
#46374=CARTESIAN_POINT('Ctrl Pts',(21.5025614451121,15.4030243280626,36.8899066949334));
#46375=CARTESIAN_POINT('Ctrl Pts',(21.4888074922623,15.4044704564735,36.8730244955106));
#46376=CARTESIAN_POINT('Ctrl Pts',(21.3766317807976,15.4161181427909,36.7399988022156));
#46377=CARTESIAN_POINT('Ctrl Pts',(21.2650796948774,15.4268853085969,36.6356660403599));
#46378=CARTESIAN_POINT('Ctrl Pts',(21.0764793588935,15.4435871507526,36.4970529223805));
#46379=CARTESIAN_POINT('Ctrl Pts',(21.0074762172974,15.449426375672,36.4528083016758));
#46380=CARTESIAN_POINT('Ctrl Pts',(20.90459061463,15.4575792001072,36.3957295971273));
#46381=CARTESIAN_POINT('Ctrl Pts',(20.8728358933348,15.4600240073143,36.3792502532933));
#46382=CARTESIAN_POINT('Ctrl Pts',(20.8339649084032,15.4629159463888,36.3604310673338));
#46383=CARTESIAN_POINT('Ctrl Pts',(20.827272186175,15.4634103337969,36.3572383197009));
#46384=CARTESIAN_POINT('Ctrl Pts',(20.8168147573747,15.4641771266634,36.3523234440498));
#46385=CARTESIAN_POINT('Ctrl Pts',(20.8130627247348,15.4644511100855,36.3505747519457));
#46386=CARTESIAN_POINT('Ctrl Pts',(20.806073533659,15.4649593316861,36.3473446749764));
#46387=CARTESIAN_POINT('Ctrl Pts',(20.8028379338008,15.4651937521809,36.3458601873363));
#46388=CARTESIAN_POINT('Ctrl Pts',(20.7954681761301,15.4657257642825,36.3425036180366));
#46389=CARTESIAN_POINT('Ctrl Pts',(20.7913315165301,15.4660230114962,36.3406371653817));
#46390=CARTESIAN_POINT('Ctrl Pts',(20.7786701451491,15.4669287457539,36.3349780694795));
#46391=CARTESIAN_POINT('Ctrl Pts',(20.7701243172957,15.4675344509599,36.3312325889039));
#46392=CARTESIAN_POINT('Ctrl Pts',(20.6873271554236,15.4733519215207,36.2956579500781));
#46393=CARTESIAN_POINT('Ctrl Pts',(20.6111625681457,15.4783104116689,36.2684562170631));
#46394=CARTESIAN_POINT('Ctrl Pts',(20.3758533671781,15.4930914553543,36.2007396417898));
#46395=CARTESIAN_POINT('Ctrl Pts',(20.2130665747769,15.5026589739064,36.1756669736538));
#46396=CARTESIAN_POINT('Ctrl Pts',(20.0097017635029,15.5153560958906,36.17049248089));
#46397=CARTESIAN_POINT('Ctrl Pts',(19.9703148218189,15.5178456812455,36.1706965404218));
#46398=CARTESIAN_POINT('Ctrl Pts',(19.9196609864837,15.5210984684024,36.1725104108669));
#46399=CARTESIAN_POINT('Ctrl Pts',(19.908362195965,15.5218272841384,36.1730145362958));
#46400=CARTESIAN_POINT('Ctrl Pts',(19.8900818619955,15.5230119706832,36.1739912993739));
#46401=CARTESIAN_POINT('Ctrl Pts',(19.8830972002918,15.5234659316877,36.1744026263949));
#46402=CARTESIAN_POINT('Ctrl Pts',(19.8697240300732,15.5243376809386,36.1752632018185));
#46403=CARTESIAN_POINT('Ctrl Pts',(19.863335206912,15.5247552716585,36.1757062845576));
#46404=CARTESIAN_POINT('Ctrl Pts',(19.8487825357766,15.5257090949591,36.176788391374));
#46405=CARTESIAN_POINT('Ctrl Pts',(19.8406203564623,15.5262459492187,36.1774475979097));
#46406=CARTESIAN_POINT('Ctrl Pts',(19.8190836109324,15.5276675812764,36.1793250722419));
#46407=CARTESIAN_POINT('Ctrl Pts',(19.8057173347676,15.5285550723517,36.1806310546143));
#46408=CARTESIAN_POINT('Ctrl Pts',(19.7040841139346,15.5353440100847,36.1916338423703));
#46409=CARTESIAN_POINT('Ctrl Pts',(19.6165805906557,15.5414307774726,36.2072736473586));
#46410=CARTESIAN_POINT('Ctrl Pts',(19.4845095896841,15.5509787547618,36.2404145359517));
#46411=CARTESIAN_POINT('Ctrl Pts',(19.4390223915042,15.5543337944147,36.2536291837778));
#46412=CARTESIAN_POINT('Ctrl Pts',(19.3941036417061,15.5577020380306,36.2684891046171));
#46413=CARTESIAN_POINT('Origin',(20.,-1.3495818343519,38.1));
#46414=CARTESIAN_POINT('',(19.3941040087494,16.5227836600514,36.2684889831927));
#46415=CARTESIAN_POINT('',(19.3941040086649,16.3533584392964,36.2684889832207));
#46416=CARTESIAN_POINT('',(19.3941040087494,-1.3495818343519,36.2684889831927));
#46417=CARTESIAN_POINT('',(18.0708704087723,15.8870818343519,38.0987441537647));
#46418=CARTESIAN_POINT('Ctrl Pts',(18.0708704087723,15.8870818343519,38.0987441537647));
#46419=CARTESIAN_POINT('Ctrl Pts',(18.0708258299364,15.8915491171253,38.1672225622242));
#46420=CARTESIAN_POINT('Ctrl Pts',(18.0744317560961,15.8960163998987,38.2357215708611));
#46421=CARTESIAN_POINT('Ctrl Pts',(18.0816682478463,15.9004836826721,38.3038279803632));
#46422=CARTESIAN_POINT('Ctrl Pts',(18.0889052732589,15.9049512948898,38.3719394124415));
#46423=CARTESIAN_POINT('Ctrl Pts',(18.0997733431619,15.9094189071075,38.4396577055612));
#46424=CARTESIAN_POINT('Ctrl Pts',(18.1142007319637,15.9138865193252,38.5065755496506));
#46425=CARTESIAN_POINT('Ctrl Pts',(18.12864536736,15.9183594721557,38.5735733877666));
#46426=CARTESIAN_POINT('Ctrl Pts',(18.1466577168547,15.9228324249861,38.6397683902669));
#46427=CARTESIAN_POINT('Ctrl Pts',(18.1681152028847,15.9273053778166,38.7047649518596));
#46428=CARTESIAN_POINT('Ctrl Pts',(18.189585184612,15.9317809354565,38.7697993639888));
#46429=CARTESIAN_POINT('Ctrl Pts',(18.2145041222011,15.9362564930965,38.8336334924981));
#46430=CARTESIAN_POINT('Ctrl Pts',(18.2427009686494,15.9407320507365,38.8958911177505));
#46431=CARTESIAN_POINT('Ctrl Pts',(18.2709554707479,15.9452167597966,38.95827604461));
#46432=CARTESIAN_POINT('Ctrl Pts',(18.3025010510645,15.9497014688567,39.0190775946588));
#46433=CARTESIAN_POINT('Ctrl Pts',(18.3371204938809,15.9541861779167,39.0779439171186));
#46434=CARTESIAN_POINT('Ctrl Pts',(18.3694527402624,15.9583745965186,39.132921128954));
#46435=CARTESIAN_POINT('Ctrl Pts',(18.4044654725367,15.9625630151205,39.1862103874997));
#46436=CARTESIAN_POINT('Ctrl Pts',(18.4419495711134,15.9667514337224,39.2375506221466));
#46437=CARTESIAN_POINT('Ctrl Pts',(18.4818491621624,15.9712097559364,39.2921992450177));
#46438=CARTESIAN_POINT('Ctrl Pts',(18.5247062532375,15.9756680781504,39.3448540605869));
#46439=CARTESIAN_POINT('Ctrl Pts',(18.5702943928871,15.9801264003644,39.3951773754548));
#46440=CARTESIAN_POINT('Ctrl Pts',(18.6181611336226,15.984807559876,39.4480159664622));
#46441=CARTESIAN_POINT('Ctrl Pts',(18.6690388463395,15.9894887193875,39.4982833864635));
#46442=CARTESIAN_POINT('Ctrl Pts',(18.7226143802393,15.9941698788991,39.5456239259672));
#46443=CARTESIAN_POINT('Ctrl Pts',(18.7735011786153,15.9986161102829,39.5905886386518));
#46444=CARTESIAN_POINT('Ctrl Pts',(18.8268211145396,16.0030623416667,39.6329127937645));
#46445=CARTESIAN_POINT('Ctrl Pts',(18.8822667904418,16.0075085730505,39.6723279012823));
#46446=CARTESIAN_POINT('Ctrl Pts',(18.9376789970235,16.0119521205038,39.7117192161987));
#46447=CARTESIAN_POINT('Ctrl Pts',(18.9952139970152,16.016395667957,39.7482046818366));
#46448=CARTESIAN_POINT('Ctrl Pts',(19.054532306503,16.0208392154103,39.7815568374139));
#46449=CARTESIAN_POINT('Ctrl Pts',(19.1138352521738,16.0252816119567,39.8149003545722));
#46450=CARTESIAN_POINT('Ctrl Pts',(19.1749201606235,16.0297240085031,39.8451119313376));
#46451=CARTESIAN_POINT('Ctrl Pts',(19.2374212105004,16.0341664050495,39.8720090707176));
#46452=CARTESIAN_POINT('Ctrl Pts',(19.2999276115479,16.0386091819419,39.8989085129577));
#46453=CARTESIAN_POINT('Ctrl Pts',(19.3638499406723,16.0430519588342,39.9224927620879));
#46454=CARTESIAN_POINT('Ctrl Pts',(19.4288022734454,16.0474947357266,39.9426273942604));
#46455=CARTESIAN_POINT('Ctrl Pts',(19.4938246176439,16.0519423014407,39.9627837293378));
#46456=CARTESIAN_POINT('Ctrl Pts',(19.5598787088476,16.0563898671548,39.9794828822013));
#46457=CARTESIAN_POINT('Ctrl Pts',(19.6265643407354,16.0608374328689,39.9926405800599));
#46458=CARTESIAN_POINT('Ctrl Pts',(19.6932916668657,16.0652877793602,40.005806504582));
#46459=CARTESIAN_POINT('Ctrl Pts',(19.7606508313349,16.0697381258515,40.015426498345));
#46460=CARTESIAN_POINT('Ctrl Pts',(19.8282351350228,16.0741884723427,40.0214680294138));
#46461=CARTESIAN_POINT('Ctrl Pts',(19.8959337368733,16.0786463452329,40.0275197778832));
#46462=CARTESIAN_POINT('Ctrl Pts',(19.9638577454947,16.083104218123,40.029980970682));
#46463=CARTESIAN_POINT('Ctrl Pts',(20.0316000601817,16.0875620910131,40.0288711706842));
#46464=CARTESIAN_POINT('Ctrl Pts',(20.0564818503092,16.0891994702226,40.0284635405234));
#46465=CARTESIAN_POINT('Ctrl Pts',(20.0813391814739,16.090836849432,40.0275746541172));
#46466=CARTESIAN_POINT('Ctrl Pts',(20.106152139383,16.0924742286414,40.0262072267034));
#46467=CARTESIAN_POINT('Ctrl Pts',(20.173713862901,16.0969325508555,40.0224839401367));
#46468=CARTESIAN_POINT('Ctrl Pts',(20.2412129184433,16.1013908730695,40.0151944025013));
#46469=CARTESIAN_POINT('Ctrl Pts',(20.3082427603914,16.1058491952835,40.0043447580641));
#46470=CARTESIAN_POINT('Ctrl Pts',(20.3786229094988,16.1105303547951,39.9929528232027));
#46471=CARTESIAN_POINT('Ctrl Pts',(20.4484851656179,16.1152115143066,39.9776355018037));
#46472=CARTESIAN_POINT('Ctrl Pts',(20.5173606764793,16.1198926738182,39.9584618606076));
#46473=CARTESIAN_POINT('Ctrl Pts',(20.5827796089495,16.124338905202,39.9402504655422));
#46474=CARTESIAN_POINT('Ctrl Pts',(20.6473079064773,16.1287851365858,39.9185606409435));
#46475=CARTESIAN_POINT('Ctrl Pts',(20.7105530140653,16.1332313679696,39.8935041040106));
#46476=CARTESIAN_POINT('Ctrl Pts',(20.7737599442709,16.1376749154228,39.8684626922474));
#46477=CARTESIAN_POINT('Ctrl Pts',(20.8356847635789,16.1421184628761,39.8400587808877));
#46478=CARTESIAN_POINT('Ctrl Pts',(20.8959518693553,16.1465620103294,39.8084533369978));
#46479=CARTESIAN_POINT('Ctrl Pts',(20.9562033655705,16.1510044068758,39.7768560791175));
#46480=CARTESIAN_POINT('Ctrl Pts',(21.014797564158,16.1554468034222,39.7420591639833));
#46481=CARTESIAN_POINT('Ctrl Pts',(21.071382244746,16.1598891999686,39.7042701276727));
#46482=CARTESIAN_POINT('Ctrl Pts',(21.1279717699611,16.164331976861,39.6664778559672));
#46483=CARTESIAN_POINT('Ctrl Pts',(21.1825510270899,16.1687747537533,39.6256932306903));
#46484=CARTESIAN_POINT('Ctrl Pts',(21.234797179945,16.1732175306457,39.5821668196596));
#46485=CARTESIAN_POINT('Ctrl Pts',(21.2870996483701,16.1776650963598,39.5385934919756));
#46486=CARTESIAN_POINT('Ctrl Pts',(21.3370636152442,16.1821126620739,39.4922727980548));
#46487=CARTESIAN_POINT('Ctrl Pts',(21.3844005403343,16.186560227788,39.4434945853341));
#46488=CARTESIAN_POINT('Ctrl Pts',(21.4317670621634,16.1910105742793,39.3946858747298));
#46489=CARTESIAN_POINT('Ctrl Pts',(21.4765029496675,16.1954609207705,39.3434169593205));
#46490=CARTESIAN_POINT('Ctrl Pts',(21.518359532079,16.1999112672618,39.2900112975282));
#46491=CARTESIAN_POINT('Ctrl Pts',(21.5602869020876,16.204369140152,39.2365153164062));
#46492=CARTESIAN_POINT('Ctrl Pts',(21.599324968236,16.2088270130421,39.1808757818233));
#46493=CARTESIAN_POINT('Ctrl Pts',(21.6352685418066,16.2132848859323,39.1234448461338));
#46494=CARTESIAN_POINT('Ctrl Pts',(21.648470636511,16.2149222651417,39.102350431288));
#46495=CARTESIAN_POINT('Ctrl Pts',(21.6612557070673,16.2165596443511,39.0810145693996));
#46496=CARTESIAN_POINT('Ctrl Pts',(21.6736151911431,16.2181970235605,39.0594554439238));
#46497=CARTESIAN_POINT('Ctrl Pts',(21.7072680933499,16.2226553457745,39.0007533867142));
#46498=CARTESIAN_POINT('Ctrl Pts',(21.737895270719,16.2271136679885,38.9401626624699));
#46499=CARTESIAN_POINT('Ctrl Pts',(21.7652805802521,16.2315719902026,38.8780276536762));
#46500=CARTESIAN_POINT('Ctrl Pts',(21.7940346711506,16.2362531497141,38.8127869928512));
#46501=CARTESIAN_POINT('Ctrl Pts',(21.8192139749583,16.2409343092257,38.7458440483039));
#46502=CARTESIAN_POINT('Ctrl Pts',(21.840621216576,16.2456154687372,38.6776297204874));
#46503=CARTESIAN_POINT('Ctrl Pts',(21.8609541168514,16.250061700121,38.6128387890064));
#46504=CARTESIAN_POINT('Ctrl Pts',(21.8778842710905,16.2545079315048,38.5469015495251));
#46505=CARTESIAN_POINT('Ctrl Pts',(21.8912917135977,16.2589541628886,38.4802081153482));
#46506=CARTESIAN_POINT('Ctrl Pts',(21.904691062814,16.2633977103419,38.4135549401073));
#46507=CARTESIAN_POINT('Ctrl Pts',(21.9145718215884,16.2678412577952,38.3461469581401));
#46508=CARTESIAN_POINT('Ctrl Pts',(21.9208645661169,16.2722848052484,38.2783868704155));
#46509=CARTESIAN_POINT('Ctrl Pts',(21.9271556807847,16.2767272017949,38.2106443329817));
#46510=CARTESIAN_POINT('Ctrl Pts',(21.9298605807061,16.2811695983413,38.1425503616818));
#46511=CARTESIAN_POINT('Ctrl Pts',(21.9289616351069,16.2856119948877,38.0745133920303));
#46512=CARTESIAN_POINT('Ctrl Pts',(21.9280626125424,16.29005477178,38.006470597238));
#46513=CARTESIAN_POINT('Ctrl Pts',(21.9235591412097,16.2944975486724,37.9384853068167));
#46514=CARTESIAN_POINT('Ctrl Pts',(21.9154856831222,16.2989403255648,37.8709647305463));
#46515=CARTESIAN_POINT('Ctrl Pts',(21.9074035227406,16.3033878912789,37.8033713745681));
#46516=CARTESIAN_POINT('Ctrl Pts',(21.8957437563881,16.307835456993,37.7362442226867));
#46517=CARTESIAN_POINT('Ctrl Pts',(21.880592464984,16.3122830227071,37.6699830962096));
#46518=CARTESIAN_POINT('Ctrl Pts',(21.8654317004505,16.3167333691984,37.6036805409059));
#46519=CARTESIAN_POINT('Ctrl Pts',(21.846775202115,16.3211837156896,37.5382455625848));
#46520=CARTESIAN_POINT('Ctrl Pts',(21.8247589484297,16.3256340621809,37.474062833005));
#46521=CARTESIAN_POINT('Ctrl Pts',(21.8027054609903,16.3300919350711,37.4097715579841));
#46522=CARTESIAN_POINT('Ctrl Pts',(21.7772810652795,16.3345498079612,37.3467372140123));
#46523=CARTESIAN_POINT('Ctrl Pts',(21.7486694789839,16.3390076808514,37.2853236162928));
#46524=CARTESIAN_POINT('Ctrl Pts',(21.7381604273121,16.3406450600608,37.2627663674526));
#46525=CARTESIAN_POINT('Ctrl Pts',(21.727221832481,16.3422824392702,37.2404275184496));
#46526=CARTESIAN_POINT('Ctrl Pts',(21.7158642872202,16.3439198184796,37.2183241498474));
#46527=CARTESIAN_POINT('Ctrl Pts',(21.6849395044685,16.3483781406936,37.1581402054823));
#46528=CARTESIAN_POINT('Ctrl Pts',(21.6507833706219,16.3528364629077,37.0994663750406));
#46529=CARTESIAN_POINT('Ctrl Pts',(21.6135671226712,16.3572947851217,37.0426714335011));
#46530=CARTESIAN_POINT('Ctrl Pts',(21.5744907202232,16.3619759446332,36.9830377488924));
#46531=CARTESIAN_POINT('Ctrl Pts',(21.5320404435069,16.3666571041448,36.9254762237944));
#46532=CARTESIAN_POINT('Ctrl Pts',(21.4864703771001,16.3713382636563,36.8703869003203));
#46533=CARTESIAN_POINT('Ctrl Pts',(21.443187284755,16.3757844950401,36.8180622832379));
#46534=CARTESIAN_POINT('Ctrl Pts',(21.397090356213,16.380230726424,36.7679681433413));
#46535=CARTESIAN_POINT('Ctrl Pts',(21.3484415432906,16.3846769578078,36.7204174684971));
#46536=CARTESIAN_POINT('Ctrl Pts',(21.299822096819,16.389120505261,36.6728954972217));
#46537=CARTESIAN_POINT('Ctrl Pts',(21.248654173654,16.3935640527143,36.6279142893029));
#46538=CARTESIAN_POINT('Ctrl Pts',(21.1952377967429,16.3980076001676,36.5857512865658));
#46539=CARTESIAN_POINT('Ctrl Pts',(21.1418352550107,16.402449996714,36.5435992043126));
#46540=CARTESIAN_POINT('Ctrl Pts',(21.0861858026918,16.4068923932604,36.5042641834334));
#46541=CARTESIAN_POINT('Ctrl Pts',(21.028622466044,16.4113347898068,36.4679833397758));
#46542=CARTESIAN_POINT('Ctrl Pts',(20.9710542009795,16.4157775666991,36.4316993898507));
#46543=CARTESIAN_POINT('Ctrl Pts',(20.9115721449349,16.4202203435915,36.3984703968417));
#46544=CARTESIAN_POINT('Ctrl Pts',(20.8505366518943,16.4246631204838,36.3684891104344));
#46545=CARTESIAN_POINT('Ctrl Pts',(20.7894353693477,16.4291106861979,36.3384755075187));
#46546=CARTESIAN_POINT('Ctrl Pts',(20.7267777522623,16.433558251912,36.3117168137485));
#46547=CARTESIAN_POINT('Ctrl Pts',(20.6629460546769,16.4380058176261,36.2883584555745));
#46548=CARTESIAN_POINT('Ctrl Pts',(20.5990744472308,16.4424561641174,36.2649854929194));
#46549=CARTESIAN_POINT('Ctrl Pts',(20.534027769881,16.4469065106087,36.2450172410239));
#46550=CARTESIAN_POINT('Ctrl Pts',(20.4682027292008,16.4513568571,36.2285490224778));
#46551=CARTESIAN_POINT('Ctrl Pts',(20.4022663656128,16.4558147299901,36.2120529529808));
#46552=CARTESIAN_POINT('Ctrl Pts',(20.3355494955993,16.4602726028803,36.199068821404));
#46553=CARTESIAN_POINT('Ctrl Pts',(20.2684573160064,16.4647304757704,36.1896405504768));
#46554=CARTESIAN_POINT('Ctrl Pts',(20.2438143208631,16.4663678549799,36.1861775412844));
#46555=CARTESIAN_POINT('Ctrl Pts',(20.2191207186607,16.4680052341893,36.1831937447171));
#46556=CARTESIAN_POINT('Ctrl Pts',(20.1943966037298,16.4696426133987,36.1806895724354));
#46557=CARTESIAN_POINT('Ctrl Pts',(20.127098987393,16.4740994652675,36.1738733597649));
#46558=CARTESIAN_POINT('Ctrl Pts',(20.0593095425683,16.4785563171364,36.1705874988833));
#46559=CARTESIAN_POINT('Ctrl Pts',(19.9914304332523,16.4830131690052,36.1708890339263));
#46560=CARTESIAN_POINT('Ctrl Pts',(19.9236402064552,16.4874641849662,36.1711901741321));
#46561=CARTESIAN_POINT('Ctrl Pts',(19.8557610364843,16.4919152009273,36.175069395944));
#46562=CARTESIAN_POINT('Ctrl Pts',(19.7882002399354,16.4963662168883,36.1825320293323));
#46563=CARTESIAN_POINT('Ctrl Pts',(19.7207080449641,16.5008127132651,36.1899870851245));
#46564=CARTESIAN_POINT('Ctrl Pts',(19.6535340697983,16.5052592096418,36.2010182803379));
#46565=CARTESIAN_POINT('Ctrl Pts',(19.5870837668045,16.5097057060186,36.2155789373753));
#46566=CARTESIAN_POINT('Ctrl Pts',(19.5219362937988,16.5140650240295,36.229854116999));
#46567=CARTESIAN_POINT('Ctrl Pts',(19.4574848266426,16.5184243420404,36.2475214961663));
#46568=CARTESIAN_POINT('Ctrl Pts',(19.3941040087494,16.5227836600514,36.2684889831927));
#46569=CARTESIAN_POINT('Ctrl Pts',(18.0708704684672,15.888364045083,38.0986555789572));
#46570=CARTESIAN_POINT('Ctrl Pts',(18.0708912412105,15.8863049758138,38.0688484639846));
#46571=CARTESIAN_POINT('Ctrl Pts',(18.0716028362428,15.8842285687181,38.0390467538345));
#46572=CARTESIAN_POINT('Ctrl Pts',(18.0806190769073,15.8707814731016,37.8475435862666));
#46573=CARTESIAN_POINT('Ctrl Pts',(18.108562109285,15.8589884944695,37.6874266600154));
#46574=CARTESIAN_POINT('Ctrl Pts',(18.1650638281681,15.8457398489798,37.5037904775019));
#46575=CARTESIAN_POINT('Ctrl Pts',(18.1746331290121,15.8436810920069,37.47510593915));
#46576=CARTESIAN_POINT('Ctrl Pts',(18.1872605696966,15.8411862927403,37.4400242446107));
#46577=CARTESIAN_POINT('Ctrl Pts',(18.1896841193672,15.8407166131998,37.433405178542));
#46578=CARTESIAN_POINT('Ctrl Pts',(18.1935604131709,15.8399797481432,37.4229955302891));
#46579=CARTESIAN_POINT('Ctrl Pts',(18.1949889051835,15.8397111744467,37.4191960772611));
#46580=CARTESIAN_POINT('Ctrl Pts',(18.1976970829768,15.8392075902526,37.4120614032367));
#46581=CARTESIAN_POINT('Ctrl Pts',(18.1989740254791,15.8389724300697,37.4087252666437));
#46582=CARTESIAN_POINT('Ctrl Pts',(18.2019109386235,15.8384367306763,37.4011156739411));
#46583=CARTESIAN_POINT('Ctrl Pts',(18.2035768796426,15.838136550097,37.3968445779438));
#46584=CARTESIAN_POINT('Ctrl Pts',(18.2080355006489,15.8373427614742,37.3855329562127));
#46585=CARTESIAN_POINT('Ctrl Pts',(18.2108544791983,15.8368506721617,37.378502783401));
#46586=CARTESIAN_POINT('Ctrl Pts',(18.2310304380513,15.8333954792238,37.3290319745208));
#46587=CARTESIAN_POINT('Ctrl Pts',(18.249855880067,15.8305134187825,37.2872015364051));
#46588=CARTESIAN_POINT('Ctrl Pts',(18.2830126667148,15.8258883937181,37.2200337155476));
#46589=CARTESIAN_POINT('Ctrl Pts',(18.2964563063084,15.8241158841955,37.1942819596982));
#46590=CARTESIAN_POINT('Ctrl Pts',(18.3732551148158,15.8144771990911,37.0549356056278));
#46591=CARTESIAN_POINT('Ctrl Pts',(18.4473911111264,15.8068583103847,36.9476695806962));
#46592=CARTESIAN_POINT('Ctrl Pts',(18.5644446688361,15.7958651074082,36.8103245298996));
#46593=CARTESIAN_POINT('Ctrl Pts',(18.5986194346535,15.792757314733,36.7732694842231));
#46594=CARTESIAN_POINT('Ctrl Pts',(18.6492168153398,15.7882578975943,36.7225460963469));
#46595=CARTESIAN_POINT('Ctrl Pts',(18.6644772143478,15.7869132016272,36.7077452447665));
#46596=CARTESIAN_POINT('Ctrl Pts',(18.6918729654712,15.7845180812797,36.6820394036079));
#46597=CARTESIAN_POINT('Ctrl Pts',(18.7039080520054,15.7834720983905,36.6710303615469));
#46598=CARTESIAN_POINT('Ctrl Pts',(18.7220785543886,15.7819012294717,36.6548273774493));
#46599=CARTESIAN_POINT('Ctrl Pts',(18.7281093918435,15.7813811980409,36.6495168364326));
#46600=CARTESIAN_POINT('Ctrl Pts',(18.7388183076559,15.7804600449974,36.6402050871432));
#46601=CARTESIAN_POINT('Ctrl Pts',(18.7434827175248,15.7800595726533,36.6361882750554));
#46602=CARTESIAN_POINT('Ctrl Pts',(18.7528300675857,15.7792584791092,36.6282162898978));
#46603=CARTESIAN_POINT('Ctrl Pts',(18.7575127929514,15.7788578702894,36.6242609754751));
#46604=CARTESIAN_POINT('Ctrl Pts',(18.7702376735659,15.7777711216595,36.6136162671512));
#46605=CARTESIAN_POINT('Ctrl Pts',(18.7783154248599,15.7770832565011,36.6069699358751));
#46606=CARTESIAN_POINT('Ctrl Pts',(18.8089611902156,15.7744807752047,36.5821699790695));
#46607=CARTESIAN_POINT('Ctrl Pts',(18.8318820399488,15.7725487276503,36.5644604543241));
#46608=CARTESIAN_POINT('Ctrl Pts',(19.0190996213222,15.756872714049,36.4264269140187));
#46609=CARTESIAN_POINT('Ctrl Pts',(19.2010276616791,15.7420786631794,36.3323620249649));
#46610=CARTESIAN_POINT('Ctrl Pts',(19.3941040321498,15.7277949589794,36.2684889754514));
#46611=CARTESIAN_POINT('Ctrl Pts',(19.3941036417061,15.5577020380306,36.2684891046171));
#46612=CARTESIAN_POINT('Ctrl Pts',(19.2869970961409,15.5657334489655,36.3039218536502));
#46613=CARTESIAN_POINT('Ctrl Pts',(19.1831232854518,15.5738530125418,36.3487083168368));
#46614=CARTESIAN_POINT('Ctrl Pts',(19.0553917185764,15.5838795943166,36.4176528830577));
#46615=CARTESIAN_POINT('Ctrl Pts',(19.0274780399817,15.5860723441457,36.433633304655));
#46616=CARTESIAN_POINT('Ctrl Pts',(18.993831322998,15.5887058060737,36.4540295367776));
#46617=CARTESIAN_POINT('Ctrl Pts',(18.9877083263234,15.5891846387715,36.4577881550207));
#46618=CARTESIAN_POINT('Ctrl Pts',(18.9781335750634,15.5899326002304,36.4637395420871));
#46619=CARTESIAN_POINT('Ctrl Pts',(18.974667628943,15.5902031862987,36.4659091805605));
#46620=CARTESIAN_POINT('Ctrl Pts',(18.9681912005816,15.5907084484641,36.4699920609818));
#46621=CARTESIAN_POINT('Ctrl Pts',(18.9651791590267,15.5909432865005,36.4719026112726));
#46622=CARTESIAN_POINT('Ctrl Pts',(18.9582835531318,15.5914805940458,36.4763033893199));
#46623=CARTESIAN_POINT('Ctrl Pts',(18.9544036140944,15.5917826917262,36.4787991987169));
#46624=CARTESIAN_POINT('Ctrl Pts',(18.9442349812674,15.5925739393219,36.4853919629071));
#46625=CARTESIAN_POINT('Ctrl Pts',(18.9379611040761,15.5930616241092,36.4895117894826));
#46626=CARTESIAN_POINT('Ctrl Pts',(18.8946445730371,15.5964264221926,36.5183193873449));
#46627=CARTESIAN_POINT('Ctrl Pts',(18.8584387820557,15.5992271802138,36.544248451166));
#46628=CARTESIAN_POINT('Ctrl Pts',(18.812831010448,15.6027852741695,36.5793612334981));
#46629=CARTESIAN_POINT('Ctrl Pts',(18.8025831017928,15.603586801466,36.5874176874242));
#46630=CARTESIAN_POINT('Ctrl Pts',(18.6959617403419,15.6119565832057,36.673001423528));
#46631=CARTESIAN_POINT('Ctrl Pts',(18.6071716438318,15.6192085344496,36.7595250644808));
#46632=CARTESIAN_POINT('Ctrl Pts',(18.4846420144578,15.6306457413503,36.9043457506566));
#46633=CARTESIAN_POINT('Ctrl Pts',(18.4446274980962,15.6346721667358,36.956883998806));
#46634=CARTESIAN_POINT('Ctrl Pts',(18.385597510942,15.6412050888006,37.0432417770369));
#46635=CARTESIAN_POINT('Ctrl Pts',(18.3647721701891,15.6436470086323,37.0757622540142));
#46636=CARTESIAN_POINT('Ctrl Pts',(18.3391665132472,15.6468458065496,37.1185210825483));
#46637=CARTESIAN_POINT('Ctrl Pts',(18.3334798199011,15.6475697182027,37.1282082441341));
#46638=CARTESIAN_POINT('Ctrl Pts',(18.3243973422061,15.648748382999,37.1439942430759));
#46639=CARTESIAN_POINT('Ctrl Pts',(18.3209494343859,15.6492012624353,37.1500629125732));
#46640=CARTESIAN_POINT('Ctrl Pts',(18.3143988270053,15.6500722639972,37.1617397378559));
#46641=CARTESIAN_POINT('Ctrl Pts',(18.3112909880277,15.6504901958677,37.167344916303));
#46642=CARTESIAN_POINT('Ctrl Pts',(18.3042594265255,15.6514466535268,37.1801771422932));
#46643=CARTESIAN_POINT('Ctrl Pts',(18.3003538894875,15.6519858131637,37.1874139615466));
#46644=CARTESIAN_POINT('Ctrl Pts',(18.2901370557493,15.6534175664577,37.206638480791));
#46645=CARTESIAN_POINT('Ctrl Pts',(18.2839056546269,15.6543129357391,37.218667897973));
#46646=CARTESIAN_POINT('Ctrl Pts',(18.2356481551378,15.6614265674354,37.3142791795196));
#46647=CARTESIAN_POINT('Ctrl Pts',(18.1996322050242,15.6678514045526,37.4007391986645));
#46648=CARTESIAN_POINT('Ctrl Pts',(18.1196494045866,15.6856107167885,37.6404706421115));
#46649=CARTESIAN_POINT('Ctrl Pts',(18.0881546282936,15.6971993715924,37.7971291161458));
#46650=CARTESIAN_POINT('Ctrl Pts',(18.0741080035625,15.7101467503915,37.9846162497938));
#46651=CARTESIAN_POINT('Ctrl Pts',(18.0725988536963,15.7121076618656,38.013406506713));
#46652=CARTESIAN_POINT('Ctrl Pts',(18.0715274966347,15.7145005989365,38.0491613869317));
#46653=CARTESIAN_POINT('Ctrl Pts',(18.0713570150662,15.714963153547,38.0561023792882));
#46654=CARTESIAN_POINT('Ctrl Pts',(18.0711466967848,15.7156913730726,38.0670792116388));
#46655=CARTESIAN_POINT('Ctrl Pts',(18.0710820472771,15.715958373322,38.0711144320343));
#46656=CARTESIAN_POINT('Ctrl Pts',(18.0709839831674,15.7164606873023,38.0787265745219));
#46657=CARTESIAN_POINT('Ctrl Pts',(18.070947854407,15.7166961410382,38.0823033437412));
#46658=CARTESIAN_POINT('Ctrl Pts',(18.0708878345154,15.7172346571461,38.0905034407253));
#46659=CARTESIAN_POINT('Ctrl Pts',(18.0708706149258,15.7175373470127,38.0951267672208));
#46660=CARTESIAN_POINT('Ctrl Pts',(18.0708687175602,15.7184937220807,38.1097777941016));
#46661=CARTESIAN_POINT('Ctrl Pts',(18.0709456043656,15.7191441023902,38.1198055367509));
#46662=CARTESIAN_POINT('Ctrl Pts',(18.0725489127073,15.7258284678507,38.2234717436469));
#46663=CARTESIAN_POINT('Ctrl Pts',(18.0808141358278,15.7315243111535,38.3168952652223));
#46664=CARTESIAN_POINT('Ctrl Pts',(18.1239389744769,15.7476723293987,38.5823360778873));
#46665=CARTESIAN_POINT('Ctrl Pts',(18.175474274834,15.7579487416281,38.7506564847968));
#46666=CARTESIAN_POINT('Ctrl Pts',(18.2572446703788,15.7703215911005,38.9274842366739));
#46667=CARTESIAN_POINT('Ctrl Pts',(18.2657369204047,15.7715743681337,38.9451377561642));
#46668=CARTESIAN_POINT('Ctrl Pts',(18.2780829696466,15.7733530898951,38.9698325298594));
#46669=CARTESIAN_POINT('Ctrl Pts',(18.2817143116101,15.7738713533578,38.9769841385757));
#46670=CARTESIAN_POINT('Ctrl Pts',(18.2881197570375,15.7747771804813,38.9894065806581));
#46671=CARTESIAN_POINT('Ctrl Pts',(18.2908738881414,15.7751640441944,38.9946876351029));
#46672=CARTESIAN_POINT('Ctrl Pts',(18.2966886942705,15.7759754567683,39.0057127103645));
#46673=CARTESIAN_POINT('Ctrl Pts',(18.299754065628,15.7764001668133,39.0114541562005));
#46674=CARTESIAN_POINT('Ctrl Pts',(18.307115635575,15.7774130159262,39.0250760202525));
#46675=CARTESIAN_POINT('Ctrl Pts',(18.3114378612145,15.77800206908,39.0329421275891));
#46676=CARTESIAN_POINT('Ctrl Pts',(18.3262071033728,15.7799963451693,39.0593821040779));
#46677=CARTESIAN_POINT('Ctrl Pts',(18.3369066344292,15.7814105163175,39.0778123941949));
#46678=CARTESIAN_POINT('Ctrl Pts',(18.3977756341009,15.7892943747446,39.1787711966674));
#46679=CARTESIAN_POINT('Ctrl Pts',(18.4537753268077,15.795975443966,39.2576072008973));
#46680=CARTESIAN_POINT('Ctrl Pts',(18.5988347376314,15.8120167046537,39.4324173471321));
#46681=CARTESIAN_POINT('Ctrl Pts',(18.6922247669043,15.8214620944786,39.5241922487582));
#46682=CARTESIAN_POINT('Ctrl Pts',(18.8273877902515,15.8335304431883,39.6324275422832));
#46683=CARTESIAN_POINT('Ctrl Pts',(18.8614799810774,15.8364540505741,39.6579237378771));
#46684=CARTESIAN_POINT('Ctrl Pts',(18.9024682167112,15.8398058305002,39.6865123538986));
#46685=CARTESIAN_POINT('Ctrl Pts',(18.9085703629601,15.8403007085932,39.6907164474301));
#46686=CARTESIAN_POINT('Ctrl Pts',(18.9184869940928,15.8410980990487,39.6974646142678));
#46687=CARTESIAN_POINT('Ctrl Pts',(18.9222865184618,15.8414020057658,39.7000303836402));
#46688=CARTESIAN_POINT('Ctrl Pts',(18.9290559442393,15.8419405538096,39.7045666357803));
#46689=CARTESIAN_POINT('Ctrl Pts',(18.932022190421,15.8421755475241,39.7065424545358));
#46690=CARTESIAN_POINT('Ctrl Pts',(18.9384188786956,15.8426801756568,39.7107777475625));
#46691=CARTESIAN_POINT('Ctrl Pts',(18.9418510593831,15.8429496286759,39.713034484877));
#46692=CARTESIAN_POINT('Ctrl Pts',(18.9513770459187,15.8436939548103,39.7192545502481));
#46693=CARTESIAN_POINT('Ctrl Pts',(18.9574861632985,15.8441673067411,39.7231944747047));
#46694=CARTESIAN_POINT('Ctrl Pts',(18.9918147323132,15.8468057779922,39.7450600826409));
#46695=CARTESIAN_POINT('Ctrl Pts',(19.0204761370866,15.8489281310645,39.7622856369383));
#46696=CARTESIAN_POINT('Ctrl Pts',(19.1130622147582,15.8555794946669,39.8147031302438));
#46697=CARTESIAN_POINT('Ctrl Pts',(19.1785450580316,15.8599836043246,39.8470200338396));
#46698=CARTESIAN_POINT('Ctrl Pts',(19.3978167480666,15.874256711025,39.9401715287537));
#46699=CARTESIAN_POINT('Ctrl Pts',(19.5575809925073,15.8839960978198,39.9849709489789));
#46700=CARTESIAN_POINT('Ctrl Pts',(19.741617304748,15.8957939248933,40.0118606410352));
#46701=CARTESIAN_POINT('Ctrl Pts',(19.7621863248979,15.8971192127927,40.0145279655806));
#46702=CARTESIAN_POINT('Ctrl Pts',(19.7909587415547,15.8989840057287,40.0177882658027));
#46703=CARTESIAN_POINT('Ctrl Pts',(19.7991294676282,15.899514791359,40.0186612796394));
#46704=CARTESIAN_POINT('Ctrl Pts',(19.813280958913,15.9004363244824,40.0200819314596));
#46705=CARTESIAN_POINT('Ctrl Pts',(19.8192592099493,15.9008263094618,40.0206538962762));
#46706=CARTESIAN_POINT('Ctrl Pts',(19.831683892206,15.9016382905178,40.0217840961897));
#46707=CARTESIAN_POINT('Ctrl Pts',(19.8381306473514,15.9020604215699,40.0223378307354));
#46708=CARTESIAN_POINT('Ctrl Pts',(19.8533099954289,15.9030563484596,40.02356474031));
#46709=CARTESIAN_POINT('Ctrl Pts',(19.8620445700562,15.9036309777231,40.0242108935067));
#46710=CARTESIAN_POINT('Ctrl Pts',(19.8907857816746,15.9055270648773,40.0261403689782));
#46711=CARTESIAN_POINT('Ctrl Pts',(19.9108074904933,15.9068563147904,40.0271712719554));
#46712=CARTESIAN_POINT('Ctrl Pts',(20.0166666201352,15.9139311224526,40.0309687453286));
#46713=CARTESIAN_POINT('Ctrl Pts',(20.1025899923874,15.9198423254634,40.028312663476));
#46714=CARTESIAN_POINT('Ctrl Pts',(20.3225121917313,15.9353708769068,40.006773311396));
#46715=CARTESIAN_POINT('Ctrl Pts',(20.4552192054987,15.9451469449962,39.9795136485195));
#46716=CARTESIAN_POINT('Ctrl Pts',(20.5995649313296,15.9557553068453,39.9336661778171));
#46717=CARTESIAN_POINT('Ctrl Pts',(20.6150811552164,15.9568948008357,39.9285198820794));
#46718=CARTESIAN_POINT('Ctrl Pts',(20.6636095378439,15.9604524176345,39.9117367463128));
#46719=CARTESIAN_POINT('Ctrl Pts',(20.6963737282762,15.9628452633845,39.8993975832509));
#46720=CARTESIAN_POINT('Ctrl Pts',(20.7352565521427,15.9656593243584,39.8835327841649));
#46721=CARTESIAN_POINT('Ctrl Pts',(20.7417124800203,15.9661256939503,39.8808576558203));
#46722=CARTESIAN_POINT('Ctrl Pts',(20.7522616973358,15.9668861735468,39.8764190826822));
#46723=CARTESIAN_POINT('Ctrl Pts',(20.7563635958752,15.967181479647,39.8746764579557));
#46724=CARTESIAN_POINT('Ctrl Pts',(20.7637258773089,15.9677107510131,39.8715185501777));
#46725=CARTESIAN_POINT('Ctrl Pts',(20.7669884039073,15.9679450208548,39.8701084650987));
#46726=CARTESIAN_POINT('Ctrl Pts',(20.7740986930358,15.9684549872236,39.8670120029411));
#46727=CARTESIAN_POINT('Ctrl Pts',(20.7779448407974,15.9687304654288,39.8653220756013));
#46728=CARTESIAN_POINT('Ctrl Pts',(20.7888238260632,15.9695086837216,39.860499588454));
#46729=CARTESIAN_POINT('Ctrl Pts',(20.7958435731577,15.9700096677815,39.8573374295857));
#46730=CARTESIAN_POINT('Ctrl Pts',(20.8400547107147,15.9731586927237,39.8371025577971));
#46731=CARTESIAN_POINT('Ctrl Pts',(20.8767169876627,15.9757421504856,39.8188906625709));
#46732=CARTESIAN_POINT('Ctrl Pts',(21.1017175270485,15.9915914328455,39.6980481150119));
#46733=CARTESIAN_POINT('Ctrl Pts',(21.2724227389719,16.0037652492423,39.5657755505596));
#46734=CARTESIAN_POINT('Ctrl Pts',(21.4221805566214,16.0176209350939,39.403451286135));
#46735=CARTESIAN_POINT('Ctrl Pts',(21.4264586119289,16.0180197334227,39.3987681155713));
#46736=CARTESIAN_POINT('Ctrl Pts',(21.4492062243499,16.0201565495294,39.3736184198046));
#46737=CARTESIAN_POINT('Ctrl Pts',(21.4672578155048,16.0219101934134,39.3527796858451));
#46738=CARTESIAN_POINT('Ctrl Pts',(21.4914029399349,16.024341247279,39.3236686629225));
#46739=CARTESIAN_POINT('Ctrl Pts',(21.4978867322923,16.0250029016052,39.3157232647534));
#46740=CARTESIAN_POINT('Ctrl Pts',(21.508119262313,16.0260615121883,39.3029779437222));
#46741=CARTESIAN_POINT('Ctrl Pts',(21.5119092150417,16.0264568223624,39.2982112361784));
#46742=CARTESIAN_POINT('Ctrl Pts',(21.5196497931874,16.0272709012468,39.2883805425136));
#46743=CARTESIAN_POINT('Ctrl Pts',(21.5235978217379,16.0276897654326,39.2833146173721));
#46744=CARTESIAN_POINT('Ctrl Pts',(21.5326859620323,16.0286625306022,39.2715322570529));
#46745=CARTESIAN_POINT('Ctrl Pts',(21.5378073182029,16.0292171552301,39.2648015864387));
#46746=CARTESIAN_POINT('Ctrl Pts',(21.5539176154117,16.0309826429167,39.2433374095512));
#46747=CARTESIAN_POINT('Ctrl Pts',(21.5647400614439,16.0321998892498,39.2284807876686));
#46748=CARTESIAN_POINT('Ctrl Pts',(21.6174000396667,16.0382827099655,39.1539770830104));
#46749=CARTESIAN_POINT('Ctrl Pts',(21.656042610418,16.0432661215702,39.0921548099639));
#46750=CARTESIAN_POINT('Ctrl Pts',(21.7602152333657,16.0583711125733,38.9023829117062));
#46751=CARTESIAN_POINT('Ctrl Pts',(21.815049972143,16.0687664173458,38.7691517164068));
#46752=CARTESIAN_POINT('Ctrl Pts',(21.8583464299399,16.0798248207854,38.6179550335928));
#46753=CARTESIAN_POINT('Ctrl Pts',(21.8619647960517,16.0807811953353,38.604793010247));
#46754=CARTESIAN_POINT('Ctrl Pts',(21.8765968061019,16.0847865554465,38.5492691126538));
#46755=CARTESIAN_POINT('Ctrl Pts',(21.8863077688563,16.0877958052176,38.506573485836));
#46756=CARTESIAN_POINT('Ctrl Pts',(21.8959661438272,16.091233408145,38.4562453224704));
#46757=CARTESIAN_POINT('Ctrl Pts',(21.8973312991366,16.0917323021278,38.4489015535523));
#46758=CARTESIAN_POINT('Ctrl Pts',(21.8994686545502,16.0925348780592,38.4370201329837));
#46759=CARTESIAN_POINT('Ctrl Pts',(21.9002673136042,16.0928399833277,38.4324874096735));
#46760=CARTESIAN_POINT('Ctrl Pts',(21.9016559350232,16.0933798484322,38.4244379393035));
#46761=CARTESIAN_POINT('Ctrl Pts',(21.9022523758598,16.0936149672875,38.4209223752977));
#46762=CARTESIAN_POINT('Ctrl Pts',(21.9035129904778,16.0941189622365,38.41336500823));
#46763=CARTESIAN_POINT('Ctrl Pts',(21.9041740395822,16.0943876616608,38.4093227457755));
#46764=CARTESIAN_POINT('Ctrl Pts',(21.9059641175534,16.0951277795626,38.3981533321763));
#46765=CARTESIAN_POINT('Ctrl Pts',(21.9070660540942,16.0955977049496,38.3910218140008));
#46766=CARTESIAN_POINT('Ctrl Pts',(21.9129288647931,16.0981807192963,38.3516149174707));
#46767=CARTESIAN_POINT('Ctrl Pts',(21.9169107556176,16.1002531274229,38.3192267528916));
#46768=CARTESIAN_POINT('Ctrl Pts',(21.9268512776214,16.1066780338116,38.2170238135291));
#46769=CARTESIAN_POINT('Ctrl Pts',(21.9298304492828,16.1109152445045,38.146973058454));
#46770=CARTESIAN_POINT('Ctrl Pts',(21.9269596624187,16.1252991119664,37.907136373432));
#46771=CARTESIAN_POINT('Ctrl Pts',(21.902526078526,16.1352823332234,37.7383940334527));
#46772=CARTESIAN_POINT('Ctrl Pts',(21.8508071594415,16.1473439614687,37.5555122877789));
#46773=CARTESIAN_POINT('Ctrl Pts',(21.8449799101426,16.1486405512961,37.5360823714243));
#46774=CARTESIAN_POINT('Ctrl Pts',(21.8363899095221,16.1504705897332,37.5090002257812));
#46775=CARTESIAN_POINT('Ctrl Pts',(21.833883363494,16.1509957333026,37.5012676401687));
#46776=CARTESIAN_POINT('Ctrl Pts',(21.8294471914287,16.1519101756742,37.4878714776959));
#46777=CARTESIAN_POINT('Ctrl Pts',(21.8275399348718,16.1522987403073,37.4822005672105));
#46778=CARTESIAN_POINT('Ctrl Pts',(21.8235099535232,16.1531103893557,37.4704000605686));
#46779=CARTESIAN_POINT('Ctrl Pts',(21.8213826342789,16.1535336203286,37.4642721241306));
#46780=CARTESIAN_POINT('Ctrl Pts',(21.8162790875504,16.1545368745571,37.4498067960898));
#46781=CARTESIAN_POINT('Ctrl Pts',(21.8132763167223,16.1551177660886,37.4414789896335));
#46782=CARTESIAN_POINT('Ctrl Pts',(21.8030994121153,16.1570560499383,37.4138520654741));
#46783=CARTESIAN_POINT('Ctrl Pts',(21.7956738475728,16.1584217208557,37.3946477081509));
#46784=CARTESIAN_POINT('Ctrl Pts',(21.7540038472708,16.16583713931,37.2918038083168));
#46785=CARTESIAN_POINT('Ctrl Pts',(21.7142259252815,16.1720710294932,37.2105418146579));
#46786=CARTESIAN_POINT('Ctrl Pts',(21.6072983958624,16.1870841695487,37.0261189922751));
#46787=CARTESIAN_POINT('Ctrl Pts',(21.535687663546,16.1959494295251,36.9259939225626));
#46788=CARTESIAN_POINT('Ctrl Pts',(21.446113193511,16.2055419127306,36.8230958078543));
#46789=CARTESIAN_POINT('Ctrl Pts',(21.4370710713829,16.2064952558663,36.8129279606627));
#46790=CARTESIAN_POINT('Ctrl Pts',(21.3984569386715,16.2105013188572,36.7704207395617));
#46791=CARTESIAN_POINT('Ctrl Pts',(21.3678925207309,16.2135142061465,36.7389953846546));
#46792=CARTESIAN_POINT('Ctrl Pts',(21.3308925545814,16.2169554499253,36.7034602069073));
#46793=CARTESIAN_POINT('Ctrl Pts',(21.3254734278085,16.2174545122743,36.698315805132));
#46794=CARTESIAN_POINT('Ctrl Pts',(21.3166675937732,16.2182573055299,36.6900531236828));
#46795=CARTESIAN_POINT('Ctrl Pts',(21.3132994395944,16.2185624609764,36.6869153140806));
#46796=CARTESIAN_POINT('Ctrl Pts',(21.3073022842271,16.2191023813366,36.681368261367));
#46797=CARTESIAN_POINT('Ctrl Pts',(21.3046778052385,16.2193375055471,36.6789542240014));
#46798=CARTESIAN_POINT('Ctrl Pts',(21.2990246834704,16.2198414745197,36.6737832559247));
#46799=CARTESIAN_POINT('Ctrl Pts',(21.2959939567884,16.2201101428084,36.67102869375));
#46800=CARTESIAN_POINT('Ctrl Pts',(21.2876007113126,16.2208500869718,36.663448920715));
#46801=CARTESIAN_POINT('Ctrl Pts',(21.2822197962694,16.2213198709107,36.6586440435366));
#46802=CARTESIAN_POINT('Ctrl Pts',(21.2523803710457,16.2239006280113,36.6322983358931));
#46803=CARTESIAN_POINT('Ctrl Pts',(21.2274042923977,16.2259710040507,36.6113483360834));
#46804=CARTESIAN_POINT('Ctrl Pts',(21.1472007481222,16.2323868092534,36.5474651060373));
#46805=CARTESIAN_POINT('Ctrl Pts',(21.0901599992564,16.2366173288045,36.5068939345288));
#46806=CARTESIAN_POINT('Ctrl Pts',(20.8873717884223,16.2510063943458,36.3786613475407));
#46807=CARTESIAN_POINT('Ctrl Pts',(20.7323481303306,16.2610000385843,36.3072099643337));
#46808=CARTESIAN_POINT('Ctrl Pts',(20.5506201225371,16.2730725399204,36.2510082750945));
#46809=CARTESIAN_POINT('Ctrl Pts',(20.531174649527,16.2743674328571,36.2453285033589));
#46810=CARTESIAN_POINT('Ctrl Pts',(20.5038105973388,16.2761954658364,36.2378014492333));
#46811=CARTESIAN_POINT('Ctrl Pts',(20.4959638526631,16.2767203253261,36.2356962656227));
#46812=CARTESIAN_POINT('Ctrl Pts',(20.4823168372403,16.2776344112656,36.2321271967539));
#46813=CARTESIAN_POINT('Ctrl Pts',(20.4765225791104,16.2780229049668,36.2306405988007));
#46814=CARTESIAN_POINT('Ctrl Pts',(20.4644300846062,16.278834540476,36.2275979753454));
#46815=CARTESIAN_POINT('Ctrl Pts',(20.4581307350189,16.2792578294344,36.2260467259486));
#46816=CARTESIAN_POINT('Ctrl Pts',(20.4432125706244,16.2802614650448,36.2224527622065));
#46817=CARTESIAN_POINT('Ctrl Pts',(20.434587334874,16.2808426817892,36.2204375889954));
#46818=CARTESIAN_POINT('Ctrl Pts',(20.4058397606352,16.282783174912,36.2139295514483));
#46819=CARTESIAN_POINT('Ctrl Pts',(20.3856598772002,16.2841507557915,36.2097000101705));
#46820=CARTESIAN_POINT('Ctrl Pts',(20.2764405878086,16.2915842950627,36.1886301936745));
#46821=CARTESIAN_POINT('Ctrl Pts',(20.1863786603329,16.2978354107713,36.1777584165985));
#46822=CARTESIAN_POINT('Ctrl Pts',(20.0037008364913,16.3107178574364,36.1686662355575));
#46823=CARTESIAN_POINT('Ctrl Pts',(19.9112963063757,16.3173377122446,36.1707011108718));
#46824=CARTESIAN_POINT('Ctrl Pts',(19.7338807752746,16.3300094562802,36.1873837410124));
#46825=CARTESIAN_POINT('Ctrl Pts',(19.6489849581971,16.3360532915388,36.2011286245633));
#46826=CARTESIAN_POINT('Ctrl Pts',(19.556151955251,16.3424575820897,36.2226004069515));
#46827=CARTESIAN_POINT('Ctrl Pts',(19.5470400522203,16.3430839158982,36.2247779829559));
#46828=CARTESIAN_POINT('Ctrl Pts',(19.5335308176872,16.3440087721624,36.2281106545147));
#46829=CARTESIAN_POINT('Ctrl Pts',(19.5291212900785,16.3443100588853,36.2292150146577));
#46830=CARTESIAN_POINT('Ctrl Pts',(19.5212648856942,16.3448457472243,36.2312121777692));
#46831=CARTESIAN_POINT('Ctrl Pts',(19.5178165464636,16.3450804867097,36.2320989447926));
#46832=CARTESIAN_POINT('Ctrl Pts',(19.5103695401307,16.3455865873703,36.2340359968137));
#46833=CARTESIAN_POINT('Ctrl Pts',(19.5063717969718,16.3458577564778,36.2350895875706));
#46834=CARTESIAN_POINT('Ctrl Pts',(19.4952366903268,16.3466116892272,36.2380625190705));
#46835=CARTESIAN_POINT('Ctrl Pts',(19.488106829744,16.3470928666756,36.2400100623306));
#46836=CARTESIAN_POINT('Ctrl Pts',(19.4518241462968,16.3495343189641,36.2501452218776));
#46837=CARTESIAN_POINT('Ctrl Pts',(19.4228546889411,16.3514599956209,36.2589777535486));
#46838=CARTESIAN_POINT('Ctrl Pts',(19.3941040086649,16.3533584392964,36.2684889832207));
#46839=CARTESIAN_POINT('Origin',(20.,-1.3495818343519,38.1));
#46840=CARTESIAN_POINT('',(19.3941042778786,17.3167366370521,36.2684888941601));
#46841=CARTESIAN_POINT('',(19.3941038273433,17.1441450759092,36.2684890432051));
#46842=CARTESIAN_POINT('',(19.3941040087494,-1.3495818343519,36.2684889831927));
#46843=CARTESIAN_POINT('',(18.0708706155933,16.6808318343519,38.1015411420322));
#46844=CARTESIAN_POINT('Ctrl Pts',(19.3941042778785,17.3167366370521,36.2684888941601));
#46845=CARTESIAN_POINT('Ctrl Pts',(19.4281871155912,17.3145880936754,36.2572136987753));
#46846=CARTESIAN_POINT('Ctrl Pts',(19.46260186465,17.3124312953361,36.2468841883503));
#46847=CARTESIAN_POINT('Ctrl Pts',(19.5829650804439,17.304887334255,36.2143977898005));
#46848=CARTESIAN_POINT('Ctrl Pts',(19.6701023250286,17.2994185812263,36.1972182799032));
#46849=CARTESIAN_POINT('Ctrl Pts',(19.7714268990586,17.2928953712717,36.18441204836));
#46850=CARTESIAN_POINT('Ctrl Pts',(19.7847656655755,17.2920335568093,36.18286749816));
#46851=CARTESIAN_POINT('Ctrl Pts',(19.8062624355353,17.2906392378957,36.1806054706029));
#46852=CARTESIAN_POINT('Ctrl Pts',(19.8144109346658,17.2901094624296,36.179800453392));
#46853=CARTESIAN_POINT('Ctrl Pts',(19.8289411902752,17.2891624473647,36.1784583133964));
#46854=CARTESIAN_POINT('Ctrl Pts',(19.8353209993806,17.2887458419386,36.1779010444703));
#46855=CARTESIAN_POINT('Ctrl Pts',(19.8486769192441,17.2878719685739,36.1768014034601));
#46856=CARTESIAN_POINT('Ctrl Pts',(19.8556534306891,17.2874145147964,36.1762651996013));
#46857=CARTESIAN_POINT('Ctrl Pts',(19.8739153474177,17.28621442272,36.1749615157659));
#46858=CARTESIAN_POINT('Ctrl Pts',(19.8852047239045,17.2854698900579,36.174255328249));
#46859=CARTESIAN_POINT('Ctrl Pts',(19.9358376520919,17.2821183369448,36.1715348821427));
#46860=CARTESIAN_POINT('Ctrl Pts',(19.9752287091522,17.2794773243628,36.1706269110206));
#46861=CARTESIAN_POINT('Ctrl Pts',(20.1787082841269,17.265650624921,36.1721687849205));
#46862=CARTESIAN_POINT('Ctrl Pts',(20.3419495258714,17.253858496796,36.194344631026));
#46863=CARTESIAN_POINT('Ctrl Pts',(20.5783598985063,17.2364751141869,36.2578375345807));
#46864=CARTESIAN_POINT('Ctrl Pts',(20.6549620945363,17.2308080596357,36.2836601153899));
#46865=CARTESIAN_POINT('Ctrl Pts',(20.7383646899343,17.2247527887509,36.317740987687));
#46866=CARTESIAN_POINT('Ctrl Pts',(20.7469757608084,17.2241290478238,36.3213328519177));
#46867=CARTESIAN_POINT('Ctrl Pts',(20.7597361889154,17.2232072659518,36.3267645180577));
#46868=CARTESIAN_POINT('Ctrl Pts',(20.7639055024686,17.2229064868673,36.328556651905));
#46869=CARTESIAN_POINT('Ctrl Pts',(20.7713340820626,17.2223713488074,36.3317808496668));
#46870=CARTESIAN_POINT('Ctrl Pts',(20.7745957361451,17.2221366547824,36.333207234558));
#46871=CARTESIAN_POINT('Ctrl Pts',(20.7816416246043,17.2216302521696,36.3363118009727));
#46872=CARTESIAN_POINT('Ctrl Pts',(20.7854244030634,17.2213587377764,36.337993132655));
#46873=CARTESIAN_POINT('Ctrl Pts',(20.7959682379737,17.2206028700787,36.3427202531467));
#46874=CARTESIAN_POINT('Ctrl Pts',(20.8027172779841,17.2201201162039,36.3457929083102));
#46875=CARTESIAN_POINT('Ctrl Pts',(20.84191862705,17.2173213742833,36.3639138361014));
#46876=CARTESIAN_POINT('Ctrl Pts',(20.8739674772866,17.2150544910922,36.3798246057999));
#46877=CARTESIAN_POINT('Ctrl Pts',(20.9778730853969,17.2077154139262,36.4350632768938));
#46878=CARTESIAN_POINT('Ctrl Pts',(21.0476732303559,17.2027997698563,36.4780773414972));
#46879=CARTESIAN_POINT('Ctrl Pts',(21.2387556794776,17.1888041565934,36.6133293554147));
#46880=CARTESIAN_POINT('Ctrl Pts',(21.3521221612718,17.1797765042327,36.715635660708));
#46881=CARTESIAN_POINT('Ctrl Pts',(21.4666200602742,17.1687542590053,36.8465877075465));
#46882=CARTESIAN_POINT('Ctrl Pts',(21.4806748970894,17.1673637889837,36.8632225082155));
#46883=CARTESIAN_POINT('Ctrl Pts',(21.4997488994942,17.1654219495028,36.8865890421413));
#46884=CARTESIAN_POINT('Ctrl Pts',(21.5050106001505,17.1648802892535,36.8931213797629));
#46885=CARTESIAN_POINT('Ctrl Pts',(21.5139936709352,17.163945031626,36.904423853835));
#46886=CARTESIAN_POINT('Ctrl Pts',(21.517735540974,17.1635522521395,36.9091776021621));
#46887=CARTESIAN_POINT('Ctrl Pts',(21.5254163031002,17.1627393173712,36.919030409412));
#46888=CARTESIAN_POINT('Ctrl Pts',(21.5293521288331,17.1623190485116,36.9241317522757));
#46889=CARTESIAN_POINT('Ctrl Pts',(21.5384763259027,17.1613360186798,36.9360812027116));
#46890=CARTESIAN_POINT('Ctrl Pts',(21.5436446186186,17.1607724854494,36.9429444008907));
#46891=CARTESIAN_POINT('Ctrl Pts',(21.5601610435394,17.1589496089931,36.9651848987605));
#46892=CARTESIAN_POINT('Ctrl Pts',(21.5713262743592,17.1576832814578,36.9806959792602));
#46893=CARTESIAN_POINT('Ctrl Pts',(21.6271218040417,17.1511757134947,37.0606892435713));
#46894=CARTESIAN_POINT('Ctrl Pts',(21.6680153232685,17.1457972521931,37.1276758365361));
#46895=CARTESIAN_POINT('Ctrl Pts',(21.7437826644862,17.1344675250176,37.2707053720839));
#46896=CARTESIAN_POINT('Ctrl Pts',(21.7780204811686,17.1285129506588,37.3469069363996));
#46897=CARTESIAN_POINT('Ctrl Pts',(21.845512231974,17.1147494020431,37.5276279218981));
#46898=CARTESIAN_POINT('Ctrl Pts',(21.8750164121986,17.1069615102386,37.6332618751013));
#46899=CARTESIAN_POINT('Ctrl Pts',(21.8971077617695,17.0989890865743,37.7498447409936));
#46900=CARTESIAN_POINT('Ctrl Pts',(21.8987500320998,17.098376455114,37.7588623607206));
#46901=CARTESIAN_POINT('Ctrl Pts',(21.9011036501247,17.0974678623231,37.7723297879298));
#46902=CARTESIAN_POINT('Ctrl Pts',(21.9018637507879,17.0971692735105,37.7767707766027));
#46903=CARTESIAN_POINT('Ctrl Pts',(21.9031961446014,17.096636499546,37.7847229045073));
#46904=CARTESIAN_POINT('Ctrl Pts',(21.9037742888977,17.0964019915165,37.7882329886122));
#46905=CARTESIAN_POINT('Ctrl Pts',(21.905007978081,17.0958942368306,37.7958544873169));
#46906=CARTESIAN_POINT('Ctrl Pts',(21.9056599229384,17.0956211937426,37.79996642129));
#46907=CARTESIAN_POINT('Ctrl Pts',(21.9074527515177,17.0948567319759,37.8115157322452));
#46908=CARTESIAN_POINT('Ctrl Pts',(21.90856345719,17.0943669721446,37.8189578209101));
#46909=CARTESIAN_POINT('Ctrl Pts',(21.9149698209953,17.0914402952128,37.8636730003941));
#46910=CARTESIAN_POINT('Ctrl Pts',(21.9192174248217,17.0890578768056,37.9010909816715));
#46911=CARTESIAN_POINT('Ctrl Pts',(21.9361722578641,17.076441613781,38.1030481244513));
#46912=CARTESIAN_POINT('Ctrl Pts',(21.9288237836707,17.066909168669,38.2685877918623));
#46913=CARTESIAN_POINT('Ctrl Pts',(21.886992507127,17.0520938115641,38.508635064019));
#46914=CARTESIAN_POINT('Ctrl Pts',(21.8687754774423,17.047224201557,38.5851796416428));
#46915=CARTESIAN_POINT('Ctrl Pts',(21.8421278896749,17.0413627331971,38.6729570505444));
#46916=CARTESIAN_POINT('Ctrl Pts',(21.8381857813128,17.0405198042687,38.6854809675704));
#46917=CARTESIAN_POINT('Ctrl Pts',(21.8315783806381,17.039144505992,38.7057476598368));
#46918=CARTESIAN_POINT('Ctrl Pts',(21.8289910464911,17.0386146764053,38.7135155582986));
#46919=CARTESIAN_POINT('Ctrl Pts',(21.8242977037496,17.0376686871039,38.7273127048152));
#46920=CARTESIAN_POINT('Ctrl Pts',(21.8222110437213,17.0372531668932,38.7333484444092));
#46921=CARTESIAN_POINT('Ctrl Pts',(21.8177519505329,17.0363756875683,38.7460420717497));
#46922=CARTESIAN_POINT('Ctrl Pts',(21.8153728250399,17.0359135131126,38.7526974919599));
#46923=CARTESIAN_POINT('Ctrl Pts',(21.8089817574152,17.034687518446,38.7702707301721));
#46924=CARTESIAN_POINT('Ctrl Pts',(21.8049076032049,17.0339216514101,38.7811654602706));
#46925=CARTESIAN_POINT('Ctrl Pts',(21.7853930729776,17.0303242772647,38.8319448833872));
#46926=CARTESIAN_POINT('Ctrl Pts',(21.7687286524114,17.0274523476216,38.8713431151353));
#46927=CARTESIAN_POINT('Ctrl Pts',(21.6807703592888,17.0131834111643,39.0614242660291));
#46928=CARTESIAN_POINT('Ctrl Pts',(21.5914669370899,17.001172778885,39.202969059165));
#46929=CARTESIAN_POINT('Ctrl Pts',(21.4661724424056,16.9872604410897,39.3540981044645));
#46930=CARTESIAN_POINT('Ctrl Pts',(21.4467014677595,16.9851676096115,39.3765103494249));
#46931=CARTESIAN_POINT('Ctrl Pts',(21.3957926806449,16.9798835546014,39.4324476308416));
#46932=CARTESIAN_POINT('Ctrl Pts',(21.3636577081549,16.9767201228571,39.4653176688622));
#46933=CARTESIAN_POINT('Ctrl Pts',(21.3248885332307,16.9731280992817,39.5022376274033));
#46934=CARTESIAN_POINT('Ctrl Pts',(21.3193696432545,16.9726218326444,39.5074316105119));
#46935=CARTESIAN_POINT('Ctrl Pts',(21.3104623290637,16.9718130301125,39.5157160978284));
#46936=CARTESIAN_POINT('Ctrl Pts',(21.3070933115626,16.9715089982495,39.518827213402));
#46937=CARTESIAN_POINT('Ctrl Pts',(21.3010801010035,16.9709697336735,39.5243405102416));
#46938=CARTESIAN_POINT('Ctrl Pts',(21.2984402946963,16.9707341501535,39.5267473918853));
#46939=CARTESIAN_POINT('Ctrl Pts',(21.2927872830349,16.9702321323524,39.5318729228909));
#46940=CARTESIAN_POINT('Ctrl Pts',(21.2897721854437,16.9699658593025,39.5345893966195));
#46941=CARTESIAN_POINT('Ctrl Pts',(21.281499594735,16.9692392544401,39.5419954848587));
#46942=CARTESIAN_POINT('Ctrl Pts',(21.2762248848906,16.968780327066,39.5466659035823));
#46943=CARTESIAN_POINT('Ctrl Pts',(21.2482171053427,16.9663657139601,39.5711926000204));
#46944=CARTESIAN_POINT('Ctrl Pts',(21.2250444879024,16.964444714477,39.5905434770603));
#46945=CARTESIAN_POINT('Ctrl Pts',(21.0747367525486,16.9523928928381,39.7101872467629));
#46946=CARTESIAN_POINT('Ctrl Pts',(20.9358428206229,16.9430217029138,39.7946895349736));
#46947=CARTESIAN_POINT('Ctrl Pts',(20.7064178950063,16.9278169286061,39.8973610059144));
#46948=CARTESIAN_POINT('Ctrl Pts',(20.6223981801577,16.9223089650795,39.9281548646624));
#46949=CARTESIAN_POINT('Ctrl Pts',(20.5236107877748,16.9157405151792,39.9567595060637));
#46950=CARTESIAN_POINT('Ctrl Pts',(20.5106292669834,16.9148757410076,39.9603714299476));
#46951=CARTESIAN_POINT('Ctrl Pts',(20.489686815378,16.9134775584102,39.9659626609822));
#46952=CARTESIAN_POINT('Ctrl Pts',(20.4817490886396,16.9129469037005,39.9680277410985));
#46953=CARTESIAN_POINT('Ctrl Pts',(20.4675886719125,16.9119988853508,39.9716154595967));
#46954=CARTESIAN_POINT('Ctrl Pts',(20.461371074914,16.9115821607335,39.9731578482037));
#46955=CARTESIAN_POINT('Ctrl Pts',(20.4483530300245,16.9107086209183,39.9763184648224));
#46956=CARTESIAN_POINT('Ctrl Pts',(20.4415512495908,16.9102516227865,39.9779307529276));
#46957=CARTESIAN_POINT('Ctrl Pts',(20.4237505924778,16.9090540319972,39.9820481508835));
#46958=CARTESIAN_POINT('Ctrl Pts',(20.4127383702476,16.908311559457,39.9844937875892));
#46959=CARTESIAN_POINT('Ctrl Pts',(20.3634782489339,16.9049827500904,39.9949811819017));
#46960=CARTESIAN_POINT('Ctrl Pts',(20.3250150257307,16.9023629858092,40.0019555659445));
#46961=CARTESIAN_POINT('Ctrl Pts',(20.21992409561,16.8951438960991,40.0177305136863));
#46962=CARTESIAN_POINT('Ctrl Pts',(20.1530102890439,16.8904794074338,40.0242253433794));
#46963=CARTESIAN_POINT('Ctrl Pts',(19.9689033532457,16.8774972245874,40.0324313494698));
#46964=CARTESIAN_POINT('Ctrl Pts',(19.8516811132925,16.8690544046441,40.0269815365718));
#46965=CARTESIAN_POINT('Ctrl Pts',(19.7218971844104,16.8598193273474,40.0090298512959));
#46966=CARTESIAN_POINT('Ctrl Pts',(19.7081354343519,16.858841788071,40.0069743675738));
#46967=CARTESIAN_POINT('Ctrl Pts',(19.6468562091218,16.854499593023,39.9971426709642));
#46968=CARTESIAN_POINT('Ctrl Pts',(19.5996129992631,16.8511803084583,39.9877372672365));
#46969=CARTESIAN_POINT('Ctrl Pts',(19.5453030545746,16.8474335774071,39.9747938876659));
#46970=CARTESIAN_POINT('Ctrl Pts',(19.5378495243433,16.8469209070608,39.972970468549));
#46971=CARTESIAN_POINT('Ctrl Pts',(19.5259321670112,16.8461038785093,39.9699795537022));
#46972=CARTESIAN_POINT('Ctrl Pts',(19.5214613974063,16.8457979766243,39.9688404555933));
#46973=CARTESIAN_POINT('Ctrl Pts',(19.5135328720823,16.845256612305,39.9667900460725));
#46974=CARTESIAN_POINT('Ctrl Pts',(19.5100735145414,16.8450207889507,39.965885147141));
#46975=CARTESIAN_POINT('Ctrl Pts',(19.5027095711172,16.8445196230953,39.9639369945216));
#46976=CARTESIAN_POINT('Ctrl Pts',(19.4988057473897,16.8442544348125,39.9628910897039));
#46977=CARTESIAN_POINT('Ctrl Pts',(19.4881793775291,16.8435338534812,39.9600082723597));
#46978=CARTESIAN_POINT('Ctrl Pts',(19.4814633710813,16.8430798261188,39.9581471661116));
#46979=CARTESIAN_POINT('Ctrl Pts',(19.4466954266358,16.8407358893149,39.9483092637592));
#46980=CARTESIAN_POINT('Ctrl Pts',(19.4188151889925,16.8388783010891,39.9397330034957));
#46981=CARTESIAN_POINT('Ctrl Pts',(19.3356094989334,16.8333711660076,39.9120575064723));
#46982=CARTESIAN_POINT('Ctrl Pts',(19.280945267054,16.8298020628967,39.8910690970269));
#46983=CARTESIAN_POINT('Ctrl Pts',(19.0761997057163,16.816330260708,39.80156849493));
#46984=CARTESIAN_POINT('Ctrl Pts',(18.9341882198839,16.8067016513006,39.7164115031853));
#46985=CARTESIAN_POINT('Ctrl Pts',(18.7999675471508,16.796001752138,39.6104640384852));
#46986=CARTESIAN_POINT('Ctrl Pts',(18.7952145825897,16.7956206545821,39.6066756771933));
#46987=CARTESIAN_POINT('Ctrl Pts',(18.787140488361,16.7949694397525,39.6001775674453));
#46988=CARTESIAN_POINT('Ctrl Pts',(18.7838103236156,16.7946997258505,39.5974790814781));
#46989=CARTESIAN_POINT('Ctrl Pts',(18.7757232510012,16.7940419789368,39.5908812266464));
#46990=CARTESIAN_POINT('Ctrl Pts',(18.77097596805,16.7936535222693,39.5869701804986));
#46991=CARTESIAN_POINT('Ctrl Pts',(18.7486382180114,16.7918143952374,39.5683871893661));
#46992=CARTESIAN_POINT('Ctrl Pts',(18.7312918630492,16.7903529082178,39.5534258975904));
#46993=CARTESIAN_POINT('Ctrl Pts',(18.7071292097087,16.7882670030527,39.531823333334));
#46994=CARTESIAN_POINT('Ctrl Pts',(18.7000888825141,16.7876530336796,39.5254346774271));
#46995=CARTESIAN_POINT('Ctrl Pts',(18.6887199836951,16.7866512888932,39.5149638410944));
#46996=CARTESIAN_POINT('Ctrl Pts',(18.6843625108631,16.7862648442354,39.5109131612635));
#46997=CARTESIAN_POINT('Ctrl Pts',(18.6756218710228,16.7854845848731,39.5027122173662));
#46998=CARTESIAN_POINT('Ctrl Pts',(18.6712393084315,16.785090749409,39.4985614095984));
#46999=CARTESIAN_POINT('Ctrl Pts',(18.6607374380898,16.7841406426356,39.4885209686807));
#47000=CARTESIAN_POINT('Ctrl Pts',(18.6546374464177,16.7835835161957,39.4826114008394));
#47001=CARTESIAN_POINT('Ctrl Pts',(18.6352255108945,16.7817934739054,39.463555347721));
#47002=CARTESIAN_POINT('Ctrl Pts',(18.6220660503181,16.7805538975073,39.4502557465257));
#47003=CARTESIAN_POINT('Ctrl Pts',(18.5915747533609,16.7776185452663,39.4185297527463));
#47004=CARTESIAN_POINT('Ctrl Pts',(18.5744081437317,16.7759160735809,39.3999500538575));
#47005=CARTESIAN_POINT('Ctrl Pts',(18.5144420850611,16.7697857674479,39.3324311869077));
#47006=CARTESIAN_POINT('Ctrl Pts',(18.4737605416144,16.7652784345264,39.2816770242643));
#47007=CARTESIAN_POINT('Ctrl Pts',(18.3553176578211,16.7510396579551,39.1175650204416));
#47008=CARTESIAN_POINT('Ctrl Pts',(18.2870491594544,16.7410914972882,38.9978953179414));
#47009=CARTESIAN_POINT('Ctrl Pts',(18.213946410057,16.7283350701578,38.8304838333039));
#47010=CARTESIAN_POINT('Ctrl Pts',(18.1972867661624,16.725218063774,38.7883457049693));
#47011=CARTESIAN_POINT('Ctrl Pts',(18.1795995125193,16.7216725343194,38.7385464366185));
#47012=CARTESIAN_POINT('Ctrl Pts',(18.1771159181849,16.721168515013,38.7314215037241));
#47013=CARTESIAN_POINT('Ctrl Pts',(18.1731933416226,16.7203626014581,38.7199523600361));
#47014=CARTESIAN_POINT('Ctrl Pts',(18.1717279325836,16.7200592278309,38.7156173684854));
#47015=CARTESIAN_POINT('Ctrl Pts',(18.1691463606597,16.719520699493,38.7078900076647));
#47016=CARTESIAN_POINT('Ctrl Pts',(18.1680241782992,16.7192851975376,38.7044997101753));
#47017=CARTESIAN_POINT('Ctrl Pts',(18.165644958836,16.7187828667323,38.6972442204242));
#47018=CARTESIAN_POINT('Ctrl Pts',(18.1643907222123,16.7185162016301,38.6933781727775));
#47019=CARTESIAN_POINT('Ctrl Pts',(18.1609874359256,16.717787417369,38.6827738564739));
#47020=CARTESIAN_POINT('Ctrl Pts',(18.158863182502,16.7173267167846,38.6760276049391));
#47021=CARTESIAN_POINT('Ctrl Pts',(18.1477572945606,16.7148858924912,38.6400681310749));
#47022=CARTESIAN_POINT('Ctrl Pts',(18.1394331483969,16.7129413547455,38.6106543561473));
#47023=CARTESIAN_POINT('Ctrl Pts',(18.0914719636826,16.70088054343,38.424395222669));
#47024=CARTESIAN_POINT('Ctrl Pts',(18.0709952650174,16.6915185538119,38.2632773658475));
#47025=CARTESIAN_POINT('Ctrl Pts',(18.0708705729314,16.6817303897375,38.101486781031));
#47026=CARTESIAN_POINT('Ctrl Pts',(19.3941040087494,16.5227836600514,36.2684889831927));
#47027=CARTESIAN_POINT('Ctrl Pts',(19.3295148449261,16.5272260878162,36.2898562122619));
#47028=CARTESIAN_POINT('Ctrl Pts',(19.2660380494538,16.531668515581,36.3146505999152));
#47029=CARTESIAN_POINT('Ctrl Pts',(19.2040551538421,16.5361109433459,36.3427253035525));
#47030=CARTESIAN_POINT('Ctrl Pts',(19.1420684686983,16.5405536427134,36.3708017236309));
#47031=CARTESIAN_POINT('Ctrl Pts',(19.0815763128461,16.544996342081,36.4021586519863));
#47032=CARTESIAN_POINT('Ctrl Pts',(19.0229383238685,16.5494390414485,36.4366019604631));
#47033=CARTESIAN_POINT('Ctrl Pts',(18.964238019985,16.5538864620966,36.4710818720289));
#47034=CARTESIAN_POINT('Ctrl Pts',(18.9073962411138,16.5583338827446,36.5086544587853));
#47035=CARTESIAN_POINT('Ctrl Pts',(18.8527452760582,16.5627813033926,36.5490811899737));
#47036=CARTESIAN_POINT('Ctrl Pts',(18.7980613409524,16.5672314070982,36.5895323099604));
#47037=CARTESIAN_POINT('Ctrl Pts',(18.7455712304066,16.5716815108037,36.6328406872743));
#47038=CARTESIAN_POINT('Ctrl Pts',(18.6955734437814,16.5761316145093,36.6787280639048));
#47039=CARTESIAN_POINT('Ctrl Pts',(18.6454900528359,16.5805893375142,36.7246940071671));
#47040=CARTESIAN_POINT('Ctrl Pts',(18.5979078468069,16.5850470605191,36.7732474100531));
#47041=CARTESIAN_POINT('Ctrl Pts',(18.5530871921838,16.589504783524,36.8240744992447));
#47042=CARTESIAN_POINT('Ctrl Pts',(18.5334450984166,16.5914583251219,36.8463488381677));
#47043=CARTESIAN_POINT('Ctrl Pts',(18.5143328255968,16.5934118667198,36.8690594374671));
#47044=CARTESIAN_POINT('Ctrl Pts',(18.4957696697059,16.5953654083177,36.8921781297214));
#47045=CARTESIAN_POINT('Ctrl Pts',(18.4535300638365,16.5998106022076,36.944783648674));
#47046=CARTESIAN_POINT('Ctrl Pts',(18.4139654211078,16.6042557960976,36.9997171835828));
#47047=CARTESIAN_POINT('Ctrl Pts',(18.3773430117714,16.6087009899876,37.0566750959299));
#47048=CARTESIAN_POINT('Ctrl Pts',(18.3407736908796,16.6131397400516,37.1135504411539));
#47049=CARTESIAN_POINT('Ctrl Pts',(18.3071384107541,16.6175784901157,37.1724439311144));
#47050=CARTESIAN_POINT('Ctrl Pts',(18.2766639897095,16.6220172401797,37.2330192894095));
#47051=CARTESIAN_POINT('Ctrl Pts',(18.2462230981501,16.6264511065085,37.2935279996597));
#47052=CARTESIAN_POINT('Ctrl Pts',(18.2189363873649,16.6308849728373,37.3557144662688));
#47053=CARTESIAN_POINT('Ctrl Pts',(18.1949861550876,16.6353188391661,37.4192154697891));
#47054=CARTESIAN_POINT('Ctrl Pts',(18.1710517467709,16.6397497760316,37.4826745180844));
#47055=CARTESIAN_POINT('Ctrl Pts',(18.1504496195063,16.6441807128971,37.5474459179093));
#47056=CARTESIAN_POINT('Ctrl Pts',(18.1333143395094,16.6486116497626,37.6131456051151));
#47057=CARTESIAN_POINT('Ctrl Pts',(18.1161856421353,16.6530408844565,37.6788200533834));
#47058=CARTESIAN_POINT('Ctrl Pts',(18.1025212694212,16.6574701191505,37.7454216006164));
#47059=CARTESIAN_POINT('Ctrl Pts',(18.0924056487478,16.6618993538444,37.8125520082335));
#47060=CARTESIAN_POINT('Ctrl Pts',(18.0822874619202,16.6663297121569,37.8796994456486));
#47061=CARTESIAN_POINT('Ctrl Pts',(18.0757198989312,16.6707600704694,37.947375520813));
#47062=CARTESIAN_POINT('Ctrl Pts',(18.0727358351024,16.6751904287819,38.0151743222739));
#47063=CARTESIAN_POINT('Ctrl Pts',(18.0714692472317,16.6770708973052,38.0439515685084));
#47064=CARTESIAN_POINT('Ctrl Pts',(18.0708476156394,16.6789513658286,38.0727508773751));
#47065=CARTESIAN_POINT('Ctrl Pts',(18.0708706155933,16.6808318343519,38.1015411420322));
#47066=CARTESIAN_POINT('',(18.0708705531879,16.5088527686983,38.0985390611445));
#47067=CARTESIAN_POINT('Ctrl Pts',(19.3941040086649,16.3533584392964,36.2684889832207));
#47068=CARTESIAN_POINT('Ctrl Pts',(19.3892758720374,16.3536772472466,36.2700862155613));
#47069=CARTESIAN_POINT('Ctrl Pts',(19.3844539050878,16.3539952867857,36.2717025877808));
#47070=CARTESIAN_POINT('Ctrl Pts',(19.3036135955524,16.3593220282272,36.2991571688369));
#47071=CARTESIAN_POINT('Ctrl Pts',(19.2292683506885,16.3641458421739,36.3296995152239));
#47072=CARTESIAN_POINT('Ctrl Pts',(19.0150878285822,16.3783853895655,36.4337480053713));
#47073=CARTESIAN_POINT('Ctrl Pts',(18.8821542772439,16.3877359897341,36.5198538405314));
#47074=CARTESIAN_POINT('Ctrl Pts',(18.7460531018636,16.3990146866174,36.633865659235));
#47075=CARTESIAN_POINT('Ctrl Pts',(18.7311073465873,16.4002783176956,36.6467814628489));
#47076=CARTESIAN_POINT('Ctrl Pts',(18.7105131007799,16.4020563815016,36.665138506828));
#47077=CARTESIAN_POINT('Ctrl Pts',(18.7046951223494,16.4025629024981,36.6703884307929));
#47078=CARTESIAN_POINT('Ctrl Pts',(18.6941083082209,16.4034924436621,36.6800592511146));
#47079=CARTESIAN_POINT('Ctrl Pts',(18.6893295089091,16.4039149969786,36.684469109109));
#47080=CARTESIAN_POINT('Ctrl Pts',(18.6802040288119,16.4047276634437,36.6929758960852));
#47081=CARTESIAN_POINT('Ctrl Pts',(18.6758538943057,16.4051176122385,36.6970690237963));
#47082=CARTESIAN_POINT('Ctrl Pts',(18.6653935398326,16.4060615138464,36.7070033712748));
#47083=CARTESIAN_POINT('Ctrl Pts',(18.6593026105019,16.4066163240264,36.7128646363392));
#47084=CARTESIAN_POINT('Ctrl Pts',(18.6386789552232,16.4085128418678,36.7329733877274));
#47085=CARTESIAN_POINT('Ctrl Pts',(18.6243336658668,16.4098627627312,36.747410324934));
#47086=CARTESIAN_POINT('Ctrl Pts',(18.5907218837777,16.4131012150043,36.7823247242782));
#47087=CARTESIAN_POINT('Ctrl Pts',(18.5716698310308,16.414998403525,36.8030012599432));
#47088=CARTESIAN_POINT('Ctrl Pts',(18.5025802854964,16.4221139922531,36.8813507630506));
#47089=CARTESIAN_POINT('Ctrl Pts',(18.4555328128699,16.4274425041934,36.9415568101993));
#47090=CARTESIAN_POINT('Ctrl Pts',(18.3424271484451,16.4415385188585,37.1054753230042));
#47091=CARTESIAN_POINT('Ctrl Pts',(18.2824882795144,16.4504065451616,37.2129933448711));
#47092=CARTESIAN_POINT('Ctrl Pts',(18.2157287901588,16.4620030874774,37.3652839764697));
#47093=CARTESIAN_POINT('Ctrl Pts',(18.1996283741878,16.4649905415365,37.4056700557658));
#47094=CARTESIAN_POINT('Ctrl Pts',(18.1823798919577,16.4684063222219,37.4535827448098));
#47095=CARTESIAN_POINT('Ctrl Pts',(18.1798955768499,16.4689042044245,37.4606112151402));
#47096=CARTESIAN_POINT('Ctrl Pts',(18.1759448517806,16.4697054742374,37.4719979979293));
#47097=CARTESIAN_POINT('Ctrl Pts',(18.1744532031112,16.4700102778456,37.4763473788992));
#47098=CARTESIAN_POINT('Ctrl Pts',(18.1718325418937,16.4705498109589,37.4840787277562));
#47099=CARTESIAN_POINT('Ctrl Pts',(18.1706973415091,16.4707848978146,37.4874585296661));
#47100=CARTESIAN_POINT('Ctrl Pts',(18.1682772127539,16.4712890498219,37.494730648508));
#47101=CARTESIAN_POINT('Ctrl Pts',(18.1669953197539,16.4715579371223,37.4986239112319));
#47102=CARTESIAN_POINT('Ctrl Pts',(18.1634868383316,16.4722991035999,37.5093950342462));
#47103=CARTESIAN_POINT('Ctrl Pts',(18.1612864589617,16.4727698827081,37.5162814577283));
#47104=CARTESIAN_POINT('Ctrl Pts',(18.1493104754225,16.4753665741367,37.5545018722405));
#47105=CARTESIAN_POINT('Ctrl Pts',(18.1402964179168,16.4774512964463,37.5860711902189));
#47106=CARTESIAN_POINT('Ctrl Pts',(18.0915649400639,16.489648591173,37.7748657998577));
#47107=CARTESIAN_POINT('Ctrl Pts',(18.0709933689859,16.4990290997554,37.9363641887504));
#47108=CARTESIAN_POINT('Ctrl Pts',(18.0708705531879,16.5088527686983,38.0985390611445));
#47109=CARTESIAN_POINT('Ctrl Pts',(18.0708705515757,16.508852897749,38.0985411915881));
#47110=CARTESIAN_POINT('Ctrl Pts',(18.0708048840684,16.5141131180069,38.1853799573665));
#47111=CARTESIAN_POINT('Ctrl Pts',(18.0766025970578,16.51947261588,38.2721161168967));
#47112=CARTESIAN_POINT('Ctrl Pts',(18.0896070740216,16.5256819604477,38.368418578429));
#47113=CARTESIAN_POINT('Ctrl Pts',(18.0910745387327,16.526345734488,38.3786633121205));
#47114=CARTESIAN_POINT('Ctrl Pts',(18.0936889979285,16.5274698009348,38.3959247591256));
#47115=CARTESIAN_POINT('Ctrl Pts',(18.0947924896503,16.527928736344,38.4029479162796));
#47116=CARTESIAN_POINT('Ctrl Pts',(18.0968949595824,16.5287756866617,38.4158630624971));
#47117=CARTESIAN_POINT('Ctrl Pts',(18.0978825470846,16.5291633405541,38.4217568384629));
#47118=CARTESIAN_POINT('Ctrl Pts',(18.0999771375618,16.5299651381418,38.4339102989339));
#47119=CARTESIAN_POINT('Ctrl Pts',(18.1010877264973,16.5303793902422,38.4401692835154));
#47120=CARTESIAN_POINT('Ctrl Pts',(18.1036471904395,16.5313104256268,38.4541905276434));
#47121=CARTESIAN_POINT('Ctrl Pts',(18.1051128237493,16.531827731907,38.4619495743343));
#47122=CARTESIAN_POINT('Ctrl Pts',(18.108959006785,16.5331464364166,38.4816473737806));
#47123=CARTESIAN_POINT('Ctrl Pts',(18.1114049782844,16.5339498899954,38.4935728501705));
#47124=CARTESIAN_POINT('Ctrl Pts',(18.1265076518352,16.5387135329302,38.5638219446732));
#47125=CARTESIAN_POINT('Ctrl Pts',(18.141751243414,16.5427551525522,38.6215502180609));
#47126=CARTESIAN_POINT('Ctrl Pts',(18.1722239688591,16.5497658266291,38.7184960156624));
#47127=CARTESIAN_POINT('Ctrl Pts',(18.18610533051,16.5526947584643,38.7580944548697));
#47128=CARTESIAN_POINT('Ctrl Pts',(18.2539947573515,16.5659249763226,38.9332433614372));
#47129=CARTESIAN_POINT('Ctrl Pts',(18.3219828480587,16.5765116980917,39.0628530756643));
#47130=CARTESIAN_POINT('Ctrl Pts',(18.4239828347039,16.589094361589,39.2130980059608));
#47131=CARTESIAN_POINT('Ctrl Pts',(18.4448545091076,16.5915347533597,39.2420771329861));
#47132=CARTESIAN_POINT('Ctrl Pts',(18.4710167783678,16.5944221893445,39.2763535997964));
#47133=CARTESIAN_POINT('Ctrl Pts',(18.4755474239509,16.5949163212764,39.2822190285856));
#47134=CARTESIAN_POINT('Ctrl Pts',(18.4826606387968,16.5956828051361,39.2913189951439));
#47135=CARTESIAN_POINT('Ctrl Pts',(18.4852199445685,16.5959567330136,39.294571500461));
#47136=CARTESIAN_POINT('Ctrl Pts',(18.4900001824561,16.59646490507,39.3006064224812));
#47137=CARTESIAN_POINT('Ctrl Pts',(18.4922183285059,16.596699331235,39.3033909016249));
#47138=CARTESIAN_POINT('Ctrl Pts',(18.4972823988856,16.5972314246571,39.3097119383247));
#47139=CARTESIAN_POINT('Ctrl Pts',(18.5001331011952,16.5975287470949,39.3132445958398));
#47140=CARTESIAN_POINT('Ctrl Pts',(18.5088848943855,16.5984349386969,39.3240120350952));
#47141=CARTESIAN_POINT('Ctrl Pts',(18.5148261652614,16.599041021927,39.3312142012477));
#47142=CARTESIAN_POINT('Ctrl Pts',(18.5730932063897,16.6049005083537,39.4008115314335));
#47143=CARTESIAN_POINT('Ctrl Pts',(18.6292751009563,16.609896526903,39.4598861798208));
#47144=CARTESIAN_POINT('Ctrl Pts',(18.7188166577528,16.6172623210434,39.5428306656738));
#47145=CARTESIAN_POINT('Ctrl Pts',(18.7494671964654,16.6196903702658,39.5694757293745));
#47146=CARTESIAN_POINT('Ctrl Pts',(18.8639114875287,16.6285115260933,39.662788351631));
#47147=CARTESIAN_POINT('Ctrl Pts',(18.9523683812009,16.6348854436372,39.7234131928609));
#47148=CARTESIAN_POINT('Ctrl Pts',(19.0756163316627,16.6436501439676,39.7935958702582));
#47149=CARTESIAN_POINT('Ctrl Pts',(19.1062972069616,16.6458219306448,39.8099845728939));
#47150=CARTESIAN_POINT('Ctrl Pts',(19.1520433312004,16.6490564619415,39.8328531238861));
#47151=CARTESIAN_POINT('Ctrl Pts',(19.1667758854631,16.6500975693242,39.8399850604511));
#47152=CARTESIAN_POINT('Ctrl Pts',(19.1935668655181,16.6519908898884,39.8525361274739));
#47153=CARTESIAN_POINT('Ctrl Pts',(19.205593736679,16.6528408561154,39.8580204644013));
#47154=CARTESIAN_POINT('Ctrl Pts',(19.2244219360543,16.6541719556873,39.8663735991807));
#47155=CARTESIAN_POINT('Ctrl Pts',(19.2311851318865,16.6546501866125,39.8693277596945));
#47156=CARTESIAN_POINT('Ctrl Pts',(19.2380142396075,16.6551332130436,39.8722641622308));
#47157=CARTESIAN_POINT('Ctrl Pts',(19.2380634440926,16.6551366933101,39.8722853169116));
#47158=CARTESIAN_POINT('Ctrl Pts',(19.2381632319464,16.6551437513867,39.8723282141785));
#47159=CARTESIAN_POINT('Ctrl Pts',(19.2382138152254,16.6551473291908,39.8723499565881));
#47160=CARTESIAN_POINT('Ctrl Pts',(19.2383164044322,16.6551545854396,39.8723940477069));
#47161=CARTESIAN_POINT('Ctrl Pts',(19.2383684103648,16.6551582638849,39.872416396272));
#47162=CARTESIAN_POINT('Ctrl Pts',(19.2384738903531,16.6551657246338,39.8724617188005));
#47163=CARTESIAN_POINT('Ctrl Pts',(19.2385273644588,16.6551695069413,39.8724846926304));
#47164=CARTESIAN_POINT('Ctrl Pts',(19.2386358275189,16.6551771787209,39.8725312852934));
#47165=CARTESIAN_POINT('Ctrl Pts',(19.2386908167319,16.6551810682118,39.872554904073));
#47166=CARTESIAN_POINT('Ctrl Pts',(19.2388023593083,16.6551889578468,39.8726028073129));
#47167=CARTESIAN_POINT('Ctrl Pts',(19.2388589126022,16.6551929579866,39.8726270915686));
#47168=CARTESIAN_POINT('Ctrl Pts',(19.2389736369529,16.655201072713,39.8726763482528));
#47169=CARTESIAN_POINT('Ctrl Pts',(19.2390318080577,16.6552051873039,39.8727013205154));
#47170=CARTESIAN_POINT('Ctrl Pts',(19.2391498044112,16.6552135335072,39.8727519682716));
#47171=CARTESIAN_POINT('Ctrl Pts',(19.2392096391798,16.6552177657938,39.872777647654));
#47172=CARTESIAN_POINT('Ctrl Pts',(19.2393310307579,16.6552263521934,39.8728297381919));
#47173=CARTESIAN_POINT('Ctrl Pts',(19.239392586876,16.6552307062581,39.8728561488419));
#47174=CARTESIAN_POINT('Ctrl Pts',(19.2395174778464,16.6552395402259,39.8729097256056));
#47175=CARTESIAN_POINT('Ctrl Pts',(19.2395808117616,16.6552440200634,39.8729368910955));
#47176=CARTESIAN_POINT('Ctrl Pts',(19.2397093165288,16.6552531096956,39.8729920018303));
#47177=CARTESIAN_POINT('Ctrl Pts',(19.2397744865614,16.6552577194331,39.873019946488));
#47178=CARTESIAN_POINT('Ctrl Pts',(19.2399067242232,16.6552670731584,39.8730766408542));
#47179=CARTESIAN_POINT('Ctrl Pts',(19.2399737909936,16.6552718170861,39.8731053899437));
#47180=CARTESIAN_POINT('Ctrl Pts',(19.240109883194,16.6552814435134,39.8731637185887));
#47181=CARTESIAN_POINT('Ctrl Pts',(19.2401789081103,16.6552863259773,39.8731932976581));
#47182=CARTESIAN_POINT('Ctrl Pts',(19.2403005649729,16.6552949313769,39.8732454225508));
#47183=CARTESIAN_POINT('Ctrl Pts',(19.2403531921221,16.6552986539672,39.8732679683169));
#47184=CARTESIAN_POINT('Ctrl Pts',(19.240465576667,16.6553066035246,39.8733161085656));
#47185=CARTESIAN_POINT('Ctrl Pts',(19.2405253344068,16.6553108305185,39.8733417023936));
#47186=CARTESIAN_POINT('Ctrl Pts',(19.2406529615775,16.6553198583138,39.8733963565965));
#47187=CARTESIAN_POINT('Ctrl Pts',(19.240720831173,16.6553246591301,39.8734254160053));
#47188=CARTESIAN_POINT('Ctrl Pts',(19.2408657821892,16.6553349123986,39.8734874691633));
#47189=CARTESIAN_POINT('Ctrl Pts',(19.2409428725203,16.6553403654852,39.8735204653889));
#47190=CARTESIAN_POINT('Ctrl Pts',(19.2411075500892,16.6553520142095,39.8735909380246));
#47191=CARTESIAN_POINT('Ctrl Pts',(19.2411951362286,16.6553582097745,39.8736284122364));
#47192=CARTESIAN_POINT('Ctrl Pts',(19.24138225509,16.6553714460176,39.8737084556729));
#47193=CARTESIAN_POINT('Ctrl Pts',(19.2414817871999,16.6553784866591,39.8737510224011));
#47194=CARTESIAN_POINT('Ctrl Pts',(19.241694451821,16.6553935300632,39.8738419511439));
#47195=CARTESIAN_POINT('Ctrl Pts',(19.241807584085,16.6554015328172,39.873890310162));
#47196=CARTESIAN_POINT('Ctrl Pts',(19.2420493345522,16.6554186338536,39.8739936203969));
#47197=CARTESIAN_POINT('Ctrl Pts',(19.2421779532428,16.6554277321819,39.8740485680812));
#47198=CARTESIAN_POINT('Ctrl Pts',(19.2482003280666,16.6558537499625,39.8766206354833));
#47199=CARTESIAN_POINT('Ctrl Pts',(19.2541065239219,16.6562716561318,39.8791083580916));
#47200=CARTESIAN_POINT('Ctrl Pts',(19.2676169838662,16.657227917164,39.8847199380488));
#47201=CARTESIAN_POINT('Ctrl Pts',(19.2752289989173,16.6577669049676,39.8878246927638));
#47202=CARTESIAN_POINT('Ctrl Pts',(19.2954290224283,16.6591979030618,39.8959135813905));
#47203=CARTESIAN_POINT('Ctrl Pts',(19.3080498709512,16.660092684301,39.9008139430155));
#47204=CARTESIAN_POINT('Ctrl Pts',(19.4073701333949,16.6671409334648,39.9381792961426));
#47205=CARTESIAN_POINT('Ctrl Pts',(19.4962399461726,16.6734965042636,39.9644930833565));
#47206=CARTESIAN_POINT('Ctrl Pts',(19.7428410696045,16.6912302729811,40.0185889517726));
#47207=CARTESIAN_POINT('Ctrl Pts',(19.902682996777,16.7028729836506,40.0332980420404));
#47208=CARTESIAN_POINT('Ctrl Pts',(20.0915535513515,16.7158892770902,40.0271754745477));
#47209=CARTESIAN_POINT('Ctrl Pts',(20.1205808260772,16.7178669469609,40.0255772776378));
#47210=CARTESIAN_POINT('Ctrl Pts',(20.1565032150207,16.7202773680959,40.0227838573251));
#47211=CARTESIAN_POINT('Ctrl Pts',(20.1634408436874,16.720741170757,40.0222065738543));
#47212=CARTESIAN_POINT('Ctrl Pts',(20.1743993201883,16.7214709050329,40.0212349553996));
#47213=CARTESIAN_POINT('Ctrl Pts',(20.1784222308775,16.7217381811788,40.0208655301726));
#47214=CARTESIAN_POINT('Ctrl Pts',(20.1860040828835,16.7222407148417,40.0201452618601));
#47215=CARTESIAN_POINT('Ctrl Pts',(20.1895631666149,16.7224761140691,40.0197971641791));
#47216=CARTESIAN_POINT('Ctrl Pts',(20.1977144711185,16.7230141229276,40.0189770335114));
#47217=CARTESIAN_POINT('Ctrl Pts',(20.2023059783428,16.7233163625422,40.0184984126789));
#47218=CARTESIAN_POINT('Ctrl Pts',(20.2145340923705,16.7241192276073,40.0171793611415));
#47219=CARTESIAN_POINT('Ctrl Pts',(20.2221675666111,16.7246182784717,40.0163097757611));
#47220=CARTESIAN_POINT('Ctrl Pts',(20.2778328036758,16.728243173976,40.0096314456327));
#47221=CARTESIAN_POINT('Ctrl Pts',(20.3256407191787,16.731278701166,40.0020626551314));
#47222=CARTESIAN_POINT('Ctrl Pts',(20.3869701489886,16.7351301078639,39.9899724884853));
#47223=CARTESIAN_POINT('Ctrl Pts',(20.400792424318,16.7359952863547,39.9870896509842));
#47224=CARTESIAN_POINT('Ctrl Pts',(20.4519075089283,16.7391881925269,39.9758418935097));
#47225=CARTESIAN_POINT('Ctrl Pts',(20.4889818762031,16.7414911980869,39.9665208590865));
#47226=CARTESIAN_POINT('Ctrl Pts',(20.6006214650739,16.7484490032239,39.9348980801802));
#47227=CARTESIAN_POINT('Ctrl Pts',(20.674134766144,16.7530648098837,39.9091819639176));
#47228=CARTESIAN_POINT('Ctrl Pts',(20.8082117080879,16.7618228256356,39.8529696283095));
#47229=CARTESIAN_POINT('Ctrl Pts',(20.8691089693926,16.7659408105452,39.8235884450813));
#47230=CARTESIAN_POINT('Ctrl Pts',(20.962730954298,16.7726075730337,39.7721935251985));
#47231=CARTESIAN_POINT('Ctrl Pts',(20.9965397206275,16.7750882517998,39.7522682358746));
#47232=CARTESIAN_POINT('Ctrl Pts',(21.0392677385793,16.7783309555674,39.7252977320796));
#47233=CARTESIAN_POINT('Ctrl Pts',(21.048766416575,16.7790588621646,39.7191847161454));
#47234=CARTESIAN_POINT('Ctrl Pts',(21.0640582328197,16.780242432276,39.7091524306178));
#47235=CARTESIAN_POINT('Ctrl Pts',(21.069884795773,16.7806961926983,39.7052843951885));
#47236=CARTESIAN_POINT('Ctrl Pts',(21.0810070467701,16.7815678019452,39.6978133016485));
#47237=CARTESIAN_POINT('Ctrl Pts',(21.0863060848072,16.7819854545864,39.6942153777166));
#47238=CARTESIAN_POINT('Ctrl Pts',(21.0983440428411,16.7829397600718,39.6859539970318));
#47239=CARTESIAN_POINT('Ctrl Pts',(21.1050713249971,16.7834770368238,39.6812738789735));
#47240=CARTESIAN_POINT('Ctrl Pts',(21.1227614361319,16.7849005219975,39.6687989847128));
#47241=CARTESIAN_POINT('Ctrl Pts',(21.1336727518421,16.7857894550613,39.6609322769185));
#47242=CARTESIAN_POINT('Ctrl Pts',(21.2165287255565,16.7926250389024,39.5998687658727));
#47243=CARTESIAN_POINT('Ctrl Pts',(21.2847656267366,16.7987599608654,39.5418465712944));
#47244=CARTESIAN_POINT('Ctrl Pts',(21.4645927727506,16.816401581958,39.3660068648197));
#47245=CARTESIAN_POINT('Ctrl Pts',(21.5657164710697,16.828205867248,39.2385666477072));
#47246=CARTESIAN_POINT('Ctrl Pts',(21.6652937100119,16.8414500383529,39.0742907730592));
#47247=CARTESIAN_POINT('Ctrl Pts',(21.6802697807159,16.8434962242681,39.0482295937541));
#47248=CARTESIAN_POINT('Ctrl Pts',(21.6979935662528,16.8459779650842,39.0156472584597));
#47249=CARTESIAN_POINT('Ctrl Pts',(21.7013216099445,16.8464467500478,39.0094486441043));
#47250=CARTESIAN_POINT('Ctrl Pts',(21.7065148357539,16.8471825295303,38.9996477779586));
#47251=CARTESIAN_POINT('Ctrl Pts',(21.7084026537535,16.8474509055507,38.9960576892344));
#47252=CARTESIAN_POINT('Ctrl Pts',(21.7119320062898,16.8479543272985,38.9892941737394));
#47253=CARTESIAN_POINT('Ctrl Pts',(21.7135760290826,16.8481895215035,38.9861221780354));
#47254=CARTESIAN_POINT('Ctrl Pts',(21.7173116908061,16.848725562675,38.9788652763391));
#47255=CARTESIAN_POINT('Ctrl Pts',(21.719397570841,16.8490260493152,38.9747774641543));
#47256=CARTESIAN_POINT('Ctrl Pts',(21.7248945865409,16.8498211862155,38.9639090422948));
#47257=CARTESIAN_POINT('Ctrl Pts',(21.728280367606,16.8503143095044,38.9571155952236));
#47258=CARTESIAN_POINT('Ctrl Pts',(21.7519959245775,16.8537938231324,38.9088192654342));
#47259=CARTESIAN_POINT('Ctrl Pts',(21.7708705153623,16.8566978739915,38.8666138102017));
#47260=CARTESIAN_POINT('Ctrl Pts',(21.8391703937921,16.8679347553882,38.697865264324));
#47261=CARTESIAN_POINT('Ctrl Pts',(21.8766928425007,16.8758695684353,38.5669261176721));
#47262=CARTESIAN_POINT('Ctrl Pts',(21.9114395305059,16.8880053667299,38.3687293978406));
#47263=CARTESIAN_POINT('Ctrl Pts',(21.9194472444387,16.891995210404,38.3038081702987));
#47264=CARTESIAN_POINT('Ctrl Pts',(21.926900042496,16.8984745513019,38.2003501407733));
#47265=CARTESIAN_POINT('Ctrl Pts',(21.9285142459604,16.9009008495183,38.1620194394894));
#47266=CARTESIAN_POINT('Ctrl Pts',(21.9291223062796,16.9040819392762,38.1124615190334));
#47267=CARTESIAN_POINT('Ctrl Pts',(21.9291621446617,16.9048042228001,38.1012542044362));
#47268=CARTESIAN_POINT('Ctrl Pts',(21.9290683459695,16.9059808887089,38.0830733388994));
#47269=CARTESIAN_POINT('Ctrl Pts',(21.9289945478482,16.9064334093115,38.076099633173));
#47270=CARTESIAN_POINT('Ctrl Pts',(21.9287803398671,16.9073041668063,38.0627165418849));
#47271=CARTESIAN_POINT('Ctrl Pts',(21.9286457913376,16.907722215872,38.0563071447044));
#47272=CARTESIAN_POINT('Ctrl Pts',(21.9282654232338,16.908679566519,38.0416661958792));
#47273=CARTESIAN_POINT('Ctrl Pts',(21.9279988380418,16.9092195060696,38.0334353539084));
#47274=CARTESIAN_POINT('Ctrl Pts',(21.9271527729192,16.9106546886913,38.0116293930573));
#47275=CARTESIAN_POINT('Ctrl Pts',(21.9264825667578,16.9115527286651,37.998058456264));
#47276=CARTESIAN_POINT('Ctrl Pts',(21.9199643883761,16.9187840503034,37.8893881361967));
#47277=CARTESIAN_POINT('Ctrl Pts',(21.9072226524958,16.9253319313523,37.7948486711656));
#47278=CARTESIAN_POINT('Ctrl Pts',(21.8673310773225,16.9389177790299,37.60582563805));
#47279=CARTESIAN_POINT('Ctrl Pts',(21.8398413969882,16.9459449686918,37.5116840336201));
#47280=CARTESIAN_POINT('Ctrl Pts',(21.7845941813676,16.95708606465,37.3649995230995));
#47281=CARTESIAN_POINT('Ctrl Pts',(21.7613546738252,16.9612346648168,37.3109291466405));
#47282=CARTESIAN_POINT('Ctrl Pts',(21.722908729966,16.9673030829408,37.2316774103787));
#47283=CARTESIAN_POINT('Ctrl Pts',(21.7095403446508,16.9692941492747,37.2056451202246));
#47284=CARTESIAN_POINT('Ctrl Pts',(21.6922568738773,16.9717185355463,37.1737938157794));
#47285=CARTESIAN_POINT('Ctrl Pts',(21.6888964114489,16.9721833274401,37.1676802383608));
#47286=CARTESIAN_POINT('Ctrl Pts',(21.6835360864481,16.9729142622165,37.1580524703537));
#47287=CARTESIAN_POINT('Ctrl Pts',(21.6815582541132,16.9731817569379,37.1545261813513));
#47288=CARTESIAN_POINT('Ctrl Pts',(21.6778104741126,16.9736844655346,37.1478932026651));
#47289=CARTESIAN_POINT('Ctrl Pts',(21.6760429967702,16.9739198224689,37.1447852525284));
#47290=CARTESIAN_POINT('Ctrl Pts',(21.6719763595535,16.9744574334195,37.1376804741705));
#47291=CARTESIAN_POINT('Ctrl Pts',(21.6696715048969,16.974759319374,37.1336869640118));
#47292=CARTESIAN_POINT('Ctrl Pts',(21.6634975756277,16.9755606233294,37.1230777365469));
#47293=CARTESIAN_POINT('Ctrl Pts',(21.6596033100083,16.9760584764191,37.1164766646993));
#47294=CARTESIAN_POINT('Ctrl Pts',(21.631070971093,16.9796530335569,37.068764236932));
#47295=CARTESIAN_POINT('Ctrl Pts',(21.604945388601,16.9826611177903,37.0285566342898));
#47296=CARTESIAN_POINT('Ctrl Pts',(21.5694738780134,16.9864586609536,36.9781794713609));
#47297=CARTESIAN_POINT('Ctrl Pts',(21.5614823107467,16.9872970414794,36.9670822805398));
#47298=CARTESIAN_POINT('Ctrl Pts',(21.4832965562056,16.9953455826715,36.8609116690367));
#47299=CARTESIAN_POINT('Ctrl Pts',(21.4046218278169,17.0022856152925,36.7723899072505));
#47300=CARTESIAN_POINT('Ctrl Pts',(21.2522960428598,17.0148599307573,36.6298026482158));
#47301=CARTESIAN_POINT('Ctrl Pts',(21.1819961387515,17.0203998380739,36.5727122814233));
#47302=CARTESIAN_POINT('Ctrl Pts',(21.0910933403258,17.02744775451,36.5089367640741));
#47303=CARTESIAN_POINT('Ctrl Pts',(21.0740421841855,17.0287647619614,36.4973770772044));
#47304=CARTESIAN_POINT('Ctrl Pts',(21.0494021113822,17.0306624653907,36.4812424004517));
#47305=CARTESIAN_POINT('Ctrl Pts',(21.0419613227749,17.0312348306714,36.4764429313934));
#47306=CARTESIAN_POINT('Ctrl Pts',(21.0290124117632,17.032229815672,36.4682162843196));
#47307=CARTESIAN_POINT('Ctrl Pts',(21.0235195109459,17.0326515529918,36.46476532347));
#47308=CARTESIAN_POINT('Ctrl Pts',(21.0129275177004,17.033464204081,36.4581850917118));
#47309=CARTESIAN_POINT('Ctrl Pts',(21.0078310612019,17.0338549611085,36.4550517029655));
#47310=CARTESIAN_POINT('Ctrl Pts',(20.9957771612093,17.0347785962841,36.447717804969));
#47311=CARTESIAN_POINT('Ctrl Pts',(20.9888076290942,17.0353121990037,36.4435374812456));
#47312=CARTESIAN_POINT('Ctrl Pts',(20.9643595421604,17.0371826099326,36.4290827995079));
#47313=CARTESIAN_POINT('Ctrl Pts',(20.9467461110923,17.0385276869294,36.4190403438669));
#47314=CARTESIAN_POINT('Ctrl Pts',(20.7800809126728,17.0512370168745,36.3274650817796));
#47315=CARTESIAN_POINT('Ctrl Pts',(20.621055989094,17.0633270664663,36.2656959297271));
#47316=CARTESIAN_POINT('Ctrl Pts',(20.3880287364013,17.0804222288587,36.2090011340592));
#47317=CARTESIAN_POINT('Ctrl Pts',(20.3191543659163,17.0853884480983,36.1961657438722));
#47318=CARTESIAN_POINT('Ctrl Pts',(20.2173956455247,17.0924801451444,36.1828810552826));
#47319=CARTESIAN_POINT('Ctrl Pts',(20.1849565924284,17.0947044193416,36.1794799442602));
#47320=CARTESIAN_POINT('Ctrl Pts',(20.1452522744402,17.0973703724086,36.1763325679926));
#47321=CARTESIAN_POINT('Ctrl Pts',(20.1380566183715,17.0978512644894,36.1758027683279));
#47322=CARTESIAN_POINT('Ctrl Pts',(20.126771776997,17.0986017211274,36.1750355203207));
#47323=CARTESIAN_POINT('Ctrl Pts',(20.1226846117667,17.0988727587352,36.1747707102059));
#47324=CARTESIAN_POINT('Ctrl Pts',(20.1150374748267,17.0993784055375,36.1742996983896));
#47325=CARTESIAN_POINT('Ctrl Pts',(20.1114778130096,17.0996131794006,36.1740903526583));
#47326=CARTESIAN_POINT('Ctrl Pts',(20.1033218899369,17.100149743641,36.1736333864251));
#47327=CARTESIAN_POINT('Ctrl Pts',(20.0987253138087,17.1004511660056,36.1733923449928));
#47328=CARTESIAN_POINT('Ctrl Pts',(20.0866662398352,17.1012394816692,36.172803246054));
#47329=CARTESIAN_POINT('Ctrl Pts',(20.0792024183489,17.1017249273355,36.1724820761246));
#47330=CARTESIAN_POINT('Ctrl Pts',(20.0279739035153,17.1050410096144,36.170575770234));
#47331=CARTESIAN_POINT('Ctrl Pts',(19.9841642853814,17.1077977712606,36.1704377925896));
#47332=CARTESIAN_POINT('Ctrl Pts',(19.9369685161855,17.1107185364186,36.1718969770219));
#47333=CARTESIAN_POINT('Ctrl Pts',(19.9335530689153,17.1109296275034,36.1720116595888));
#47334=CARTESIAN_POINT('Ctrl Pts',(19.8085918932259,17.1186432322514,36.1765400102261));
#47335=CARTESIAN_POINT('Ctrl Pts',(19.6877269909218,17.1257872421719,36.1924295107725));
#47336=CARTESIAN_POINT('Ctrl Pts',(19.5100385753546,17.1367334237182,36.2331420115103));
#47337=CARTESIAN_POINT('Ctrl Pts',(19.4516240808264,17.1404040562064,36.2494603274301));
#47338=CARTESIAN_POINT('Ctrl Pts',(19.3941038273433,17.1441450759092,36.2684890432051));
#47339=CARTESIAN_POINT('Origin',(20.,-1.3495818343519,38.1));
#47340=CARTESIAN_POINT('',(19.3941040099181,18.1086029180356,36.2684889828061));
#47341=CARTESIAN_POINT('',(19.3941039849792,17.9383397493623,36.2684889910563));
#47342=CARTESIAN_POINT('',(19.3941040087494,-1.3495818343519,36.2684889831927));
#47343=CARTESIAN_POINT('Ctrl Pts',(19.3941040099181,18.1086029180356,36.2684889828061));
#47344=CARTESIAN_POINT('Ctrl Pts',(19.4118925383936,18.1073231984833,36.2626042253727));
#47345=CARTESIAN_POINT('Ctrl Pts',(19.4297674431853,18.1060547358816,36.2569784117878));
#47346=CARTESIAN_POINT('Ctrl Pts',(19.4548261523261,18.1043034292345,36.2494911535087));
#47347=CARTESIAN_POINT('Ctrl Pts',(19.4619415653936,18.1038091547017,36.2474097483609));
#47348=CARTESIAN_POINT('Ctrl Pts',(19.4730482051212,18.1030424978933,36.2442302149794));
#47349=CARTESIAN_POINT('Ctrl Pts',(19.4770311717749,18.1027685385463,36.2431038546473));
#47350=CARTESIAN_POINT('Ctrl Pts',(19.4844465176776,18.1022603376764,36.2410325884398));
#47351=CARTESIAN_POINT('Ctrl Pts',(19.4878778550252,18.1020259139842,36.2400843730626));
#47352=CARTESIAN_POINT('Ctrl Pts',(19.4956899539437,18.1014938639647,36.2379488368605));
#47353=CARTESIAN_POINT('Ctrl Pts',(19.5000722862947,18.1011965822233,36.2367674759141));
#47354=CARTESIAN_POINT('Ctrl Pts',(19.5134785406461,18.1002906405667,36.2332042078609));
#47355=CARTESIAN_POINT('Ctrl Pts',(19.5225157773626,18.099684764339,36.2308722661144));
#47356=CARTESIAN_POINT('Ctrl Pts',(19.6102157059773,18.0938486371635,36.2089200241802));
#47357=CARTESIAN_POINT('Ctrl Pts',(19.6900353381661,18.0888734817033,36.1942086492662));
#47358=CARTESIAN_POINT('Ctrl Pts',(19.9332760717362,18.074087065427,36.1650713069205));
#47359=CARTESIAN_POINT('Ctrl Pts',(20.0978087127406,18.0645279247874,36.166393570264));
#47360=CARTESIAN_POINT('Ctrl Pts',(20.2991118818064,18.0518466700567,36.1937950672755));
#47361=CARTESIAN_POINT('Ctrl Pts',(20.3378558179994,18.049363557701,36.200279423009));
#47362=CARTESIAN_POINT('Ctrl Pts',(20.3874553776625,18.0461180973221,36.21014588673));
#47363=CARTESIAN_POINT('Ctrl Pts',(20.3985181124923,18.0453899407151,36.2124477373304));
#47364=CARTESIAN_POINT('Ctrl Pts',(20.4163948641007,18.0442060627775,36.2163315585643));
#47365=CARTESIAN_POINT('Ctrl Pts',(20.4232217271286,18.0437522463795,36.2178536593391));
#47366=CARTESIAN_POINT('Ctrl Pts',(20.4362837856676,18.0428805965614,36.2208406034761));
#47367=CARTESIAN_POINT('Ctrl Pts',(20.4425202703756,18.0424629596926,36.2222994413824));
#47368=CARTESIAN_POINT('Ctrl Pts',(20.4567179752734,18.0415087832948,36.2256952275226));
#47369=CARTESIAN_POINT('Ctrl Pts',(20.464674309474,18.0409716204638,36.2276518828765));
#47370=CARTESIAN_POINT('Ctrl Pts',(20.4856536365578,18.0395486376356,36.232953164777));
#47371=CARTESIAN_POINT('Ctrl Pts',(20.4986543557239,18.038660096089,36.2363833125745));
#47372=CARTESIAN_POINT('Ctrl Pts',(20.5978633149255,18.03182676355,36.2636713159341));
#47373=CARTESIAN_POINT('Ctrl Pts',(20.6823414646879,18.0256938153348,36.2933596084965));
#47374=CARTESIAN_POINT('Ctrl Pts',(20.9131470930805,18.0080612837136,36.3929745257305));
#47375=CARTESIAN_POINT('Ctrl Pts',(21.0531639647008,17.9962644847465,36.4756182898083));
#47376=CARTESIAN_POINT('Ctrl Pts',(21.205059700778,17.9830173562508,36.5932538459348));
#47377=CARTESIAN_POINT('Ctrl Pts',(21.2284788021932,17.9809628522973,36.6122860026398));
#47378=CARTESIAN_POINT('Ctrl Pts',(21.2568041645154,17.9784724696886,36.6364305725844));
#47379=CARTESIAN_POINT('Ctrl Pts',(21.2621400485983,17.9780030918089,36.6410295827833));
#47380=CARTESIAN_POINT('Ctrl Pts',(21.2705100424778,17.9772665926524,36.6483239835229));
#47381=CARTESIAN_POINT('Ctrl Pts',(21.273560977239,17.9769980854496,36.6509998402827));
#47382=CARTESIAN_POINT('Ctrl Pts',(21.2792817985447,17.9764945556946,36.6560493779564));
#47383=CARTESIAN_POINT('Ctrl Pts',(21.2819535043678,17.9762593838645,36.6584208201161));
#47384=CARTESIAN_POINT('Ctrl Pts',(21.288040014378,17.9757235688279,36.663853590367));
#47385=CARTESIAN_POINT('Ctrl Pts',(21.2914504979222,17.9754232848245,36.6669196808877));
#47386=CARTESIAN_POINT('Ctrl Pts',(21.3004685120442,17.9746290411675,36.6750853867043));
#47387=CARTESIAN_POINT('Ctrl Pts',(21.3060570458569,17.9741366030221,36.6802059996072));
#47388=CARTESIAN_POINT('Ctrl Pts',(21.3453284545495,17.97067323034,36.7166173590701));
#47389=CARTESIAN_POINT('Ctrl Pts',(21.3779165668895,17.9677837737747,36.7490733189066));
#47390=CARTESIAN_POINT('Ctrl Pts',(21.4295724695379,17.9631135437123,36.8043360701767));
#47391=CARTESIAN_POINT('Ctrl Pts',(21.4493266779553,17.9613039127331,36.8264715265518));
#47392=CARTESIAN_POINT('Ctrl Pts',(21.5766436967247,17.9494143031022,36.9759369436844));
#47393=CARTESIAN_POINT('Ctrl Pts',(21.6678210560629,17.9397218858216,37.1162841720173));
#47394=CARTESIAN_POINT('Ctrl Pts',(21.7582953243033,17.9266846652254,37.3051617910635));
#47395=CARTESIAN_POINT('Ctrl Pts',(21.7754761284208,17.9239868220147,37.3443186442393));
#47396=CARTESIAN_POINT('Ctrl Pts',(21.7956576152852,17.9204988438613,37.3948109883221));
#47397=CARTESIAN_POINT('Ctrl Pts',(21.7998762110594,17.9197496696103,37.4056489153392));
#47398=CARTESIAN_POINT('Ctrl Pts',(21.8065004587066,17.9185399729726,37.423133248058));
#47399=CARTESIAN_POINT('Ctrl Pts',(21.8089680712289,17.9180815131348,37.429755997963));
#47400=CARTESIAN_POINT('Ctrl Pts',(21.8135960750535,17.9172064738151,37.4423887021355));
#47401=CARTESIAN_POINT('Ctrl Pts',(21.8157631278886,17.9167901213956,37.4483961293169));
#47402=CARTESIAN_POINT('Ctrl Pts',(21.820640459409,17.9158376847898,37.4621301700074));
#47403=CARTESIAN_POINT('Ctrl Pts',(21.8233314396808,17.915300973691,37.4698634592071));
#47404=CARTESIAN_POINT('Ctrl Pts',(21.8302097171325,17.913899248518,37.4900431230368));
#47405=CARTESIAN_POINT('Ctrl Pts',(21.8343192467537,17.9130317109787,37.5025153667216));
#47406=CARTESIAN_POINT('Ctrl Pts',(21.8621572879076,17.9069373598143,37.5899977240461));
#47407=CARTESIAN_POINT('Ctrl Pts',(21.8814020138474,17.9015664073956,37.6663461714946));
#47408=CARTESIAN_POINT('Ctrl Pts',(21.926408496641,17.8845678755002,37.9057979591838));
#47409=CARTESIAN_POINT('Ctrl Pts',(21.9359561248284,17.8725522417409,38.071169461438));
#47410=CARTESIAN_POINT('Ctrl Pts',(21.9217008124161,17.8584912562595,38.2732786460712));
#47411=CARTESIAN_POINT('Ctrl Pts',(21.917953697406,17.8559150443154,38.3107452920163));
#47412=CARTESIAN_POINT('Ctrl Pts',(21.9121446312209,17.8528894701586,38.3555427111758));
#47413=CARTESIAN_POINT('Ctrl Pts',(21.9111333961986,17.8523877319157,38.3629986966895));
#47414=CARTESIAN_POINT('Ctrl Pts',(21.9094948995196,17.8516120518263,38.3745707880648));
#47415=CARTESIAN_POINT('Ctrl Pts',(21.9088979061786,17.8513364735977,38.3786910001237));
#47416=CARTESIAN_POINT('Ctrl Pts',(21.9077660589251,17.850826813554,38.3863282669433));
#47417=CARTESIAN_POINT('Ctrl Pts',(21.9072348194431,17.8505925399766,38.3898457449876));
#47418=CARTESIAN_POINT('Ctrl Pts',(21.9060086786201,17.8500627913441,38.3978149998396));
#47419=CARTESIAN_POINT('Ctrl Pts',(21.905307910748,17.8497676487444,38.4022658157372));
#47420=CARTESIAN_POINT('Ctrl Pts',(21.9031342364536,17.8488746609396,38.4157635990298));
#47421=CARTESIAN_POINT('Ctrl Pts',(21.9016124137082,17.8482794846267,38.4248027224624));
#47422=CARTESIAN_POINT('Ctrl Pts',(21.88108920582,17.8406209264802,38.5416122681688));
#47423=CARTESIAN_POINT('Ctrl Pts',(21.8530123106157,17.8340264779236,38.647604613245));
#47424=CARTESIAN_POINT('Ctrl Pts',(21.7879615680553,17.8224864414853,38.8291720982697));
#47425=CARTESIAN_POINT('Ctrl Pts',(21.7547697802853,17.817534779018,38.9057798127984));
#47426=CARTESIAN_POINT('Ctrl Pts',(21.6809243565284,17.8077234430567,39.0498397900059));
#47427=CARTESIAN_POINT('Ctrl Pts',(21.6408979395498,17.8028849308972,39.1174252450024));
#47428=CARTESIAN_POINT('Ctrl Pts',(21.5861427964035,17.7966812750198,39.1982072440891));
#47429=CARTESIAN_POINT('Ctrl Pts',(21.5751808696584,17.7954575763647,39.2138731111288));
#47430=CARTESIAN_POINT('Ctrl Pts',(21.5589575305216,17.7936711498592,39.2363396572517));
#47431=CARTESIAN_POINT('Ctrl Pts',(21.5538804253971,17.793115448697,39.2432725039365));
#47432=CARTESIAN_POINT('Ctrl Pts',(21.5449155792835,17.7921399347723,39.2553440732947));
#47433=CARTESIAN_POINT('Ctrl Pts',(21.541048067607,17.7917209080448,39.2604977063565));
#47434=CARTESIAN_POINT('Ctrl Pts',(21.5334996652656,17.7909065257766,39.2704520187741));
#47435=CARTESIAN_POINT('Ctrl Pts',(21.5298218651462,17.790511294044,39.2752549558051));
#47436=CARTESIAN_POINT('Ctrl Pts',(21.5209917332053,17.7895660220169,39.2866747801002));
#47437=CARTESIAN_POINT('Ctrl Pts',(21.5158187596667,17.7890151735486,39.2932754796357));
#47438=CARTESIAN_POINT('Ctrl Pts',(21.4970653567611,17.7870284569142,39.31688604061));
#47439=CARTESIAN_POINT('Ctrl Pts',(21.4832407404018,17.7855829242982,39.3336989740883));
#47440=CARTESIAN_POINT('Ctrl Pts',(21.370372898292,17.7739258380785,39.4663244048278));
#47441=CARTESIAN_POINT('Ctrl Pts',(21.2582264811461,17.7631474187531,39.5702423589567));
#47442=CARTESIAN_POINT('Ctrl Pts',(21.0689348433601,17.7464425533277,39.7079825149376));
#47443=CARTESIAN_POINT('Ctrl Pts',(20.9998173153705,17.7406112843658,39.7518463842731));
#47444=CARTESIAN_POINT('Ctrl Pts',(20.8967893918773,17.7324679970661,39.8083877320062));
#47445=CARTESIAN_POINT('Ctrl Pts',(20.8649838068752,17.730025078358,39.8247096192004));
#47446=CARTESIAN_POINT('Ctrl Pts',(20.8260535130041,17.7271350641949,39.8433396426975));
#47447=CARTESIAN_POINT('Ctrl Pts',(20.8193478083841,17.7266407850355,39.8465012709508));
#47448=CARTESIAN_POINT('Ctrl Pts',(20.8088699341412,17.7258741226311,39.8513677851575));
#47449=CARTESIAN_POINT('Ctrl Pts',(20.8051103107286,17.7256001622782,39.8530992777373));
#47450=CARTESIAN_POINT('Ctrl Pts',(20.7981067897734,17.7250919605112,39.8562974641224));
#47451=CARTESIAN_POINT('Ctrl Pts',(20.7948644356946,17.7248575369217,39.8577672654692));
#47452=CARTESIAN_POINT('Ctrl Pts',(20.7874789972542,17.7243254883749,39.8610905670619));
#47453=CARTESIAN_POINT('Ctrl Pts',(20.7833334353033,17.7240282079958,39.8629384239635));
#47454=CARTESIAN_POINT('Ctrl Pts',(20.7706436801045,17.7231222746209,39.8685412000521));
#47455=CARTESIAN_POINT('Ctrl Pts',(20.762078571648,17.7225164052385,39.8722488304663));
#47456=CARTESIAN_POINT('Ctrl Pts',(20.6788649250874,17.7166810366408,39.9075551979002));
#47457=CARTESIAN_POINT('Ctrl Pts',(20.6023113760885,17.7117065587598,39.9344857258165));
#47458=CARTESIAN_POINT('Ctrl Pts',(20.3665569866555,17.6969203627755,40.0010626799827));
#47459=CARTESIAN_POINT('Ctrl Pts',(20.2038103148295,17.6873608829233,40.0253217744567));
#47460=CARTESIAN_POINT('Ctrl Pts',(20.0006833195611,17.6746789836716,40.0295297437341));
#47461=CARTESIAN_POINT('Ctrl Pts',(19.961398130099,17.6721956070027,40.0291436067419));
#47462=CARTESIAN_POINT('Ctrl Pts',(19.9108632608321,17.6689498473738,40.0271027192245));
#47463=CARTESIAN_POINT('Ctrl Pts',(19.8995768095378,17.6682216637664,40.0265475396934));
#47464=CARTESIAN_POINT('Ctrl Pts',(19.8813132082476,17.6670377526727,40.0254882307833));
#47465=CARTESIAN_POINT('Ctrl Pts',(19.8743326691789,17.666583930318,40.0250452465468));
#47466=CARTESIAN_POINT('Ctrl Pts',(19.8609650901427,17.6657122763461,40.0241239234207));
#47467=CARTESIAN_POINT('Ctrl Pts',(19.8545777095706,17.6652946413202,40.0236517186411));
#47468=CARTESIAN_POINT('Ctrl Pts',(19.8400250367448,17.6643404792608,40.0225029771382));
#47469=CARTESIAN_POINT('Ctrl Pts',(19.8318615092212,17.6638033289915,40.0218062156222));
#47470=CARTESIAN_POINT('Ctrl Pts',(19.8103141274487,17.6623804012654,40.0198287924061));
#47471=CARTESIAN_POINT('Ctrl Pts',(19.7969389885318,17.6614919025972,40.0184601983193));
#47472=CARTESIAN_POINT('Ctrl Pts',(19.6947210385149,17.6546603080292,40.0069199731989));
#47473=CARTESIAN_POINT('Ctrl Pts',(19.6066809751332,17.6485291662192,39.990723400181));
#47474=CARTESIAN_POINT('Ctrl Pts',(19.3632897158655,17.6309034189659,39.9282099086753));
#47475=CARTESIAN_POINT('Ctrl Pts',(19.212191915359,17.6191118337248,39.8683626782545));
#47476=CARTESIAN_POINT('Ctrl Pts',(19.043837546314,17.6058626322531,39.7757718409627));
#47477=CARTESIAN_POINT('Ctrl Pts',(19.0176724466505,17.6038023215361,39.7605693995809));
#47478=CARTESIAN_POINT('Ctrl Pts',(18.9858631155754,17.6013059089861,39.741072406246));
#47479=CARTESIAN_POINT('Ctrl Pts',(18.9798722728871,17.600836119417,39.7373550888729));
#47480=CARTESIAN_POINT('Ctrl Pts',(18.9704642763188,17.6000991209037,39.7314457482434));
#47481=CARTESIAN_POINT('Ctrl Pts',(18.967033505964,17.5998305229565,39.729275685313));
#47482=CARTESIAN_POINT('Ctrl Pts',(18.9605967001205,17.599326918891,39.7251757127561));
#47483=CARTESIAN_POINT('Ctrl Pts',(18.9575892099003,17.5990917629391,39.7232483057331));
#47484=CARTESIAN_POINT('Ctrl Pts',(18.9507345848953,17.5985561056465,39.7188284829377));
#47485=CARTESIAN_POINT('Ctrl Pts',(18.9468909707872,17.598255962729,39.7163307032178));
#47486=CARTESIAN_POINT('Ctrl Pts',(18.9367217851823,17.5974623397868,39.7096705661399));
#47487=CARTESIAN_POINT('Ctrl Pts',(18.9304116779904,17.5969703774822,39.7054845746948));
#47488=CARTESIAN_POINT('Ctrl Pts',(18.8862134354731,17.5935267295442,39.6757881572355));
#47489=CARTESIAN_POINT('Ctrl Pts',(18.8492137031909,17.59065544682,39.648974013418));
#47490=CARTESIAN_POINT('Ctrl Pts',(18.7897710514215,17.5859992803231,39.6025882491681));
#47491=CARTESIAN_POINT('Ctrl Pts',(18.7667690405704,17.5841861444455,39.5837678672533));
#47492=CARTESIAN_POINT('Ctrl Pts',(18.6570936630613,17.5754359098643,39.4897177034113));
#47493=CARTESIAN_POINT('Ctrl Pts',(18.5768163269402,17.5686887543726,39.4073875049407));
#47494=CARTESIAN_POINT('Ctrl Pts',(18.4664635073572,17.5581170463351,39.2719229011525));
#47495=CARTESIAN_POINT('Ctrl Pts',(18.4307857151483,17.5544444831011,39.2237006307591));
#47496=CARTESIAN_POINT('Ctrl Pts',(18.3840787503288,17.5491938562941,39.1539994466186));
#47497=CARTESIAN_POINT('Ctrl Pts',(18.3711167748953,17.5476829191788,39.1338547680373));
#47498=CARTESIAN_POINT('Ctrl Pts',(18.3490275472192,17.5450071361184,39.0980781207879));
#47499=CARTESIAN_POINT('Ctrl Pts',(18.3397388002028,17.5438481559237,39.0825490766422));
#47500=CARTESIAN_POINT('Ctrl Pts',(18.3264577867222,17.5421393259518,39.0596195344377));
#47501=CARTESIAN_POINT('Ctrl Pts',(18.3222930846104,17.5415956627208,39.0523196379774));
#47502=CARTESIAN_POINT('Ctrl Pts',(18.3150338679249,17.5406340120544,39.0394002568107));
#47503=CARTESIAN_POINT('Ctrl Pts',(18.3119194140304,17.5402167420926,39.0337920766176));
#47504=CARTESIAN_POINT('Ctrl Pts',(18.3058947595475,17.5394002842184,39.0228148709993));
#47505=CARTESIAN_POINT('Ctrl Pts',(18.302981965041,17.5390011944096,39.0174473496889));
#47506=CARTESIAN_POINT('Ctrl Pts',(18.2952042948898,17.5379236830919,39.0029513587995));
#47507=CARTESIAN_POINT('Ctrl Pts',(18.2903873266715,17.5372435879305,38.9937975456882));
#47508=CARTESIAN_POINT('Ctrl Pts',(18.2727277611512,17.5347017555788,38.9595735055242));
#47509=CARTESIAN_POINT('Ctrl Pts',(18.2603616546485,17.5328236112877,38.9342627189391));
#47510=CARTESIAN_POINT('Ctrl Pts',(18.2477996478815,17.5308054884993,38.9070562103519));
#47511=CARTESIAN_POINT('Ctrl Pts',(18.2470469457882,17.5306841213707,38.9054200086445));
#47512=CARTESIAN_POINT('Ctrl Pts',(18.1781034665633,17.5195266732942,38.7549982476611));
#47513=CARTESIAN_POINT('Ctrl Pts',(18.1291330819691,17.50783057734,38.5981633331092));
#47514=CARTESIAN_POINT('Ctrl Pts',(18.0848760386854,17.489793819444,38.3487689649297));
#47515=CARTESIAN_POINT('Ctrl Pts',(18.0753806866286,17.4834612818344,38.2594682013972));
#47516=CARTESIAN_POINT('Ctrl Pts',(18.0717263166812,17.4766534019954,38.1585662706702));
#47517=CARTESIAN_POINT('Ctrl Pts',(18.0714172442492,17.4758986732864,38.1473072396621));
#47518=CARTESIAN_POINT('Ctrl Pts',(18.0711152466552,17.4748231012477,38.1311475055862));
#47519=CARTESIAN_POINT('Ctrl Pts',(18.0710423641021,17.4744980594845,38.1262487906072));
#47520=CARTESIAN_POINT('Ctrl Pts',(18.0709482487533,17.4739356415033,38.117745209663));
#47521=CARTESIAN_POINT('Ctrl Pts',(18.0709184571446,17.4736977962621,38.1141404862414));
#47522=CARTESIAN_POINT('Ctrl Pts',(18.0708799478177,17.4732336793544,38.1070893228041));
#47523=CARTESIAN_POINT('Ctrl Pts',(18.0708703611119,17.4730073581601,38.1036429461361));
#47524=CARTESIAN_POINT('Ctrl Pts',(18.0708693982257,17.472388062245,38.0941912351593));
#47525=CARTESIAN_POINT('Ctrl Pts',(18.070896827741,17.4719961188606,38.0881858736622));
#47526=CARTESIAN_POINT('Ctrl Pts',(18.0711274071889,17.4703730295024,38.0632243279425));
#47527=CARTESIAN_POINT('Ctrl Pts',(18.0715819316287,17.4691550794148,38.0442707557716));
#47528=CARTESIAN_POINT('Ctrl Pts',(18.0735232595446,17.4659657751023,37.9941559548935));
#47529=CARTESIAN_POINT('Ctrl Pts',(18.0754866312828,17.4640159203536,37.9630178426873));
#47530=CARTESIAN_POINT('Ctrl Pts',(18.0903074492742,17.4535111332103,37.7935398740277));
#47531=CARTESIAN_POINT('Ctrl Pts',(18.1173257451411,17.4454043963285,37.6568444483357));
#47532=CARTESIAN_POINT('Ctrl Pts',(18.1869115785594,17.4313288350367,37.4343224430347));
#47533=CARTESIAN_POINT('Ctrl Pts',(18.2215703195123,17.4255376757858,37.3466072988216));
#47534=CARTESIAN_POINT('Ctrl Pts',(18.2683858522368,17.418657163266,37.2495654342183));
#47535=CARTESIAN_POINT('Ctrl Pts',(18.2744075236705,17.4177867994886,37.2374125563218));
#47536=CARTESIAN_POINT('Ctrl Pts',(18.2842873157464,17.4163813224155,37.2179907928233));
#47537=CARTESIAN_POINT('Ctrl Pts',(18.2880647449704,17.4158490098224,37.2106811957506));
#47538=CARTESIAN_POINT('Ctrl Pts',(18.2948678638846,17.4148990960941,37.1977206414477));
#47539=CARTESIAN_POINT('Ctrl Pts',(18.2978751928127,17.414482143134,37.1920601442882));
#47540=CARTESIAN_POINT('Ctrl Pts',(18.3042150619795,17.4136092146317,37.1802692306864));
#47541=CARTESIAN_POINT('Ctrl Pts',(18.3075527589765,17.413153061573,37.1741417072553));
#47542=CARTESIAN_POINT('Ctrl Pts',(18.3163455203352,17.4119601109682,37.1582059093984));
#47543=CARTESIAN_POINT('Ctrl Pts',(18.3218530018213,17.4112214602914,37.148427007793));
#47544=CARTESIAN_POINT('Ctrl Pts',(18.3466371663738,17.4079344063016,37.1053054699215));
#47545=CARTESIAN_POINT('Ctrl Pts',(18.3668233149437,17.4053535989622,37.0724984555972));
#47546=CARTESIAN_POINT('Ctrl Pts',(18.4241002075291,17.3982733530597,36.9853668299652));
#47547=CARTESIAN_POINT('Ctrl Pts',(18.4630066037813,17.3937118192467,36.932302676801));
#47548=CARTESIAN_POINT('Ctrl Pts',(18.5880297443326,17.3797818986968,36.7788836309515));
#47549=CARTESIAN_POINT('Ctrl Pts',(18.6818185119012,17.3702236525022,36.6852900730718));
#47550=CARTESIAN_POINT('Ctrl Pts',(18.7885694746814,17.3605993881295,36.5986649310363));
#47551=CARTESIAN_POINT('Ctrl Pts',(18.7927178673631,17.3602272253861,36.5953270255304));
#47552=CARTESIAN_POINT('Ctrl Pts',(18.8314099969384,17.3567734759212,36.56445735214));
#47553=CARTESIAN_POINT('Ctrl Pts',(18.866879228292,17.3537356999173,36.5380999255529));
#47554=CARTESIAN_POINT('Ctrl Pts',(18.9093860567517,17.3502695504009,36.508723824417));
#47555=CARTESIAN_POINT('Ctrl Pts',(18.9155717218329,17.3497693372931,36.504501972999));
#47556=CARTESIAN_POINT('Ctrl Pts',(18.9256032804263,17.3489650583872,36.4977405071107));
#47557=CARTESIAN_POINT('Ctrl Pts',(18.9294338896121,17.3486595597016,36.495178515234));
#47558=CARTESIAN_POINT('Ctrl Pts',(18.9362452312241,17.3481192605502,36.4906581880005));
#47559=CARTESIAN_POINT('Ctrl Pts',(18.9392222475974,17.3478840988925,36.4886943689302));
#47560=CARTESIAN_POINT('Ctrl Pts',(18.9456268841808,17.3473803045836,36.4844949287534));
#47561=CARTESIAN_POINT('Ctrl Pts',(18.9490561700199,17.3471118470737,36.4822619589121));
#47562=CARTESIAN_POINT('Ctrl Pts',(18.9585377044504,17.3463730809225,36.4761309574922));
#47563=CARTESIAN_POINT('Ctrl Pts',(18.9646047834258,17.3459042563914,36.4722558156308));
#47564=CARTESIAN_POINT('Ctrl Pts',(18.998070730984,17.3433387569583,36.4511433948529));
#47565=CARTESIAN_POINT('Ctrl Pts',(19.0258802789082,17.341282115695,36.4345626902992));
#47566=CARTESIAN_POINT('Ctrl Pts',(19.1623974783928,17.3314787247161,36.3577582494407));
#47567=CARTESIAN_POINT('Ctrl Pts',(19.2762675852966,17.3241649283083,36.3074713211389));
#47568=CARTESIAN_POINT('Ctrl Pts',(19.3941042778785,17.3167366370521,36.2684888941601));
#47569=CARTESIAN_POINT('Ctrl Pts',(19.3941038273433,17.1441450759092,36.2684890432051));
#47570=CARTESIAN_POINT('Ctrl Pts',(19.3466248561783,17.1472330276451,36.2841959254401));
#47571=CARTESIAN_POINT('Ctrl Pts',(19.2997551437927,17.1503686465276,36.3017494977559));
#47572=CARTESIAN_POINT('Ctrl Pts',(19.2399626035716,17.1545108494447,36.3268377160733));
#47573=CARTESIAN_POINT('Ctrl Pts',(19.2263901883899,17.1554607606846,36.3327170093857));
#47574=CARTESIAN_POINT('Ctrl Pts',(19.2058106178431,17.1569164892568,36.341914149156));
#47575=CARTESIAN_POINT('Ctrl Pts',(19.1987534281107,17.1574184785392,36.3451192172076));
#47576=CARTESIAN_POINT('Ctrl Pts',(19.186508805378,17.1582944063562,36.3507694492945));
#47577=CARTESIAN_POINT('Ctrl Pts',(19.1813125692244,17.1586676838802,36.3531953936529));
#47578=CARTESIAN_POINT('Ctrl Pts',(19.1696707294073,17.1595075407258,36.3586939253644));
#47579=CARTESIAN_POINT('Ctrl Pts',(19.163231240171,17.1599745517349,36.361779190253));
#47580=CARTESIAN_POINT('Ctrl Pts',(19.1460522088869,17.1612271021231,36.370127529649));
#47581=CARTESIAN_POINT('Ctrl Pts',(19.1353443726138,17.1620148494721,36.3754547762477));
#47582=CARTESIAN_POINT('Ctrl Pts',(19.0880756679491,17.165524107264,36.3995222880841));
#47583=CARTESIAN_POINT('Ctrl Pts',(19.0520717705113,17.1682824582813,36.4193268987948));
#47584=CARTESIAN_POINT('Ctrl Pts',(18.8819208397601,17.1817466190809,36.5201287164591));
#47585=CARTESIAN_POINT('Ctrl Pts',(18.757361200035,17.192988669626,36.6161106409262));
#47586=CARTESIAN_POINT('Ctrl Pts',(18.603357035822,17.2083624659885,36.7679029118649));
#47587=CARTESIAN_POINT('Ctrl Pts',(18.5628708565167,17.212567769212,36.8116851789057));
#47588=CARTESIAN_POINT('Ctrl Pts',(18.5054677623278,17.218708179541,36.8798416234997));
#47589=CARTESIAN_POINT('Ctrl Pts',(18.4869801654571,17.2207163440911,36.9028432481728));
#47590=CARTESIAN_POINT('Ctrl Pts',(18.4647705805944,17.2231585398011,36.9318124670456));
#47591=CARTESIAN_POINT('Ctrl Pts',(18.460544959657,17.223624583518,36.9373867088218));
#47592=CARTESIAN_POINT('Ctrl Pts',(18.4539223589926,17.2243570373054,36.9462223506294));
#47593=CARTESIAN_POINT('Ctrl Pts',(18.4515052155018,17.2246248084857,36.9494684535655));
#47594=CARTESIAN_POINT('Ctrl Pts',(18.4469724342115,17.2251277394576,36.9555959129854));
#47595=CARTESIAN_POINT('Ctrl Pts',(18.4448546143096,17.2253630440113,36.958475508769));
#47596=CARTESIAN_POINT('Ctrl Pts',(18.4400273386381,17.2259001566168,36.9650775140074));
#47597=CARTESIAN_POINT('Ctrl Pts',(18.4373231973705,17.2262015990583,36.9688037460218));
#47598=CARTESIAN_POINT('Ctrl Pts',(18.4301669489574,17.2270009466881,36.9787394920532));
#47599=CARTESIAN_POINT('Ctrl Pts',(18.4257382930485,17.2274972990487,36.9849659119414));
#47600=CARTESIAN_POINT('Ctrl Pts',(18.3941205226583,17.2310543931837,37.0299824490496));
#47601=CARTESIAN_POINT('Ctrl Pts',(18.3683287675448,17.2340285880918,37.0697396972218));
#47602=CARTESIAN_POINT('Ctrl Pts',(18.3347048283782,17.2380705512396,37.1260058294533));
#47603=CARTESIAN_POINT('Ctrl Pts',(18.3256054359271,17.2391829480689,37.1417330602599));
#47604=CARTESIAN_POINT('Ctrl Pts',(18.2340295586326,17.2505978997766,37.3052993094812));
#47605=CARTESIAN_POINT('Ctrl Pts',(18.1711329317403,17.2604053948541,37.4632509139808));
#47606=CARTESIAN_POINT('Ctrl Pts',(18.1176245190937,17.2739379495544,37.675008797129));
#47607=CARTESIAN_POINT('Ctrl Pts',(18.1074155606695,17.2770273077828,37.7230670163355));
#47608=CARTESIAN_POINT('Ctrl Pts',(18.0969799969047,17.2809549122344,37.7834475823612));
#47609=CARTESIAN_POINT('Ctrl Pts',(18.0950215768474,17.2817381665362,37.7954548282611));
#47610=CARTESIAN_POINT('Ctrl Pts',(18.0920872617245,17.2829897432161,37.8145824494882));
#47611=CARTESIAN_POINT('Ctrl Pts',(18.0910373375921,17.2834557367545,37.8216912753144));
#47612=CARTESIAN_POINT('Ctrl Pts',(18.0891324357876,17.2843368247811,37.8351071583112));
#47613=CARTESIAN_POINT('Ctrl Pts',(18.0882689034234,17.2847516447674,37.8414129193153));
#47614=CARTESIAN_POINT('Ctrl Pts',(18.0863921324074,17.285689241329,37.8556410905807));
#47615=CARTESIAN_POINT('Ctrl Pts',(18.0853968629311,17.2862125731413,37.8635657135242));
#47616=CARTESIAN_POINT('Ctrl Pts',(18.082973899544,17.2875569089069,37.8838774337265));
#47617=CARTESIAN_POINT('Ctrl Pts',(18.0816170590858,17.2883801080357,37.8962724536678));
#47618=CARTESIAN_POINT('Ctrl Pts',(18.0739981010538,17.293475326153,37.9727174843485));
#47619=CARTESIAN_POINT('Ctrl Pts',(18.0708247853875,17.2978424889978,38.0370276239346));
#47620=CARTESIAN_POINT('Ctrl Pts',(18.0709935737147,17.31428569618,38.2746646705139));
#47621=CARTESIAN_POINT('Ctrl Pts',(18.0944642165516,17.326905137099,38.4471231725448));
#47622=CARTESIAN_POINT('Ctrl Pts',(18.1522690508712,17.3420340636733,38.6561813429429));
#47623=CARTESIAN_POINT('Ctrl Pts',(18.1653254647837,17.3450344570083,38.6978439437836));
#47624=CARTESIAN_POINT('Ctrl Pts',(18.182257501738,17.3484631941258,38.7460731132526));
#47625=CARTESIAN_POINT('Ctrl Pts',(18.1847706380065,17.3489616776403,38.7531007773961));
#47626=CARTESIAN_POINT('Ctrl Pts',(18.1888988060585,17.3497637237206,38.764436745071));
#47627=CARTESIAN_POINT('Ctrl Pts',(18.1904885463405,17.3500687066338,38.7687540826491));
#47628=CARTESIAN_POINT('Ctrl Pts',(18.1933377586298,17.3506084370403,38.7764072855746));
#47629=CARTESIAN_POINT('Ctrl Pts',(18.1945910478656,17.350843542876,38.7797453837177));
#47630=CARTESIAN_POINT('Ctrl Pts',(18.1973043402401,17.3513476013438,38.7869117128464));
#47631=CARTESIAN_POINT('Ctrl Pts',(18.1987672828435,17.3516163768279,38.7907387656566));
#47632=CARTESIAN_POINT('Ctrl Pts',(18.202842378769,17.3523569191907,38.8012982167963));
#47633=CARTESIAN_POINT('Ctrl Pts',(18.2054801919365,17.3528271901558,38.8080207390469));
#47634=CARTESIAN_POINT('Ctrl Pts',(18.2202726030742,17.3554157298151,38.8451057299544));
#47635=CARTESIAN_POINT('Ctrl Pts',(18.2331608717979,17.3574931123817,38.8751722125266));
#47636=CARTESIAN_POINT('Ctrl Pts',(18.2761570799848,17.3639403345041,38.9688245067489));
#47637=CARTESIAN_POINT('Ctrl Pts',(18.3089827411975,17.3681939570088,39.0311029445779));
#47638=CARTESIAN_POINT('Ctrl Pts',(18.4321675306111,17.3825664174381,39.2367138311544));
#47639=CARTESIAN_POINT('Ctrl Pts',(18.5379298023348,17.3925253510255,39.3698669711246));
#47640=CARTESIAN_POINT('Ctrl Pts',(18.6743206414446,17.4045595746219,39.5016167243006));
#47641=CARTESIAN_POINT('Ctrl Pts',(18.6891525735954,17.4058579860225,39.5154978553391));
#47642=CARTESIAN_POINT('Ctrl Pts',(18.7102345621578,17.4076909110989,39.5346128448678));
#47643=CARTESIAN_POINT('Ctrl Pts',(18.7163031315144,17.4082170978098,39.5400455707443));
#47644=CARTESIAN_POINT('Ctrl Pts',(18.7268918840167,17.4091328494995,39.5494047497403));
#47645=CARTESIAN_POINT('Ctrl Pts',(18.7313963123563,17.4095216750882,39.5533489209093));
#47646=CARTESIAN_POINT('Ctrl Pts',(18.7408167274394,17.4103333765274,39.5615204686079));
#47647=CARTESIAN_POINT('Ctrl Pts',(18.745735804203,17.4107563967674,39.5657441521222));
#47648=CARTESIAN_POINT('Ctrl Pts',(18.7574079098118,17.4117582610419,39.5756644294138));
#47649=CARTESIAN_POINT('Ctrl Pts',(18.7641789183464,17.4123379667334,39.5813395493941));
#47650=CARTESIAN_POINT('Ctrl Pts',(18.7867791445147,17.4142682099094,39.6000191298299));
#47651=CARTESIAN_POINT('Ctrl Pts',(18.802776063946,17.4156269320817,39.6128175786455));
#47652=CARTESIAN_POINT('Ctrl Pts',(18.8897476775748,17.422976644437,39.6801563748743));
#47653=CARTESIAN_POINT('Ctrl Pts',(18.9642397515028,17.4291481241327,39.7299542979281));
#47654=CARTESIAN_POINT('Ctrl Pts',(19.1486718032791,17.4441067151472,39.8354863733714));
#47655=CARTESIAN_POINT('Ctrl Pts',(19.261025986186,17.452984531183,39.8862217786245));
#47656=CARTESIAN_POINT('Ctrl Pts',(19.3889141819031,17.4624891808049,39.929826107515));
#47657=CARTESIAN_POINT('Ctrl Pts',(19.4004228934086,17.4633391538937,39.933629396558));
#47658=CARTESIAN_POINT('Ctrl Pts',(19.455728660759,17.4673960066795,39.9513299343031));
#47659=CARTESIAN_POINT('Ctrl Pts',(19.4999811172282,17.470559376807,39.9637692235998));
#47660=CARTESIAN_POINT('Ctrl Pts',(19.5520036764247,17.474151338079,39.9764059482038));
#47661=CARTESIAN_POINT('Ctrl Pts',(19.559378511362,17.4746576011455,39.9781514041098));
#47662=CARTESIAN_POINT('Ctrl Pts',(19.5712321317639,17.4754663986526,39.9808832235179));
#47663=CARTESIAN_POINT('Ctrl Pts',(19.5757043909413,17.4757704290377,39.9818971338925));
#47664=CARTESIAN_POINT('Ctrl Pts',(19.5836669684329,17.4763096914001,39.9836725100422));
#47665=CARTESIAN_POINT('Ctrl Pts',(19.587155832155,17.4765452741794,39.9844402384101));
#47666=CARTESIAN_POINT('Ctrl Pts',(19.5946127442826,17.4770472908224,39.9860594368512));
#47667=CARTESIAN_POINT('Ctrl Pts',(19.5985813462079,17.4773135634536,39.9869080771393));
#47668=CARTESIAN_POINT('Ctrl Pts',(19.6094465586485,17.47804016809,39.9891956487217));
#47669=CARTESIAN_POINT('Ctrl Pts',(19.6163485046463,17.4784990956531,39.990609352446));
#47670=CARTESIAN_POINT('Ctrl Pts',(19.65286083927,17.4809137231423,39.9978798762687));
#47671=CARTESIAN_POINT('Ctrl Pts',(19.6825997944283,17.4828347362874,40.0030793407236));
#47672=CARTESIAN_POINT('Ctrl Pts',(19.8725655977788,17.4948865477706,40.0317148910949));
#47673=CARTESIAN_POINT('Ctrl Pts',(20.0350985655018,17.5042577192961,40.0355987150944));
#47674=CARTESIAN_POINT('Ctrl Pts',(20.2851990713135,17.5194657339569,40.0100272144236));
#47675=CARTESIAN_POINT('Ctrl Pts',(20.3734259668508,17.5249770849946,39.994753912069));
#47676=CARTESIAN_POINT('Ctrl Pts',(20.4733252013152,17.531547366867,39.9702103055575));
#47677=CARTESIAN_POINT('Ctrl Pts',(20.486348052393,17.5324102894167,39.9668660612038));
#47678=CARTESIAN_POINT('Ctrl Pts',(20.5072487393737,17.5338060542022,39.9612652696919));
#47679=CARTESIAN_POINT('Ctrl Pts',(20.5151491624077,17.534336158201,39.9590941409254));
#47680=CARTESIAN_POINT('Ctrl Pts',(20.5292003551183,17.5352835470267,39.955136265343));
#47681=CARTESIAN_POINT('Ctrl Pts',(20.5353565452275,17.5357001958642,39.9533690799954));
#47682=CARTESIAN_POINT('Ctrl Pts',(20.5482170732703,17.5365739408031,39.949607937051));
#47683=CARTESIAN_POINT('Ctrl Pts',(20.5549195839117,17.5370312216496,39.947608111439));
#47684=CARTESIAN_POINT('Ctrl Pts',(20.5724213148242,17.538230368128,39.9422823018381));
#47685=CARTESIAN_POINT('Ctrl Pts',(20.5832023213006,17.5389741226529,39.938897845064));
#47686=CARTESIAN_POINT('Ctrl Pts',(20.6313222100164,17.542317078688,39.9233259550193));
#47687=CARTESIAN_POINT('Ctrl Pts',(20.6683110936727,17.5449500583316,39.9100953489295));
#47688=CARTESIAN_POINT('Ctrl Pts',(20.8574433734043,17.5587547674413,39.8358569272763));
#47689=CARTESIAN_POINT('Ctrl Pts',(21.001744542772,17.5705318381154,39.7567734683448));
#47690=CARTESIAN_POINT('Ctrl Pts',(21.1998579473352,17.5879264461201,39.6127643095402));
#47691=CARTESIAN_POINT('Ctrl Pts',(21.2623724759653,17.5936170823236,39.5610044185568));
#47692=CARTESIAN_POINT('Ctrl Pts',(21.3282496806731,17.599694283249,39.4990648460413));
#47693=CARTESIAN_POINT('Ctrl Pts',(21.3350027157138,17.6003182247579,39.4926224956073));
#47694=CARTESIAN_POINT('Ctrl Pts',(21.3449700499153,17.6012402440448,39.4829745916844));
#47695=CARTESIAN_POINT('Ctrl Pts',(21.3482200955699,17.6015410619824,39.4798064108276));
#47696=CARTESIAN_POINT('Ctrl Pts',(21.353999339144,17.6020762415774,39.4741328245952));
#47697=CARTESIAN_POINT('Ctrl Pts',(21.3565328051478,17.6023109385029,39.4716318672685));
#47698=CARTESIAN_POINT('Ctrl Pts',(21.3619969692124,17.6028173160104,39.4662078703431));
#47699=CARTESIAN_POINT('Ctrl Pts',(21.364925180861,17.6030888025655,39.4632824140943));
#47700=CARTESIAN_POINT('Ctrl Pts',(21.3730716440955,17.6038445161755,39.4550910581509));
#47701=CARTESIAN_POINT('Ctrl Pts',(21.3782690598935,17.6043271448513,39.4498044001195));
#47702=CARTESIAN_POINT('Ctrl Pts',(21.4083439720949,17.6071236847536,39.4188582545511));
#47703=CARTESIAN_POINT('Ctrl Pts',(21.4325368891581,17.6093885813076,39.3925394750878));
#47704=CARTESIAN_POINT('Ctrl Pts',(21.5096300775044,17.6167178575088,39.3038463451829));
#47705=CARTESIAN_POINT('Ctrl Pts',(21.5593003139187,17.6216261639669,39.2387773101809));
#47706=CARTESIAN_POINT('Ctrl Pts',(21.6892672435962,17.6356251438701,39.0440001113353));
#47707=CARTESIAN_POINT('Ctrl Pts',(21.7585163967497,17.6446626504381,38.9076966251383));
#47708=CARTESIAN_POINT('Ctrl Pts',(21.818508038011,17.6556957447508,38.7442397311345));
#47709=CARTESIAN_POINT('Ctrl Pts',(21.8256608063975,17.6570855495057,38.7236817093173));
#47710=CARTESIAN_POINT('Ctrl Pts',(21.8350853582162,17.6590266058653,38.6950416909375));
#47711=CARTESIAN_POINT('Ctrl Pts',(21.8376547229854,17.6595681586443,38.6870587716318));
#47712=CARTESIAN_POINT('Ctrl Pts',(21.8419877299355,17.6605032796091,38.6732890668786));
#47713=CARTESIAN_POINT('Ctrl Pts',(21.8437763678392,17.6608960304524,38.6675102249748));
#47714=CARTESIAN_POINT('Ctrl Pts',(21.8474139708435,17.6617089518437,38.6555589031751));
#47715=CARTESIAN_POINT('Ctrl Pts',(21.8492592483525,17.6621292361721,38.6493853886505));
#47716=CARTESIAN_POINT('Ctrl Pts',(21.8534931797216,17.6631123817712,38.6349574103007));
#47717=CARTESIAN_POINT('Ctrl Pts',(21.8558576621185,17.6636760158572,38.6266960528046));
#47718=CARTESIAN_POINT('Ctrl Pts',(21.8633049126199,17.6654995541002,38.6000029217329));
#47719=CARTESIAN_POINT('Ctrl Pts',(21.8681687514959,17.666766449678,38.5815117761461));
#47720=CARTESIAN_POINT('Ctrl Pts',(21.8915917510684,17.6732790334548,38.4867598634691));
#47721=CARTESIAN_POINT('Ctrl Pts',(21.9057570415868,17.6786621811664,38.4094993058944));
#47722=CARTESIAN_POINT('Ctrl Pts',(21.9251905969021,17.689993402563,38.2487962414999));
#47723=CARTESIAN_POINT('Ctrl Pts',(21.9298227348872,17.6959444392223,38.1654355077597));
#47724=CARTESIAN_POINT('Ctrl Pts',(21.9280277087644,17.7097022743309,37.9726112312428));
#47725=CARTESIAN_POINT('Ctrl Pts',(21.9176989792529,17.7174879696582,37.8634514941308));
#47726=CARTESIAN_POINT('Ctrl Pts',(21.8965296096757,17.7254584885785,37.746726703887));
#47727=CARTESIAN_POINT('Ctrl Pts',(21.894829535186,17.7260711825722,37.7377188621129));
#47728=CARTESIAN_POINT('Ctrl Pts',(21.8921981235457,17.726979849171,37.7243018242794));
#47729=CARTESIAN_POINT('Ctrl Pts',(21.8913154718088,17.7272784498782,37.7198833795929));
#47730=CARTESIAN_POINT('Ctrl Pts',(21.8897082486846,17.7278112360272,37.7119820279318));
#47731=CARTESIAN_POINT('Ctrl Pts',(21.8889895189443,17.7280457444157,37.7084980079196));
#47732=CARTESIAN_POINT('Ctrl Pts',(21.8874087570839,17.7285534894885,37.7009410170887));
#47733=CARTESIAN_POINT('Ctrl Pts',(21.8865431790448,17.7288265226612,37.6968688519004));
#47734=CARTESIAN_POINT('Ctrl Pts',(21.8840763292713,17.7295909307443,37.6854453626619));
#47735=CARTESIAN_POINT('Ctrl Pts',(21.8824452031833,17.7300806471755,37.678100458161));
#47736=CARTESIAN_POINT('Ctrl Pts',(21.8723971659813,17.7330065240863,37.6340731439594));
#47737=CARTESIAN_POINT('Ctrl Pts',(21.8629505878155,17.7353882204672,37.5976310672761));
#47738=CARTESIAN_POINT('Ctrl Pts',(21.8064155138722,17.7479958606223,37.4031551790334));
#47739=CARTESIAN_POINT('Ctrl Pts',(21.7402764417537,17.7575213592455,37.2513667855273));
#47740=CARTESIAN_POINT('Ctrl Pts',(21.6152072292645,17.7723360313542,37.04224289614));
#47741=CARTESIAN_POINT('Ctrl Pts',(21.5706897695516,17.7772136543459,36.9772017748685));
#47742=CARTESIAN_POINT('Ctrl Pts',(21.5142594828009,17.7830839248084,36.904703691549));
#47743=CARTESIAN_POINT('Ctrl Pts',(21.5060870001048,17.7839271011124,36.8944225530173));
#47744=CARTESIAN_POINT('Ctrl Pts',(21.4926496943841,17.785302723046,36.8778680510072));
#47745=CARTESIAN_POINT('Ctrl Pts',(21.4874486905661,17.7858326269113,36.871543244381));
#47746=CARTESIAN_POINT('Ctrl Pts',(21.4781199918583,17.7867786984135,36.8603449541104));
#47747=CARTESIAN_POINT('Ctrl Pts',(21.4740080424017,17.7871942261246,36.8554584649629));
#47748=CARTESIAN_POINT('Ctrl Pts',(21.4652948229567,17.7880716692282,36.8452077524058));
#47749=CARTESIAN_POINT('Ctrl Pts',(21.4606881966393,17.7885337996984,36.8398482262944));
#47750=CARTESIAN_POINT('Ctrl Pts',(21.4484240255622,17.7897595566925,36.8257372231469));
#47751=CARTESIAN_POINT('Ctrl Pts',(21.440716716112,17.7905252286306,36.8170295731357));
#47752=CARTESIAN_POINT('Ctrl Pts',(21.4043176802565,17.7941202805483,36.7766478710943));
#47753=CARTESIAN_POINT('Ctrl Pts',(21.3746591992962,17.7969900195519,36.7458653682859));
#47754=CARTESIAN_POINT('Ctrl Pts',(21.2244128649905,17.8112582015957,36.5999508609197));
#47755=CARTESIAN_POINT('Ctrl Pts',(21.0902821087874,17.8232706425524,36.4998120957231));
#47756=CARTESIAN_POINT('Ctrl Pts',(20.8802439507439,17.8403445285271,36.3817948428981));
#47757=CARTESIAN_POINT('Ctrl Pts',(20.8134411866314,17.8455396673875,36.3491789203812));
#47758=CARTESIAN_POINT('Ctrl Pts',(20.7363634780279,17.8511549138419,36.3169135302131));
#47759=CARTESIAN_POINT('Ctrl Pts',(20.7277845233722,17.8517747563765,36.3133947759825));
#47760=CARTESIAN_POINT('Ctrl Pts',(20.7149799634452,17.8526919122638,36.3082503803218));
#47761=CARTESIAN_POINT('Ctrl Pts',(20.7107736232267,17.8529919246929,36.3065775998645));
#47762=CARTESIAN_POINT('Ctrl Pts',(20.7032497179992,17.8535262322872,36.3036161163975));
#47763=CARTESIAN_POINT('Ctrl Pts',(20.699934448287,17.8537608582476,36.3023217774193));
#47764=CARTESIAN_POINT('Ctrl Pts',(20.6927477068169,17.85426772133,36.2995388438284));
#47765=CARTESIAN_POINT('Ctrl Pts',(20.6888750193855,17.854539761022,36.2980535611039));
#47766=CARTESIAN_POINT('Ctrl Pts',(20.6780304031597,17.8552985806597,36.2939344216713));
#47767=CARTESIAN_POINT('Ctrl Pts',(20.6710478643705,17.8557837408721,36.2913284242389));
#47768=CARTESIAN_POINT('Ctrl Pts',(20.6298724774408,17.858625575113,36.2762323738592));
#47769=CARTESIAN_POINT('Ctrl Pts',(20.5953441533021,17.8609313606338,36.2646707527295));
#47770=CARTESIAN_POINT('Ctrl Pts',(20.4796924579722,17.8684646130713,36.2295533124873));
#47771=CARTESIAN_POINT('Ctrl Pts',(20.3973469004971,17.8735259282211,36.2103456677576));
#47772=CARTESIAN_POINT('Ctrl Pts',(20.1673218110452,17.8874580321404,36.1723987900647));
#47773=CARTESIAN_POINT('Ctrl Pts',(20.01835609449,17.8962919318777,36.165239088503));
#47774=CARTESIAN_POINT('Ctrl Pts',(19.8481377877441,17.9071002964135,36.1767312007854));
#47775=CARTESIAN_POINT('Ctrl Pts',(19.8262505782811,17.9085025986021,36.1785848753013));
#47776=CARTESIAN_POINT('Ctrl Pts',(19.7960264935889,17.910458331585,36.1816652488226));
#47777=CARTESIAN_POINT('Ctrl Pts',(19.7876582961799,17.9110018673493,36.1825734939668));
#47778=CARTESIAN_POINT('Ctrl Pts',(19.7732786832577,17.9119394979649,36.1842294775124));
#47779=CARTESIAN_POINT('Ctrl Pts',(19.7672643038432,17.9123327652671,36.184950824484));
#47780=CARTESIAN_POINT('Ctrl Pts',(19.7548640498272,17.9131458998751,36.1864973523323));
#47781=CARTESIAN_POINT('Ctrl Pts',(19.748478717145,17.9135658771755,36.1873262015472));
#47782=CARTESIAN_POINT('Ctrl Pts',(19.7336100889894,17.9145468258784,36.1893319694351));
#47783=CARTESIAN_POINT('Ctrl Pts',(19.7251302967363,17.9151085596906,36.190533438378));
#47784=CARTESIAN_POINT('Ctrl Pts',(19.6979023691977,17.9169197516906,36.1945763876707));
#47785=CARTESIAN_POINT('Ctrl Pts',(19.6791885123543,17.9181760695534,36.1976377666332));
#47786=CARTESIAN_POINT('Ctrl Pts',(19.5844616783375,17.9245957942414,36.2145714753432));
#47787=CARTESIAN_POINT('Ctrl Pts',(19.5092953440221,17.9298922813303,36.2327241611409));
#47788=CARTESIAN_POINT('Ctrl Pts',(19.4216019214197,17.9363075520093,36.2595632930522));
#47789=CARTESIAN_POINT('Ctrl Pts',(19.4078265464337,17.9373222382774,36.2639493266696));
#47790=CARTESIAN_POINT('Ctrl Pts',(19.3941039849792,17.9383397493623,36.2684889910563));
#47791=CARTESIAN_POINT('Origin',(20.,-1.3495818343519,38.1));
#47792=CARTESIAN_POINT('',(19.3941040358239,18.9053562004634,36.268488974236));
#47793=CARTESIAN_POINT('',(19.3941040087494,18.7329718898071,36.2684889831927));
#47794=CARTESIAN_POINT('',(19.3941040087494,-1.3495818343519,36.2684889831927));
#47795=CARTESIAN_POINT('',(18.0708707114912,18.2691024802153,38.0983431603818));
#47796=CARTESIAN_POINT('Ctrl Pts',(19.3941040358239,18.9053562004634,36.268488974236));
#47797=CARTESIAN_POINT('Ctrl Pts',(19.4279865928287,18.9028884425737,36.257280030224));
#47798=CARTESIAN_POINT('Ctrl Pts',(19.4621774215529,18.9003957441515,36.2470122283997));
#47799=CARTESIAN_POINT('Ctrl Pts',(19.6279301066995,18.8883134741058,36.202210854192));
#47800=CARTESIAN_POINT('Ctrl Pts',(19.7625999656545,18.87846861129,36.180708736018));
#47801=CARTESIAN_POINT('Ctrl Pts',(19.9444078487693,18.8657482504664,36.1711210718187));
#47802=CARTESIAN_POINT('Ctrl Pts',(19.9904840652544,18.8625766649059,36.1703433869034));
#47803=CARTESIAN_POINT('Ctrl Pts',(20.0441435471345,18.8589755877585,36.1713601636353));
#47804=CARTESIAN_POINT('Ctrl Pts',(20.0517384120818,18.8584680646239,36.1715489602943));
#47805=CARTESIAN_POINT('Ctrl Pts',(20.0639211133723,18.8576576473258,36.1719238274883));
#47806=CARTESIAN_POINT('Ctrl Pts',(20.0685096516886,18.8573532478843,36.1720814165407));
#47807=CARTESIAN_POINT('Ctrl Pts',(20.0766680465245,18.8568135715132,36.1723907725738));
#47808=CARTESIAN_POINT('Ctrl Pts',(20.0802380916115,18.8565779417876,36.1725360775168));
#47809=CARTESIAN_POINT('Ctrl Pts',(20.0878588872093,18.8560760957557,36.1728674629983));
#47810=CARTESIAN_POINT('Ctrl Pts',(20.0919094542126,18.8558100392864,36.1730563962044));
#47811=CARTESIAN_POINT('Ctrl Pts',(20.1029805800088,18.8550846378359,36.1736077824848));
#47812=CARTESIAN_POINT('Ctrl Pts',(20.1099998867849,18.8546266895134,36.1739958452306));
#47813=CARTESIAN_POINT('Ctrl Pts',(20.1469385480426,18.8522264016984,36.176240601705));
#47814=CARTESIAN_POINT('Ctrl Pts',(20.1768156307629,18.8503182619047,36.1787562275007));
#47815=CARTESIAN_POINT('Ctrl Pts',(20.3677859082086,18.8382660162591,36.1993288814617));
#47816=CARTESIAN_POINT('Ctrl Pts',(20.5261336682632,18.8288854925308,36.236934522012));
#47817=CARTESIAN_POINT('Ctrl Pts',(20.7617214358697,18.8136638026088,36.325363683888));
#47818=CARTESIAN_POINT('Ctrl Pts',(20.8432163549248,18.8081487846095,36.3626063647711));
#47819=CARTESIAN_POINT('Ctrl Pts',(20.9336379624654,18.8015744429003,36.4117928055435));
#47820=CARTESIAN_POINT('Ctrl Pts',(20.9453825693801,18.8007114187338,36.4183415450199));
#47821=CARTESIAN_POINT('Ctrl Pts',(20.964171898234,18.79931552053,36.4290774265798));
#47822=CARTESIAN_POINT('Ctrl Pts',(20.9712602129664,18.7987853855734,36.4331876857271));
#47823=CARTESIAN_POINT('Ctrl Pts',(20.9838422407657,18.797837960456,36.4405910614918));
#47824=CARTESIAN_POINT('Ctrl Pts',(20.9893461761992,18.7974213064506,36.4438666352287));
#47825=CARTESIAN_POINT('Ctrl Pts',(21.0008261948645,18.7965475702287,36.4507764235942));
#47826=CARTESIAN_POINT('Ctrl Pts',(21.0067990193744,18.7960903033636,36.4544158454446));
#47827=CARTESIAN_POINT('Ctrl Pts',(21.0223683947148,18.7948912373375,36.4640192286843));
#47828=CARTESIAN_POINT('Ctrl Pts',(21.0319324603638,18.7941475497584,36.4700350903479));
#47829=CARTESIAN_POINT('Ctrl Pts',(21.0744964436095,18.7908053466849,36.4973328936649));
#47830=CARTESIAN_POINT('Ctrl Pts',(21.1068927751893,18.7881730718187,36.5195340988735));
#47831=CARTESIAN_POINT('Ctrl Pts',(21.2708892342792,18.7743702751573,36.6394372117908));
#47832=CARTESIAN_POINT('Ctrl Pts',(21.3903082149122,18.7625945067091,36.7526217243822));
#47833=CARTESIAN_POINT('Ctrl Pts',(21.5452710390451,18.7451989200551,36.942305347138));
#47834=CARTESIAN_POINT('Ctrl Pts',(21.5925746065654,18.7395062365368,37.0082908594777));
#47835=CARTESIAN_POINT('Ctrl Pts',(21.6405370062164,18.7334271307516,37.0849788209207));
#47836=CARTESIAN_POINT('Ctrl Pts',(21.6454285534588,18.7328031707232,37.0929277350625));
#47837=CARTESIAN_POINT('Ctrl Pts',(21.6526129269065,18.7318811289652,37.1047946589798));
#47838=CARTESIAN_POINT('Ctrl Pts',(21.6549498358871,18.7315803068929,37.1086856206448));
#47839=CARTESIAN_POINT('Ctrl Pts',(21.6590951614778,18.731045122223,37.1156431158905));
#47840=CARTESIAN_POINT('Ctrl Pts',(21.6609088378502,18.7308104243373,37.1187064337312));
#47841=CARTESIAN_POINT('Ctrl Pts',(21.664812923785,18.7303040473092,37.1253423073996));
#47842=CARTESIAN_POINT('Ctrl Pts',(21.6669003140247,18.730032562181,37.1289165675148));
#47843=CARTESIAN_POINT('Ctrl Pts',(21.6726941395154,18.7292768587188,37.1389111230811));
#47844=CARTESIAN_POINT('Ctrl Pts',(21.6763751438252,18.7287942386887,37.1453461909082));
#47845=CARTESIAN_POINT('Ctrl Pts',(21.6975841375381,18.7259978670986,37.1829243442474));
#47846=CARTESIAN_POINT('Ctrl Pts',(21.7142824358835,18.7237331232623,37.2145307535176));
#47847=CARTESIAN_POINT('Ctrl Pts',(21.7662636980626,18.7164046056339,37.3199103185352));
#47848=CARTESIAN_POINT('Ctrl Pts',(21.7977382892531,18.7114968679667,37.3954670749589));
#47849=CARTESIAN_POINT('Ctrl Pts',(21.8738690109192,18.6974976324576,37.6169066532795));
#47850=CARTESIAN_POINT('Ctrl Pts',(21.9061587211823,18.6884593674046,37.7663581157598));
#47851=CARTESIAN_POINT('Ctrl Pts',(21.9225827392108,18.6774254373416,37.9397130966413));
#47852=CARTESIAN_POINT('Ctrl Pts',(21.9242687082187,18.6760356831469,37.9614137158783));
#47853=CARTESIAN_POINT('Ctrl Pts',(21.9260951240433,18.6740946853724,37.9915082624133));
#47854=CARTESIAN_POINT('Ctrl Pts',(21.9265485424183,18.6735531398232,37.9998820991973));
#47855=CARTESIAN_POINT('Ctrl Pts',(21.9272350225703,18.6726180273037,38.0143009977634));
#47856=CARTESIAN_POINT('Ctrl Pts',(21.927494277311,18.6722252776356,38.0203447380468));
#47857=CARTESIAN_POINT('Ctrl Pts',(21.9279709641847,18.6714123548817,38.0328283071692));
#47858=CARTESIAN_POINT('Ctrl Pts',(21.9281845662766,18.670992067998,38.0392681982428));
#47859=CARTESIAN_POINT('Ctrl Pts',(21.9286077367307,18.670008909832,38.0542988125277));
#47860=CARTESIAN_POINT('Ctrl Pts',(21.9287921734676,18.6694452656836,38.0628900517682));
#47861=CARTESIAN_POINT('Ctrl Pts',(21.9292018549228,18.667621667027,38.090600472372));
#47862=CARTESIAN_POINT('Ctrl Pts',(21.9292002484896,18.6663547204668,38.109721361915));
#47863=CARTESIAN_POINT('Ctrl Pts',(21.9277410707954,18.6598416983572,38.2073210527086));
#47864=CARTESIAN_POINT('Ctrl Pts',(21.9217791785243,18.6544581425518,38.2856486197102));
#47865=CARTESIAN_POINT('Ctrl Pts',(21.8996781125919,18.643126792372,38.4460079327577));
#47866=CARTESIAN_POINT('Ctrl Pts',(21.8829458212707,18.6371760651468,38.5277988937013));
#47867=CARTESIAN_POINT('Ctrl Pts',(21.8321443296497,18.6234187330786,38.7138121255422));
#47868=CARTESIAN_POINT('Ctrl Pts',(21.7943791787877,18.6156332331695,38.8167477653367));
#47869=CARTESIAN_POINT('Ctrl Pts',(21.7442055763267,18.6076628822398,38.9242411610009));
#47870=CARTESIAN_POINT('Ctrl Pts',(21.7402692573582,18.6070501814031,38.9325199721509));
#47871=CARTESIAN_POINT('Ctrl Pts',(21.7343102672356,18.606141506179,38.9448258727096));
#47872=CARTESIAN_POINT('Ctrl Pts',(21.7323323265838,18.605842903625,38.9488742954846));
#47873=CARTESIAN_POINT('Ctrl Pts',(21.7287673888927,18.6053101148966,38.9561066095845));
#47874=CARTESIAN_POINT('Ctrl Pts',(21.7271857580987,18.6050756057683,38.9592930638519));
#47875=CARTESIAN_POINT('Ctrl Pts',(21.7237340492838,18.6045678598723,38.9661990622883));
#47876=CARTESIAN_POINT('Ctrl Pts',(21.7218607471181,18.604294826613,38.969916925064));
#47877=CARTESIAN_POINT('Ctrl Pts',(21.7165682537206,18.6035304201946,38.980336635482));
#47878=CARTESIAN_POINT('Ctrl Pts',(21.7131218246948,18.6030407054971,38.9870246782026));
#47879=CARTESIAN_POINT('Ctrl Pts',(21.6922015669189,18.6001148778458,39.0270451897662));
#47880=CARTESIAN_POINT('Ctrl Pts',(21.6737931588567,18.5977332267981,39.0598832445379));
#47881=CARTESIAN_POINT('Ctrl Pts',(21.5696369614075,18.5851261390324,39.233563757592));
#47882=CARTESIAN_POINT('Ctrl Pts',(21.467056640143,18.5756010858206,39.363519889001));
#47883=CARTESIAN_POINT('Ctrl Pts',(21.2928922685819,18.5607864625144,39.5339370312864));
#47884=CARTESIAN_POINT('Ctrl Pts',(21.2332835541578,18.5559083310408,39.5855151377765));
#47885=CARTESIAN_POINT('Ctrl Pts',(21.1602557659134,18.5500375004795,39.6412727244261));
#47886=CARTESIAN_POINT('Ctrl Pts',(21.1497359160123,18.5491943069441,39.6491360053703));
#47887=CARTESIAN_POINT('Ctrl Pts',(21.1325281305167,18.5478186616568,39.6617264952663));
#47888=CARTESIAN_POINT('Ctrl Pts',(21.1258888255783,18.5472887518036,39.66651969712));
#47889=CARTESIAN_POINT('Ctrl Pts',(21.1140175554239,18.5463426726037,39.67497562828));
#47890=CARTESIAN_POINT('Ctrl Pts',(21.1087975084621,18.5459271432117,39.6786549423681));
#47891=CARTESIAN_POINT('Ctrl Pts',(21.0977626717661,18.5450496996428,39.6863510390286));
#47892=CARTESIAN_POINT('Ctrl Pts',(21.0919438975729,18.5445875704024,39.690361916317));
#47893=CARTESIAN_POINT('Ctrl Pts',(21.0764928330725,18.5433618238192,39.700887553645));
#47894=CARTESIAN_POINT('Ctrl Pts',(21.0668235698513,18.5425961611333,39.7073472679779));
#47895=CARTESIAN_POINT('Ctrl Pts',(21.0213486366556,18.5390012350159,39.7371364685813));
#47896=CARTESIAN_POINT('Ctrl Pts',(20.9848349623899,18.5361316160571,39.7593578463153));
#47897=CARTESIAN_POINT('Ctrl Pts',(20.8024049678732,18.5218634648756,39.8622375198034));
#47898=CARTESIAN_POINT('Ctrl Pts',(20.6472064754203,18.5098509131442,39.9249495083712));
#47899=CARTESIAN_POINT('Ctrl Pts',(20.4572099081198,18.4959375204752,39.9744017679639));
#47900=CARTESIAN_POINT('Ctrl Pts',(20.4283265846151,18.4938456205883,39.9812122014931));
#47901=CARTESIAN_POINT('Ctrl Pts',(20.354319242381,18.4885607628087,39.9968695137484));
#47902=CARTESIAN_POINT('Ctrl Pts',(20.3090116240405,18.485395651227,40.0047752310021));
#47903=CARTESIAN_POINT('Ctrl Pts',(20.2559523982726,18.4818019558225,40.0120900541216));
#47904=CARTESIAN_POINT('Ctrl Pts',(20.2484377585391,18.481295617541,40.0130809418328));
#47905=CARTESIAN_POINT('Ctrl Pts',(20.2363672141464,18.4804867229273,40.0146002529206));
#47906=CARTESIAN_POINT('Ctrl Pts',(20.23181501808,18.480182670097,40.01515675256));
#47907=CARTESIAN_POINT('Ctrl Pts',(20.2237133447715,18.4796433820441,40.0161178611919));
#47908=CARTESIAN_POINT('Ctrl Pts',(20.2201646815855,18.4794077959006,40.0165288498716));
#47909=CARTESIAN_POINT('Ctrl Pts',(20.2125823913388,18.4789057879544,40.0173856554739));
#47910=CARTESIAN_POINT('Ctrl Pts',(20.2085484999104,18.4786395273031,40.0178286025767));
#47911=CARTESIAN_POINT('Ctrl Pts',(20.1975087096364,18.4779129913451,40.0190055984819));
#47912=CARTESIAN_POINT('Ctrl Pts',(20.1905000546746,18.4774541200304,40.0197140178416));
#47913=CARTESIAN_POINT('Ctrl Pts',(20.1534525944717,18.4750403299827,40.0232538033017));
#47914=CARTESIAN_POINT('Ctrl Pts',(20.1233524050859,18.4731200694443,40.0254187389954));
#47915=CARTESIAN_POINT('Ctrl Pts',(19.931466875929,18.4610682259363,40.0347011196064));
#47916=CARTESIAN_POINT('Ctrl Pts',(19.7693640057219,18.4516965015293,40.022130225164));
#47917=CARTESIAN_POINT('Ctrl Pts',(19.523117959376,18.4364876902177,39.9713969670692));
#47918=CARTESIAN_POINT('Ctrl Pts',(19.4368844454189,18.4309761353501,39.9472793050387));
#47919=CARTESIAN_POINT('Ctrl Pts',(19.3399759327773,18.4244056264147,39.9127580000953));
#47920=CARTESIAN_POINT('Ctrl Pts',(19.3273579228201,18.4235426967808,39.9081139227264));
#47921=CARTESIAN_POINT('Ctrl Pts',(19.3071306139714,18.4221469219908,39.9004281997334));
#47922=CARTESIAN_POINT('Ctrl Pts',(19.2994902051603,18.4216168151261,39.8974692521485));
#47923=CARTESIAN_POINT('Ctrl Pts',(19.2859112233468,18.4206694220664,39.8921107103568));
#47924=CARTESIAN_POINT('Ctrl Pts',(19.279965279406,18.4202527718719,39.8897300295323));
#47925=CARTESIAN_POINT('Ctrl Pts',(19.2685206941146,18.419447274567,39.8850814993782));
#47926=CARTESIAN_POINT('Ctrl Pts',(19.2630204616251,18.4190585685583,39.8828177397166));
#47927=CARTESIAN_POINT('Ctrl Pts',(19.2484957368356,18.4180278404939,39.8767610213651));
#47928=CARTESIAN_POINT('Ctrl Pts',(19.2394895883261,18.4173843669203,39.8729247847466));
#47929=CARTESIAN_POINT('Ctrl Pts',(19.2047780672397,18.4148870883174,39.8578259983877));
#47930=CARTESIAN_POINT('Ctrl Pts',(19.1792915255596,18.4130167389818,39.8460720554327));
#47931=CARTESIAN_POINT('Ctrl Pts',(19.1157950825728,18.4082609821854,39.815091275985));
#47932=CARTESIAN_POINT('Ctrl Pts',(19.0781502118757,18.405352447107,39.7951545449619));
#47933=CARTESIAN_POINT('Ctrl Pts',(18.951568167736,18.3952640196245,39.7226528447727));
#47934=CARTESIAN_POINT('Ctrl Pts',(18.8662141408769,18.3879106766327,39.6642049910201));
#47935=CARTESIAN_POINT('Ctrl Pts',(18.7485382815897,18.377106009697,39.5689126724992));
#47936=CARTESIAN_POINT('Ctrl Pts',(18.7122662266137,18.3736728269615,39.537220521548));
#47937=CARTESIAN_POINT('Ctrl Pts',(18.6635745399251,18.368949740658,39.4913521595892));
#47938=CARTESIAN_POINT('Ctrl Pts',(18.6501195729557,18.3676317706043,39.47830211078));
#47939=CARTESIAN_POINT('Ctrl Pts',(18.6282397353287,18.365469779963,39.4564529576632));
#47940=CARTESIAN_POINT('Ctrl Pts',(18.6197043500747,18.3646215120667,39.4477665898224));
#47941=CARTESIAN_POINT('Ctrl Pts',(18.5862182690156,18.361275996785,39.4130363828288));
#47942=CARTESIAN_POINT('Ctrl Pts',(18.5619159151269,18.3588086015177,39.3863739339686));
#47943=CARTESIAN_POINT('Ctrl Pts',(18.5337694767405,18.3559182821019,39.3536986790859));
#47944=CARTESIAN_POINT('Ctrl Pts',(18.5291945236669,18.3554474121623,39.3483283141154));
#47945=CARTESIAN_POINT('Ctrl Pts',(18.521764521934,18.3546810940101,39.3395089640379));
#47946=CARTESIAN_POINT('Ctrl Pts',(18.5188918870594,18.3543844192641,39.3360749812733));
#47947=CARTESIAN_POINT('Ctrl Pts',(18.5137594279751,18.3538536935155,39.3298959956339));
#47948=CARTESIAN_POINT('Ctrl Pts',(18.511495224394,18.3536193302982,39.3271547301269));
#47949=CARTESIAN_POINT('Ctrl Pts',(18.5065824144553,18.3531103133785,39.3211732004809));
#47950=CARTESIAN_POINT('Ctrl Pts',(18.5039367753411,18.3528358717413,39.3179305805471));
#47951=CARTESIAN_POINT('Ctrl Pts',(18.4965009742207,18.3520635205958,39.3087561241266));
#47952=CARTESIAN_POINT('Ctrl Pts',(18.4917353301862,18.3515673253521,39.3028043808685));
#47953=CARTESIAN_POINT('Ctrl Pts',(18.4625108914312,18.348515978153,39.2658595885145));
#47954=CARTESIAN_POINT('Ctrl Pts',(18.4389710669212,18.3460208678525,39.234147489685));
#47955=CARTESIAN_POINT('Ctrl Pts',(18.3462116290715,18.3359278021567,39.1008192724799));
#47956=CARTESIAN_POINT('Ctrl Pts',(18.2858046671633,18.3286983579506,38.9934175308054));
#47957=CARTESIAN_POINT('Ctrl Pts',(18.2176969925881,18.3186159956408,38.8395868333897));
#47958=CARTESIAN_POINT('Ctrl Pts',(18.2008303435292,18.3158887646577,38.7975535797615));
#47959=CARTESIAN_POINT('Ctrl Pts',(18.1765130489254,18.3115224209491,38.7301841915164));
#47960=CARTESIAN_POINT('Ctrl Pts',(18.1680764458122,18.3099056265385,38.7052212738422));
#47961=CARTESIAN_POINT('Ctrl Pts',(18.1451153433479,18.3051807115958,38.6323970628846));
#47962=CARTESIAN_POINT('Ctrl Pts',(18.1319383003056,18.3020388113213,38.5841369009836));
#47963=CARTESIAN_POINT('Ctrl Pts',(18.1177952202452,18.2980259177535,38.5230932404615));
#47964=CARTESIAN_POINT('Ctrl Pts',(18.1150601675272,18.2972116968971,38.5107365806387));
#47965=CARTESIAN_POINT('Ctrl Pts',(18.1109254715718,18.2959173272052,38.4911448223578));
#47966=CARTESIAN_POINT('Ctrl Pts',(18.1094453317726,18.2954397353801,38.4839269331126));
#47967=CARTESIAN_POINT('Ctrl Pts',(18.1067673281757,18.2945483255462,38.4704765639346));
#47968=CARTESIAN_POINT('Ctrl Pts',(18.1055587967007,18.2941348516338,38.4642462899228));
#47969=CARTESIAN_POINT('Ctrl Pts',(18.1032531762537,18.2933235075824,38.4520383207266));
#47970=CARTESIAN_POINT('Ctrl Pts',(18.1021535483972,18.2929257230616,38.4460611757613));
#47971=CARTESIAN_POINT('Ctrl Pts',(18.0997488500494,18.2920308691293,38.432633929072));
#47972=CARTESIAN_POINT('Ctrl Pts',(18.0984593192382,18.2915333157581,38.4251811807504));
#47973=CARTESIAN_POINT('Ctrl Pts',(18.095328484002,18.2902792790412,38.4064310570249));
#47974=CARTESIAN_POINT('Ctrl Pts',(18.0935438599705,18.2895210313382,38.3951246400291));
#47975=CARTESIAN_POINT('Ctrl Pts',(18.0778019814019,18.2824029989518,38.2892847239816));
#47976=CARTESIAN_POINT('Ctrl Pts',(18.0707886681054,18.2758266780971,38.1938697863096));
#47977=CARTESIAN_POINT('Ctrl Pts',(18.0708707114912,18.2691024802153,38.0983431603818));
#47978=CARTESIAN_POINT('Ctrl Pts',(18.0708707098941,18.2691026111891,38.0983450210486));
#47979=CARTESIAN_POINT('Ctrl Pts',(18.0709927887356,18.2590858989335,37.9560435925063));
#47980=CARTESIAN_POINT('Ctrl Pts',(18.0868588827055,18.2487689296965,37.8141939336366));
#47981=CARTESIAN_POINT('Ctrl Pts',(18.1270478385106,18.2360716426373,37.6360873122555));
#47982=CARTESIAN_POINT('Ctrl Pts',(18.1371422810743,18.2333104483011,37.5970820586233));
#47983=CARTESIAN_POINT('Ctrl Pts',(18.1506036166244,18.23009793581,37.5510607131297));
#47984=CARTESIAN_POINT('Ctrl Pts',(18.1527996249639,18.2295866233175,37.543715807505));
#47985=CARTESIAN_POINT('Ctrl Pts',(18.156264691227,18.2287993813945,37.5323731359882));
#47986=CARTESIAN_POINT('Ctrl Pts',(18.1575030700035,18.2285217381387,37.5283661929623));
#47987=CARTESIAN_POINT('Ctrl Pts',(18.1598152317272,18.2280101752501,37.5209704568609));
#47988=CARTESIAN_POINT('Ctrl Pts',(18.1608853062107,18.2277760517167,37.5175806178726));
#47989=CARTESIAN_POINT('Ctrl Pts',(18.1633208047732,18.2272490508019,37.5099389590244));
#47990=CARTESIAN_POINT('Ctrl Pts',(18.1646916227376,18.226956491189,37.5056889201785));
#47991=CARTESIAN_POINT('Ctrl Pts',(18.1682544544884,18.226206353967,37.4947727247075));
#47992=CARTESIAN_POINT('Ctrl Pts',(18.1704681282575,18.2257500051746,37.4881136280383));
#47993=CARTESIAN_POINT('Ctrl Pts',(18.1840886098786,18.2229992349661,37.4478757676948));
#47994=CARTESIAN_POINT('Ctrl Pts',(18.196384057608,18.2207530073682,37.4146022275572));
#47995=CARTESIAN_POINT('Ctrl Pts',(18.2616062774572,18.2098320683145,37.2520352118364));
#47996=CARTESIAN_POINT('Ctrl Pts',(18.3275546142103,18.2016718832744,37.128407939038));
#47997=CARTESIAN_POINT('Ctrl Pts',(18.4461706633492,18.1890107699173,36.9545011753525));
#47998=CARTESIAN_POINT('Ctrl Pts',(18.4892419832452,18.1847059514516,36.8982670404358));
#47999=CARTESIAN_POINT('Ctrl Pts',(18.5527205047,18.178623330714,36.8242097016456));
#48000=CARTESIAN_POINT('Ctrl Pts',(18.5705581466442,18.1769398363856,36.8042551538008));
#48001=CARTESIAN_POINT('Ctrl Pts',(18.6021370776523,18.1739975714233,36.7703744207057));
#48002=CARTESIAN_POINT('Ctrl Pts',(18.6156859794422,18.1727467061579,36.7562739941704));
#48003=CARTESIAN_POINT('Ctrl Pts',(18.6353993109885,18.1709415702723,36.7363728270069));
#48004=CARTESIAN_POINT('Ctrl Pts',(18.6413915057379,18.1703947811229,36.7304025909208));
#48005=CARTESIAN_POINT('Ctrl Pts',(18.652065087305,18.1694240592722,36.7199070978753));
#48006=CARTESIAN_POINT('Ctrl Pts',(18.6567305132805,18.169000835926,36.7153657408262));
#48007=CARTESIAN_POINT('Ctrl Pts',(18.6657058841987,18.1681886414293,36.70671710914));
#48008=CARTESIAN_POINT('Ctrl Pts',(18.6700120357579,18.1677998428589,36.702605991474));
#48009=CARTESIAN_POINT('Ctrl Pts',(18.6812601820085,18.166786465465,36.6919663848167));
#48010=CARTESIAN_POINT('Ctrl Pts',(18.6882315761584,18.1661605576443,36.6854693478907));
#48011=CARTESIAN_POINT('Ctrl Pts',(18.7122253482798,18.1640134625408,36.663438107282));
#48012=CARTESIAN_POINT('Ctrl Pts',(18.7294772451185,18.1624817388153,36.6481579022675));
#48013=CARTESIAN_POINT('Ctrl Pts',(18.7514540215372,18.1605446002153,36.6293845368507));
#48014=CARTESIAN_POINT('Ctrl Pts',(18.7559272159538,18.1601510287671,36.6255984917529));
#48015=CARTESIAN_POINT('Ctrl Pts',(18.7647635617159,18.1593749618448,36.6181883827864));
#48016=CARTESIAN_POINT('Ctrl Pts',(18.7691255852936,18.1589925207967,36.6145630604229));
#48017=CARTESIAN_POINT('Ctrl Pts',(18.8808201560189,18.1492163804646,36.5225623552322));
#48018=CARTESIAN_POINT('Ctrl Pts',(18.9973611441368,18.1393626800269,36.4460423973926));
#48019=CARTESIAN_POINT('Ctrl Pts',(19.193876158995,18.1236100169408,36.3454649978827));
#48020=CARTESIAN_POINT('Ctrl Pts',(19.2689651970021,18.1177790844306,36.3128742318829));
#48021=CARTESIAN_POINT('Ctrl Pts',(19.3618940954089,18.1109345064276,36.2793813001041));
#48022=CARTESIAN_POINT('Ctrl Pts',(19.3779634961239,18.1097640782246,36.2738285480579));
#48023=CARTESIAN_POINT('Ctrl Pts',(19.3941040099181,18.1086029180356,36.2684889828061));
#48024=CARTESIAN_POINT('',(18.0708700800916,18.0972931656481,38.1005558905092));
#48025=CARTESIAN_POINT('Ctrl Pts',(19.3941039849792,17.9383397493623,36.2684889910563));
#48026=CARTESIAN_POINT('Ctrl Pts',(19.3277365019718,17.9432608167489,36.2904445202804));
#48027=CARTESIAN_POINT('Ctrl Pts',(19.2626045320947,17.94825059431,36.3159934977218));
#48028=CARTESIAN_POINT('Ctrl Pts',(19.0990040968448,17.9610814169626,36.3906637379445));
#48029=CARTESIAN_POINT('Ctrl Pts',(19.0030818212519,17.9689029729662,36.4447706847563));
#48030=CARTESIAN_POINT('Ctrl Pts',(18.904715536788,17.9769053466831,36.5119261875009));
#48031=CARTESIAN_POINT('Ctrl Pts',(18.8971859309992,17.9775176980835,36.5171457342324));
#48032=CARTESIAN_POINT('Ctrl Pts',(18.8860098446164,17.9784259575908,36.5250114976304));
#48033=CARTESIAN_POINT('Ctrl Pts',(18.8823351203309,17.97872449042,36.5276170737809));
#48034=CARTESIAN_POINT('Ctrl Pts',(18.875857808555,17.9792504694546,36.5322440145261));
#48035=CARTESIAN_POINT('Ctrl Pts',(18.8730515018359,17.9794782698759,36.5342600536114));
#48036=CARTESIAN_POINT('Ctrl Pts',(18.8702364811364,17.9797066930512,36.5362938419746));
#48037=CARTESIAN_POINT('Ctrl Pts',(18.8702224061067,17.9797078351591,36.5363040111524));
#48038=CARTESIAN_POINT('Ctrl Pts',(18.8701944404558,17.9797101044071,36.5363242168478));
#48039=CARTESIAN_POINT('Ctrl Pts',(18.8701805493144,17.9797112315895,36.5363342537338));
#48040=CARTESIAN_POINT('Ctrl Pts',(18.8701529457148,17.9797134714514,36.5363541989603));
#48041=CARTESIAN_POINT('Ctrl Pts',(18.8701392339535,17.9797145840743,36.5363641067899));
#48042=CARTESIAN_POINT('Ctrl Pts',(18.8701119880107,17.979716794907,36.5363837946793));
#48043=CARTESIAN_POINT('Ctrl Pts',(18.8700984530356,17.9797178931811,36.5363935753054));
#48044=CARTESIAN_POINT('Ctrl Pts',(18.8700715554113,17.9797200757425,36.5364130125634));
#48045=CARTESIAN_POINT('Ctrl Pts',(18.8700581932288,17.979721159992,36.5364226688512));
#48046=CARTESIAN_POINT('Ctrl Pts',(18.8700316384551,17.9797233147261,36.5364418593885));
#48047=CARTESIAN_POINT('Ctrl Pts',(18.8700184458732,17.9797243852101,36.5364513936247));
#48048=CARTESIAN_POINT('Ctrl Pts',(18.8699922271578,17.9797265126685,36.5364703423106));
#48049=CARTESIAN_POINT('Ctrl Pts',(18.8699792009983,17.979727569645,36.5364797567726));
#48050=CARTESIAN_POINT('Ctrl Pts',(18.8699533116913,17.9797296703675,36.5364984683748));
#48051=CARTESIAN_POINT('Ctrl Pts',(18.8699404486903,17.9797307141015,36.5365077654028));
#48052=CARTESIAN_POINT('Ctrl Pts',(18.8699148828083,17.9797327885738,36.5365262442089));
#48053=CARTESIAN_POINT('Ctrl Pts',(18.8699021799507,17.9797338193101,36.536535425964));
#48054=CARTESIAN_POINT('Ctrl Pts',(18.8698769312513,17.979735868039,36.5365536764501));
#48055=CARTESIAN_POINT('Ctrl Pts',(18.8698643855199,17.9797368860226,36.5365627450955));
#48056=CARTESIAN_POINT('Ctrl Pts',(18.8665249059686,17.9800078570793,36.5389767393582));
#48057=CARTESIAN_POINT('Ctrl Pts',(18.8632056188321,17.9802770777515,36.5413923056859));
#48058=CARTESIAN_POINT('Ctrl Pts',(18.8563288971778,17.9808346597385,36.5464304013698));
#48059=CARTESIAN_POINT('Ctrl Pts',(18.8527727084887,17.981122906609,36.5490546006509));
#48060=CARTESIAN_POINT('Ctrl Pts',(18.8436975604666,17.9818583307661,36.5557996682553));
#48061=CARTESIAN_POINT('Ctrl Pts',(18.8381915396358,17.9823043688936,36.559937955469));
#48062=CARTESIAN_POINT('Ctrl Pts',(18.8222387969623,17.9835966206416,36.5720621711873));
#48063=CARTESIAN_POINT('Ctrl Pts',(18.8118511912981,17.98443798512,36.5801256994036));
#48064=CARTESIAN_POINT('Ctrl Pts',(18.6795083383585,17.9951680270764,36.6850448182652));
#48065=CARTESIAN_POINT('Ctrl Pts',(18.5696174930387,18.0042309761275,36.7962299322465));
#48066=CARTESIAN_POINT('Ctrl Pts',(18.4085889332594,18.0200426334144,37.0043369298933));
#48067=CARTESIAN_POINT('Ctrl Pts',(18.3501040333848,18.026599804252,37.0945621384814));
#48068=CARTESIAN_POINT('Ctrl Pts',(18.2929082324169,18.0343332591703,37.201350440622));
#48069=CARTESIAN_POINT('Ctrl Pts',(18.2865179946428,18.035219407154,37.2135956143202));
#48070=CARTESIAN_POINT('Ctrl Pts',(18.2764986973697,18.0366454652541,37.2333081720509));
#48071=CARTESIAN_POINT('Ctrl Pts',(18.2727853177892,18.0371824400009,37.2407323450648));
#48072=CARTESIAN_POINT('Ctrl Pts',(18.2662849442655,18.0381377069583,37.2539409672086));
#48073=CARTESIAN_POINT('Ctrl Pts',(18.2634786782526,18.0385553251934,37.2597158344308));
#48074=CARTESIAN_POINT('Ctrl Pts',(18.2576977755182,18.0394266500136,37.2717646915404));
#48075=CARTESIAN_POINT('Ctrl Pts',(18.2547280826925,18.0398805192784,37.2780409376645));
#48076=CARTESIAN_POINT('Ctrl Pts',(18.2471126302361,18.0410609237232,37.2943630302245));
#48077=CARTESIAN_POINT('Ctrl Pts',(18.2425193802715,18.0417892404303,37.3044329564387));
#48078=CARTESIAN_POINT('Ctrl Pts',(18.2229428513685,18.0449661634383,37.3483481917766));
#48079=CARTESIAN_POINT('Ctrl Pts',(18.2088496002262,18.0474445565694,37.3825792892292));
#48080=CARTESIAN_POINT('Ctrl Pts',(18.1737736068415,18.054165550835,37.4752640666428));
#48081=CARTESIAN_POINT('Ctrl Pts',(18.1546152883436,18.0584627071874,37.5343571908967));
#48082=CARTESIAN_POINT('Ctrl Pts',(18.0935163511218,18.0748294278555,37.7592688521627));
#48083=CARTESIAN_POINT('Ctrl Pts',(18.07083099567,18.0873145772518,37.9294803634274));
#48084=CARTESIAN_POINT('Ctrl Pts',(18.0708700503369,18.0989811937323,38.1004406959586));
#48085=CARTESIAN_POINT('Ctrl Pts',(18.0708700800916,18.0972931656481,38.1005558905092));
#48086=CARTESIAN_POINT('Ctrl Pts',(18.0708789271142,18.0993153349082,38.1312580803398));
#48087=CARTESIAN_POINT('Ctrl Pts',(18.0716206740858,18.1013375041683,38.1619487263116));
#48088=CARTESIAN_POINT('Ctrl Pts',(18.0730939131179,18.1033596734284,38.1926039374795));
#48089=CARTESIAN_POINT('Ctrl Pts',(18.0763419964673,18.1078179956423,38.2601901735182));
#48090=CARTESIAN_POINT('Ctrl Pts',(18.0831566834011,18.1122763178562,38.3277388219117));
#48091=CARTESIAN_POINT('Ctrl Pts',(18.0935346887358,18.1167346400701,38.394843303886));
#48092=CARTESIAN_POINT('Ctrl Pts',(18.1044314108777,18.1214157995817,38.4653018237035));
#48093=CARTESIAN_POINT('Ctrl Pts',(18.1192570644502,18.1260969590932,38.5352700676509));
#48094=CARTESIAN_POINT('Ctrl Pts',(18.137945881509,18.1307781186048,38.6042787093571));
#48095=CARTESIAN_POINT('Ctrl Pts',(18.1556967837643,18.1352243499884,38.669824091381));
#48096=CARTESIAN_POINT('Ctrl Pts',(18.1769322927136,18.1396705813721,38.7345033216825));
#48097=CARTESIAN_POINT('Ctrl Pts',(18.2015434544663,18.1441168127558,38.7979230693471));
#48098=CARTESIAN_POINT('Ctrl Pts',(18.2261397598962,18.148560360209,38.8613045342093));
#48099=CARTESIAN_POINT('Ctrl Pts',(18.2541074979079,18.1530039076621,38.923427565825));
#48100=CARTESIAN_POINT('Ctrl Pts',(18.2852883467481,18.1574474551153,38.9839154388866));
#48101=CARTESIAN_POINT('Ctrl Pts',(18.3164611195515,18.1618898516615,39.044387645207));
#48102=CARTESIAN_POINT('Ctrl Pts',(18.3508451250287,18.1663322482078,39.1032250956793));
#48103=CARTESIAN_POINT('Ctrl Pts',(18.3882353091368,18.1707746447541,39.1600741191948));
#48104=CARTESIAN_POINT('Ctrl Pts',(18.4256286944911,18.1752174216464,39.2169280099697));
#48105=CARTESIAN_POINT('Ctrl Pts',(18.4660284961405,18.1796601985386,39.2717927253538));
#48106=CARTESIAN_POINT('Ctrl Pts',(18.5091864227286,18.1841029754308,39.3243436750861));
#48107=CARTESIAN_POINT('Ctrl Pts',(18.5523908687846,18.1885505411448,39.3769512689255));
#48108=CARTESIAN_POINT('Ctrl Pts',(18.5983590580795,18.1929981068588,39.4272397392126));
#48109=CARTESIAN_POINT('Ctrl Pts',(18.6468031794314,18.1974456725728,39.4749185145684));
#48110=CARTESIAN_POINT('Ctrl Pts',(18.6952775897809,18.2018960190639,39.5226271004001));
#48111=CARTESIAN_POINT('Ctrl Pts',(18.7462306433898,18.2063463655551,39.5677224177369));
#48112=CARTESIAN_POINT('Ctrl Pts',(18.7993406385498,18.2107967120463,39.6099535273187));
#48113=CARTESIAN_POINT('Ctrl Pts',(18.85254045301,18.2152545849363,39.6522560578956));
#48114=CARTESIAN_POINT('Ctrl Pts',(18.9079040862449,18.2197124578263,39.6916844300659));
#48115=CARTESIAN_POINT('Ctrl Pts',(18.9650808375466,18.2241703307163,39.7280309837613));
#48116=CARTESIAN_POINT('Ctrl Pts',(18.9860818903373,18.2258077099267,39.7413810932995));
#48117=CARTESIAN_POINT('Ctrl Pts',(19.0073273168203,18.2274450891371,39.7543158869174));
#48118=CARTESIAN_POINT('Ctrl Pts',(19.0287989942023,18.2290824683474,39.7668266746238));
#48119=CARTESIAN_POINT('Ctrl Pts',(19.0872629441823,18.2335407905619,39.800891552447));
#48120=CARTESIAN_POINT('Ctrl Pts',(19.1476367921603,18.2379991127763,39.8319440618328));
#48121=CARTESIAN_POINT('Ctrl Pts',(19.2095776841387,18.2424574349907,39.8597656433424));
#48122=CARTESIAN_POINT('Ctrl Pts',(19.2746145257327,18.2471385945022,39.8889778121011));
#48123=CARTESIAN_POINT('Ctrl Pts',(19.3413787477654,18.2518197540137,39.9146272530517));
#48124=CARTESIAN_POINT('Ctrl Pts',(19.4094408477271,18.2565009135252,39.9365136657718));
#48125=CARTESIAN_POINT('Ctrl Pts',(19.4740871910489,18.2609471449094,39.9573016895264));
#48126=CARTESIAN_POINT('Ctrl Pts',(19.539903742999,18.2653933762936,39.9746951125107));
#48127=CARTESIAN_POINT('Ctrl Pts',(19.6065012435478,18.2698396076778,39.9885712286198));
#48128=CARTESIAN_POINT('Ctrl Pts',(19.67305854307,18.2742831551314,40.0024389685271));
#48129=CARTESIAN_POINT('Ctrl Pts',(19.7403953742742,18.2787267025851,40.0127935129869));
#48130=CARTESIAN_POINT('Ctrl Pts',(19.8081095343543,18.2831702500388,40.0195626080163));
#48131=CARTESIAN_POINT('Ctrl Pts',(19.8758061560391,18.2876126465856,40.0263299498073));
#48132=CARTESIAN_POINT('Ctrl Pts',(19.9438794220707,18.2920550431324,40.0295136368982));
#48133=CARTESIAN_POINT('Ctrl Pts',(20.0119210310178,18.2964974396792,40.0290931667287));
#48134=CARTESIAN_POINT('Ctrl Pts',(20.079968465503,18.3009402165719,40.0286726605597));
#48135=CARTESIAN_POINT('Ctrl Pts',(20.1479837444357,18.3053829934647,40.0246473903624));
#48136=CARTESIAN_POINT('Ctrl Pts',(20.2155594257593,18.3098257703574,40.0170489536958));
#48137=CARTESIAN_POINT('Ctrl Pts',(20.2832079461876,18.3142733360719,40.0094423267556));
#48138=CARTESIAN_POINT('Ctrl Pts',(20.3504154326781,18.3187209017864,39.9982549038406));
#48139=CARTESIAN_POINT('Ctrl Pts',(20.4167814684665,18.3231684675009,39.9835699520971));
#48140=CARTESIAN_POINT('Ctrl Pts',(20.4831889986744,18.3276188139925,39.9688758187964));
#48141=CARTESIAN_POINT('Ctrl Pts',(20.5487535562374,18.3320691604842,39.9506799371097));
#48142=CARTESIAN_POINT('Ctrl Pts',(20.6130895226733,18.3365195069758,39.9291155770176));
#48143=CARTESIAN_POINT('Ctrl Pts',(20.6775342937034,18.3409773798663,39.9075147474111));
#48144=CARTESIAN_POINT('Ctrl Pts',(20.7407458698446,18.3454352527569,39.8825342538263));
#48145=CARTESIAN_POINT('Ctrl Pts',(20.8023591529402,18.3498931256474,39.8543552509663));
#48146=CARTESIAN_POINT('Ctrl Pts',(20.8249897462869,18.3515305048537,39.8440050874528));
#48147=CARTESIAN_POINT('Ctrl Pts',(20.8474049658539,18.3531678840601,39.8332238555599));
#48148=CARTESIAN_POINT('Ctrl Pts',(20.8695876570089,18.3548052632665,39.8220220276401));
#48149=CARTESIAN_POINT('Ctrl Pts',(20.9299875841307,18.3592635854801,39.791521238297));
#48150=CARTESIAN_POINT('Ctrl Pts',(20.9889001583487,18.3637219076937,39.757778558256));
#48151=CARTESIAN_POINT('Ctrl Pts',(21.0459554096211,18.3681802299074,39.7209626269549));
#48152=CARTESIAN_POINT('Ctrl Pts',(21.1058624148533,18.372861389419,39.6823065499085));
#48153=CARTESIAN_POINT('Ctrl Pts',(21.1637210377508,18.3775425489306,39.6402621100675));
#48154=CARTESIAN_POINT('Ctrl Pts',(21.2191294593047,18.3822237084422,39.5950805725296));
#48155=CARTESIAN_POINT('Ctrl Pts',(21.2717571602427,18.3866699398256,39.5521665103929));
#48156=CARTESIAN_POINT('Ctrl Pts',(21.3221742267561,18.391116171209,39.5064229963557));
#48157=CARTESIAN_POINT('Ctrl Pts',(21.3700658366063,18.3955624025924,39.4581097747474));
#48158=CARTESIAN_POINT('Ctrl Pts',(21.4179285370851,18.4000059500453,39.4098257170128));
#48159=CARTESIAN_POINT('Ctrl Pts',(21.4632684585658,18.4044494974982,39.3589753783089));
#48160=CARTESIAN_POINT('Ctrl Pts',(21.5058060562462,18.4088930449511,39.305856823123));
#48161=CARTESIAN_POINT('Ctrl Pts',(21.5483326364202,18.4133354414971,39.2527520259784));
#48162=CARTESIAN_POINT('Ctrl Pts',(21.5880580257213,18.4177778380432,39.1973805635166));
#48163=CARTESIAN_POINT('Ctrl Pts',(21.6247427722402,18.4222202345892,39.1400737863023));
#48164=CARTESIAN_POINT('Ctrl Pts',(21.6614306596078,18.4266630114812,39.082762102637));
#48165=CARTESIAN_POINT('Ctrl Pts',(21.6950771238612,18.4311057883732,39.0235151920824));
#48166=CARTESIAN_POINT('Ctrl Pts',(21.7254868859807,18.4355485652652,38.9626920442479));
#48167=CARTESIAN_POINT('Ctrl Pts',(21.7559294264579,18.4399961309789,38.901803335792));
#48168=CARTESIAN_POINT('Ctrl Pts',(21.7831280828116,18.4444436966927,38.8393354419349));
#48169=CARTESIAN_POINT('Ctrl Pts',(21.8069347440799,18.4488912624064,38.7756695845877));
#48170=CARTESIAN_POINT('Ctrl Pts',(21.8307562901244,18.4533416088974,38.711963921069));
#48171=CARTESIAN_POINT('Ctrl Pts',(21.8511814729861,18.4577919553883,38.6470592739138));
#48172=CARTESIAN_POINT('Ctrl Pts',(21.8681121826909,18.4622423018792,38.5813516695534));
#48173=CARTESIAN_POINT('Ctrl Pts',(21.8850715255088,18.466700174769,38.5155329408929));
#48174=CARTESIAN_POINT('Ctrl Pts',(21.8985245059642,18.4711580476588,38.4489090282691));
#48175=CARTESIAN_POINT('Ctrl Pts',(21.9084243529671,18.4756159205486,38.3818848096334));
#48176=CARTESIAN_POINT('Ctrl Pts',(21.912060572323,18.4772532997609,38.3572667765423));
#48177=CARTESIAN_POINT('Ctrl Pts',(21.9152179467829,18.4788906789733,38.3325947676987));
#48178=CARTESIAN_POINT('Ctrl Pts',(21.9178959233884,18.4805280581856,38.3078888740416));
#48179=CARTESIAN_POINT('Ctrl Pts',(21.9251876261883,18.484986380399,38.2406186695197));
#48180=CARTESIAN_POINT('Ctrl Pts',(21.9289501929268,18.4894447026124,38.1728314808468));
#48181=CARTESIAN_POINT('Ctrl Pts',(21.9291237019229,18.4939030248258,38.1049294603374));
#48182=CARTESIAN_POINT('Ctrl Pts',(21.9293058833016,18.4985841843374,38.0336335391473));
#48183=CARTESIAN_POINT('Ctrl Pts',(21.9255306696707,18.503265343849,37.9622115332449));
#48184=CARTESIAN_POINT('Ctrl Pts',(21.9177901148132,18.5079465033606,37.8911372880935));
#48185=CARTESIAN_POINT('Ctrl Pts',(21.9104380265441,18.5123927347438,37.8236299667682));
#48186=CARTESIAN_POINT('Ctrl Pts',(21.8995090759222,18.5168389661269,37.7564369038082));
#48187=CARTESIAN_POINT('Ctrl Pts',(21.8850497851158,18.5212851975101,37.6899635814528));
#48188=CARTESIAN_POINT('Ctrl Pts',(21.8705992225398,18.5257287449627,37.6235303851648));
#48189=CARTESIAN_POINT('Ctrl Pts',(21.8526226517929,18.5301722924153,37.557816548496));
#48190=CARTESIAN_POINT('Ctrl Pts',(21.8312179433442,18.5346158398679,37.493218819611));
#48191=CARTESIAN_POINT('Ctrl Pts',(21.8098187788502,18.5390582364137,37.428637821946));
#48192=CARTESIAN_POINT('Ctrl Pts',(21.7849933945691,18.5435006329594,37.3651728260429));
#48193=CARTESIAN_POINT('Ctrl Pts',(21.7568894075675,18.5479430295052,37.3032050662328));
#48194=CARTESIAN_POINT('Ctrl Pts',(21.7287830143787,18.5523858063969,37.2412320009111));
#48195=CARTESIAN_POINT('Ctrl Pts',(21.6973976674127,18.5568285832886,37.1807568741046));
#48196=CARTESIAN_POINT('Ctrl Pts',(21.6629282141081,18.5612713601803,37.1221389098531));
#48197=CARTESIAN_POINT('Ctrl Pts',(21.6284216065481,18.5657189258937,37.0634577619243));
#48198=CARTESIAN_POINT('Ctrl Pts',(21.5908245101539,18.5701664916071,37.0066381965217));
#48199=CARTESIAN_POINT('Ctrl Pts',(21.5503760975718,18.5746140573206,36.9520119717618));
#48200=CARTESIAN_POINT('Ctrl Pts',(21.5099023951951,18.5790644038112,36.8973515927322));
#48201=CARTESIAN_POINT('Ctrl Pts',(21.466574143152,18.5835147503018,36.8448876632989));
#48202=CARTESIAN_POINT('Ctrl Pts',(21.4206701504348,18.5879650967924,36.7949180559967));
#48203=CARTESIAN_POINT('Ctrl Pts',(21.3746885251648,18.5924229696819,36.744863940399));
#48204=CARTESIAN_POINT('Ctrl Pts',(21.3261228195484,18.5968808425714,36.6973129082982));
#48205=CARTESIAN_POINT('Ctrl Pts',(21.27528721341,18.6013387154609,36.6525245839003));
#48206=CARTESIAN_POINT('Ctrl Pts',(21.2566152667401,18.6029760946755,36.6360738072082));
#48207=CARTESIAN_POINT('Ctrl Pts',(21.2376373892696,18.6046134738901,36.6199953370601));
#48208=CARTESIAN_POINT('Ctrl Pts',(21.2183701336408,18.6062508531047,36.6043005735269));
#48209=CARTESIAN_POINT('Ctrl Pts',(21.1659084723098,18.6107091753216,36.5615662378739));
#48210=CARTESIAN_POINT('Ctrl Pts',(21.1110920955775,18.6151674975385,36.521510967239));
#48211=CARTESIAN_POINT('Ctrl Pts',(21.0542257384865,18.6196258197553,36.4844039337716));
#48212=CARTESIAN_POINT('Ctrl Pts',(20.9945170688538,18.6243069792665,36.4454422046282));
#48213=CARTESIAN_POINT('Ctrl Pts',(20.9325484801317,18.6289881387777,36.409731573502));
#48214=CARTESIAN_POINT('Ctrl Pts',(20.8687131405122,18.6336692982889,36.3775366371381));
#48215=CARTESIAN_POINT('Ctrl Pts',(20.808081433792,18.6381155296755,36.3469574320908));
#48216=CARTESIAN_POINT('Ctrl Pts',(20.7457663349597,18.6425617610622,36.3195498029366));
#48217=CARTESIAN_POINT('Ctrl Pts',(20.6821333135934,18.6470079924488,36.2954954421265));
#48218=CARTESIAN_POINT('Ctrl Pts',(20.6185387037704,18.6514515399049,36.271455601531));
#48219=CARTESIAN_POINT('Ctrl Pts',(20.5536282098857,18.655895087361,36.2507651879098));
#48220=CARTESIAN_POINT('Ctrl Pts',(20.4877879254899,18.6603386348171,36.2335580650215));
#48221=CARTESIAN_POINT('Ctrl Pts',(20.4219646941437,18.6647810313663,36.2163553988867));
#48222=CARTESIAN_POINT('Ctrl Pts',(20.355212627337,18.6692234279155,36.2026343568969));
#48223=CARTESIAN_POINT('Ctrl Pts',(20.2879318834082,18.6736658244648,36.1924786272712));
#48224=CARTESIAN_POINT('Ctrl Pts',(20.2206453790846,18.6781086013599,36.1823220281396));
#48225=CARTESIAN_POINT('Ctrl Pts',(20.1528305957856,18.6825513782551,36.1757314182156));
#48226=CARTESIAN_POINT('Ctrl Pts',(20.0848949372993,18.6869941551503,36.1727388847069));
#48227=CARTESIAN_POINT('Ctrl Pts',(20.0168860516933,18.6914417208671,36.1697431255783));
#48228=CARTESIAN_POINT('Ctrl Pts',(19.9487565244515,18.695889286584,36.1703532028808));
#48229=CARTESIAN_POINT('Ctrl Pts',(19.8809148468747,18.7003368523008,36.1745490701643));
#48230=CARTESIAN_POINT('Ctrl Pts',(19.8130307522546,18.7047871987949,36.1787475608541));
#48231=CARTESIAN_POINT('Ctrl Pts',(19.7454353552026,18.7092375452889,36.186536246299));
#48232=CARTESIAN_POINT('Ctrl Pts',(19.6785302969749,18.7136878917829,36.1978433852764));
#48233=CARTESIAN_POINT('Ctrl Pts',(19.6115120893214,18.7181457646757,36.2091696468181));
#48234=CARTESIAN_POINT('Ctrl Pts',(19.5451870305379,18.7226036375686,36.2240261268957));
#48235=CARTESIAN_POINT('Ctrl Pts',(19.4799439301978,18.7270615104614,36.2422905929177));
#48236=CARTESIAN_POINT('Ctrl Pts',(19.455980103236,18.7286988896488,36.2489991414236));
#48237=CARTESIAN_POINT('Ctrl Pts',(19.4321620631573,18.7303362688363,36.2561669850272));
#48238=CARTESIAN_POINT('Ctrl Pts',(19.4085083833019,18.7319736480237,36.2637864437175));
#48239=CARTESIAN_POINT('Ctrl Pts',(19.4037014960229,18.7323063952849,36.2653348657505));
#48240=CARTESIAN_POINT('Ctrl Pts',(19.398899982941,18.732639142546,36.2669023907506));
#48241=CARTESIAN_POINT('Ctrl Pts',(19.3941040087494,18.7329718898071,36.2684889831927));
#48242=CARTESIAN_POINT('Origin',(20.,-1.3495818343519,38.1));
#48243=CARTESIAN_POINT('',(19.3941041453487,19.6985952145508,36.2684889380033));
#48244=CARTESIAN_POINT('',(19.3941040005193,19.5258959448669,36.2684889859154));
#48245=CARTESIAN_POINT('',(19.3941040087494,-1.3495818343519,36.2684889831927));
#48246=CARTESIAN_POINT('Ctrl Pts',(19.3941041453486,19.6985952145508,36.2684889380033));
#48247=CARTESIAN_POINT('Ctrl Pts',(19.4450720666877,19.6953436865102,36.2516278592469));
#48248=CARTESIAN_POINT('Ctrl Pts',(19.4967669479744,19.6920519773128,36.2368866026938));
#48249=CARTESIAN_POINT('Ctrl Pts',(19.5872481096025,19.6862432079621,36.2151336500013));
#48250=CARTESIAN_POINT('Ctrl Pts',(19.6257066615318,19.6837600036393,36.2071213884289));
#48251=CARTESIAN_POINT('Ctrl Pts',(19.6755084276242,19.6805144398755,36.1983229870329));
#48252=CARTESIAN_POINT('Ctrl Pts',(19.6866527598072,19.6797862746826,36.1964549544536));
#48253=CARTESIAN_POINT('Ctrl Pts',(19.7047208584644,19.6786023867189,36.1935893126101));
#48254=CARTESIAN_POINT('Ctrl Pts',(19.711634877699,19.6781485689502,36.1925312493969));
#48255=CARTESIAN_POINT('Ctrl Pts',(19.7248907374021,19.6772769191734,36.1905764030618));
#48256=CARTESIAN_POINT('Ctrl Pts',(19.7312316006745,19.676859283731,36.189673555441));
#48257=CARTESIAN_POINT('Ctrl Pts',(19.7456939561376,19.6759051143159,36.1876877546404));
#48258=CARTESIAN_POINT('Ctrl Pts',(19.7538180439075,19.6753679570666,36.1866249377858));
#48259=CARTESIAN_POINT('Ctrl Pts',(19.7752910791765,19.6739449970673,36.1839547934479));
#48260=CARTESIAN_POINT('Ctrl Pts',(19.7886502929527,19.6730564728975,36.1824352374703));
#48261=CARTESIAN_POINT('Ctrl Pts',(19.8909905440559,19.6662238034002,36.1718768750724));
#48262=CARTESIAN_POINT('Ctrl Pts',(19.9804742634496,19.6600915429246,36.1688976224292));
#48263=CARTESIAN_POINT('Ctrl Pts',(20.2316577276156,19.642461665015,36.1779959611759));
#48264=CARTESIAN_POINT('Ctrl Pts',(20.3920906973116,19.6306669272838,36.2042082385043));
#48265=CARTESIAN_POINT('Ctrl Pts',(20.5763214509395,19.6174190056741,36.2587209840939));
#48266=CARTESIAN_POINT('Ctrl Pts',(20.6050808027085,19.6153622280458,36.2679704417416));
#48267=CARTESIAN_POINT('Ctrl Pts',(20.6402685646424,19.6128694846665,36.2802065019418));
#48268=CARTESIAN_POINT('Ctrl Pts',(20.6469115693081,19.6123999458869,36.2825573913535));
#48269=CARTESIAN_POINT('Ctrl Pts',(20.6573602689549,19.6116632518081,36.2863196241069));
#48270=CARTESIAN_POINT('Ctrl Pts',(20.6611745644145,19.6113947093778,36.2877066393029));
#48271=CARTESIAN_POINT('Ctrl Pts',(20.6683378568902,19.6108911508514,36.2903370956704));
#48272=CARTESIAN_POINT('Ctrl Pts',(20.671687738482,19.6106559852612,36.2915777869976));
#48273=CARTESIAN_POINT('Ctrl Pts',(20.6793295390427,19.6101202319867,36.2944322338715));
#48274=CARTESIAN_POINT('Ctrl Pts',(20.6836191611811,19.6098200032003,36.2960519895978));
#48275=CARTESIAN_POINT('Ctrl Pts',(20.69498156031,19.6090260028816,36.3003887662237));
#48276=CARTESIAN_POINT('Ctrl Pts',(20.7020442616477,19.6085337513689,36.3031322193441));
#48277=CARTESIAN_POINT('Ctrl Pts',(20.7516096732668,19.6050870164219,36.3227223834682));
#48278=CARTESIAN_POINT('Ctrl Pts',(20.7935217398094,19.6022130868392,36.3410352917277));
#48279=CARTESIAN_POINT('Ctrl Pts',(20.8709346850246,19.596910671452,36.3781909061901));
#48280=CARTESIAN_POINT('Ctrl Pts',(20.9065731311006,19.5944719941572,36.3966858093375));
#48281=CARTESIAN_POINT('Ctrl Pts',(21.0353392133235,19.585579747793,36.4686974476995));
#48282=CARTESIAN_POINT('Ctrl Pts',(21.1245271061465,19.579249798928,36.5288493356327));
#48283=CARTESIAN_POINT('Ctrl Pts',(21.2699502421611,19.5679478801657,36.6456844163888));
#48284=CARTESIAN_POINT('Ctrl Pts',(21.3285378578071,19.563070066982,36.6990030662686));
#48285=CARTESIAN_POINT('Ctrl Pts',(21.3970638577969,19.5568191566934,36.7695399359665));
#48286=CARTESIAN_POINT('Ctrl Pts',(21.4102395078475,19.5555900523645,36.7835138082815));
#48287=CARTESIAN_POINT('Ctrl Pts',(21.4290154720382,19.55379715977,36.8040326216604));
#48288=CARTESIAN_POINT('Ctrl Pts',(21.4347843222286,19.5532404707329,36.8104223133957));
#48289=CARTESIAN_POINT('Ctrl Pts',(21.444797592595,19.5522638104782,36.8216635720516));
#48290=CARTESIAN_POINT('Ctrl Pts',(21.4490608538908,19.5518446309552,36.8264982345394));
#48291=CARTESIAN_POINT('Ctrl Pts',(21.4572751243033,19.5510303845625,36.8359081080643));
#48292=CARTESIAN_POINT('Ctrl Pts',(21.461229020697,19.5506354435315,36.8404807080284));
#48293=CARTESIAN_POINT('Ctrl Pts',(21.4706059137799,19.5496915613067,36.851428474423));
#48294=CARTESIAN_POINT('Ctrl Pts',(21.4760090049088,19.5491418173647,36.8578204550754));
#48295=CARTESIAN_POINT('Ctrl Pts',(21.4952462139623,19.5471631334401,36.8808812418922));
#48296=CARTESIAN_POINT('Ctrl Pts',(21.5088405160797,19.5457246306201,36.8977471068365));
#48297=CARTESIAN_POINT('Ctrl Pts',(21.6168046330804,19.5339626365527,37.0364093936724));
#48298=CARTESIAN_POINT('Ctrl Pts',(21.6965386268226,19.5230580575429,37.1688606242217));
#48299=CARTESIAN_POINT('Ctrl Pts',(21.7926845956981,19.506318879313,37.382841529062));
#48300=CARTESIAN_POINT('Ctrl Pts',(21.8210722022559,19.5005761306837,37.4583365240643));
#48301=CARTESIAN_POINT('Ctrl Pts',(21.8550280454731,19.4925391297536,37.5692747715017));
#48302=CARTESIAN_POINT('Ctrl Pts',(21.8644647222796,19.4901173817071,37.6034418380367));
#48303=CARTESIAN_POINT('Ctrl Pts',(21.8747269826856,19.4872489673208,37.6450318842951));
#48304=CARTESIAN_POINT('Ctrl Pts',(21.8764573343121,19.4867559189422,37.6522220161931));
#48305=CARTESIAN_POINT('Ctrl Pts',(21.8790907223582,19.4859907450418,37.663447925789));
#48306=CARTESIAN_POINT('Ctrl Pts',(21.8800221786886,19.4857170521077,37.6674768621368));
#48307=CARTESIAN_POINT('Ctrl Pts',(21.8817315189482,19.4852090882355,37.6749803247635));
#48308=CARTESIAN_POINT('Ctrl Pts',(21.8825127314461,19.4849746367145,37.6784539764126));
#48309=CARTESIAN_POINT('Ctrl Pts',(21.8842691623348,19.4844421938637,37.6863661865534));
#48310=CARTESIAN_POINT('Ctrl Pts',(21.8852383156825,19.4841445491747,37.6908060339177));
#48311=CARTESIAN_POINT('Ctrl Pts',(21.8881558937132,19.4832363995607,37.7044023340271));
#48312=CARTESIAN_POINT('Ctrl Pts',(21.8900534014347,19.4826286981317,37.7135697468165));
#48313=CARTESIAN_POINT('Ctrl Pts',(21.9084459662552,19.4765574017428,37.8058074632603));
#48314=CARTESIAN_POINT('Ctrl Pts',(21.9195226661703,19.4713724424426,37.8898764808825));
#48315=CARTESIAN_POINT('Ctrl Pts',(21.9320124983956,19.4598106414727,38.0813224927145));
#48316=CARTESIAN_POINT('Ctrl Pts',(21.9300690586937,19.4534950127833,38.188627698923));
#48317=CARTESIAN_POINT('Ctrl Pts',(21.9112254697708,19.4422127118766,38.373883479013));
#48318=CARTESIAN_POINT('Ctrl Pts',(21.8983957625082,19.43733954541,38.4519748630206));
#48319=CARTESIAN_POINT('Ctrl Pts',(21.8765434173371,19.4310942230102,38.5477675947507));
#48320=CARTESIAN_POINT('Ctrl Pts',(21.8719952854018,19.4298657574009,38.566416793531));
#48321=CARTESIAN_POINT('Ctrl Pts',(21.8650059611557,19.4280736291312,38.593324840563));
#48322=CARTESIAN_POINT('Ctrl Pts',(21.8627864732165,19.4275170571197,38.6016404935037));
#48323=CARTESIAN_POINT('Ctrl Pts',(21.8588076293095,19.4265405331711,38.6161572434294));
#48324=CARTESIAN_POINT('Ctrl Pts',(21.8570726889956,19.4261213722608,38.6223649383649));
#48325=CARTESIAN_POINT('Ctrl Pts',(21.8536502720967,19.4253071112306,38.6343779317725));
#48326=CARTESIAN_POINT('Ctrl Pts',(21.8519665501002,19.4249121367109,38.6401842288741));
#48327=CARTESIAN_POINT('Ctrl Pts',(21.8478862505894,19.423968092992,38.6540117736719));
#48328=CARTESIAN_POINT('Ctrl Pts',(21.8454647133025,19.4234182204107,38.6620254698071));
#48329=CARTESIAN_POINT('Ctrl Pts',(21.8365868932361,19.4214386019765,38.6907291226157));
#48330=CARTESIAN_POINT('Ctrl Pts',(21.8298343990209,19.4199992814802,38.711325052741));
#48331=CARTESIAN_POINT('Ctrl Pts',(21.7723371871785,19.4082489441412,38.8772033569532));
#48332=CARTESIAN_POINT('Ctrl Pts',(21.7047302169484,19.3973584360644,39.01602443409));
#48333=CARTESIAN_POINT('Ctrl Pts',(21.5776462431174,19.3806230929494,39.2131433939542));
#48334=CARTESIAN_POINT('Ctrl Pts',(21.5296992873417,19.374870503537,39.2781670624535));
#48335=CARTESIAN_POINT('Ctrl Pts',(21.4550176825506,19.3668216735174,39.3671717560366));
#48336=CARTESIAN_POINT('Ctrl Pts',(21.4314711366642,19.3643975594919,39.3937122914088));
#48337=CARTESIAN_POINT('Ctrl Pts',(21.4021443421209,19.3615267309661,39.424986233868));
#48338=CARTESIAN_POINT('Ctrl Pts',(21.3970532826923,19.3610335450384,39.4303531131852));
#48339=CARTESIAN_POINT('Ctrl Pts',(21.3890679805113,19.3602682051111,39.4386746451258));
#48340=CARTESIAN_POINT('Ctrl Pts',(21.3861949617295,19.3599944826119,39.4416494284491));
#48341=CARTESIAN_POINT('Ctrl Pts',(21.3808307476517,19.3594864927861,39.447168022063));
#48342=CARTESIAN_POINT('Ctrl Pts',(21.3783421001483,19.3592520446986,39.4497141507026));
#48343=CARTESIAN_POINT('Ctrl Pts',(21.372661390296,19.3587196468601,39.4554939725149));
#48344=CARTESIAN_POINT('Ctrl Pts',(21.3694649483432,19.3584220435173,39.4587232824368));
#48345=CARTESIAN_POINT('Ctrl Pts',(21.3596503603843,19.3575141451976,39.4685689712746));
#48346=CARTESIAN_POINT('Ctrl Pts',(21.3529953345434,19.3569066514613,39.4751486337439));
#48347=CARTESIAN_POINT('Ctrl Pts',(21.2859861874224,19.3508672100184,39.5404415593539));
#48348=CARTESIAN_POINT('Ctrl Pts',(21.2218887321146,19.3457106441534,39.5952003657285));
#48349=CARTESIAN_POINT('Ctrl Pts',(21.068282226226,19.3341543407665,39.7099290911365));
#48350=CARTESIAN_POINT('Ctrl Pts',(20.9769295745816,19.3278182468496,39.7669455683943));
#48351=CARTESIAN_POINT('Ctrl Pts',(20.8108627474162,19.3165078459909,39.8522313143818));
#48352=CARTESIAN_POINT('Ctrl Pts',(20.7382700510883,19.3116279718792,39.8840314227108));
#48353=CARTESIAN_POINT('Ctrl Pts',(20.6458981760785,19.3053745840151,39.9178908445439));
#48354=CARTESIAN_POINT('Ctrl Pts',(20.6277646190432,19.3041451975773,39.9242321993967));
#48355=CARTESIAN_POINT('Ctrl Pts',(20.6013715413927,19.3023519680904,39.9330218078398));
#48356=CARTESIAN_POINT('Ctrl Pts',(20.5931851812922,19.3017952280787,39.9356873414509));
#48357=CARTESIAN_POINT('Ctrl Pts',(20.5788388433847,19.3008185091516,39.9402526189426));
#48358=CARTESIAN_POINT('Ctrl Pts',(20.5726866306861,19.3003993222265,39.9421764653505));
#48359=CARTESIAN_POINT('Ctrl Pts',(20.5607466989577,19.2995850840942,39.9458445860728));
#48360=CARTESIAN_POINT('Ctrl Pts',(20.5549601892242,19.2991901588316,39.9475925642055));
#48361=CARTESIAN_POINT('Ctrl Pts',(20.5411430862195,19.2982463505971,39.951695642823));
#48362=CARTESIAN_POINT('Ctrl Pts',(20.5331052493393,19.2976966651614,39.9540257233425));
#48363=CARTESIAN_POINT('Ctrl Pts',(20.5042138946991,19.2957184017191,39.9621975993413));
#48364=CARTESIAN_POINT('Ctrl Pts',(20.4832781574332,19.2942802661506,39.9677402679551));
#48365=CARTESIAN_POINT('Ctrl Pts',(20.3125840944265,19.2825130422236,40.0098689605594));
#48366=CARTESIAN_POINT('Ctrl Pts',(20.1590536403926,19.2716021474951,40.0287280325526));
#48367=CARTESIAN_POINT('Ctrl Pts',(19.9244406995905,19.2548612125593,40.0293303338055));
#48368=CARTESIAN_POINT('Ctrl Pts',(19.8439897192502,19.2491228451965,40.0244966058679));
#48369=CARTESIAN_POINT('Ctrl Pts',(19.7289161547196,19.2410911133007,40.010316936358));
#48370=CARTESIAN_POINT('Ctrl Pts',(19.6938835775469,19.2386704205275,40.0050171587509));
#48371=CARTESIAN_POINT('Ctrl Pts',(19.651736395961,19.2358030840346,39.9974482059737));
#48372=CARTESIAN_POINT('Ctrl Pts',(19.6444659718951,19.2353100979693,39.9960993622347));
#48373=CARTESIAN_POINT('Ctrl Pts',(19.6331421769379,19.2345449997506,39.9939310949199));
#48374=CARTESIAN_POINT('Ctrl Pts',(19.6290834773675,19.2342713206704,39.993140403848));
#48375=CARTESIAN_POINT('Ctrl Pts',(19.6215347350776,19.2337633693316,39.9916445958848));
#48376=CARTESIAN_POINT('Ctrl Pts',(19.618044135358,19.2335289165715,39.990942873721));
#48377=CARTESIAN_POINT('Ctrl Pts',(19.6101024412371,19.2329964541702,39.9893234513936));
#48378=CARTESIAN_POINT('Ctrl Pts',(19.6056526410239,19.2326987912737,39.9883996854022));
#48379=CARTESIAN_POINT('Ctrl Pts',(19.5940861156019,19.2319267381675,39.9859558405408));
#48380=CARTESIAN_POINT('Ctrl Pts',(19.5869745731398,19.2314537003442,39.984411185184));
#48381=CARTESIAN_POINT('Ctrl Pts',(19.5408534729607,19.2283955848688,39.9741198616671));
#48382=CARTESIAN_POINT('Ctrl Pts',(19.502111895418,19.2258719484957,39.9642019090557));
#48383=CARTESIAN_POINT('Ctrl Pts',(19.4473033568271,19.2223301999119,39.9483399223784));
#48384=CARTESIAN_POINT('Ctrl Pts',(19.4309665588301,19.221278189424,39.9433759844735));
#48385=CARTESIAN_POINT('Ctrl Pts',(19.2923859472791,19.2123692471506,39.8992503289609));
#48386=CARTESIAN_POINT('Ctrl Pts',(19.1742620739815,19.2048545266816,39.8481932884131));
#48387=CARTESIAN_POINT('Ctrl Pts',(18.9866830634279,19.19189445825,39.7438296160297));
#48388=CARTESIAN_POINT('Ctrl Pts',(18.9141934864965,19.1865982271348,39.6968746206688));
#48389=CARTESIAN_POINT('Ctrl Pts',(18.8289971432027,19.1798438790131,39.6331988625736));
#48390=CARTESIAN_POINT('Ctrl Pts',(18.8130890398742,19.1785585489264,39.6209170809926));
#48391=CARTESIAN_POINT('Ctrl Pts',(18.7905211566732,19.1766985450429,39.6029239324556));
#48392=CARTESIAN_POINT('Ctrl Pts',(18.783703569337,19.1761317469183,39.5974119031835));
#48393=CARTESIAN_POINT('Ctrl Pts',(18.7719188923142,19.1751432978828,39.5877503945955));
#48394=CARTESIAN_POINT('Ctrl Pts',(18.7669346347629,19.1747224969671,39.583622002745));
#48395=CARTESIAN_POINT('Ctrl Pts',(18.7573671819744,19.1739093965603,39.5756158978629));
#48396=CARTESIAN_POINT('Ctrl Pts',(18.7527811220519,19.1735172431074,39.5717417122524));
#48397=CARTESIAN_POINT('Ctrl Pts',(18.7419671935788,19.172586791467,39.5625195389416));
#48398=CARTESIAN_POINT('Ctrl Pts',(18.7357552696216,19.1720477425517,39.557153115501));
#48399=CARTESIAN_POINT('Ctrl Pts',(18.7140065591769,19.1701441642938,39.5381208475781));
#48400=CARTESIAN_POINT('Ctrl Pts',(18.6986560307569,19.1687709899912,39.5242452455318));
#48401=CARTESIAN_POINT('Ctrl Pts',(18.5623517787118,19.1563029174824,39.3969940754952));
#48402=CARTESIAN_POINT('Ctrl Pts',(18.456282740426,19.1445218917116,39.2687345441868));
#48403=CARTESIAN_POINT('Ctrl Pts',(18.3348668565016,19.1282825548101,39.076073766007));
#48404=CARTESIAN_POINT('Ctrl Pts',(18.304350245548,19.1238751604866,39.0220418128906));
#48405=CARTESIAN_POINT('Ctrl Pts',(18.2571630108873,19.1165556478289,38.9281982465478));
#48406=CARTESIAN_POINT('Ctrl Pts',(18.2391269934606,19.1136014338433,38.8891261149081));
#48407=CARTESIAN_POINT('Ctrl Pts',(18.2193803784843,19.1101952269226,38.8422918423713));
#48408=CARTESIAN_POINT('Ctrl Pts',(18.2163931226765,19.1096747857568,38.8350849801464));
#48409=CARTESIAN_POINT('Ctrl Pts',(18.2118562782806,19.1088765341861,38.8239491839253));
#48410=CARTESIAN_POINT('Ctrl Pts',(18.2102757777372,19.1085969346908,38.8200330544664));
#48411=CARTESIAN_POINT('Ctrl Pts',(18.2073892744807,19.108083529655,38.8128127148643));
#48412=CARTESIAN_POINT('Ctrl Pts',(18.2060795479295,19.1078495088071,38.8095101068849));
#48413=CARTESIAN_POINT('Ctrl Pts',(18.2031572756354,19.1073249322055,38.8020814797013));
#48414=CARTESIAN_POINT('Ctrl Pts',(18.2015498172477,19.1070346810466,38.7979535237887));
#48415=CARTESIAN_POINT('Ctrl Pts',(18.1974747715305,19.1062944016079,38.7873812441126));
#48416=CARTESIAN_POINT('Ctrl Pts',(18.1950274905477,19.1058455483315,38.7809290841404));
#48417=CARTESIAN_POINT('Ctrl Pts',(18.1808481821289,19.1032186673913,38.7429322767487));
#48418=CARTESIAN_POINT('Ctrl Pts',(18.1699078159981,19.1010839772322,38.7110958829762));
#48419=CARTESIAN_POINT('Ctrl Pts',(18.1171494330601,19.0901038169597,38.5434139665161));
#48420=CARTESIAN_POINT('Ctrl Pts',(18.0896019951648,19.0818077924057,38.4035292550389));
#48421=CARTESIAN_POINT('Ctrl Pts',(18.0731693937776,19.0700277856654,38.2083869054541));
#48422=CARTESIAN_POINT('Ctrl Pts',(18.0708998576667,19.06677159649,38.154735945049));
#48423=CARTESIAN_POINT('Ctrl Pts',(18.0708405336757,19.0601259833274,38.047037329303));
#48424=CARTESIAN_POINT('Ctrl Pts',(18.0730802280306,19.0567388060469,37.9930390220168));
#48425=CARTESIAN_POINT('Ctrl Pts',(18.0786629930108,19.0524510066424,37.9262913183339));
#48426=CARTESIAN_POINT('Ctrl Pts',(18.0798736154291,19.0516172565417,37.9133847419403));
#48427=CARTESIAN_POINT('Ctrl Pts',(18.0819834858798,19.0502987050167,37.893092917687));
#48428=CARTESIAN_POINT('Ctrl Pts',(18.0827955512464,19.0498166249753,37.8856988374519));
#48429=CARTESIAN_POINT('Ctrl Pts',(18.0843063968132,19.0489621934366,37.8726386869787));
#48430=CARTESIAN_POINT('Ctrl Pts',(18.0849876070335,19.0485903956126,37.8669706422672));
#48431=CARTESIAN_POINT('Ctrl Pts',(18.086608664564,19.0477353202312,37.8539699089489));
#48432=CARTESIAN_POINT('Ctrl Pts',(18.0875655183115,19.0472515155099,37.8466394685128));
#48433=CARTESIAN_POINT('Ctrl Pts',(18.0903358956867,19.0459061103242,37.8263260881715));
#48434=CARTESIAN_POINT('Ctrl Pts',(18.0922396282903,19.045041698526,37.8133560551673));
#48435=CARTESIAN_POINT('Ctrl Pts',(18.104103395452,19.0399798686261,37.7378901712751));
#48436=CARTESIAN_POINT('Ctrl Pts',(18.1170005986991,19.0356908817312,37.6759019367349));
#48437=CARTESIAN_POINT('Ctrl Pts',(18.172561706311,19.0204299960564,37.4621586618875));
#48438=CARTESIAN_POINT('Ctrl Pts',(18.2307402348806,19.0090224172787,37.315091480492));
#48439=CARTESIAN_POINT('Ctrl Pts',(18.312548660812,18.9969778469887,37.1649972625554));
#48440=CARTESIAN_POINT('Ctrl Pts',(18.3190845663261,18.9960366179365,37.1532975870443));
#48441=CARTESIAN_POINT('Ctrl Pts',(18.3495360791105,18.9917485655328,37.1000972094078));
#48442=CARTESIAN_POINT('Ctrl Pts',(18.374872494873,18.9884470837344,37.0594240949823));
#48443=CARTESIAN_POINT('Ctrl Pts',(18.4059900989788,18.9847179830776,37.0133842865465));
#48444=CARTESIAN_POINT('Ctrl Pts',(18.4103188832894,18.9842060189076,37.0070611978567));
#48445=CARTESIAN_POINT('Ctrl Pts',(18.4173124014179,18.9833898970632,36.996975168647));
#48446=CARTESIAN_POINT('Ctrl Pts',(18.4199530945883,18.9830842010024,36.9931957756318));
#48447=CARTESIAN_POINT('Ctrl Pts',(18.4246656173793,18.9825430683793,36.9865023920771));
#48448=CARTESIAN_POINT('Ctrl Pts',(18.4267320273631,18.9823072720096,36.9835846530051));
#48449=CARTESIAN_POINT('Ctrl Pts',(18.4311525889381,18.9818060150649,36.9773795362099));
#48450=CARTESIAN_POINT('Ctrl Pts',(18.4335089636096,18.9815407094704,36.9740938144905));
#48451=CARTESIAN_POINT('Ctrl Pts',(18.4399596391441,18.9808194771465,36.9651584647831));
#48452=CARTESIAN_POINT('Ctrl Pts',(18.4440743366094,18.9803649202693,36.9595235332574));
#48453=CARTESIAN_POINT('Ctrl Pts',(18.4656100668299,18.9780134668609,36.9303646087596));
#48454=CARTESIAN_POINT('Ctrl Pts',(18.48353537507,18.9761491388541,36.9072155758794));
#48455=CARTESIAN_POINT('Ctrl Pts',(18.5390689781861,18.9706144781517,36.8387753298248));
#48456=CARTESIAN_POINT('Ctrl Pts',(18.5782316603997,18.9670255381835,36.794786225617));
#48457=CARTESIAN_POINT('Ctrl Pts',(18.6876666813502,18.9575806870015,36.6826459768143));
#48458=CARTESIAN_POINT('Ctrl Pts',(18.7612115035457,18.9518042810597,36.6179356887756));
#48459=CARTESIAN_POINT('Ctrl Pts',(18.9154896320085,18.9401489516138,36.5017301011671));
#48460=CARTESIAN_POINT('Ctrl Pts',(18.9957678457011,18.9342918513032,36.4501080202648));
#48461=CARTESIAN_POINT('Ctrl Pts',(19.0914669957831,18.9273381220598,36.3981495400453));
#48462=CARTESIAN_POINT('Ctrl Pts',(19.1034769382696,18.9264661251862,36.3917922865043));
#48463=CARTESIAN_POINT('Ctrl Pts',(19.1228718226222,18.9250585174983,36.3817868171329));
#48464=CARTESIAN_POINT('Ctrl Pts',(19.1302148555712,18.9245257211837,36.3780580206053));
#48465=CARTESIAN_POINT('Ctrl Pts',(19.1433160567111,18.9235752535755,36.3715104056125));
#48466=CARTESIAN_POINT('Ctrl Pts',(19.1490648589008,18.9231582331296,36.3686730405306));
#48467=CARTESIAN_POINT('Ctrl Pts',(19.1610966907538,18.9222854787511,36.3628090401666));
#48468=CARTESIAN_POINT('Ctrl Pts',(19.1673821932796,18.9218295688681,36.3597877201389));
#48469=CARTESIAN_POINT('Ctrl Pts',(19.1838104083296,18.9206379537884,36.3520003729702));
#48470=CARTESIAN_POINT('Ctrl Pts',(19.1939783953937,18.9199004031342,36.3472885834794));
#48471=CARTESIAN_POINT('Ctrl Pts',(19.23912257793,18.9166252632111,36.326844924855));
#48472=CARTESIAN_POINT('Ctrl Pts',(19.2745201939101,18.9140555587858,36.3120704521873));
#48473=CARTESIAN_POINT('Ctrl Pts',(19.3380287010232,18.9094386430806,36.2877593874139));
#48474=CARTESIAN_POINT('Ctrl Pts',(19.3659600201675,18.9074060049298,36.2777995081405));
#48475=CARTESIAN_POINT('Ctrl Pts',(19.3941040358239,18.9053562004634,36.268488974236));
#48476=CARTESIAN_POINT('',(18.0708707698807,18.8910431656481,38.0982765153061));
#48477=CARTESIAN_POINT('Ctrl Pts',(19.3941040087494,18.7329718898071,36.2684889831927));
#48478=CARTESIAN_POINT('Ctrl Pts',(19.3298530882588,18.7374296531232,36.2897443154305));
#48479=CARTESIAN_POINT('Ctrl Pts',(19.2665971548675,18.7418874164393,36.3144260076521));
#48480=CARTESIAN_POINT('Ctrl Pts',(19.2047269033099,18.7463451797554,36.3424211942047));
#48481=CARTESIAN_POINT('Ctrl Pts',(19.1403324023001,18.7509848157215,36.3715585586625));
#48482=CARTESIAN_POINT('Ctrl Pts',(19.0774396255052,18.7556244516877,36.4042855416477));
#48483=CARTESIAN_POINT('Ctrl Pts',(19.0164715912724,18.7602640876538,36.4404173940036));
#48484=CARTESIAN_POINT('Ctrl Pts',(18.9580479481332,18.7647100967698,36.4750413485818));
#48485=CARTESIAN_POINT('Ctrl Pts',(18.9013920663298,18.7691561058858,36.5127913535199));
#48486=CARTESIAN_POINT('Ctrl Pts',(18.8468535916639,18.7736021150017,36.5534567843602));
#48487=CARTESIAN_POINT('Ctrl Pts',(18.7923468103982,18.7780455404527,36.594098583704));
#48488=CARTESIAN_POINT('Ctrl Pts',(18.7399553898737,18.7824889659038,36.6376521538038));
#48489=CARTESIAN_POINT('Ctrl Pts',(18.6899997011006,18.7869323913548,36.6838637869952));
#48490=CARTESIAN_POINT('Ctrl Pts',(18.6400558261219,18.7913747660002,36.730064491807));
#48491=CARTESIAN_POINT('Ctrl Pts',(18.5925469010025,18.7958171406457,36.7789216767792));
#48492=CARTESIAN_POINT('Ctrl Pts',(18.5477585210014,18.8002595152912,36.830142825521));
#48493=CARTESIAN_POINT('Ctrl Pts',(18.5029652977025,18.8047023703234,36.8813695131832));
#48494=CARTESIAN_POINT('Ctrl Pts',(18.4608935259458,18.8091452253556,36.9349602989744));
#48495=CARTESIAN_POINT('Ctrl Pts',(18.421789162117,18.8135880803878,36.9905888462394));
#48496=CARTESIAN_POINT('Ctrl Pts',(18.3826421080963,18.81803578568,37.0462781231293));
#48497=CARTESIAN_POINT('Ctrl Pts',(18.3464692088349,18.8224834909722,37.104009195492));
#48498=CARTESIAN_POINT('Ctrl Pts',(18.3134730224323,18.8269311962645,37.1634268256903));
#48499=CARTESIAN_POINT('Ctrl Pts',(18.2804555392723,18.831381772243,37.2228828058617));
#48500=CARTESIAN_POINT('Ctrl Pts',(18.2506190645463,18.8358323482216,37.2840270667302));
#48501=CARTESIAN_POINT('Ctrl Pts',(18.2241188731087,18.8402829242001,37.3464823956593));
#48502=CARTESIAN_POINT('Ctrl Pts',(18.1975743674798,18.8447409425278,37.4090421637356));
#48503=CARTESIAN_POINT('Ctrl Pts',(18.1743774426708,18.8491989608554,37.4729169108286));
#48504=CARTESIAN_POINT('Ctrl Pts',(18.1546338850032,18.853656979183,37.5377131883803));
#48505=CARTESIAN_POINT('Ctrl Pts',(18.148670593706,18.8550034671029,37.5572840825687));
#48506=CARTESIAN_POINT('Ctrl Pts',(18.1430219876732,18.8563499550229,37.5769389731496));
#48507=CARTESIAN_POINT('Ctrl Pts',(18.1376900600936,18.8576964429428,37.5966668651619));
#48508=CARTESIAN_POINT('Ctrl Pts',(18.1153926025753,18.8633272878381,37.6791664541953));
#48509=CARTESIAN_POINT('Ctrl Pts',(18.0985664791579,18.8689581327334,37.7632031113543));
#48510=CARTESIAN_POINT('Ctrl Pts',(18.0873818825785,18.8745889776287,37.848137946862));
#48511=CARTESIAN_POINT('Ctrl Pts',(18.0764875166079,18.8800737069685,37.9308687968393));
#48512=CARTESIAN_POINT('Ctrl Pts',(18.0709456587466,18.8855584363083,38.0144519820069));
#48513=CARTESIAN_POINT('Ctrl Pts',(18.0708707698807,18.8910431656481,38.0982765153061));
#48514=CARTESIAN_POINT('Ctrl Pts',(18.0708707514445,18.8906962854919,38.098297276432));
#48515=CARTESIAN_POINT('Ctrl Pts',(18.0707906498881,18.8961279122774,38.1890496793503));
#48516=CARTESIAN_POINT('Ctrl Pts',(18.0771143768436,18.9016047975629,38.2796889011574));
#48517=CARTESIAN_POINT('Ctrl Pts',(18.0945784531256,18.9094020141416,38.4034535409684));
#48518=CARTESIAN_POINT('Ctrl Pts',(18.1002652032124,18.9115621796977,38.4372281166426));
#48519=CARTESIAN_POINT('Ctrl Pts',(18.1088383024623,18.9144118889741,38.4809950696164));
#48520=CARTESIAN_POINT('Ctrl Pts',(18.1109108385906,18.9150761028551,38.4911418449372));
#48521=CARTESIAN_POINT('Ctrl Pts',(18.1145443264148,18.9162007928593,38.5082279306263));
#48522=CARTESIAN_POINT('Ctrl Pts',(18.1160621540314,18.9166599095217,38.5151762646294));
#48523=CARTESIAN_POINT('Ctrl Pts',(18.1191379160774,18.9175697357968,38.5288923010251));
#48524=CARTESIAN_POINT('Ctrl Pts',(18.1206940418777,18.9180203820005,38.5356603014891));
#48525=CARTESIAN_POINT('Ctrl Pts',(18.1237590521184,18.9188898985739,38.5486687884058));
#48526=CARTESIAN_POINT('Ctrl Pts',(18.1252626150435,18.9193085939407,38.5549104439087));
#48527=CARTESIAN_POINT('Ctrl Pts',(18.1287809599841,18.9202707709,38.5692022211786));
#48528=CARTESIAN_POINT('Ctrl Pts',(18.1308165731257,18.9208149127047,38.5772470357692));
#48529=CARTESIAN_POINT('Ctrl Pts',(18.1363761821166,18.9222686196259,38.5986374881804));
#48530=CARTESIAN_POINT('Ctrl Pts',(18.1399915614944,18.9231810979369,38.6119586615496));
#48531=CARTESIAN_POINT('Ctrl Pts',(18.1727572078703,18.9311771051349,38.7277558081209));
#48532=CARTESIAN_POINT('Ctrl Pts',(18.2102023315209,18.9385317273811,38.8276750477035));
#48533=CARTESIAN_POINT('Ctrl Pts',(18.2848351165201,18.950874838632,38.9856672731724));
#48534=CARTESIAN_POINT('Ctrl Pts',(18.3172265037518,18.9557511408271,39.0457641994098));
#48535=CARTESIAN_POINT('Ctrl Pts',(18.3891686105606,18.9656080080847,39.1637980136889));
#48536=CARTESIAN_POINT('Ctrl Pts',(18.4288351832321,18.9705808123152,39.2215553381599));
#48537=CARTESIAN_POINT('Ctrl Pts',(18.4931045497217,18.9778773835261,39.3050128380167));
#48538=CARTESIAN_POINT('Ctrl Pts',(18.5154186923663,18.9802908761362,39.3323995156586));
#48539=CARTESIAN_POINT('Ctrl Pts',(18.5433164774905,18.9831530124948,39.3647808967306));
#48540=CARTESIAN_POINT('Ctrl Pts',(18.5481915395274,18.98364767971,39.3703738819675));
#48541=CARTESIAN_POINT('Ctrl Pts',(18.5558373109765,18.9844148110008,39.3790441068246));
#48542=CARTESIAN_POINT('Ctrl Pts',(18.5585858005894,18.9846888552475,39.3821407122887));
#48543=CARTESIAN_POINT('Ctrl Pts',(18.5637159031975,18.9851971311477,39.3878832332648));
#48544=CARTESIAN_POINT('Ctrl Pts',(18.5660948480465,18.9854315454793,39.3905313807794));
#48545=CARTESIAN_POINT('Ctrl Pts',(18.5715224320732,18.9859634687333,39.3965396169135));
#48546=CARTESIAN_POINT('Ctrl Pts',(18.5745755979911,18.9862606337284,39.3998955402232));
#48547=CARTESIAN_POINT('Ctrl Pts',(18.5839393811803,18.9871658682378,39.4101151910373));
#48548=CARTESIAN_POINT('Ctrl Pts',(18.5902880581646,18.9877711603867,39.4169440912465));
#48549=CARTESIAN_POINT('Ctrl Pts',(18.6516553300898,18.9935446270373,39.4820009736538));
#48550=CARTESIAN_POINT('Ctrl Pts',(18.7102086178773,18.99846379317,39.5368025678053));
#48551=CARTESIAN_POINT('Ctrl Pts',(18.8988367481208,19.0132325226787,39.6924903988199));
#48552=CARTESIAN_POINT('Ctrl Pts',(19.0385214428604,19.0228200872732,39.7805191474336));
#48553=CARTESIAN_POINT('Ctrl Pts',(19.2114467774253,19.0347173185124,39.8607989697987));
#48554=CARTESIAN_POINT('Ctrl Pts',(19.2354356793378,19.0363665234294,39.871347085743));
#48555=CARTESIAN_POINT('Ctrl Pts',(19.2774226156965,19.0392559826455,39.8887972754145));
#48556=CARTESIAN_POINT('Ctrl Pts',(19.2953233188535,19.0404887606648,39.8959244141232));
#48557=CARTESIAN_POINT('Ctrl Pts',(19.3213625452887,19.0422846203926,39.9058426550988));
#48558=CARTESIAN_POINT('Ctrl Pts',(19.329418087354,19.0428405443534,39.9088494642769));
#48559=CARTESIAN_POINT('Ctrl Pts',(19.3435727206139,19.043818113442,39.9140252710871));
#48560=CARTESIAN_POINT('Ctrl Pts',(19.349663173035,19.0442389796953,39.9162176265688));
#48561=CARTESIAN_POINT('Ctrl Pts',(19.3614218152065,19.0450520413457,39.920383608365));
#48562=CARTESIAN_POINT('Ctrl Pts',(19.3670884163065,19.0454440899248,39.9223615188978));
#48563=CARTESIAN_POINT('Ctrl Pts',(19.3805212896988,19.046374034607,39.9269800140273));
#48564=CARTESIAN_POINT('Ctrl Pts',(19.3882953066201,19.0469126794931,39.9295975537703));
#48565=CARTESIAN_POINT('Ctrl Pts',(19.4157035295922,19.0488134915824,39.9386317917897));
#48566=CARTESIAN_POINT('Ctrl Pts',(19.4354232952824,19.0501842709797,39.9447824585889));
#48567=CARTESIAN_POINT('Ctrl Pts',(19.6159199254433,19.0627643895206,39.9979149630277));
#48568=CARTESIAN_POINT('Ctrl Pts',(19.7820487445648,19.0746758760273,40.0240770974184));
#48569=CARTESIAN_POINT('Ctrl Pts',(20.0207665283856,19.0917017002924,40.0303380376165));
#48570=CARTESIAN_POINT('Ctrl Pts',(20.0921656977009,19.096768124827,40.0282487097215));
#48571=CARTESIAN_POINT('Ctrl Pts',(20.1956632830447,19.1039485014327,40.0194567164022));
#48572=CARTESIAN_POINT('Ctrl Pts',(20.2279652136805,19.1061657258914,40.0158889251795));
#48573=CARTESIAN_POINT('Ctrl Pts',(20.2676182481678,19.1088460980912,40.0104919858527));
#48574=CARTESIAN_POINT('Ctrl Pts',(20.2750668288834,19.109347777236,40.0094337901562));
#48575=CARTESIAN_POINT('Ctrl Pts',(20.2866272773809,19.1101233854474,40.0077223831495));
#48576=CARTESIAN_POINT('Ctrl Pts',(20.2907434412172,19.1103989504252,40.0070994047271));
#48577=CARTESIAN_POINT('Ctrl Pts',(20.2983732193016,19.1109085976733,40.0059193671554));
#48578=CARTESIAN_POINT('Ctrl Pts',(20.3018872794348,19.1111428716309,40.0053659183884));
#48579=CARTESIAN_POINT('Ctrl Pts',(20.3098488707188,19.1116726359383,40.0040894245128));
#48580=CARTESIAN_POINT('Ctrl Pts',(20.314295403677,19.1119677937435,40.0033605174724));
#48581=CARTESIAN_POINT('Ctrl Pts',(20.3277806210479,19.1128608757421,40.0011013805808));
#48582=CARTESIAN_POINT('Ctrl Pts',(20.3368111500519,19.11345613021,39.9995222694242));
#48583=CARTESIAN_POINT('Ctrl Pts',(20.4534515621832,19.1211122342419,39.9782681261434));
#48584=CARTESIAN_POINT('Ctrl Pts',(20.5592274462939,19.1277044941696,39.9495355010542));
#48585=CARTESIAN_POINT('Ctrl Pts',(20.7404239761828,19.1392471380287,39.883335193607));
#48586=CARTESIAN_POINT('Ctrl Pts',(20.8168949191811,19.1442035541571,39.849626913998));
#48587=CARTESIAN_POINT('Ctrl Pts',(20.9605196114213,19.1540177554338,39.7748428487155));
#48588=CARTESIAN_POINT('Ctrl Pts',(21.0278173895146,19.1588540783821,39.7344068545603));
#48589=CARTESIAN_POINT('Ctrl Pts',(21.1082167820642,19.1650551008631,39.6791654447412));
#48590=CARTESIAN_POINT('Ctrl Pts',(21.1238091029239,19.1662784964438,39.6681074569081));
#48591=CARTESIAN_POINT('Ctrl Pts',(21.1461680883278,19.1680645594553,39.6517458222036));
#48592=CARTESIAN_POINT('Ctrl Pts',(21.1530680057146,19.1686202042484,39.6466255376471));
#48593=CARTESIAN_POINT('Ctrl Pts',(21.1650818638899,19.1695956518826,39.6375852247139));
#48594=CARTESIAN_POINT('Ctrl Pts',(21.1702108364198,19.170014669007,39.633685322833));
#48595=CARTESIAN_POINT('Ctrl Pts',(21.1801173168731,19.1708290567045,39.6260741373759));
#48596=CARTESIAN_POINT('Ctrl Pts',(21.1848970997114,19.1712243035831,39.6223659271176));
#48597=CARTESIAN_POINT('Ctrl Pts',(21.1962617935754,19.1721696505606,39.6134631223066));
#48598=CARTESIAN_POINT('Ctrl Pts',(21.2028303807807,19.1727205591319,39.6082479811598));
#48599=CARTESIAN_POINT('Ctrl Pts',(21.2263271732758,19.1747077205613,39.5893415439728));
#48600=CARTESIAN_POINT('Ctrl Pts',(21.2430567944686,19.1761536435346,39.5754071677336));
#48601=CARTESIAN_POINT('Ctrl Pts',(21.3749712492519,19.1878113260224,39.4616970897988));
#48602=CARTESIAN_POINT('Ctrl Pts',(21.4781786390825,19.1985899540993,39.3488935199546));
#48603=CARTESIAN_POINT('Ctrl Pts',(21.6147140008288,19.2152943951347,39.1587383294762));
#48604=CARTESIAN_POINT('Ctrl Pts',(21.6581355057822,19.2211250727037,39.0893515415398));
#48605=CARTESIAN_POINT('Ctrl Pts',(21.7140198620851,19.2292676491691,38.9859772138713));
#48606=CARTESIAN_POINT('Ctrl Pts',(21.7301395638964,19.2317104257583,38.9540709578044));
#48607=CARTESIAN_POINT('Ctrl Pts',(21.7485223977939,19.2346002939951,38.9150257287601));
#48608=CARTESIAN_POINT('Ctrl Pts',(21.7516415512461,19.2350945639704,38.9083003120531));
#48609=CARTESIAN_POINT('Ctrl Pts',(21.7564417174681,19.235861214793,38.8977920669434));
#48610=CARTESIAN_POINT('Ctrl Pts',(21.7581494143675,19.2361351726784,38.894021615889));
#48611=CARTESIAN_POINT('Ctrl Pts',(21.7613032844763,19.2366433714789,38.8869980752235));
#48612=CARTESIAN_POINT('Ctrl Pts',(21.7627525747353,19.2368777945587,38.8837465093373));
#48613=CARTESIAN_POINT('Ctrl Pts',(21.7660291691425,19.2374098439672,38.8763402156537));
#48614=CARTESIAN_POINT('Ctrl Pts',(21.7678508142366,19.2377071257072,38.872183045881));
#48615=CARTESIAN_POINT('Ctrl Pts',(21.7733733963565,19.2386130699385,38.8594580026542));
#48616=CARTESIAN_POINT('Ctrl Pts',(21.7770269116391,19.2392189487111,38.8508695122983));
#48617=CARTESIAN_POINT('Ctrl Pts',(21.8118139471688,19.2450554854268,38.7674177964319));
#48618=CARTESIAN_POINT('Ctrl Pts',(21.8382652102286,19.2500310076296,38.6906782584562));
#48619=CARTESIAN_POINT('Ctrl Pts',(21.9033471766848,19.2648175440783,38.4544988936035));
#48620=CARTESIAN_POINT('Ctrl Pts',(21.9265731119114,19.2743765017034,38.2916121687378));
#48621=CARTESIAN_POINT('Ctrl Pts',(21.9294953394293,19.2870574120657,38.0884795069982));
#48622=CARTESIAN_POINT('Ctrl Pts',(21.9288609128268,19.289540385216,38.0492040682617));
#48623=CARTESIAN_POINT('Ctrl Pts',(21.9265011223943,19.29278568671,37.998690281669));
#48624=CARTESIAN_POINT('Ctrl Pts',(21.9258746890966,19.293513827801,37.9874082299503));
#48625=CARTESIAN_POINT('Ctrl Pts',(21.924700084137,19.2946976858565,37.9691525112911));
#48626=CARTESIAN_POINT('Ctrl Pts',(21.9242130250149,19.2951514979984,37.9621750697146));
#48627=CARTESIAN_POINT('Ctrl Pts',(21.9232072916015,19.2960231432618,37.948813715414));
#48628=CARTESIAN_POINT('Ctrl Pts',(21.922694747192,19.2964407798532,37.942429423489));
#48629=CARTESIAN_POINT('Ctrl Pts',(21.9214540792651,19.2973949606404,37.9278840173042));
#48630=CARTESIAN_POINT('Ctrl Pts',(21.9207057394289,19.2979321281679,37.9197247957701));
#48631=CARTESIAN_POINT('Ctrl Pts',(21.9185921225952,19.2993551342344,37.8981891622268));
#48632=CARTESIAN_POINT('Ctrl Pts',(21.9171389541849,19.3002436944753,37.8848220225304));
#48633=CARTESIAN_POINT('Ctrl Pts',(21.9049485371264,19.30707784857,37.7826408870221));
#48634=CARTESIAN_POINT('Ctrl Pts',(21.8881863972404,19.3132116524389,37.6946684533206));
#48635=CARTESIAN_POINT('Ctrl Pts',(21.8240870167428,19.330847364444,37.4515476346088));
#48636=CARTESIAN_POINT('Ctrl Pts',(21.7632278327173,19.3426465971593,37.3007452078152));
#48637=CARTESIAN_POINT('Ctrl Pts',(21.6695501463812,19.3558927494013,37.1330187138656));
#48638=CARTESIAN_POINT('Ctrl Pts',(21.6542418935626,19.3579445363137,37.1070576523065));
#48639=CARTESIAN_POINT('Ctrl Pts',(21.6346130505554,19.3604320959398,37.0754843528617));
#48640=CARTESIAN_POINT('Ctrl Pts',(21.6308626449337,19.360901279858,37.0695247827274));
#48641=CARTESIAN_POINT('Ctrl Pts',(21.6248997907977,19.3616375432812,37.0601636236867));
#48642=CARTESIAN_POINT('Ctrl Pts',(21.6227091432955,19.3619060072656,37.0567483253507));
#48643=CARTESIAN_POINT('Ctrl Pts',(21.6185694220651,19.362409500905,37.0503389376814));
#48644=CARTESIAN_POINT('Ctrl Pts',(21.6166228294264,19.3626446795766,37.0473433858009));
#48645=CARTESIAN_POINT('Ctrl Pts',(21.6121577868753,19.363180567156,37.0405138660463));
#48646=CARTESIAN_POINT('Ctrl Pts',(21.6096339779518,19.3634809164968,37.0366834639127));
#48647=CARTESIAN_POINT('Ctrl Pts',(21.6029018196531,19.3642754490069,37.0265449171148));
#48648=CARTESIAN_POINT('Ctrl Pts',(21.5986698467693,19.3647681089002,37.0202524443057));
#48649=CARTESIAN_POINT('Ctrl Pts',(21.5684907184055,19.3682349692436,36.975945851198));
#48650=CARTESIAN_POINT('Ctrl Pts',(21.5412251838817,19.3711275117729,36.9388425691465));
#48651=CARTESIAN_POINT('Ctrl Pts',(21.4281852725925,19.3823720202558,36.7960235515076));
#48652=CARTESIAN_POINT('Ctrl Pts',(21.3326523810961,19.3903226700516,36.6985326085782));
#48653=CARTESIAN_POINT('Ctrl Pts',(21.1772583148209,19.4024726781103,36.570335873975));
#48654=CARTESIAN_POINT('Ctrl Pts',(21.1247953903617,19.406459354497,36.5313560835936));
#48655=CARTESIAN_POINT('Ctrl Pts',(21.0385666749033,19.4129340534054,36.4738414877088));
#48656=CARTESIAN_POINT('Ctrl Pts',(21.0060485440344,19.4153589954491,36.4535255069986));
#48657=CARTESIAN_POINT('Ctrl Pts',(20.963272794036,19.4185385476312,36.4285414643524));
#48658=CARTESIAN_POINT('Ctrl Pts',(20.9535482498931,19.4192606893972,36.4229747054285));
#48659=CARTESIAN_POINT('Ctrl Pts',(20.9376938149794,19.4204371813263,36.4140814083175));
#48660=CARTESIAN_POINT('Ctrl Pts',(20.93159331664,19.4208896707444,36.4107027855618));
#48661=CARTESIAN_POINT('Ctrl Pts',(20.919849620341,19.4217604072261,36.4042817646799));
#48662=CARTESIAN_POINT('Ctrl Pts',(20.9142093028479,19.422178466675,36.4012342696634));
#48663=CARTESIAN_POINT('Ctrl Pts',(20.9012883686087,19.42313589576,36.3943360035748));
#48664=CARTESIAN_POINT('Ctrl Pts',(20.8939981112202,19.4236759037267,36.3905036514571));
#48665=CARTESIAN_POINT('Ctrl Pts',(20.8746134024453,19.4251113871404,36.3804713827115));
#48666=CARTESIAN_POINT('Ctrl Pts',(20.8624777674202,19.4260096613587,36.3743524826535));
#48667=CARTESIAN_POINT('Ctrl Pts',(20.7646150946882,19.4332515272699,36.3262993834132));
#48668=CARTESIAN_POINT('Ctrl Pts',(20.6759619835534,19.4398104457271,36.2906574498809));
#48669=CARTESIAN_POINT('Ctrl Pts',(20.4915627983093,19.4534201399859,36.2319707448975));
#48670=CARTESIAN_POINT('Ctrl Pts',(20.3959467059997,19.4604600938781,36.2093937787486));
#48671=CARTESIAN_POINT('Ctrl Pts',(20.241168989698,19.4715951044553,36.1851081024778));
#48672=CARTESIAN_POINT('Ctrl Pts',(20.1829151524675,19.4757259341796,36.1786680388432));
#48673=CARTESIAN_POINT('Ctrl Pts',(20.0953347120372,19.4817717569566,36.1730061311067));
#48674=CARTESIAN_POINT('Ctrl Pts',(20.0661736991428,19.4837574347634,36.1717844136512));
#48675=CARTESIAN_POINT('Ctrl Pts',(20.0300253983929,19.4861762050208,36.1710910814191));
#48676=CARTESIAN_POINT('Ctrl Pts',(20.0230556645701,19.4866405999431,36.1709951838509));
#48677=CARTESIAN_POINT('Ctrl Pts',(20.0120438484697,19.4873710530011,36.1709033621507));
#48678=CARTESIAN_POINT('Ctrl Pts',(20.0080021209366,19.4876384600408,36.1708823625154));
#48679=CARTESIAN_POINT('Ctrl Pts',(20.0003846181427,19.4881410983609,36.1708667245096));
#48680=CARTESIAN_POINT('Ctrl Pts',(19.9968089663945,19.4883764721597,36.1708693252981));
#48681=CARTESIAN_POINT('Ctrl Pts',(19.9886202559793,19.4889142423174,36.1708980487425));
#48682=CARTESIAN_POINT('Ctrl Pts',(19.9840072711198,19.4892162698322,36.1709307760915));
#48683=CARTESIAN_POINT('Ctrl Pts',(19.9717234068829,19.4900181986092,36.1710619911814));
#48684=CARTESIAN_POINT('Ctrl Pts',(19.9640528272603,19.4905165310908,36.1711896897076));
#48685=CARTESIAN_POINT('Ctrl Pts',(19.9082870676032,19.4941231277532,36.172450856004));
#48686=CARTESIAN_POINT('Ctrl Pts',(19.8602438938308,19.4971421006209,36.175337411719));
#48687=CARTESIAN_POINT('Ctrl Pts',(19.7959945716255,19.5011204470937,36.18161668354));
#48688=CARTESIAN_POINT('Ctrl Pts',(19.7796553017627,19.5021270191859,36.1834246686603));
#48689=CARTESIAN_POINT('Ctrl Pts',(19.6497183711775,19.5101041366138,36.1994862134574));
#48690=CARTESIAN_POINT('Ctrl Pts',(19.5375685047347,19.5168343289807,36.2236180944196));
#48691=CARTESIAN_POINT('Ctrl Pts',(19.4168111704594,19.5244522547812,36.261093811437));
#48692=CARTESIAN_POINT('Ctrl Pts',(19.4054396628868,19.5251732142282,36.2647389497829));
#48693=CARTESIAN_POINT('Ctrl Pts',(19.3941040005193,19.5258959448669,36.2684889859154));
#48694=CARTESIAN_POINT('Origin',(20.,-1.3495818343519,38.1));
#48695=CARTESIAN_POINT('',(19.3941040087494,20.489691467393,36.2684889831927));
#48696=CARTESIAN_POINT('',(19.3941039696621,20.3190989370965,36.2684889961235));
#48697=CARTESIAN_POINT('',(19.3941040087494,-1.3495818343519,36.2684889831927));
#48698=CARTESIAN_POINT('',(18.0708701870214,19.8542362730884,38.1008494569394));
#48699=CARTESIAN_POINT('Ctrl Pts',(19.3941040087494,20.489691467393,36.2684889831927));
#48700=CARTESIAN_POINT('Ctrl Pts',(19.4003737701409,20.4892600094623,36.2664148360768));
#48701=CARTESIAN_POINT('Ctrl Pts',(19.4066542566161,20.4888303778034,36.2643728589592));
#48702=CARTESIAN_POINT('Ctrl Pts',(19.448459657195,20.4859868203442,36.2510176304672));
#48703=CARTESIAN_POINT('Ctrl Pts',(19.4842984026903,20.4836268337685,36.240703127972));
#48704=CARTESIAN_POINT('Ctrl Pts',(19.6764534995626,20.4712729270058,36.191384880702));
#48705=CARTESIAN_POINT('Ctrl Pts',(19.8369044177153,20.4619517070475,36.1710354838721));
#48706=CARTESIAN_POINT('Ctrl Pts',(20.0807375178535,20.4471561321505,36.1707865775156));
#48707=CARTESIAN_POINT('Ctrl Pts',(20.1633544411664,20.4420432668475,36.1760208621107));
#48708=CARTESIAN_POINT('Ctrl Pts',(20.2585168863516,20.4359139170974,36.1882240844466));
#48709=CARTESIAN_POINT('Ctrl Pts',(20.2716417480344,20.4350633368021,36.1900447967326));
#48710=CARTESIAN_POINT('Ctrl Pts',(20.2928798372764,20.4336780389967,36.1932143325977));
#48711=CARTESIAN_POINT('Ctrl Pts',(20.3010051703234,20.4331459238618,36.1944801065095));
#48712=CARTESIAN_POINT('Ctrl Pts',(20.3154295486177,20.4321974117733,36.1968217136535));
#48713=CARTESIAN_POINT('Ctrl Pts',(20.3217318467426,20.431781667431,36.1978769737692));
#48714=CARTESIAN_POINT('Ctrl Pts',(20.3349736125639,20.4309053149536,36.2001618744381));
#48715=CARTESIAN_POINT('Ctrl Pts',(20.3419118044627,20.4304444995495,36.2013982670901));
#48716=CARTESIAN_POINT('Ctrl Pts',(20.3601945091911,20.4292258058689,36.2047597288448));
#48717=CARTESIAN_POINT('Ctrl Pts',(20.3715268561706,20.4284659235933,36.206948612631));
#48718=CARTESIAN_POINT('Ctrl Pts',(20.4238094756681,20.4249388651305,36.2175347252619));
#48719=CARTESIAN_POINT('Ctrl Pts',(20.4644968816419,20.4221331606981,36.2271593311256));
#48720=CARTESIAN_POINT('Ctrl Pts',(20.6664597507865,20.40788773265,36.2819196234114));
#48721=CARTESIAN_POINT('Ctrl Pts',(20.8216704057554,20.395823118403,36.3465963751211));
#48722=CARTESIAN_POINT('Ctrl Pts',(20.9742527073621,20.3833267818593,36.4349313818391));
#48723=CARTESIAN_POINT('Ctrl Pts',(20.9819277349018,20.3826966256383,36.4394459457519));
#48724=CARTESIAN_POINT('Ctrl Pts',(21.0077735404067,20.3805697593032,36.4548906776616));
#48725=CARTESIAN_POINT('Ctrl Pts',(21.0257957161072,20.3790786018366,36.4660675079296));
#48726=CARTESIAN_POINT('Ctrl Pts',(21.0822395945951,20.3743900623568,36.5023744307044));
#48727=CARTESIAN_POINT('Ctrl Pts',(21.1199537210303,20.3712296218914,36.5285820268466));
#48728=CARTESIAN_POINT('Ctrl Pts',(21.1627629848999,20.3676406247315,36.5606552716684));
#48729=CARTESIAN_POINT('Ctrl Pts',(21.1687993348274,20.3671345249312,36.5652335450576));
#48730=CARTESIAN_POINT('Ctrl Pts',(21.1784451768992,20.366325955649,36.5726393545231));
#48731=CARTESIAN_POINT('Ctrl Pts',(21.1820717582957,20.3660219911553,36.5754443481381));
#48732=CARTESIAN_POINT('Ctrl Pts',(21.1885060175996,20.3654828150865,36.5804577129283));
#48733=CARTESIAN_POINT('Ctrl Pts',(21.1913175983449,20.3652472530296,36.5826609816062));
#48734=CARTESIAN_POINT('Ctrl Pts',(21.1973107455981,20.3647452329412,36.5873843819638));
#48735=CARTESIAN_POINT('Ctrl Pts',(21.2004904782079,20.3644789363776,36.5899067439605));
#48736=CARTESIAN_POINT('Ctrl Pts',(21.2091688514344,20.3637522186699,36.5968357049795));
#48737=CARTESIAN_POINT('Ctrl Pts',(21.2146514138149,20.3632932026094,36.6012624793627));
#48738=CARTESIAN_POINT('Ctrl Pts',(21.243502961599,20.3608773869767,36.6248203375419));
#48739=CARTESIAN_POINT('Ctrl Pts',(21.2664460462865,20.3589553133393,36.6444694059582));
#48740=CARTESIAN_POINT('Ctrl Pts',(21.4093897776415,20.3469033168646,36.7728304710716));
#48741=CARTESIAN_POINT('Ctrl Pts',(21.5157737961787,20.3375327060044,36.8957572323788));
#48742=CARTESIAN_POINT('Ctrl Pts',(21.6551366525536,20.3223255683894,37.1049802836952));
#48743=CARTESIAN_POINT('Ctrl Pts',(21.6994757243467,20.3168144994628,37.1827646391397));
#48744=CARTESIAN_POINT('Ctrl Pts',(21.7440884481492,20.3102445025727,37.2754523481984));
#48745=CARTESIAN_POINT('Ctrl Pts',(21.7497929198497,20.3093815509407,37.2876281220833));
#48746=CARTESIAN_POINT('Ctrl Pts',(21.7587680157842,20.3079857314959,37.307317995174));
#48747=CARTESIAN_POINT('Ctrl Pts',(21.762118918262,20.307455601923,37.3147951804669));
#48748=CARTESIAN_POINT('Ctrl Pts',(21.7680042324441,20.3065081625159,37.3281550558815));
#48749=CARTESIAN_POINT('Ctrl Pts',(21.7705571863148,20.3060914886762,37.334029483568));
#48750=CARTESIAN_POINT('Ctrl Pts',(21.7758368708076,20.3052176860876,37.3463456392927));
#48751=CARTESIAN_POINT('Ctrl Pts',(21.7785579099802,20.3047603725557,37.3527896910399));
#48752=CARTESIAN_POINT('Ctrl Pts',(21.7855830949605,20.303561128059,37.3696827575806));
#48753=CARTESIAN_POINT('Ctrl Pts',(21.789830527572,20.3028173079436,37.3801549215465));
#48754=CARTESIAN_POINT('Ctrl Pts',(21.8084299061664,20.2994739109204,37.4271946880162));
#48755=CARTESIAN_POINT('Ctrl Pts',(21.8217540209026,20.2968405480562,37.4641559785782));
#48756=CARTESIAN_POINT('Ctrl Pts',(21.8847996115625,20.2830336747431,37.657340703669));
#48757=CARTESIAN_POINT('Ctrl Pts',(21.9155796983059,20.2712546804561,37.8190137207699));
#48758=CARTESIAN_POINT('Ctrl Pts',(21.930484721245,20.2538623153076,38.0634575314035));
#48759=CARTESIAN_POINT('Ctrl Pts',(21.9303169727918,20.2481754728189,38.1445670231513));
#48760=CARTESIAN_POINT('Ctrl Pts',(21.9244409134107,20.2421017467532,38.234747273721));
#48761=CARTESIAN_POINT('Ctrl Pts',(21.9237664989189,20.2414778086436,38.2440559725197));
#48762=CARTESIAN_POINT('Ctrl Pts',(21.9226637112822,20.2405557773619,38.257884172203));
#48763=CARTESIAN_POINT('Ctrl Pts',(21.9222869117001,20.2402549444014,38.2624074772468));
#48764=CARTESIAN_POINT('Ctrl Pts',(21.9215860834899,20.2397197359984,38.2704762601647));
#48765=CARTESIAN_POINT('Ctrl Pts',(21.921268202413,20.239485025263,38.2740222016194));
#48766=CARTESIAN_POINT('Ctrl Pts',(21.9205594917211,20.2389786191623,38.2816891020133));
#48767=CARTESIAN_POINT('Ctrl Pts',(21.9201652154525,20.2387071178283,38.28580968003));
#48768=CARTESIAN_POINT('Ctrl Pts',(21.9190277193192,20.2379513364583,38.2973072231957));
#48769=CARTESIAN_POINT('Ctrl Pts',(21.9182552203285,20.2374686551939,38.3046813178255));
#48770=CARTESIAN_POINT('Ctrl Pts',(21.9135104383686,20.2346712922682,38.3475853321041));
#48771=CARTESIAN_POINT('Ctrl Pts',(21.9085933188767,20.2324056576276,38.3830064169601));
#48772=CARTESIAN_POINT('Ctrl Pts',(21.889195558839,20.2250727663824,38.4989697712635));
#48773=CARTESIAN_POINT('Ctrl Pts',(21.8705757360531,20.2201617540855,38.5787331131643));
#48774=CARTESIAN_POINT('Ctrl Pts',(21.8029641689762,20.2061641918161,38.8028933201032));
#48775=CARTESIAN_POINT('Ctrl Pts',(21.7418774490001,20.1971304880754,38.9429682626295));
#48776=CARTESIAN_POINT('Ctrl Pts',(21.6539641619233,20.1861016074642,39.0931863013645));
#48777=CARTESIAN_POINT('Ctrl Pts',(21.6426514600384,20.184711567242,39.1117868342778));
#48778=CARTESIAN_POINT('Ctrl Pts',(21.6265480396728,20.1827702336645,39.1372822038935));
#48779=CARTESIAN_POINT('Ctrl Pts',(21.622023180089,20.1822286427838,39.1443436673326));
#48780=CARTESIAN_POINT('Ctrl Pts',(21.6141555000811,20.1812934733463,39.1564474312123));
#48781=CARTESIAN_POINT('Ctrl Pts',(21.6108347155179,20.1809007123259,39.1615039666706));
#48782=CARTESIAN_POINT('Ctrl Pts',(21.6039279490535,20.1800877861318,39.1719138061243));
#48783=CARTESIAN_POINT('Ctrl Pts',(21.6003388248393,20.1796675072494,39.1772649244924));
#48784=CARTESIAN_POINT('Ctrl Pts',(21.5919009893504,20.1786844025845,39.1897098829243));
#48785=CARTESIAN_POINT('Ctrl Pts',(21.587031587146,20.1781208041822,39.1967894630298));
#48786=CARTESIAN_POINT('Ctrl Pts',(21.5711766741923,20.1762975005698,39.2195141190028));
#48787=CARTESIAN_POINT('Ctrl Pts',(21.5600061435348,20.1750308064343,39.2350281017775));
#48788=CARTESIAN_POINT('Ctrl Pts',(21.5018191277852,20.1685200280092,39.3133581990986));
#48789=CARTESIAN_POINT('Ctrl Pts',(21.4512381610161,20.1631385692436,39.3734220790766));
#48790=CARTESIAN_POINT('Ctrl Pts',(21.3396191206589,20.1518076081176,39.490655754728));
#48791=CARTESIAN_POINT('Ctrl Pts',(21.2782352683836,20.1458550071135,39.5472787744822));
#48792=CARTESIAN_POINT('Ctrl Pts',(21.1282938938944,20.1320944440345,39.6685901398657));
#48793=CARTESIAN_POINT('Ctrl Pts',(21.0374888772426,20.1243075787417,39.7300750890072));
#48794=CARTESIAN_POINT('Ctrl Pts',(20.9339500509643,20.1163360914232,39.7880058845919));
#48795=CARTESIAN_POINT('Ctrl Pts',(20.9259193923395,20.1157234634645,39.7924242527095));
#48796=CARTESIAN_POINT('Ctrl Pts',(20.9138945509943,20.1148148777526,39.7989289583606));
#48797=CARTESIAN_POINT('Ctrl Pts',(20.9099241988567,20.1145162924837,39.8010587318643));
#48798=CARTESIAN_POINT('Ctrl Pts',(20.9028057230424,20.1139835257834,39.8048451653439));
#48799=CARTESIAN_POINT('Ctrl Pts',(20.8996604563077,20.1137490214714,39.8065070393645));
#48800=CARTESIAN_POINT('Ctrl Pts',(20.8928242438943,20.1132412762867,39.8100949559024));
#48801=CARTESIAN_POINT('Ctrl Pts',(20.8891316636332,20.1129682389719,39.8120177493889));
#48802=CARTESIAN_POINT('Ctrl Pts',(20.8787481064662,20.1122037974739,39.8173820000232));
#48803=CARTESIAN_POINT('Ctrl Pts',(20.8720430878048,20.1117140520603,39.820796334889));
#48804=CARTESIAN_POINT('Ctrl Pts',(20.8316730017611,20.108787551232,39.8410570624259));
#48805=CARTESIAN_POINT('Ctrl Pts',(20.7975380820846,20.1064052882328,39.856955645222));
#48806=CARTESIAN_POINT('Ctrl Pts',(20.6114211785716,20.0937908323632,39.9370975943917));
#48807=CARTESIAN_POINT('Ctrl Pts',(20.4521296888376,20.084259855219,39.9826451868081));
#48808=CARTESIAN_POINT('Ctrl Pts',(20.2112119950715,20.0694446065732,40.0191449631258));
#48809=CARTESIAN_POINT('Ctrl Pts',(20.1328135344972,20.0645732723176,40.0261584024903));
#48810=CARTESIAN_POINT('Ctrl Pts',(20.0410869297276,20.0587099148586,40.0287371068022));
#48811=CARTESIAN_POINT('Ctrl Pts',(20.0279586103288,20.0578669399302,40.0289720748049));
#48812=CARTESIAN_POINT('Ctrl Pts',(20.0066417668936,20.0564915852999,40.0291359416528));
#48813=CARTESIAN_POINT('Ctrl Pts',(19.9984541510758,20.0559617457923,40.0291467547585));
#48814=CARTESIAN_POINT('Ctrl Pts',(19.9838806731041,20.0550157506369,40.0290732251716));
#48815=CARTESIAN_POINT('Ctrl Pts',(19.9774947933731,20.0546002345826,40.029009293605));
#48816=CARTESIAN_POINT('Ctrl Pts',(19.9640425569834,20.0537227763279,40.0288078107569));
#48817=CARTESIAN_POINT('Ctrl Pts',(19.9569764170965,20.0532606188512,40.028663132231));
#48818=CARTESIAN_POINT('Ctrl Pts',(19.9382845129511,20.0520346979228,40.0281776446066));
#48819=CARTESIAN_POINT('Ctrl Pts',(19.9266609056931,20.0512688880094,40.0277705251759));
#48820=CARTESIAN_POINT('Ctrl Pts',(19.8723227018726,20.0476721196193,40.0253751688434));
#48821=CARTESIAN_POINT('Ctrl Pts',(19.8296810551059,20.0448007543591,40.0220723192203));
#48822=CARTESIAN_POINT('Ctrl Pts',(19.621517706548,20.0305321820696,39.9989676574683));
#48823=CARTESIAN_POINT('Ctrl Pts',(19.4589481812864,20.0185212663477,39.9591858631507));
#48824=CARTESIAN_POINT('Ctrl Pts',(19.2343013014001,20.0014495686247,39.8722196713413));
#48825=CARTESIAN_POINT('Ctrl Pts',(19.166646686512,19.9962550564477,39.8414310083441));
#48826=CARTESIAN_POINT('Ctrl Pts',(19.0927234829816,19.9906402366373,39.8024916717616));
#48827=CARTESIAN_POINT('Ctrl Pts',(19.0845489837594,19.9900202472735,39.7981101307208));
#48828=CARTESIAN_POINT('Ctrl Pts',(19.0724316744723,19.9891029190971,39.7915023064882));
#48829=CARTESIAN_POINT('Ctrl Pts',(19.0684647368697,19.9888028796957,39.7893209008237));
#48830=CARTESIAN_POINT('Ctrl Pts',(19.0616156964443,19.9882853745138,39.7855231751664));
#48831=CARTESIAN_POINT('Ctrl Pts',(19.0587300356605,19.9880675005104,39.783913397426));
#48832=CARTESIAN_POINT('Ctrl Pts',(19.0558353878591,19.9878491161366,39.7822888403319));
#48833=CARTESIAN_POINT('Ctrl Pts',(19.0558223181413,19.9878481301057,39.7822815050415));
#48834=CARTESIAN_POINT('Ctrl Pts',(19.0557964587149,19.9878461791754,39.7822669912174));
#48835=CARTESIAN_POINT('Ctrl Pts',(19.0557836688964,19.9878452142677,39.7822598126307));
#48836=CARTESIAN_POINT('Ctrl Pts',(19.0557583637688,19.9878433051685,39.7822456091527));
#48837=CARTESIAN_POINT('Ctrl Pts',(19.055745848148,19.9878423609534,39.7822385840945));
#48838=CARTESIAN_POINT('Ctrl Pts',(19.055721083711,19.9878404926579,39.782224683373));
#48839=CARTESIAN_POINT('Ctrl Pts',(19.0557088356575,19.9878395686349,39.7822178081456));
#48840=CARTESIAN_POINT('Ctrl Pts',(19.0556846016916,19.9878377403712,39.7822042044908));
#48841=CARTESIAN_POINT('Ctrl Pts',(19.0556726156993,19.9878368361244,39.7821974760261));
#48842=CARTESIAN_POINT('Ctrl Pts',(19.0556488995763,19.9878350469392,39.7821841623941));
#48843=CARTESIAN_POINT('Ctrl Pts',(19.0556371695779,19.9878341620105,39.7821775773081));
#48844=CARTESIAN_POINT('Ctrl Pts',(19.0556149503129,19.9878324857611,39.782165103363));
#48845=CARTESIAN_POINT('Ctrl Pts',(19.0556044603603,19.987831694388,39.7821592141511));
#48846=CARTESIAN_POINT('Ctrl Pts',(19.055583533059,19.9878301156146,39.7821474650024));
#48847=CARTESIAN_POINT('Ctrl Pts',(19.0555730956278,19.987829328208,39.7821416050206));
#48848=CARTESIAN_POINT('Ctrl Pts',(19.0555522720801,19.9878277572705,39.7821299136122));
#48849=CARTESIAN_POINT('Ctrl Pts',(19.0555418865022,19.98782697378,39.7821240824892));
#48850=CARTESIAN_POINT('Ctrl Pts',(19.0555211666731,19.9878254106755,39.7821124488089));
#48851=CARTESIAN_POINT('Ctrl Pts',(19.0555108325336,19.9878246310698,39.7821066463156));
#48852=CARTESIAN_POINT('Ctrl Pts',(19.0554902167756,19.9878230758247,39.782095070569));
#48853=CARTESIAN_POINT('Ctrl Pts',(19.0554799345472,19.9878223001394,39.7820892969745));
#48854=CARTESIAN_POINT('Ctrl Pts',(19.0554594193368,19.9878207524879,39.7820777771905));
#48855=CARTESIAN_POINT('Ctrl Pts',(19.0554491873856,19.9878199805995,39.782072031581));
#48856=CARTESIAN_POINT('Ctrl Pts',(19.0519432002418,19.9875554930758,39.7801032513371));
#48857=CARTESIAN_POINT('Ctrl Pts',(19.0484535323508,19.9872924769294,39.7781293011416));
#48858=CARTESIAN_POINT('Ctrl Pts',(19.0388907116957,19.9865723168476,39.772680617711));
#48859=CARTESIAN_POINT('Ctrl Pts',(19.0328301950448,19.9861165644643,39.7691836582528));
#48860=CARTESIAN_POINT('Ctrl Pts',(19.0193217612953,19.9851018868962,39.7612909253694));
#48861=CARTESIAN_POINT('Ctrl Pts',(19.0118840577534,19.9845440034456,39.756877858411));
#48862=CARTESIAN_POINT('Ctrl Pts',(18.9889695117246,19.9828269030545,39.7430726218083));
#48863=CARTESIAN_POINT('Ctrl Pts',(18.9735945575059,19.9816771439145,39.7335122307388));
#48864=CARTESIAN_POINT('Ctrl Pts',(18.9140856136334,19.977226997675,39.6953366130109));
#48865=CARTESIAN_POINT('Ctrl Pts',(18.8709918687905,19.9740041243062,39.6651359170821));
#48866=CARTESIAN_POINT('Ctrl Pts',(18.7189588231242,19.962428226304,39.5490377515313));
#48867=CARTESIAN_POINT('Ctrl Pts',(18.6181340363325,19.9543162195343,39.4532273600515));
#48868=CARTESIAN_POINT('Ctrl Pts',(18.4863238528572,19.9418282736787,39.2977360580864));
#48869=CARTESIAN_POINT('Ctrl Pts',(18.4467441915504,19.9377662233058,39.2459416007988));
#48870=CARTESIAN_POINT('Ctrl Pts',(18.4027813614186,19.9328005428525,39.1819388202106));
#48871=CARTESIAN_POINT('Ctrl Pts',(18.3958004422882,19.9319970485034,39.1715608976178));
#48872=CARTESIAN_POINT('Ctrl Pts',(18.384521403601,19.9306735365962,39.1544360768183));
#48873=CARTESIAN_POINT('Ctrl Pts',(18.3801633899499,19.9301557493874,39.147728919658));
#48874=CARTESIAN_POINT('Ctrl Pts',(18.3724121512867,19.9292230926605,39.135635493439));
#48875=CARTESIAN_POINT('Ctrl Pts',(18.3690036191451,19.9288087951847,39.1302591346693));
#48876=CARTESIAN_POINT('Ctrl Pts',(18.3618081080542,19.9279252062136,39.1187842824862));
#48877=CARTESIAN_POINT('Ctrl Pts',(18.3580284432119,19.9274556550819,39.1126813385448));
#48878=CARTESIAN_POINT('Ctrl Pts',(18.347952775824,19.9261891543135,39.0962076674093));
#48879=CARTESIAN_POINT('Ctrl Pts',(18.3417204808408,19.9253899101199,39.0857985455884));
#48880=CARTESIAN_POINT('Ctrl Pts',(18.3109722631222,19.9213653498243,39.0333264016633));
#48881=CARTESIAN_POINT('Ctrl Pts',(18.2879586301262,19.9180869924393,38.9904080509311));
#48882=CARTESIAN_POINT('Ctrl Pts',(18.1937215998474,19.9033946155962,38.7974741855524));
#48883=CARTESIAN_POINT('Ctrl Pts',(18.1404230227594,19.8914011227261,38.6395083032005));
#48884=CARTESIAN_POINT('Ctrl Pts',(18.101595012653,19.8773424045315,38.4444994512527));
#48885=CARTESIAN_POINT('Ctrl Pts',(18.0960045662866,19.8750354701613,38.4121264920453));
#48886=CARTESIAN_POINT('Ctrl Pts',(18.0874485233809,19.870937757559,38.3537218757529));
#48887=CARTESIAN_POINT('Ctrl Pts',(18.0841812655951,19.8691376835596,38.3277425383711));
#48888=CARTESIAN_POINT('Ctrl Pts',(18.0798398901284,19.8663202441359,38.2864483784812));
#48889=CARTESIAN_POINT('Ctrl Pts',(18.0784180241057,19.8652875669206,38.2711741556486));
#48890=CARTESIAN_POINT('Ctrl Pts',(18.0767161523157,19.8638827102765,38.2501816528894));
#48891=CARTESIAN_POINT('Ctrl Pts',(18.0762792202875,19.8635024160761,38.2444771656254));
#48892=CARTESIAN_POINT('Ctrl Pts',(18.0756237848887,19.862898973685,38.2353891940913));
#48893=CARTESIAN_POINT('Ctrl Pts',(18.0753888167711,19.8626749270359,38.2320069884387));
#48894=CARTESIAN_POINT('Ctrl Pts',(18.0749368562799,19.8622279809938,38.2252434810152));
#48895=CARTESIAN_POINT('Ctrl Pts',(18.0747198550971,19.8620050866324,38.2218622200099));
#48896=CARTESIAN_POINT('Ctrl Pts',(18.0742918900555,19.8615476980728,38.2149071306376));
#48897=CARTESIAN_POINT('Ctrl Pts',(18.0740819632888,19.8613132609208,38.2113332374332));
#48898=CARTESIAN_POINT('Ctrl Pts',(18.0736138254768,19.8607657116984,38.2029655762043));
#48899=CARTESIAN_POINT('Ctrl Pts',(18.07336355577,19.860453029011,38.1981713615322));
#48900=CARTESIAN_POINT('Ctrl Pts',(18.0725608731067,19.8593761387495,38.1816075671736));
#48901=CARTESIAN_POINT('Ctrl Pts',(18.072098377572,19.8586166108388,38.1698336116703));
#48902=CARTESIAN_POINT('Ctrl Pts',(18.0711698321106,19.856640967472,38.1389930577971));
#48903=CARTESIAN_POINT('Ctrl Pts',(18.070878585341,19.8554331419902,38.1199221704454));
#48904=CARTESIAN_POINT('Ctrl Pts',(18.0708701870214,19.8542362730884,38.1008494569394));
#48905=CARTESIAN_POINT('Ctrl Pts',(18.0708701880617,19.854236421143,38.1008518162642));
#48906=CARTESIAN_POINT('Ctrl Pts',(18.0708091100297,19.8455561160718,37.9625268542006));
#48907=CARTESIAN_POINT('Ctrl Pts',(18.0856255279444,19.8374582510131,37.8245739329577));
#48908=CARTESIAN_POINT('Ctrl Pts',(18.1392321285082,19.8223474198742,37.5785004745513));
#48909=CARTESIAN_POINT('Ctrl Pts',(18.1731169954809,19.81543300587,37.4699905304631));
#48910=CARTESIAN_POINT('Ctrl Pts',(18.221990390201,19.8072380567716,37.351371453203));
#48911=CARTESIAN_POINT('Ctrl Pts',(18.2278029484105,19.8062848414889,37.3377136599847));
#48912=CARTESIAN_POINT('Ctrl Pts',(18.2368941054824,19.8048250838618,37.3170182590075));
#48913=CARTESIAN_POINT('Ctrl Pts',(18.2400586284611,19.8043224026619,37.3099309094431));
#48914=CARTESIAN_POINT('Ctrl Pts',(18.2458887641138,19.8034059624922,37.2970824306239));
#48915=CARTESIAN_POINT('Ctrl Pts',(18.2485402184746,19.8029926909948,37.2913149666476));
#48916=CARTESIAN_POINT('Ctrl Pts',(18.2543217979133,19.8020989806512,37.2789006458326));
#48917=CARTESIAN_POINT('Ctrl Pts',(18.2574615171412,19.8016182177089,37.272258393035));
#48918=CARTESIAN_POINT('Ctrl Pts',(18.2660729604281,19.8003117563123,37.2543065425659));
#48919=CARTESIAN_POINT('Ctrl Pts',(18.2716172731191,19.7994835666037,37.2430323580796));
#48920=CARTESIAN_POINT('Ctrl Pts',(18.2992494156332,19.7954173258601,37.1882023421582));
#48921=CARTESIAN_POINT('Ctrl Pts',(18.3228738648243,19.7921261874945,37.1454452756538));
#48922=CARTESIAN_POINT('Ctrl Pts',(18.362825455119,19.7868291677138,37.0792082988996));
#48923=CARTESIAN_POINT('Ctrl Pts',(18.3780970858714,19.7848587384307,37.055113882836));
#48924=CARTESIAN_POINT('Ctrl Pts',(18.4811127871359,19.7719141658629,36.9002861888563));
#48925=CARTESIAN_POINT('Ctrl Pts',(18.5840357248168,19.7604827095395,36.7803905230257));
#48926=CARTESIAN_POINT('Ctrl Pts',(18.7245931820472,19.7471767133356,36.652258960152));
#48927=CARTESIAN_POINT('Ctrl Pts',(18.7493737309762,19.7449067313305,36.6307992433851));
#48928=CARTESIAN_POINT('Ctrl Pts',(18.7848481676727,19.7417745606744,36.6016270374404));
#48929=CARTESIAN_POINT('Ctrl Pts',(18.7950913406793,19.740883366401,36.593377733195));
#48930=CARTESIAN_POINT('Ctrl Pts',(18.8108271566163,19.7395352653638,36.5809680863722));
#48931=CARTESIAN_POINT('Ctrl Pts',(18.8162588305159,19.7390736745732,36.576731522965));
#48932=CARTESIAN_POINT('Ctrl Pts',(18.8252127795837,19.7383190380686,36.569824494193));
#48933=CARTESIAN_POINT('Ctrl Pts',(18.8287216918494,19.7380248766503,36.5671369214369));
#48934=CARTESIAN_POINT('Ctrl Pts',(18.835507601989,19.7374590636384,36.5619763117143));
#48935=CARTESIAN_POINT('Ctrl Pts',(18.8387833144664,19.7371873014419,36.5595016323373));
#48936=CARTESIAN_POINT('Ctrl Pts',(18.8420791353039,19.7369152622612,36.5570282477525));
#48937=CARTESIAN_POINT('Ctrl Pts',(18.8420913312268,19.7369142556209,36.5570190954155));
#48938=CARTESIAN_POINT('Ctrl Pts',(18.8421158820842,19.7369122292541,36.5570006718676));
#48939=CARTESIAN_POINT('Ctrl Pts',(18.8421282370558,19.736911209525,36.5569914006348));
#48940=CARTESIAN_POINT('Ctrl Pts',(18.8421531089581,19.7369091567387,36.556972737101));
#48941=CARTESIAN_POINT('Ctrl Pts',(18.8421656259683,19.7369081236756,36.5569633447467));
#48942=CARTESIAN_POINT('Ctrl Pts',(18.8421908252211,19.7369060439525,36.5569444365321));
#48943=CARTESIAN_POINT('Ctrl Pts',(18.8422035072118,19.736904997314,36.5569349208673));
#48944=CARTESIAN_POINT('Ctrl Pts',(18.8422290394414,19.7369028901931,36.5569157637882));
#48945=CARTESIAN_POINT('Ctrl Pts',(18.8422418897859,19.7369018297025,36.5569061223012));
#48946=CARTESIAN_POINT('Ctrl Pts',(18.8422677614208,19.7368996946565,36.5568867115732));
#48947=CARTESIAN_POINT('Ctrl Pts',(18.8422807834257,19.7368986200426,36.5568769418029));
#48948=CARTESIAN_POINT('Ctrl Pts',(18.8423070023105,19.7368964564275,36.5568572715809));
#48949=CARTESIAN_POINT('Ctrl Pts',(18.8423201986639,19.7368953674703,36.5568473715311));
#48950=CARTESIAN_POINT('Ctrl Pts',(18.8423467697354,19.7368931748822,36.556827438153));
#48951=CARTESIAN_POINT('Ctrl Pts',(18.8423601443966,19.7368920712567,36.5568174048746));
#48952=CARTESIAN_POINT('Ctrl Pts',(18.8423870753308,19.7368898490659,36.556797202625));
#48953=CARTESIAN_POINT('Ctrl Pts',(18.8424006316561,19.736888730497,36.5567870336221));
#48954=CARTESIAN_POINT('Ctrl Pts',(18.8424279292402,19.7368864781472,36.5567665574541));
#48955=CARTESIAN_POINT('Ctrl Pts',(18.8424416708629,19.736885344337,36.5567562500238));
#48956=CARTESIAN_POINT('Ctrl Pts',(18.8424693430418,19.7368830611766,36.556735494024));
#48957=CARTESIAN_POINT('Ctrl Pts',(18.842483273294,19.7368819118521,36.5567250456905));
#48958=CARTESIAN_POINT('Ctrl Pts',(18.842511326397,19.7368795973629,36.556704005159));
#48959=CARTESIAN_POINT('Ctrl Pts',(18.8425254494117,19.7368784321852,36.5566934128463));
#48960=CARTESIAN_POINT('Ctrl Pts',(18.8425538919978,19.7368760856652,36.5566720814127));
#48961=CARTESIAN_POINT('Ctrl Pts',(18.8425682113416,19.7368749043422,36.556661342471));
#48962=CARTESIAN_POINT('Ctrl Pts',(18.8425970504491,19.736872525215,36.5566397149077));
#48963=CARTESIAN_POINT('Ctrl Pts',(18.8426115703182,19.7368713274027,36.5566288262158));
#48964=CARTESIAN_POINT('Ctrl Pts',(18.8453866452453,19.7366424035945,36.5545478124496));
#48965=CARTESIAN_POINT('Ctrl Pts',(18.8481527114923,19.7364152045513,36.5524851253677));
#48966=CARTESIAN_POINT('Ctrl Pts',(18.8545696927986,19.7358903763614,36.5477266465612));
#48967=CARTESIAN_POINT('Ctrl Pts',(18.8582245929671,19.7355931248567,36.5450363112323));
#48968=CARTESIAN_POINT('Ctrl Pts',(18.869422791922,19.734687365083,36.5368541997474));
#48969=CARTESIAN_POINT('Ctrl Pts',(18.876996605687,19.7340816388856,36.531404130722));
#48970=CARTESIAN_POINT('Ctrl Pts',(18.9507572628083,19.728245639569,36.4791345080919));
#48971=CARTESIAN_POINT('Ctrl Pts',(19.0198030212804,19.7232704718756,36.4364698257077));
#48972=CARTESIAN_POINT('Ctrl Pts',(19.1884639327844,19.7117301072578,36.3464108328363));
#48973=CARTESIAN_POINT('Ctrl Pts',(19.2897609130543,19.7052518514458,36.3030075020567));
#48974=CARTESIAN_POINT('Ctrl Pts',(19.3941041453486,19.6985952145508,36.2684889380033));
#48975=CARTESIAN_POINT('Ctrl Pts',(19.3941040005193,19.5258959448669,36.2684889859154));
#48976=CARTESIAN_POINT('Ctrl Pts',(19.3415821206899,19.5292445953932,36.2858641458948));
#48977=CARTESIAN_POINT('Ctrl Pts',(19.2898298048738,19.5326322553754,36.3054911807356));
#48978=CARTESIAN_POINT('Ctrl Pts',(19.2030432776394,19.5385283134163,36.3427484989325));
#48979=CARTESIAN_POINT('Ctrl Pts',(19.1675765517045,19.5410017085718,36.3592691986031));
#48980=CARTESIAN_POINT('Ctrl Pts',(19.1225592024759,19.5442361646493,36.3819291247166));
#48981=CARTESIAN_POINT('Ctrl Pts',(19.1125249506485,19.5449633252282,36.3870908040291));
#48982=CARTESIAN_POINT('Ctrl Pts',(19.0963482812722,19.5461459791928,36.395592477484));
#48983=CARTESIAN_POINT('Ctrl Pts',(19.0901776263136,19.5465995749868,36.3988784059397));
#48984=CARTESIAN_POINT('Ctrl Pts',(19.0783873460837,19.547471069662,36.405239336154));
#48985=CARTESIAN_POINT('Ctrl Pts',(19.072764899316,19.5478887734634,36.4083089354191));
#48986=CARTESIAN_POINT('Ctrl Pts',(19.0599800054246,19.548843476423,36.4153717879625));
#48987=CARTESIAN_POINT('Ctrl Pts',(19.0528275613209,19.5493811013265,36.4193828006046));
#48988=CARTESIAN_POINT('Ctrl Pts',(19.033995280774,19.5508061143219,36.4301021416205));
#48989=CARTESIAN_POINT('Ctrl Pts',(19.0223599220834,19.5516962364436,36.4368873046387));
#48990=CARTESIAN_POINT('Ctrl Pts',(18.9346299025045,19.5584828628202,36.4892858555637));
#48991=CARTESIAN_POINT('Ctrl Pts',(18.8617032176302,19.564564300891,36.5399712077307));
#48992=CARTESIAN_POINT('Ctrl Pts',(18.6674534305352,19.5820293040815,36.6958692655711));
#48993=CARTESIAN_POINT('Ctrl Pts',(18.5553910253139,19.5937053146319,36.8114485461492));
#48994=CARTESIAN_POINT('Ctrl Pts',(18.4395692318108,19.6070058566656,36.9652605107531));
#48995=CARTESIAN_POINT('Ctrl Pts',(18.4208584871502,19.6091999753845,36.9914467660389));
#48996=CARTESIAN_POINT('Ctrl Pts',(18.3987803971043,19.6118348490982,37.0240399752427));
#48997=CARTESIAN_POINT('Ctrl Pts',(18.3947836363795,19.6123137718489,37.0300118591568));
#48998=CARTESIAN_POINT('Ctrl Pts',(18.3885648676515,19.6130618423814,37.0394170974552));
#48999=CARTESIAN_POINT('Ctrl Pts',(18.3863202999148,19.6133324481579,37.042835346201));
#49000=CARTESIAN_POINT('Ctrl Pts',(18.3821382779975,19.6138377269317,37.0492484937209));
#49001=CARTESIAN_POINT('Ctrl Pts',(18.3801982817636,19.6140725619882,37.0522415959099));
#49002=CARTESIAN_POINT('Ctrl Pts',(18.3757683865344,19.6146098364044,37.0591179217868));
#49003=CARTESIAN_POINT('Ctrl Pts',(18.3732841087053,19.6149119041044,37.0630047034698));
#49004=CARTESIAN_POINT('Ctrl Pts',(18.3667952438504,19.6157030217426,37.0732375691009));
#49005=CARTESIAN_POINT('Ctrl Pts',(18.3628136534178,19.6161906073289,37.0795982477356));
#49006=CARTESIAN_POINT('Ctrl Pts',(18.3354870599342,19.6195532597479,37.1238247995337));
#49007=CARTESIAN_POINT('Ctrl Pts',(18.3134186791527,19.6223520812968,37.1624683940899));
#49008=CARTESIAN_POINT('Ctrl Pts',(18.2330347889182,19.6330253904887,37.3152692855635));
#49009=CARTESIAN_POINT('Ctrl Pts',(18.184812631099,19.6405369101579,37.4343663126572));
#49010=CARTESIAN_POINT('Ctrl Pts',(18.1215139347474,19.6540652691665,37.6503183865293));
#49011=CARTESIAN_POINT('Ctrl Pts',(18.1013118793282,19.6599757960112,37.7451712908246));
#49012=CARTESIAN_POINT('Ctrl Pts',(18.0854535891291,19.6674709217803,37.8622815225971));
#49013=CARTESIAN_POINT('Ctrl Pts',(18.0829409932539,19.6688346858568,37.8834757729418));
#49014=CARTESIAN_POINT('Ctrl Pts',(18.0798714525872,19.6707878959632,37.913641282179));
#49015=CARTESIAN_POINT('Ctrl Pts',(18.0790247131448,19.67136831644,37.9225819819815));
#49016=CARTESIAN_POINT('Ctrl Pts',(18.0776719661654,19.6723728088424,37.9380127757344));
#49017=CARTESIAN_POINT('Ctrl Pts',(18.0771363197066,19.6727959510853,37.9445001743605));
#49018=CARTESIAN_POINT('Ctrl Pts',(18.0761735484981,19.6736081609936,37.9569272801874));
#49019=CARTESIAN_POINT('Ctrl Pts',(18.0757410718514,19.6739970569009,37.9628665075173));
#49020=CARTESIAN_POINT('Ctrl Pts',(18.0746874911003,19.6750110646436,37.9783231088647));
#49021=CARTESIAN_POINT('Ctrl Pts',(18.074109462834,19.6756375087594,37.9878431629173));
#49022=CARTESIAN_POINT('Ctrl Pts',(18.0723734082309,19.6777884155946,38.0204285011433));
#49023=CARTESIAN_POINT('Ctrl Pts',(18.0715590161227,19.6793234654075,38.0435093447891));
#49024=CARTESIAN_POINT('Ctrl Pts',(18.071058997622,19.6812590414813,38.0723839147349));
#49025=CARTESIAN_POINT('Ctrl Pts',(18.070984842271,19.6816476510426,38.0781697719728));
#49026=CARTESIAN_POINT('Ctrl Pts',(18.0708898030658,19.6824166638025,38.0895967615056));
#49027=CARTESIAN_POINT('Ctrl Pts',(18.0708676302825,19.6827970246205,38.0952378284071));
#49028=CARTESIAN_POINT('Ctrl Pts',(18.0708935746107,19.686644300265,38.152186426451));
#49029=CARTESIAN_POINT('Ctrl Pts',(18.0729637986998,19.6901702229334,38.2034684945277));
#49030=CARTESIAN_POINT('Ctrl Pts',(18.0884522498189,19.7036367555213,38.3961104757965));
#49031=CARTESIAN_POINT('Ctrl Pts',(18.115415396985,19.7139011109103,38.535925591211));
#49032=CARTESIAN_POINT('Ctrl Pts',(18.161471180383,19.7248559260875,38.6844118298183));
#49033=CARTESIAN_POINT('Ctrl Pts',(18.1656128373047,19.7258057191734,38.6972848213081));
#49034=CARTESIAN_POINT('Ctrl Pts',(18.185042950921,19.7301034287197,38.7555678423087));
#49035=CARTESIAN_POINT('Ctrl Pts',(18.2018860133886,19.7334060511824,38.8004464683576));
#49036=CARTESIAN_POINT('Ctrl Pts',(18.2233426233009,19.7371362810372,38.8517245833627));
#49037=CARTESIAN_POINT('Ctrl Pts',(18.2263428677531,19.737648289919,38.8587764265059));
#49038=CARTESIAN_POINT('Ctrl Pts',(18.2312154145351,19.7384644687757,38.8700421451077));
#49039=CARTESIAN_POINT('Ctrl Pts',(18.2330609028965,19.738770177474,38.8742674235953));
#49040=CARTESIAN_POINT('Ctrl Pts',(18.2363643522775,19.7393113239191,38.8817574061843));
#49041=CARTESIAN_POINT('Ctrl Pts',(18.2378162608873,19.739547121543,38.8850247196504));
#49042=CARTESIAN_POINT('Ctrl Pts',(18.2409294047999,19.7400483717136,38.8919782478189));
#49043=CARTESIAN_POINT('Ctrl Pts',(18.2425931447712,19.7403136693292,38.8956632766784));
#49044=CARTESIAN_POINT('Ctrl Pts',(18.2471592623024,19.7410348582048,38.9056926077548));
#49045=CARTESIAN_POINT('Ctrl Pts',(18.2500845247922,19.7414893798912,38.9120265163091));
#49046=CARTESIAN_POINT('Ctrl Pts',(18.2654584674742,19.7438403373042,38.9448459440278));
#49047=CARTESIAN_POINT('Ctrl Pts',(18.2784750561068,19.7457042208986,38.9710631953126));
#49048=CARTESIAN_POINT('Ctrl Pts',(18.319441590841,19.7512370663827,39.0490668617792));
#49049=CARTESIAN_POINT('Ctrl Pts',(18.3491702436532,19.7548246984331,39.0998833324394));
#49050=CARTESIAN_POINT('Ctrl Pts',(18.4344010093902,19.7642704127695,39.2313787042275));
#49051=CARTESIAN_POINT('Ctrl Pts',(18.4937949076322,19.7700488225071,39.309324021222));
#49052=CARTESIAN_POINT('Ctrl Pts',(18.622213014459,19.781706017784,39.4536364447325));
#49053=CARTESIAN_POINT('Ctrl Pts',(18.6907615680156,19.7875628712116,39.5200421428112));
#49054=CARTESIAN_POINT('Ctrl Pts',(18.774362896092,19.7945163249079,39.5898123688211));
#49055=CARTESIAN_POINT('Ctrl Pts',(18.7848870767143,19.7953883147591,39.598408413382));
#49056=CARTESIAN_POINT('Ctrl Pts',(18.8019339523593,19.7967959128715,39.6120344328661));
#49057=CARTESIAN_POINT('Ctrl Pts',(18.8083997034176,19.7973287066942,39.6171351655042));
#49058=CARTESIAN_POINT('Ctrl Pts',(18.8199563959602,19.7982791709333,39.6261326118605));
#49059=CARTESIAN_POINT('Ctrl Pts',(18.8250345054307,19.7986961905141,39.6300456664229));
#49060=CARTESIAN_POINT('Ctrl Pts',(18.835677278457,19.799568944179,39.6381624729912));
#49061=CARTESIAN_POINT('Ctrl Pts',(18.8412454124866,19.800024854218,39.6423615001005));
#49062=CARTESIAN_POINT('Ctrl Pts',(18.8558202165034,19.801216472131,39.6532291426539));
#49063=CARTESIAN_POINT('Ctrl Pts',(18.8648623394408,19.8019540254815,39.6598495533795));
#49064=CARTESIAN_POINT('Ctrl Pts',(18.9051018102497,19.8052292014499,39.6887766880532));
#49065=CARTESIAN_POINT('Ctrl Pts',(18.9369007395075,19.8077989400824,39.7102276291891));
#49066=CARTESIAN_POINT('Ctrl Pts',(19.0245657006077,19.8148399622077,39.765635747505));
#49067=CARTESIAN_POINT('Ctrl Pts',(19.0815490398656,19.8193724898872,39.7977222544556));
#49068=CARTESIAN_POINT('Ctrl Pts',(19.2617839279286,19.8335409247069,39.8874772958144));
#49069=CARTESIAN_POINT('Ctrl Pts',(19.3895845625096,19.8433853497653,39.9350556206581));
#49070=CARTESIAN_POINT('Ctrl Pts',(19.5659714343517,19.8561071876829,39.9802356389194));
#49071=CARTESIAN_POINT('Ctrl Pts',(19.6110199764226,19.8592805851452,39.9900693603643));
#49072=CARTESIAN_POINT('Ctrl Pts',(19.6638448671375,19.8628825252023,39.9996314934443));
#49073=CARTESIAN_POINT('Ctrl Pts',(19.6713163084197,19.8633892156679,40.0009384839476));
#49074=CARTESIAN_POINT('Ctrl Pts',(19.6833189167202,19.8641985625954,40.0029652371825));
#49075=CARTESIAN_POINT('Ctrl Pts',(19.6878451888825,19.8645027181646,40.0037129451171));
#49076=CARTESIAN_POINT('Ctrl Pts',(19.6959009548881,19.865042120699,40.0050141969574));
#49077=CARTESIAN_POINT('Ctrl Pts',(19.6994293656359,19.8652777191444,40.0055740905056));
#49078=CARTESIAN_POINT('Ctrl Pts',(19.706968132521,19.865779676766,40.0067488932045));
#49079=CARTESIAN_POINT('Ctrl Pts',(19.7109788724427,19.8660458751868,40.0073609531684));
#49080=CARTESIAN_POINT('Ctrl Pts',(19.721954165511,19.8667720685376,40.0090004270416));
#49081=CARTESIAN_POINT('Ctrl Pts',(19.7289225441078,19.8672306616814,40.010002390879));
#49082=CARTESIAN_POINT('Ctrl Pts',(19.765725932666,19.8696403904388,40.0150887749485));
#49083=CARTESIAN_POINT('Ctrl Pts',(19.7956499520157,19.8715570059891,40.018512615742));
#49084=CARTESIAN_POINT('Ctrl Pts',(19.9869626806524,19.8836089350197,40.0358746570323));
#49085=CARTESIAN_POINT('Ctrl Pts',(20.1494994290245,19.8929832748013,40.0301406576609));
#49086=CARTESIAN_POINT('Ctrl Pts',(20.3977273971722,19.9081959553671,39.9898040293313));
#49087=CARTESIAN_POINT('Ctrl Pts',(20.4849169449891,19.9137085849372,39.9693311039662));
#49088=CARTESIAN_POINT('Ctrl Pts',(20.5832092666239,19.9202802811138,39.9389100845173));
#49089=CARTESIAN_POINT('Ctrl Pts',(20.5960118125928,19.9211432375117,39.9348006028424));
#49090=CARTESIAN_POINT('Ctrl Pts',(20.6165449315399,19.9225390460061,39.9279721107334));
#49091=CARTESIAN_POINT('Ctrl Pts',(20.624303111645,19.923069159575,39.9253370405521));
#49092=CARTESIAN_POINT('Ctrl Pts',(20.6380955101542,19.9240165587032,39.920554228504));
#49093=CARTESIAN_POINT('Ctrl Pts',(20.6441362981052,19.9244332082163,39.9184256946104));
#49094=CARTESIAN_POINT('Ctrl Pts',(20.6567515355234,19.9253069475784,39.9139098377531));
#49095=CARTESIAN_POINT('Ctrl Pts',(20.6633238139053,19.9257642221371,39.9115167663185));
#49096=CARTESIAN_POINT('Ctrl Pts',(20.6804791100472,19.9269633364443,39.9051643729277));
#49097=CARTESIAN_POINT('Ctrl Pts',(20.6910404864623,19.9277070649088,39.9011477644518));
#49098=CARTESIAN_POINT('Ctrl Pts',(20.7381502318148,19.9310497413131,39.8827560705485));
#49099=CARTESIAN_POINT('Ctrl Pts',(20.7742875464824,19.9336824605317,39.8673605705435));
#49100=CARTESIAN_POINT('Ctrl Pts',(20.9586846468133,19.947486442863,39.7820612650716));
#49101=CARTESIAN_POINT('Ctrl Pts',(21.098046650583,19.9592630111454,39.6945789253741));
#49102=CARTESIAN_POINT('Ctrl Pts',(21.2872933814515,19.9766579990536,39.5390943181407));
#49103=CARTESIAN_POINT('Ctrl Pts',(21.3466424930026,19.9823494276627,39.4837174323383));
#49104=CARTESIAN_POINT('Ctrl Pts',(21.4087448344611,19.9884273640325,39.4179786229729));
#49105=CARTESIAN_POINT('Ctrl Pts',(21.415104696274,19.9890513113821,39.4111477286774));
#49106=CARTESIAN_POINT('Ctrl Pts',(21.4244834570584,19.9899733372056,39.4009266071075));
#49107=CARTESIAN_POINT('Ctrl Pts',(21.4275402531487,19.9902741559051,39.3975715715132));
#49108=CARTESIAN_POINT('Ctrl Pts',(21.4329734857427,19.9908093357816,39.391565801319));
#49109=CARTESIAN_POINT('Ctrl Pts',(21.4353544462621,19.9910440322346,39.3889192543719));
#49110=CARTESIAN_POINT('Ctrl Pts',(21.4404879009132,19.9915504073736,39.3831813185249));
#49111=CARTESIAN_POINT('Ctrl Pts',(21.443237770038,19.9918218920406,39.3800876645061));
#49112=CARTESIAN_POINT('Ctrl Pts',(21.4508849322831,19.9925775974396,39.3714284987859));
#49113=CARTESIAN_POINT('Ctrl Pts',(21.4557601979659,19.9930602198377,39.365843499257));
#49114=CARTESIAN_POINT('Ctrl Pts',(21.4839493924061,19.9958566650691,39.3331723083263));
#49115=CARTESIAN_POINT('Ctrl Pts',(21.5065409697201,19.9981214768895,39.3054685569875));
#49116=CARTESIAN_POINT('Ctrl Pts',(21.5782443308917,20.0054503343531,39.2123726570944));
#49117=CARTESIAN_POINT('Ctrl Pts',(21.623972727932,20.0103583263228,39.1444821263853));
#49118=CARTESIAN_POINT('Ctrl Pts',(21.7421847579459,20.024357512336,38.9423508726343));
#49119=CARTESIAN_POINT('Ctrl Pts',(21.803247398264,20.0333955004431,38.8021789440624));
#49120=CARTESIAN_POINT('Ctrl Pts',(21.853459103103,20.0444291324234,38.6354490173847));
#49121=CARTESIAN_POINT('Ctrl Pts',(21.8593821209898,20.045818910604,38.6145039983423));
#49122=CARTESIAN_POINT('Ctrl Pts',(21.8670944600564,20.0477599354255,38.5853567367578));
#49123=CARTESIAN_POINT('Ctrl Pts',(21.8691866933235,20.0483014836361,38.5772357766965));
#49124=CARTESIAN_POINT('Ctrl Pts',(21.8726968802224,20.049236598572,38.5632337919081));
#49125=CARTESIAN_POINT('Ctrl Pts',(21.8741402553103,20.0496293479759,38.5573592168126));
#49126=CARTESIAN_POINT('Ctrl Pts',(21.8770639289843,20.0504422681274,38.5452135230475));
#49127=CARTESIAN_POINT('Ctrl Pts',(21.8785404849612,20.0508625526628,38.5389415898211));
#49128=CARTESIAN_POINT('Ctrl Pts',(21.8819128338881,20.0518457017517,38.5242882093645));
#49129=CARTESIAN_POINT('Ctrl Pts',(21.8837840890325,20.0524093391408,38.5159013114189));
#49130=CARTESIAN_POINT('Ctrl Pts',(21.8896380575043,20.0542329007129,38.4888137629913));
#49131=CARTESIAN_POINT('Ctrl Pts',(21.8933987025167,20.0554998165771,38.4700668040557));
#49132=CARTESIAN_POINT('Ctrl Pts',(21.911171544734,20.0620125854446,38.3740916890476));
#49133=CARTESIAN_POINT('Ctrl Pts',(21.9207381032398,20.0673959068206,38.2961255799988));
#49134=CARTESIAN_POINT('Ctrl Pts',(21.9306229199611,20.0787271659919,38.1345535081039));
#49135=CARTESIAN_POINT('Ctrl Pts',(21.9303115787479,20.084678053253,38.051066871815));
#49136=CARTESIAN_POINT('Ctrl Pts',(21.917104114957,20.0984356395888,37.8586905182416));
#49137=CARTESIAN_POINT('Ctrl Pts',(21.9003312084986,20.1062212347068,37.7503350490334));
#49138=CARTESIAN_POINT('Ctrl Pts',(21.8722890258634,20.114191667664,37.6350694819463));
#49139=CARTESIAN_POINT('Ctrl Pts',(21.8700586465307,20.1148043648038,37.6261780401029));
#49140=CARTESIAN_POINT('Ctrl Pts',(21.8666375294097,20.1157130354577,37.6129402583701));
#49141=CARTESIAN_POINT('Ctrl Pts',(21.8654948446682,20.1160116370992,37.6085818036971));
#49142=CARTESIAN_POINT('Ctrl Pts',(21.8634226611789,20.1165444256061,37.6007894254387));
#49143=CARTESIAN_POINT('Ctrl Pts',(21.8624989279312,20.1167789354115,37.5973540449845));
#49144=CARTESIAN_POINT('Ctrl Pts',(21.8604735363488,20.117286685113,37.5899038236642));
#49145=CARTESIAN_POINT('Ctrl Pts',(21.859368385821,20.1175597214878,37.5858899969992));
#49146=CARTESIAN_POINT('Ctrl Pts',(21.8562295404201,20.1183241383047,37.5746324558864));
#49147=CARTESIAN_POINT('Ctrl Pts',(21.8541664229512,20.1188138602521,37.56739691733));
#49148=CARTESIAN_POINT('Ctrl Pts',(21.8415293831332,20.121739770149,37.524041194732));
#49149=CARTESIAN_POINT('Ctrl Pts',(21.8299418049666,20.1241214935229,37.4882218869513));
#49150=CARTESIAN_POINT('Ctrl Pts',(21.7619906241205,20.1367294843981,37.2974288475974));
#49151=CARTESIAN_POINT('Ctrl Pts',(21.6869784015494,20.1462552807949,37.1498179120137));
#49152=CARTESIAN_POINT('Ctrl Pts',(21.5497478396496,20.1610698670012,36.9484684581051));
#49153=CARTESIAN_POINT('Ctrl Pts',(21.5014625468668,20.1659470288155,36.886183209152));
#49154=CARTESIAN_POINT('Ctrl Pts',(21.4408447232797,20.1718167945172,36.8171588075002));
#49155=CARTESIAN_POINT('Ctrl Pts',(21.4320780642923,20.1726599602635,36.8073796203603));
#49156=CARTESIAN_POINT('Ctrl Pts',(21.4176844586401,20.1740355706943,36.7916497462919));
#49157=CARTESIAN_POINT('Ctrl Pts',(21.4121181715104,20.1745654737412,36.7856439306882));
#49158=CARTESIAN_POINT('Ctrl Pts',(21.4021428979645,20.1755115474532,36.7750174954372));
#49159=CARTESIAN_POINT('Ctrl Pts',(21.3977488590059,20.1759270782182,36.7703829614419));
#49160=CARTESIAN_POINT('Ctrl Pts',(21.3884439932401,20.1768045315955,36.7606659184575));
#49161=CARTESIAN_POINT('Ctrl Pts',(21.3835280970315,20.1772666693066,36.7555884161321));
#49162=CARTESIAN_POINT('Ctrl Pts',(21.3704497934732,20.1784924544795,36.7422278713968));
#49163=CARTESIAN_POINT('Ctrl Pts',(21.3622402999766,20.1792581474768,36.7339915283004));
#49164=CARTESIAN_POINT('Ctrl Pts',(21.3235123683717,20.1828534046414,36.6958332537641));
#49165=CARTESIAN_POINT('Ctrl Pts',(21.2920815265358,20.1857233329509,36.6668586671162));
#49166=CARTESIAN_POINT('Ctrl Pts',(21.133459230111,20.1999916283318,36.5300942851992));
#49167=CARTESIAN_POINT('Ctrl Pts',(20.9936366308077,20.2120039634669,36.4380727606343));
#49168=CARTESIAN_POINT('Ctrl Pts',(20.7769844192553,20.2290775021017,36.3326989191347));
#49169=CARTESIAN_POINT('Ctrl Pts',(20.7083709819766,20.2342724132195,36.3040960237335));
#49170=CARTESIAN_POINT('Ctrl Pts',(20.6295203537795,20.2398875366485,36.2764505278996));
#49171=CARTESIAN_POINT('Ctrl Pts',(20.6207469974858,20.2405074612004,36.2734453945825));
#49172=CARTESIAN_POINT('Ctrl Pts',(20.6076589673942,20.2414247152248,36.2690675519348));
#49173=CARTESIAN_POINT('Ctrl Pts',(20.60336073944,20.2417247445791,36.2676466309217));
#49174=CARTESIAN_POINT('Ctrl Pts',(20.5956744667335,20.2422590697356,36.2651356581803));
#49175=CARTESIAN_POINT('Ctrl Pts',(20.5922883800514,20.242493696438,36.264039842817));
#49176=CARTESIAN_POINT('Ctrl Pts',(20.5849497045539,20.2430005455212,36.2616872949759));
#49177=CARTESIAN_POINT('Ctrl Pts',(20.5809960986943,20.2432725705557,36.2604339391005));
#49178=CARTESIAN_POINT('Ctrl Pts',(20.5699277126936,20.2440313183915,36.2569643275209));
#49179=CARTESIAN_POINT('Ctrl Pts',(20.5628039929789,20.2445164219025,36.2547765019864));
#49180=CARTESIAN_POINT('Ctrl Pts',(20.520821252716,20.2473573086006,36.2421485771388));
#49181=CARTESIAN_POINT('Ctrl Pts',(20.4856825200526,20.2496622418272,36.232654399755));
#49182=CARTESIAN_POINT('Ctrl Pts',(20.3682236419186,20.2571912186197,36.204458520344));
#49183=CARTESIAN_POINT('Ctrl Pts',(20.2849421147792,20.2622493213279,36.1901632192109));
#49184=CARTESIAN_POINT('Ctrl Pts',(20.0530552173636,20.2761827986977,36.165871940095));
#49185=CARTESIAN_POINT('Ctrl Pts',(19.9038480656321,20.2850209714909,36.1675366158263));
#49186=CARTESIAN_POINT('Ctrl Pts',(19.734535230508,20.2958340683796,36.1890962103837));
#49187=CARTESIAN_POINT('Ctrl Pts',(19.7127999590524,20.2972361284344,36.1922419149831));
#49188=CARTESIAN_POINT('Ctrl Pts',(19.6828156951633,20.2991915729042,36.1971054904579));
#49189=CARTESIAN_POINT('Ctrl Pts',(19.6745166013135,20.2997350659232,36.1985074411959));
#49190=CARTESIAN_POINT('Ctrl Pts',(19.6602611282363,20.3006726387018,36.2010116518228));
#49191=CARTESIAN_POINT('Ctrl Pts',(19.6543002290282,20.3010658911029,36.2020877484819));
#49192=CARTESIAN_POINT('Ctrl Pts',(19.642013522804,20.3018790097305,36.2043656210585));
#49193=CARTESIAN_POINT('Ctrl Pts',(19.6356884742876,20.302298986016,36.205571028771));
#49194=CARTESIAN_POINT('Ctrl Pts',(19.620964322683,20.303279957875,36.2084535772744));
#49195=CARTESIAN_POINT('Ctrl Pts',(19.612570171059,20.3038417160265,36.2101550228484));
#49196=CARTESIAN_POINT('Ctrl Pts',(19.585626616049,20.3056530926891,36.2158033776958));
#49197=CARTESIAN_POINT('Ctrl Pts',(19.567124463433,20.3069095730287,36.2199678355833));
#49198=CARTESIAN_POINT('Ctrl Pts',(19.4965550129601,20.3117518853395,36.2369485162783));
#49199=CARTESIAN_POINT('Ctrl Pts',(19.4449830273365,20.3153962277656,36.2516573096051));
#49200=CARTESIAN_POINT('Ctrl Pts',(19.3941039696621,20.3190989370965,36.2684889961235));
#49201=CARTESIAN_POINT('Origin',(20.,-1.3495818343519,38.1));
#49202=CARTESIAN_POINT('',(19.3941043260691,21.2861174117667,36.2684888782178));
#49203=CARTESIAN_POINT('',(19.3941040087494,21.1141809091495,36.2684889831927));
#49204=CARTESIAN_POINT('',(19.3941040087494,-1.3495818343519,36.2684889831927));
#49205=CARTESIAN_POINT('Ctrl Pts',(19.3941043260691,21.2861174117667,36.2684888782178));
#49206=CARTESIAN_POINT('Ctrl Pts',(19.4530786536075,21.2817380599914,36.2489791468798));
#49207=CARTESIAN_POINT('Ctrl Pts',(19.513005684334,21.2773036111486,36.2323143814167));
#49208=CARTESIAN_POINT('Ctrl Pts',(19.6542575541718,21.2669641769365,36.2003077326673));
#49209=CARTESIAN_POINT('Ctrl Pts',(19.7359292577877,21.2610689936283,36.1872436377992));
#49210=CARTESIAN_POINT('Ctrl Pts',(19.8540254899233,21.2528461851445,36.1760640370774));
#49211=CARTESIAN_POINT('Ctrl Pts',(19.8899504322543,21.2503850532323,36.1736750926777));
#49212=CARTESIAN_POINT('Ctrl Pts',(19.9333558357535,21.2474758123637,36.1720071504368));
#49213=CARTESIAN_POINT('Ctrl Pts',(19.9407895419167,21.2469798467427,36.1717645375422));
#49214=CARTESIAN_POINT('Ctrl Pts',(19.9523714299181,21.2462108574831,36.1714535824357));
#49215=CARTESIAN_POINT('Ctrl Pts',(19.9565186440202,21.2459362457946,36.171355621719));
#49216=CARTESIAN_POINT('Ctrl Pts',(19.9642163443898,21.2454279595525,36.1711986375657));
#49217=CARTESIAN_POINT('Ctrl Pts',(19.9677666707605,21.2451940943045,36.1711360393342));
#49218=CARTESIAN_POINT('Ctrl Pts',(19.9758248462538,21.2446645706607,36.171016215258));
#49219=CARTESIAN_POINT('Ctrl Pts',(19.9803327248656,21.2443692489433,36.1709649875726));
#49220=CARTESIAN_POINT('Ctrl Pts',(19.9940939636114,21.2434703599312,36.1708568477203));
#49221=CARTESIAN_POINT('Ctrl Pts',(20.0033477575419,21.2428695451387,36.1708507097407));
#49222=CARTESIAN_POINT('Ctrl Pts',(20.0885530179799,21.2373680965722,36.1714072993462));
#49223=CARTESIAN_POINT('Ctrl Pts',(20.1644192405313,21.2326925888865,36.1763886224085));
#49224=CARTESIAN_POINT('Ctrl Pts',(20.4053846792953,21.2180052321809,36.2065762507952));
#49225=CARTESIAN_POINT('Ctrl Pts',(20.5675666773086,21.2083026314686,36.248714299268));
#49226=CARTESIAN_POINT('Ctrl Pts',(20.7604899077144,21.1953394782839,36.3266152572359));
#49227=CARTESIAN_POINT('Ctrl Pts',(20.7981684855944,21.1927393247003,36.3432515763493));
#49228=CARTESIAN_POINT('Ctrl Pts',(20.8455913928736,21.1893644891853,36.366030994445));
#49229=CARTESIAN_POINT('Ctrl Pts',(20.85585449596,21.1886278783365,36.3710736312747));
#49230=CARTESIAN_POINT('Ctrl Pts',(20.8723214668155,21.1874356206372,36.379347004679));
#49231=CARTESIAN_POINT('Ctrl Pts',(20.8785537583876,21.1869819647847,36.3825208114063));
#49232=CARTESIAN_POINT('Ctrl Pts',(20.8904101581071,21.1861142288381,36.3886401276433));
#49233=CARTESIAN_POINT('Ctrl Pts',(20.8960372648553,21.1857003635763,36.3915796533806));
#49234=CARTESIAN_POINT('Ctrl Pts',(20.9088810185705,21.1847510057067,36.3983699700053));
#49235=CARTESIAN_POINT('Ctrl Pts',(20.9160878491944,21.1842148737211,36.4022389703014));
#49236=CARTESIAN_POINT('Ctrl Pts',(20.9348584711648,21.1828093685556,36.4124703278089));
#49237=CARTESIAN_POINT('Ctrl Pts',(20.9463817963244,21.181937409327,36.4189056431971));
#49238=CARTESIAN_POINT('Ctrl Pts',(21.0298614889384,21.1755526819184,36.4666560392451));
#49239=CARTESIAN_POINT('Ctrl Pts',(21.0991419192553,21.169877751565,36.5124513219875));
#49240=CARTESIAN_POINT('Ctrl Pts',(21.2943721212357,21.1527427812399,36.6604194150749));
#49241=CARTESIAN_POINT('Ctrl Pts',(21.4106373212665,21.1409379368308,36.7741462546931));
#49242=CARTESIAN_POINT('Ctrl Pts',(21.5345450015419,21.1270994775988,36.9303372496378));
#49243=CARTESIAN_POINT('Ctrl Pts',(21.5569184125529,21.1245415249144,36.9602873934727));
#49244=CARTESIAN_POINT('Ctrl Pts',(21.5827031305217,21.1215376499932,36.9969818056244));
#49245=CARTESIAN_POINT('Ctrl Pts',(21.5869616573707,21.1210396066896,37.003117581942));
#49246=CARTESIAN_POINT('Ctrl Pts',(21.5935202523732,21.1202697330977,37.0126854970061));
#49247=CARTESIAN_POINT('Ctrl Pts',(21.5958450526281,21.119996276264,37.0161004696246));
#49248=CARTESIAN_POINT('Ctrl Pts',(21.6001464149953,21.119489313078,37.0224627152164));
#49249=CARTESIAN_POINT('Ctrl Pts',(21.602125792458,21.1192556226636,37.0254079402611));
#49250=CARTESIAN_POINT('Ctrl Pts',(21.6065987840943,21.1187265911647,37.032103382718));
#49251=CARTESIAN_POINT('Ctrl Pts',(21.6090874019486,21.1184315850437,37.0358568836092));
#49252=CARTESIAN_POINT('Ctrl Pts',(21.6165931069662,21.1175396846526,37.0472640258523));
#49253=CARTESIAN_POINT('Ctrl Pts',(21.6215689879624,21.1169454480223,37.0549448196159));
#49254=CARTESIAN_POINT('Ctrl Pts',(21.6857361985965,21.1092394010588,37.1555554463062));
#49255=CARTESIAN_POINT('Ctrl Pts',(21.7369247673846,21.1026029143702,37.253370230959));
#49256=CARTESIAN_POINT('Ctrl Pts',(21.812183949424,21.0909436145242,37.4331404862799));
#49257=CARTESIAN_POINT('Ctrl Pts',(21.8397040202578,21.0859163435093,37.5133136160916));
#49258=CARTESIAN_POINT('Ctrl Pts',(21.8820351897066,21.0761070359057,37.6693931048017));
#49259=CARTESIAN_POINT('Ctrl Pts',(21.897727972401,21.0713530011949,37.7448869903914));
#49260=CARTESIAN_POINT('Ctrl Pts',(21.9116047707611,21.065249769927,37.8398672342602));
#49261=CARTESIAN_POINT('Ctrl Pts',(21.9140683977022,21.0640364059259,37.8586620963925));
#49262=CARTESIAN_POINT('Ctrl Pts',(21.9172437241738,21.062261568147,37.8860079486286));
#49263=CARTESIAN_POINT('Ctrl Pts',(21.918176017861,21.0617069651693,37.8945325900674));
#49264=CARTESIAN_POINT('Ctrl Pts',(21.9197101998067,21.0607319086572,37.9094824209609));
#49265=CARTESIAN_POINT('Ctrl Pts',(21.9203367476118,21.0603122293246,37.9159049885079));
#49266=CARTESIAN_POINT('Ctrl Pts',(21.921490574949,21.0594954809485,37.9283799656088));
#49267=CARTESIAN_POINT('Ctrl Pts',(21.9220215115702,21.0590985309182,37.9344319672444));
#49268=CARTESIAN_POINT('Ctrl Pts',(21.9232224994058,21.0581473643596,37.9489067617029));
#49269=CARTESIAN_POINT('Ctrl Pts',(21.9238658138255,21.0575923236917,37.9573315891652));
#49270=CARTESIAN_POINT('Ctrl Pts',(21.92599124032,21.0555795844935,37.9878015899245));
#49271=CARTESIAN_POINT('Ctrl Pts',(21.9271498894069,21.0541119290967,38.0098668963292));
#49272=CARTESIAN_POINT('Ctrl Pts',(21.9330165595865,21.0429770023299,38.1760673539951));
#49273=CARTESIAN_POINT('Ctrl Pts',(21.921926607354,21.0328099751706,38.3202776090934));
#49274=CARTESIAN_POINT('Ctrl Pts',(21.8785680200289,21.0163278764021,38.5473149834864));
#49275=CARTESIAN_POINT('Ctrl Pts',(21.856490665271,21.0101155227914,38.6315568006907));
#49276=CARTESIAN_POINT('Ctrl Pts',(21.817019995336,21.0015161281742,38.7491155977939));
#49277=CARTESIAN_POINT('Ctrl Pts',(21.8042297042457,20.9989842712054,38.7838628045715));
#49278=CARTESIAN_POINT('Ctrl Pts',(21.7876508626281,20.9960021214082,38.8251919269138));
#49279=CARTESIAN_POINT('Ctrl Pts',(21.7848146217099,20.9955014613372,38.8321445951326));
#49280=CARTESIAN_POINT('Ctrl Pts',(21.7803401539089,20.9947264001822,38.8429326236933));
#49281=CARTESIAN_POINT('Ctrl Pts',(21.7787300017751,20.9944503818302,38.8467794376971));
#49282=CARTESIAN_POINT('Ctrl Pts',(21.775719304002,20.9939396379641,38.8539073129886));
#49283=CARTESIAN_POINT('Ctrl Pts',(21.7743221400591,20.9937047214475,38.8571896901662));
#49284=CARTESIAN_POINT('Ctrl Pts',(21.7711313980161,20.9931729638317,38.8646284189198));
#49285=CARTESIAN_POINT('Ctrl Pts',(21.7693322946587,20.9928764594571,38.8687823360134));
#49286=CARTESIAN_POINT('Ctrl Pts',(21.7646305596737,20.9921100416799,38.8795341564602));
#49287=CARTESIAN_POINT('Ctrl Pts',(21.7617055088434,20.9916414441549,38.8861222661129));
#49288=CARTESIAN_POINT('Ctrl Pts',(21.7428801021627,20.9886761357281,38.9278900409968));
#49289=CARTESIAN_POINT('Ctrl Pts',(21.7259624042659,20.9862365757345,38.9626049113432));
#49290=CARTESIAN_POINT('Ctrl Pts',(21.7024018777434,20.9830862984951,39.0074778724268));
#49291=CARTESIAN_POINT('Ctrl Pts',(21.6966906319288,20.9823399963124,39.0181117321505));
#49292=CARTESIAN_POINT('Ctrl Pts',(21.6251243888338,20.9731897381084,39.1484132593932));
#49293=CARTESIAN_POINT('Ctrl Pts',(21.5468367123748,20.9652128951141,39.2608189840831));
#49294=CARTESIAN_POINT('Ctrl Pts',(21.4018331783591,20.9518403516606,39.4279982559164));
#49295=CARTESIAN_POINT('Ctrl Pts',(21.342192640408,20.9466366368227,39.4882478086865));
#49296=CARTESIAN_POINT('Ctrl Pts',(21.2638892331462,20.9399937019944,39.5575742638341));
#49297=CARTESIAN_POINT('Ctrl Pts',(21.24878380741,20.938720486148,39.5705365291897));
#49298=CARTESIAN_POINT('Ctrl Pts',(21.2267643605746,20.9368747640557,39.588847900649));
#49299=CARTESIAN_POINT('Ctrl Pts',(21.2200099939171,20.9363099568753,39.5943876599692));
#49300=CARTESIAN_POINT('Ctrl Pts',(21.2081887341865,20.9353236785883,39.6039495960522));
#49301=CARTESIAN_POINT('Ctrl Pts',(21.2031387634259,20.9349030447146,39.6079925461116));
#49302=CARTESIAN_POINT('Ctrl Pts',(21.1933540759508,20.9340893271147,39.6157456211735));
#49303=CARTESIAN_POINT('Ctrl Pts',(21.1886221472469,20.9336963850587,39.6194591565408));
#49304=CARTESIAN_POINT('Ctrl Pts',(21.177361187723,20.9327625844666,39.6282117689243));
#49305=CARTESIAN_POINT('Ctrl Pts',(21.1708170993336,20.9322209636444,39.6332311937149));
#49306=CARTESIAN_POINT('Ctrl Pts',(21.1475714980462,20.9303005457373,39.6508253532704));
#49307=CARTESIAN_POINT('Ctrl Pts',(21.1306984734675,20.9289129084639,39.6631700238439));
#49308=CARTESIAN_POINT('Ctrl Pts',(20.9797784232138,20.9165518939551,39.7698643380567));
#49309=CARTESIAN_POINT('Ctrl Pts',(20.8344380519894,20.9049100657465,39.8470271596253));
#49310=CARTESIAN_POINT('Ctrl Pts',(20.6118752125089,20.8879419200109,39.9310193124834));
#49311=CARTESIAN_POINT('Ctrl Pts',(20.5411611809335,20.8826798684249,39.9531511186928));
#49312=CARTESIAN_POINT('Ctrl Pts',(20.4366324219033,20.8752250306513,39.9793701553393));
#49313=CARTESIAN_POINT('Ctrl Pts',(20.4037069540682,20.8729227015064,39.9867170135623));
#49314=CARTESIAN_POINT('Ctrl Pts',(20.3634514272122,20.870176555391,39.9945972469143));
#49315=CARTESIAN_POINT('Ctrl Pts',(20.3562914207787,20.869690742674,39.9959567757769));
#49316=CARTESIAN_POINT('Ctrl Pts',(20.345080360158,20.8689343483586,39.9980197587123));
#49317=CARTESIAN_POINT('Ctrl Pts',(20.3410345626943,20.8686622552477,39.998750875513));
#49318=CARTESIAN_POINT('Ctrl Pts',(20.333479800961,20.8681558365528,40.0000911721797));
#49319=CARTESIAN_POINT('Ctrl Pts',(20.3299715217119,20.8679213391175,40.0007035632666));
#49320=CARTESIAN_POINT('Ctrl Pts',(20.3219533526429,20.8673869135395,40.0020803132277));
#49321=CARTESIAN_POINT('Ctrl Pts',(20.3174424333628,20.8670873437189,40.0028383488388));
#49322=CARTESIAN_POINT('Ctrl Pts',(20.3056453041331,20.8663066465731,40.0047776741459));
#49323=CARTESIAN_POINT('Ctrl Pts',(20.298354851389,20.865826924639,40.0059332167614));
#49324=CARTESIAN_POINT('Ctrl Pts',(20.2494790731442,20.8626280621921,40.0133927483809));
#49325=CARTESIAN_POINT('Ctrl Pts',(20.2077002527982,20.8599770802714,40.0183776573052));
#49326=CARTESIAN_POINT('Ctrl Pts',(20.1583209762786,20.8569066141167,40.0226370438984));
#49327=CARTESIAN_POINT('Ctrl Pts',(20.150849784348,20.8564437345537,40.0232376554204));
#49328=CARTESIAN_POINT('Ctrl Pts',(20.1298918897804,20.8551495544537,40.0247995904074));
#49329=CARTESIAN_POINT('Ctrl Pts',(20.1163981485239,20.8543212503624,40.02566270417));
#49330=CARTESIAN_POINT('Ctrl Pts',(19.9847847460247,20.8462812323355,40.032692726101));
#49331=CARTESIAN_POINT('Ctrl Pts',(19.8663397391472,20.8393363118176,40.0281260326375));
#49332=CARTESIAN_POINT('Ctrl Pts',(19.6835322088371,20.8282215762719,40.0041422777983));
#49333=CARTESIAN_POINT('Ctrl Pts',(19.6184994585567,20.8241906396675,39.9921854860312));
#49334=CARTESIAN_POINT('Ctrl Pts',(19.5166213884595,20.8176514627929,39.9679883405995));
#49335=CARTESIAN_POINT('Ctrl Pts',(19.4793097206715,20.8152080408505,39.9579334304749));
#49336=CARTESIAN_POINT('Ctrl Pts',(19.4315771843869,20.8120079228133,39.9435195022696));
#49337=CARTESIAN_POINT('Ctrl Pts',(19.4208561228392,20.8112842695956,39.9401796144482));
#49338=CARTESIAN_POINT('Ctrl Pts',(19.4035241307728,20.8101061885651,39.9346137859423));
#49339=CARTESIAN_POINT('Ctrl Pts',(19.396894937397,20.8096536355749,39.9324452208689));
#49340=CARTESIAN_POINT('Ctrl Pts',(19.3842030378788,20.8087833761557,39.9282170701286));
#49341=CARTESIAN_POINT('Ctrl Pts',(19.3781385294055,20.8083658604063,39.9261631536649));
#49342=CARTESIAN_POINT('Ctrl Pts',(19.3643186995108,20.8074105187375,39.9214058564097));
#49343=CARTESIAN_POINT('Ctrl Pts',(19.3565702337417,20.8068720606466,39.9186830790249));
#49344=CARTESIAN_POINT('Ctrl Pts',(19.3361085881551,20.8054425384426,39.9113458163529));
#49345=CARTESIAN_POINT('Ctrl Pts',(19.3234263284071,20.8045487069609,39.9066470392066));
#49346=CARTESIAN_POINT('Ctrl Pts',(19.2240385739183,20.7974810827014,39.8686306263865));
#49347=CARTESIAN_POINT('Ctrl Pts',(19.1398058304123,20.7911035751112,39.8292286529764));
#49348=CARTESIAN_POINT('Ctrl Pts',(18.9193057411064,20.7733565314104,39.7059769132127));
#49349=CARTESIAN_POINT('Ctrl Pts',(18.7900926816148,20.7617248975331,39.6110208129822));
#49350=CARTESIAN_POINT('Ctrl Pts',(18.6529510204969,20.7487191795197,39.4812481908839));
#49351=CARTESIAN_POINT('Ctrl Pts',(18.6322900881075,20.7467412802435,39.4607929087645));
#49352=CARTESIAN_POINT('Ctrl Pts',(18.6072660011793,20.74433095791,39.4348718915644));
#49353=CARTESIAN_POINT('Ctrl Pts',(18.6024609566081,20.7438674411294,39.4298404356177));
#49354=CARTESIAN_POINT('Ctrl Pts',(18.5949112795147,20.7431382195105,39.4218489083909));
#49355=CARTESIAN_POINT('Ctrl Pts',(18.592148595844,20.7428711701187,39.4189060897612));
#49356=CARTESIAN_POINT('Ctrl Pts',(18.5869563238376,20.7423689236967,39.4133403626425));
#49357=CARTESIAN_POINT('Ctrl Pts',(18.5845248198157,20.7421335856978,39.4107194029951));
#49358=CARTESIAN_POINT('Ctrl Pts',(18.5789708506079,20.7415956851671,39.4046992056137));
#49359=CARTESIAN_POINT('Ctrl Pts',(18.5758532885409,20.741293492685,39.4012955105899));
#49360=CARTESIAN_POINT('Ctrl Pts',(18.5675814949199,20.7404908946309,39.3921991927915));
#49361=CARTESIAN_POINT('Ctrl Pts',(18.562448923044,20.7399920615767,39.3864868570794));
#49362=CARTESIAN_POINT('Ctrl Pts',(18.5252953457473,20.7363737080218,39.344636500091));
#49363=CARTESIAN_POINT('Ctrl Pts',(18.4946039320468,20.7333441227353,39.3073348356099));
#49364=CARTESIAN_POINT('Ctrl Pts',(18.4569991913185,20.7295200251917,39.257964005415));
#49365=CARTESIAN_POINT('Ctrl Pts',(18.4487736885712,20.7286761324003,39.2469215657361));
#49366=CARTESIAN_POINT('Ctrl Pts',(18.3686241837584,20.7203688115048,39.1368839964109));
#49367=CARTESIAN_POINT('Ctrl Pts',(18.306153006079,20.7131922398046,39.031343336422));
#49368=CARTESIAN_POINT('Ctrl Pts',(18.2270148952385,20.7019606705466,38.8629681662927));
#49369=CARTESIAN_POINT('Ctrl Pts',(18.2028024607114,20.6980703894045,38.8040430365984));
#49370=CARTESIAN_POINT('Ctrl Pts',(18.1689728312178,20.6917369514213,38.708523675981));
#49371=CARTESIAN_POINT('Ctrl Pts',(18.1574404500939,20.6893533089713,38.6726565824612));
#49372=CARTESIAN_POINT('Ctrl Pts',(18.1438681532177,20.686220444831,38.6257767673026));
#49373=CARTESIAN_POINT('Ctrl Pts',(18.140863176003,20.6855024856943,38.6150503886727));
#49374=CARTESIAN_POINT('Ctrl Pts',(18.1361316589063,20.6843310145616,38.5975799608769));
#49375=CARTESIAN_POINT('Ctrl Pts',(18.1343484026852,20.6838793316209,38.5908514293874));
#49376=CARTESIAN_POINT('Ctrl Pts',(18.1309909504513,20.6830089112049,38.5779005381241));
#49377=CARTESIAN_POINT('Ctrl Pts',(18.1294113132571,20.6825903547232,38.5716796741426));
#49378=CARTESIAN_POINT('Ctrl Pts',(18.1258668752172,20.6816300446292,38.5574232369915));
#49379=CARTESIAN_POINT('Ctrl Pts',(18.1239226685804,20.6810876408784,38.5493827211766));
#49380=CARTESIAN_POINT('Ctrl Pts',(18.1188942129158,20.6796419680049,38.5279853848949));
#49381=CARTESIAN_POINT('Ctrl Pts',(18.1159005632451,20.6787358388782,38.5146079689316));
#49382=CARTESIAN_POINT('Ctrl Pts',(18.0848801270923,20.668826538751,38.3687106412563));
#49383=CARTESIAN_POINT('Ctrl Pts',(18.0707478826055,20.659371969667,38.2336496127508));
#49384=CARTESIAN_POINT('Ctrl Pts',(18.0709928462404,20.6401631583163,37.9637962455339));
#49385=CARTESIAN_POINT('Ctrl Pts',(18.0851705182672,20.6304706736182,37.8297155384801));
#49386=CARTESIAN_POINT('Ctrl Pts',(18.1161120013264,20.620408379265,37.6844198972611));
#49387=CARTESIAN_POINT('Ctrl Pts',(18.11919551829,20.6194616306672,37.6706803717333));
#49388=CARTESIAN_POINT('Ctrl Pts',(18.1236983313918,20.6181544599231,37.6515971218349));
#49389=CARTESIAN_POINT('Ctrl Pts',(18.1249904825226,20.61778729405,37.646224280073));
#49390=CARTESIAN_POINT('Ctrl Pts',(18.1271039921872,20.6171993621344,37.6375993618584));
#49391=CARTESIAN_POINT('Ctrl Pts',(18.127910764255,20.6169777789537,37.6343437962699));
#49392=CARTESIAN_POINT('Ctrl Pts',(18.1296179757692,20.6165148013958,37.6275308414398));
#49393=CARTESIAN_POINT('Ctrl Pts',(18.1305200792661,20.6162735090259,37.6239738992171));
#49394=CARTESIAN_POINT('Ctrl Pts',(18.1327397539886,20.6156878057185,37.6153254811324));
#49395=CARTESIAN_POINT('Ctrl Pts',(18.1340680199539,20.6153440032017,37.6102367275803));
#49396=CARTESIAN_POINT('Ctrl Pts',(18.1388622324917,20.6141262696561,37.5921721260313));
#49397=CARTESIAN_POINT('Ctrl Pts',(18.1424429528276,20.6132586438342,37.579226747897));
#49398=CARTESIAN_POINT('Ctrl Pts',(18.1653294684156,20.6079553450875,37.4997260748553));
#49399=CARTESIAN_POINT('Ctrl Pts',(18.1880768118965,20.6036922667605,37.434206287396));
#49400=CARTESIAN_POINT('Ctrl Pts',(18.2668309394992,20.5910952720247,37.2415489187266));
#49401=CARTESIAN_POINT('Ctrl Pts',(18.3330727075436,20.5829761589737,37.1190985668106));
#49402=CARTESIAN_POINT('Ctrl Pts',(18.4489458117829,20.5704728911086,36.951072028565));
#49403=CARTESIAN_POINT('Ctrl Pts',(18.4887088310256,20.5664027502613,36.8992493226898));
#49404=CARTESIAN_POINT('Ctrl Pts',(18.5391303563616,20.5614281283557,36.8400162540496));
#49405=CARTESIAN_POINT('Ctrl Pts',(18.5473342185821,20.5606242115891,36.8305665549551));
#49406=CARTESIAN_POINT('Ctrl Pts',(18.560932907847,20.5593001394236,36.8152072255856));
#49407=CARTESIAN_POINT('Ctrl Pts',(18.5662736787097,20.5587822174707,36.8092500624174));
#49408=CARTESIAN_POINT('Ctrl Pts',(18.57593029567,20.557849406416,36.7986128318426));
#49409=CARTESIAN_POINT('Ctrl Pts',(18.5802325671074,20.5574350900605,36.7939205540572));
#49410=CARTESIAN_POINT('Ctrl Pts',(18.5894346797119,20.5565515557838,36.783983453731));
#49411=CARTESIAN_POINT('Ctrl Pts',(18.5943407126723,20.5560820787099,36.7787445218794));
#49412=CARTESIAN_POINT('Ctrl Pts',(18.6076141547584,20.5548160105801,36.7647280152689));
#49413=CARTESIAN_POINT('Ctrl Pts',(18.6160351717435,20.5540171277593,36.7560018757322));
#49414=CARTESIAN_POINT('Ctrl Pts',(18.6586246307406,20.5499976713498,36.71269396313));
#49415=CARTESIAN_POINT('Ctrl Pts',(18.6940067056829,20.5467242182585,36.6793358170251));
#49416=CARTESIAN_POINT('Ctrl Pts',(18.8552168211107,20.5320756402526,36.5384628965962));
#49417=CARTESIAN_POINT('Ctrl Pts',(18.9933083352661,20.5201252832972,36.4460705891164));
#49418=CARTESIAN_POINT('Ctrl Pts',(19.2030934478916,20.5035569674476,36.341813392907));
#49419=CARTESIAN_POINT('Ctrl Pts',(19.2663346837732,20.4987558837779,36.3144979396941));
#49420=CARTESIAN_POINT('Ctrl Pts',(19.3395314034464,20.4935121198439,36.2874304622701));
#49421=CARTESIAN_POINT('Ctrl Pts',(19.3481780820398,20.4928975294562,36.2843030837612));
#49422=CARTESIAN_POINT('Ctrl Pts',(19.3610999829948,20.4919866217655,36.2797336252887));
#49423=CARTESIAN_POINT('Ctrl Pts',(19.3653582839632,20.4916876572992,36.2782445828467));
#49424=CARTESIAN_POINT('Ctrl Pts',(19.3729840108008,20.4911544984062,36.2756080021452));
#49425=CARTESIAN_POINT('Ctrl Pts',(19.3763494125397,20.4909199788694,36.2744548326584));
#49426=CARTESIAN_POINT('Ctrl Pts',(19.3836555889905,20.4904125306446,36.2719739018155));
#49427=CARTESIAN_POINT('Ctrl Pts',(19.3875974635277,20.4901398037333,36.2706495735492));
#49428=CARTESIAN_POINT('Ctrl Pts',(19.3923968938888,20.4898089912107,36.2690543888959));
#49429=CARTESIAN_POINT('Ctrl Pts',(19.3932503519079,20.489750212374,36.2687713878594));
#49430=CARTESIAN_POINT('Ctrl Pts',(19.3941040087494,20.489691467393,36.2684889831927));
#49431=CARTESIAN_POINT('',(18.0708703408215,20.4785431656481,38.1011467247646));
#49432=CARTESIAN_POINT('Ctrl Pts',(19.3941039696621,20.3190989370965,36.2684889961235));
#49433=CARTESIAN_POINT('Ctrl Pts',(19.3716471618326,20.3207332250667,36.2759181028497));
#49434=CARTESIAN_POINT('Ctrl Pts',(19.3493253354268,20.3223787230364,36.2837607820347));
#49435=CARTESIAN_POINT('Ctrl Pts',(19.2482078801407,20.3299262073019,36.3213920884692));
#49436=CARTESIAN_POINT('Ctrl Pts',(19.1712792221264,20.3359349437724,36.3559077664399));
#49437=CARTESIAN_POINT('Ctrl Pts',(18.9996103855285,20.3497960266246,36.44685915099));
#49438=CARTESIAN_POINT('Ctrl Pts',(18.906938389977,20.3576277663694,36.5066148479924));
#49439=CARTESIAN_POINT('Ctrl Pts',(18.8126148015479,20.3656391045745,36.579558341963));
#49440=CARTESIAN_POINT('Ctrl Pts',(18.8054093265105,20.3662512927585,36.5852130262149));
#49441=CARTESIAN_POINT('Ctrl Pts',(18.7947208197537,20.3671593554595,36.5937248120561));
#49442=CARTESIAN_POINT('Ctrl Pts',(18.7912072068778,20.3674578531395,36.5965430406995));
#49443=CARTESIAN_POINT('Ctrl Pts',(18.7849363823635,20.3679905251424,36.6016089910456));
#49444=CARTESIAN_POINT('Ctrl Pts',(18.7821754976225,20.3682250218602,36.6038520485203));
#49445=CARTESIAN_POINT('Ctrl Pts',(18.7794083306838,20.3684600241805,36.6061129447132));
#49446=CARTESIAN_POINT('Ctrl Pts',(18.7793959008334,20.3684610797881,36.6061231007023));
#49447=CARTESIAN_POINT('Ctrl Pts',(18.7793712052984,20.3684631770605,36.6061432790605));
#49448=CARTESIAN_POINT('Ctrl Pts',(18.7793589399764,20.3684642186945,36.6061533011265));
#49449=CARTESIAN_POINT('Ctrl Pts',(18.7793345722372,20.368466288127,36.6061732126485));
#49450=CARTESIAN_POINT('Ctrl Pts',(18.7793224691425,20.3684673159829,36.6061831026515));
#49451=CARTESIAN_POINT('Ctrl Pts',(18.7792984214893,20.3684693582303,36.6062027535976));
#49452=CARTESIAN_POINT('Ctrl Pts',(18.7792864772904,20.3684703725911,36.6062125142405));
#49453=CARTESIAN_POINT('Ctrl Pts',(18.7760953336031,20.3687413802891,36.6088203388873));
#49454=CARTESIAN_POINT('Ctrl Pts',(18.7729243998563,20.3690106410012,36.6114285752936));
#49455=CARTESIAN_POINT('Ctrl Pts',(18.7642122353526,20.3697504291266,36.6186414799745));
#49456=CARTESIAN_POINT('Ctrl Pts',(18.7586883654837,20.3702194765097,36.6232671554728));
#49457=CARTESIAN_POINT('Ctrl Pts',(18.7462596930017,20.3712751518598,36.6337939116918));
#49458=CARTESIAN_POINT('Ctrl Pts',(18.7393703388348,20.3718605519273,36.6397130708068));
#49459=CARTESIAN_POINT('Ctrl Pts',(18.7179033888305,20.3736862990958,36.6584220775019));
#49460=CARTESIAN_POINT('Ctrl Pts',(18.7034762268257,20.3749157545948,36.6713836081802));
#49461=CARTESIAN_POINT('Ctrl Pts',(18.6463164774943,20.3798084642916,36.7243158425823));
#49462=CARTESIAN_POINT('Ctrl Pts',(18.6052139254752,20.3833769835044,36.7660064240685));
#49463=CARTESIAN_POINT('Ctrl Pts',(18.5004791923888,20.3928162290999,36.8823822660866));
#49464=CARTESIAN_POINT('Ctrl Pts',(18.4405422746111,20.3986055688392,36.9601545623183));
#49465=CARTESIAN_POINT('Ctrl Pts',(18.3343681786917,20.4102884422177,37.1220697728059));
#49466=CARTESIAN_POINT('Ctrl Pts',(18.28797799341,20.4161601134303,37.2057663187303));
#49467=CARTESIAN_POINT('Ctrl Pts',(18.2422929310617,20.4231300315013,37.3048942077643));
#49468=CARTESIAN_POINT('Ctrl Pts',(18.2367337285371,20.4240023854527,37.3172999285764));
#49469=CARTESIAN_POINT('Ctrl Pts',(18.2280173795923,20.4254104578191,37.3373152674415));
#49470=CARTESIAN_POINT('Ctrl Pts',(18.2247769903029,20.4259433586893,37.3448883058201));
#49471=CARTESIAN_POINT('Ctrl Pts',(18.2191009991907,20.4268939445154,37.3583920117446));
#49472=CARTESIAN_POINT('Ctrl Pts',(18.216646259645,20.4273109780362,37.3643145410993));
#49473=CARTESIAN_POINT('Ctrl Pts',(18.2115833163227,20.4281836901362,37.3767041082259));
#49474=CARTESIAN_POINT('Ctrl Pts',(18.2089805679969,20.428639544319,37.3831732611315));
#49475=CARTESIAN_POINT('Ctrl Pts',(18.2022878343676,20.4298308594311,37.4000721234502));
#49476=CARTESIAN_POINT('Ctrl Pts',(18.1982535743931,20.4305681641121,37.4105234799487));
#49477=CARTESIAN_POINT('Ctrl Pts',(18.180824924404,20.4338406673716,37.4568727496232));
#49478=CARTESIAN_POINT('Ctrl Pts',(18.1684115238389,20.4364079173706,37.4931277598327));
#49479=CARTESIAN_POINT('Ctrl Pts',(18.1377917785253,20.4434401539474,37.5920794319352));
#49480=CARTESIAN_POINT('Ctrl Pts',(18.121675866749,20.447966194841,37.6553656297573));
#49481=CARTESIAN_POINT('Ctrl Pts',(18.0835039116005,20.4615782357669,37.8450128468811));
#49482=CARTESIAN_POINT('Ctrl Pts',(18.0708001340919,20.4708402101582,37.9728809532063));
#49483=CARTESIAN_POINT('Ctrl Pts',(18.0708702889621,20.4798373080997,38.1010558838905));
#49484=CARTESIAN_POINT('Ctrl Pts',(18.0708703408215,20.4785431656481,38.1011467247647));
#49485=CARTESIAN_POINT('Ctrl Pts',(18.0709111555238,20.483059702729,38.1698091058912));
#49486=CARTESIAN_POINT('Ctrl Pts',(18.0746175415454,20.4875762398099,38.2383609278836));
#49487=CARTESIAN_POINT('Ctrl Pts',(18.0819556351502,20.4920927768908,38.3065148211825));
#49488=CARTESIAN_POINT('Ctrl Pts',(18.0891992046318,20.4965511351406,38.37379080431));
#49489=CARTESIAN_POINT('Ctrl Pts',(18.100000955713,20.5010094933905,38.4408181004181));
#49490=CARTESIAN_POINT('Ctrl Pts',(18.1143335343437,20.5054678516404,38.507191032808));
#49491=CARTESIAN_POINT('Ctrl Pts',(18.12938235242,20.5101490066474,38.5768808081418));
#49492=CARTESIAN_POINT('Ctrl Pts',(18.1483241750998,20.5148301616545,38.6458485571126));
#49493=CARTESIAN_POINT('Ctrl Pts',(18.1710655625826,20.5195113166616,38.7136296770274));
#49494=CARTESIAN_POINT('Ctrl Pts',(18.1926658517794,20.5239575845951,38.7780097327012));
#49495=CARTESIAN_POINT('Ctrl Pts',(18.2176934096763,20.5284038525285,38.8413188378757));
#49496=CARTESIAN_POINT('Ctrl Pts',(18.2460161837978,20.532850120462,38.903170797154));
#49497=CARTESIAN_POINT('Ctrl Pts',(18.2743218618263,20.5372937045549,38.9649854215706));
#49498=CARTESIAN_POINT('Ctrl Pts',(18.3059186054943,20.5417372886478,39.0253441974552));
#49499=CARTESIAN_POINT('Ctrl Pts',(18.3406260642371,20.5461808727408,39.0838804288178));
#49500=CARTESIAN_POINT('Ctrl Pts',(18.3753245338612,20.5506233059599,39.1424014994872));
#49501=CARTESIAN_POINT('Ctrl Pts',(18.4131318675803,20.555065739179,39.1991005388149));
#49502=CARTESIAN_POINT('Ctrl Pts',(18.4538224294339,20.5595081723981,39.2536366313438));
#49503=CARTESIAN_POINT('Ctrl Pts',(18.4945164748564,20.5639509859394,39.3081773927745));
#49504=CARTESIAN_POINT('Ctrl Pts',(18.5380939413293,20.5683937994806,39.3605544462424));
#49505=CARTESIAN_POINT('Ctrl Pts',(18.5842877530733,20.5728366130219,39.410458465882));
#49506=CARTESIAN_POINT('Ctrl Pts',(18.6305313534035,20.5772842151138,39.4604162730418));
#49507=CARTESIAN_POINT('Ctrl Pts',(18.6793965899742,20.5817318172057,39.5078953655218));
#49508=CARTESIAN_POINT('Ctrl Pts',(18.7305789504475,20.5861794192976,39.5526227162801));
#49509=CARTESIAN_POINT('Ctrl Pts',(18.781793310398,20.5906298020533,39.5973780308101));
#49510=CARTESIAN_POINT('Ctrl Pts',(18.8353272890455,20.5950801848091,39.6393778759309));
#49511=CARTESIAN_POINT('Ctrl Pts',(18.8908448890875,20.5995305675649,39.6783907934465));
#49512=CARTESIAN_POINT('Ctrl Pts',(18.9464563730737,20.6039884762131,39.7174696843934));
#49513=CARTESIAN_POINT('Ctrl Pts',(19.004057754121,20.6084463848613,39.7535513079927));
#49514=CARTESIAN_POINT('Ctrl Pts',(19.063286648776,20.6129042935095,39.7864491259859));
#49515=CARTESIAN_POINT('Ctrl Pts',(19.0850374747073,20.6145413862763,39.7985303021899));
#49516=CARTESIAN_POINT('Ctrl Pts',(19.1070075813411,20.6161784790431,39.8101825734671));
#49517=CARTESIAN_POINT('Ctrl Pts',(19.129178373231,20.6178155718099,39.821398341829));
#49518=CARTESIAN_POINT('Ctrl Pts',(19.1895549429292,20.622273781784,39.851941663131));
#49519=CARTESIAN_POINT('Ctrl Pts',(19.25165968076,20.626731991758,39.8793650048683));
#49520=CARTESIAN_POINT('Ctrl Pts',(19.3151374153393,20.6311902017321,39.9034704868758));
#49521=CARTESIAN_POINT('Ctrl Pts',(19.3817897922614,20.6358713752737,39.9287815299257));
#49522=CARTESIAN_POINT('Ctrl Pts',(19.4499556611319,20.6405525488152,39.9504338143543));
#49523=CARTESIAN_POINT('Ctrl Pts',(19.5191943989729,20.6452337223567,39.9682528016628));
#49524=CARTESIAN_POINT('Ctrl Pts',(19.5849564745287,20.6496798416496,39.9851770499413));
#49525=CARTESIAN_POINT('Ctrl Pts',(19.6516857260476,20.6541259609425,39.998643539088));
#49526=CARTESIAN_POINT('Ctrl Pts',(19.7189863291311,20.6585720802353,40.008552821822));
#49527=CARTESIAN_POINT('Ctrl Pts',(19.7862463109997,20.663015515945,40.0184561235234));
#49528=CARTESIAN_POINT('Ctrl Pts',(19.8540764734469,20.6674589516547,40.024806406256));
#49529=CARTESIAN_POINT('Ctrl Pts',(19.9220710582345,20.6719023873644,40.0275553524958));
#49530=CARTESIAN_POINT('Ctrl Pts',(19.9900480394356,20.6763446726824,40.030303587042));
#49531=CARTESIAN_POINT('Ctrl Pts',(20.0581888658978,20.6807869580004,40.0294523163286));
#49532=CARTESIAN_POINT('Ctrl Pts',(20.1260847549693,20.6852292433183,40.0250052445291));
#49533=CARTESIAN_POINT('Ctrl Pts',(20.193986467695,20.6896719096658,40.0205577912895));
#49534=CARTESIAN_POINT('Ctrl Pts',(20.2616427094173,20.6941145760132,40.0125139596816));
#49535=CARTESIAN_POINT('Ctrl Pts',(20.3286486398796,20.6985572423607,40.0009294117366));
#49536=CARTESIAN_POINT('Ctrl Pts',(20.3957268230535,20.7030046992496,39.9893323721361));
#49537=CARTESIAN_POINT('Ctrl Pts',(20.4621528090275,20.7074521561386,39.9741870825268));
#49538=CARTESIAN_POINT('Ctrl Pts',(20.5275318296978,20.7118996130275,39.9556003679553));
#49539=CARTESIAN_POINT('Ctrl Pts',(20.5929517413555,20.7163498515565,39.9370020284144));
#49540=CARTESIAN_POINT('Ctrl Pts',(20.6573229182579,20.7208000900855,39.9149581406292));
#49541=CARTESIAN_POINT('Ctrl Pts',(20.7202683257296,20.7252503286145,39.8896245684083));
#49542=CARTESIAN_POINT('Ctrl Pts',(20.7833202210014,20.7297080958279,39.8642481381541));
#49543=CARTESIAN_POINT('Ctrl Pts',(20.8449410876416,20.7341658630414,39.8355711269434));
#49544=CARTESIAN_POINT('Ctrl Pts',(20.9047772110109,20.7386236302549,39.8037959840707));
#49545=CARTESIAN_POINT('Ctrl Pts',(20.9267672016582,20.7402618757462,39.792118504728));
#49546=CARTESIAN_POINT('Ctrl Pts',(20.9485164242748,20.7419001212376,39.7800230214307));
#49547=CARTESIAN_POINT('Ctrl Pts',(20.9700083480463,20.743538366729,39.7675210228421));
#49548=CARTESIAN_POINT('Ctrl Pts',(21.0284978130772,20.7479967904327,39.733497302256));
#49549=CARTESIAN_POINT('Ctrl Pts',(21.0853105251314,20.7524552141363,39.6963253160254));
#49550=CARTESIAN_POINT('Ctrl Pts',(21.1400871365967,20.75691363784,39.6561953212456));
#49551=CARTESIAN_POINT('Ctrl Pts',(21.1976001452084,20.7615947846653,39.6140606094842));
#49552=CARTESIAN_POINT('Ctrl Pts',(21.2528677787936,20.7662759314907,39.5686647970493));
#49553=CARTESIAN_POINT('Ctrl Pts',(21.3055038160382,20.770957078316,39.5202824871164));
#49554=CARTESIAN_POINT('Ctrl Pts',(21.3554995186628,20.7754034089456,39.4743271358719));
#49555=CARTESIAN_POINT('Ctrl Pts',(21.4031208630278,20.7798497395752,39.4256780713646));
#49556=CARTESIAN_POINT('Ctrl Pts',(21.4480689460585,20.7842960702048,39.3746132293213));
#49557=CARTESIAN_POINT('Ctrl Pts',(21.4929898863324,20.7887397158329,39.3235792237564));
#49558=CARTESIAN_POINT('Ctrl Pts',(21.5352404424524,20.793183361461,39.2701327039082));
#49559=CARTESIAN_POINT('Ctrl Pts',(21.574559195328,20.7976270070891,39.2145877701231));
#49560=CARTESIAN_POINT('Ctrl Pts',(21.6138677539025,20.8020695005987,39.159057237654));
#49561=CARTESIAN_POINT('Ctrl Pts',(21.6502457336331,20.8065119941083,39.1014297737565));
#49562=CARTESIAN_POINT('Ctrl Pts',(21.683473708243,20.8109544876179,39.0420503333446));
#49563=CARTESIAN_POINT('Ctrl Pts',(21.7167045175562,20.8153973601199,38.9826658272283));
#49564=CARTESIAN_POINT('Ctrl Pts',(21.7467845498965,20.8198402326219,38.9215294795391));
#49565=CARTESIAN_POINT('Ctrl Pts',(21.773540110251,20.824283105124,38.859011221413));
#49566=CARTESIAN_POINT('Ctrl Pts',(21.8003244937898,20.8287307638361,38.7964256137247));
#49567=CARTESIAN_POINT('Ctrl Pts',(21.8237770651948,20.8331784225482,38.7324555793768));
#49568=CARTESIAN_POINT('Ctrl Pts',(21.8437725306241,20.8376260812604,38.6674904512114));
#49569=CARTESIAN_POINT('Ctrl Pts',(21.8637804913952,20.8420765193535,38.6024847257673));
#49570=CARTESIAN_POINT('Ctrl Pts',(21.8803269274325,20.8465269574466,38.5364831473164));
#49571=CARTESIAN_POINT('Ctrl Pts',(21.8933373342609,20.8509773955397,38.4698868686421));
#49572=CARTESIAN_POINT('Ctrl Pts',(21.9063697352151,20.8554353571097,38.403178008789));
#49573=CARTESIAN_POINT('Ctrl Pts',(21.9158541111529,20.8598933186797,38.3358729304174));
#49574=CARTESIAN_POINT('Ctrl Pts',(21.9217677302915,20.8643512802497,38.2683785844767));
#49575=CARTESIAN_POINT('Ctrl Pts',(21.9239387650532,20.8659879073825,38.2435997531337));
#49576=CARTESIAN_POINT('Ctrl Pts',(21.9256290393793,20.8676245345153,38.2187954115716));
#49577=CARTESIAN_POINT('Ctrl Pts',(21.926839188957,20.8692611616481,38.1939856201742));
#49578=CARTESIAN_POINT('Ctrl Pts',(21.9301359006187,20.8737196912827,38.1263983316863));
#49579=CARTESIAN_POINT('Ctrl Pts',(21.9298786981062,20.8781782209172,38.0585039674556));
#49580=CARTESIAN_POINT('Ctrl Pts',(21.9260315986928,20.8826367505517,37.990707558648));
#49581=CARTESIAN_POINT('Ctrl Pts',(21.9219924226099,20.8873178841357,37.9195262338265));
#49582=CARTESIAN_POINT('Ctrl Pts',(21.9139953705416,20.8919990177197,37.8484534371793));
#49583=CARTESIAN_POINT('Ctrl Pts',(21.902060588042,20.8966801513037,37.777962616584));
#49584=CARTESIAN_POINT('Ctrl Pts',(21.8907241608886,20.9011265942843,37.711005882962));
#49585=CARTESIAN_POINT('Ctrl Pts',(21.8758354328192,20.9055730372648,37.6445747319696));
#49586=CARTESIAN_POINT('Ctrl Pts',(21.8574648725121,20.9100194802454,37.5790712099684));
#49587=CARTESIAN_POINT('Ctrl Pts',(21.8391053969685,20.9144632402502,37.5136072126764));
#49588=CARTESIAN_POINT('Ctrl Pts',(21.8172683897229,20.9189070002549,37.4490702078103));
#49589=CARTESIAN_POINT('Ctrl Pts',(21.792075060108,20.9233507602597,37.3858504807543));
#49590=CARTESIAN_POINT('Ctrl Pts',(21.7668882518946,20.9277933699781,37.322647118396));
#49591=CARTESIAN_POINT('Ctrl Pts',(21.7383470287057,20.9322359796965,37.2607608147207));
#49592=CARTESIAN_POINT('Ctrl Pts',(21.7066213401951,20.9366785894149,37.2005634218631));
#49593=CARTESIAN_POINT('Ctrl Pts',(21.6748929334973,20.9411215797663,37.1403608714253));
#49594=CARTESIAN_POINT('Ctrl Pts',(21.6399797521761,20.9455645701177,37.0818479539657));
#49595=CARTESIAN_POINT('Ctrl Pts',(21.6020975899296,20.9500075604692,37.0253717530039));
#49596=CARTESIAN_POINT('Ctrl Pts',(21.5641746049835,20.9544553386904,36.9688346919739));
#49597=CARTESIAN_POINT('Ctrl Pts',(21.5232765305345,20.9589031169116,36.914339136874));
#49598=CARTESIAN_POINT('Ctrl Pts',(21.4796617814511,20.9633508951328,36.8622021290158));
#49599=CARTESIAN_POINT('Ctrl Pts',(21.4360197670868,20.9678014538337,36.8100325282804));
#49600=CARTESIAN_POINT('Ctrl Pts',(21.3896580345579,20.9722520125346,36.7602247695383));
#49601=CARTESIAN_POINT('Ctrl Pts',(21.3408725598251,20.9767025712355,36.7130597218308));
#49602=CARTESIAN_POINT('Ctrl Pts',(21.2920046098859,20.9811606539125,36.6658149383605));
#49603=CARTESIAN_POINT('Ctrl Pts',(21.2407051137358,20.9856187365895,36.6212221032468));
#49604=CARTESIAN_POINT('Ctrl Pts',(21.1873030923581,20.9900768192665,36.5795218108185));
#49605=CARTESIAN_POINT('Ctrl Pts',(21.167709388815,20.9917125317001,36.5642215816057));
#49606=CARTESIAN_POINT('Ctrl Pts',(21.147832913589,20.9933482441336,36.5493103278902));
#49607=CARTESIAN_POINT('Ctrl Pts',(21.1276908112208,20.9949839565672,36.5347984183536));
#49608=CARTESIAN_POINT('Ctrl Pts',(21.0727993548713,20.9994416162496,36.4952504191275));
#49609=CARTESIAN_POINT('Ctrl Pts',(21.0157162941417,21.003899275932,36.4585151822182));
#49610=CARTESIAN_POINT('Ctrl Pts',(20.9567616502993,21.0083569356144,36.4248433800338));
#49611=CARTESIAN_POINT('Ctrl Pts',(20.8979095980615,21.0128068381733,36.3912301727961));
#49612=CARTESIAN_POINT('Ctrl Pts',(20.8371928576362,21.0172567407321,36.3606700527017));
#49613=CARTESIAN_POINT('Ctrl Pts',(20.7749613541135,21.0217066432909,36.3333711605064));
#49614=CARTESIAN_POINT('Ctrl Pts',(20.7127908879904,21.0261521813323,36.3060990433896));
#49615=CARTESIAN_POINT('Ctrl Pts',(20.6491090545898,21.0305977193737,36.2820820077792));
#49616=CARTESIAN_POINT('Ctrl Pts',(20.5842901976383,21.0350432574151,36.2614822487004));
#49617=CARTESIAN_POINT('Ctrl Pts',(20.519512553486,21.0394859689169,36.2408955872566));
#49618=CARTESIAN_POINT('Ctrl Pts',(20.4535997892027,21.0439286804187,36.2237220405848));
#49619=CARTESIAN_POINT('Ctrl Pts',(20.3869443306759,21.0483713919205,36.2100749639582));
#49620=CARTESIAN_POINT('Ctrl Pts',(20.3203082581246,21.0528128113106,36.1964318564272));
#49621=CARTESIAN_POINT('Ctrl Pts',(20.2529304033284,21.0572542307007,36.1863132808701));
#49622=CARTESIAN_POINT('Ctrl Pts',(20.1852145989036,21.0616956500908,36.1797817547859));
#49623=CARTESIAN_POINT('Ctrl Pts',(20.1174534960788,21.0661400405627,36.1732458594458));
#49624=CARTESIAN_POINT('Ctrl Pts',(20.0493544834623,21.0705844310346,36.1703018605945));
#49625=CARTESIAN_POINT('Ctrl Pts',(19.9813266676957,21.0750288215065,36.1709603779184));
#49626=CARTESIAN_POINT('Ctrl Pts',(19.9132787554393,21.0794745249214,36.1716190897788));
#49627=CARTESIAN_POINT('Ctrl Pts',(19.845302575557,21.0839202283363,36.1758824135838));
#49628=CARTESIAN_POINT('Ctrl Pts',(19.7778046531292,21.0883659317512,36.1837088465661));
#49629=CARTESIAN_POINT('Ctrl Pts',(19.7101977872644,21.0928188106494,36.1915479116188));
#49630=CARTESIAN_POINT('Ctrl Pts',(19.6430712100821,21.0972716895475,36.2029614995978));
#49631=CARTESIAN_POINT('Ctrl Pts',(19.5768230943422,21.1017245684457,36.2178565773518));
#49632=CARTESIAN_POINT('Ctrl Pts',(19.5150496424909,21.1058766820136,36.2317455817134));
#49633=CARTESIAN_POINT('Ctrl Pts',(19.4540401875754,21.1100287955816,36.2486610432304));
#49634=CARTESIAN_POINT('Ctrl Pts',(19.3941040087494,21.1141809091495,36.2684889831927));
#49635=CARTESIAN_POINT('Origin',(20.,-0.075,38.1));
#49636=CARTESIAN_POINT('',(17.6365301745119,0.384026849772126,38.099091756019));
#49637=CARTESIAN_POINT('',(21.0904144288932,0.125000000000002,36.00310066666));
#49638=CARTESIAN_POINT('Ctrl Pts',(17.6365301745122,0.384026849728286,38.0990917552036));
#49639=CARTESIAN_POINT('Ctrl Pts',(17.6365466202516,0.381726187737689,38.056296014461));
#49640=CARTESIAN_POINT('Ctrl Pts',(17.6377253551942,0.379425525747093,38.0135219170556));
#49641=CARTESIAN_POINT('Ctrl Pts',(17.6400633130001,0.377124863756497,37.9708130259966));
#49642=CARTESIAN_POINT('Ctrl Pts',(17.6443776509738,0.372879349416942,37.8920004015614));
#49643=CARTESIAN_POINT('Ctrl Pts',(17.6526523098677,0.368633835077388,37.8132585686871));
#49644=CARTESIAN_POINT('Ctrl Pts',(17.6648817042177,0.364388320737833,37.7350164584497));
#49645=CARTESIAN_POINT('Ctrl Pts',(17.6770934799562,0.360148922814607,37.6568870698479));
#49646=CARTESIAN_POINT('Ctrl Pts',(17.6932486037894,0.355909524891381,37.5792564315695));
#49647=CARTESIAN_POINT('Ctrl Pts',(17.7132895602032,0.351670126968155,37.5025505833759));
#49648=CARTESIAN_POINT('Ctrl Pts',(17.7333070781187,0.34743568714769,37.4259344449676));
#49649=CARTESIAN_POINT('Ctrl Pts',(17.7572012787173,0.343201247327225,37.3502413964795));
#49650=CARTESIAN_POINT('Ctrl Pts',(17.7848634742222,0.33896680750676,37.2758879851228));
#49651=CARTESIAN_POINT('Ctrl Pts',(17.8125079350198,0.334735082458186,37.2015822430116));
#49652=CARTESIAN_POINT('Ctrl Pts',(17.8439154327941,0.330503357409613,37.1286148695029));
#49653=CARTESIAN_POINT('Ctrl Pts',(17.8789276000118,0.32627163236104,37.0573867855681));
#49654=CARTESIAN_POINT('Ctrl Pts',(17.9139281139794,0.322041315775697,36.9861824087825));
#49655=CARTESIAN_POINT('Ctrl Pts',(17.952530708808,0.317810999190353,36.9167165905492));
#49656=CARTESIAN_POINT('Ctrl Pts',(17.9945296831701,0.31358068260501,36.8493684598515));
#49657=CARTESIAN_POINT('Ctrl Pts',(18.0365276259034,0.309350469929734,36.7820219834388));
#49658=CARTESIAN_POINT('Ctrl Pts',(18.081921534115,0.305120257254458,36.7167934865995));
#49659=CARTESIAN_POINT('Ctrl Pts',(18.1304614998172,0.300890044579181,36.6540344965268));
#49660=CARTESIAN_POINT('Ctrl Pts',(18.1790478208794,0.296655792077581,36.591215572016));
#49661=CARTESIAN_POINT('Ctrl Pts',(18.2307859149217,0.292421539575981,36.5308712355465));
#49662=CARTESIAN_POINT('Ctrl Pts',(18.28538492457,0.28818728707438,36.4733206880248));
#49663=CARTESIAN_POINT('Ctrl Pts',(18.3400093704208,0.283951061949012,36.4157433292588));
#49664=CARTESIAN_POINT('Ctrl Pts',(18.3974970493029,0.279714836823644,36.3609626755641));
#49665=CARTESIAN_POINT('Ctrl Pts',(18.4575213005469,0.275478611698276,36.3092599567125));
#49666=CARTESIAN_POINT('Ctrl Pts',(18.5176502304147,0.271234998855322,36.2574670714806));
#49667=CARTESIAN_POINT('Ctrl Pts',(18.5803242023937,0.266991386012368,36.2087631341215));
#49668=CARTESIAN_POINT('Ctrl Pts',(18.645184842545,0.262747773169415,36.1633879247433));
#49669=CARTESIAN_POINT('Ctrl Pts',(18.7029885484259,0.258965871725414,36.1229496057401));
#49670=CARTESIAN_POINT('Ctrl Pts',(18.7625283691001,0.255183970281414,36.0851545808996));
#49671=CARTESIAN_POINT('Ctrl Pts',(18.8235345245485,0.251402068837414,36.0501416083128));
#49672=CARTESIAN_POINT('Ctrl Pts',(18.8919721557191,0.247159474393527,36.0108635242166));
#49673=CARTESIAN_POINT('Ctrl Pts',(18.962503989743,0.242916879949641,35.9749447688772));
#49674=CARTESIAN_POINT('Ctrl Pts',(19.0347671401997,0.238674285505754,35.9426136258746));
#49675=CARTESIAN_POINT('Ctrl Pts',(19.1069281207725,0.234437689490933,35.91032819454));
#49676=CARTESIAN_POINT('Ctrl Pts',(19.1808151329091,0.230201093476113,35.8816204907315));
#49677=CARTESIAN_POINT('Ctrl Pts',(19.2560395078073,0.225964497461293,35.8566736245129));
#49678=CARTESIAN_POINT('Ctrl Pts',(19.3311791878672,0.221732671413845,35.8317548458762));
#49679=CARTESIAN_POINT('Ctrl Pts',(19.4076527967903,0.217500845366396,35.8105886361722));
#49680=CARTESIAN_POINT('Ctrl Pts',(19.4850518236164,0.213269019318948,35.7933099868992));
#49681=CARTESIAN_POINT('Ctrl Pts',(19.5624033121621,0.209039792448016,35.7760419501274));
#49682=CARTESIAN_POINT('Ctrl Pts',(19.6406786352875,0.204810565577084,35.7626568355487));
#49683=CARTESIAN_POINT('Ctrl Pts',(19.7194554280259,0.200581338706152,35.7532394276288));
#49684=CARTESIAN_POINT('Ctrl Pts',(19.7982081837649,0.19635340229044,35.7438248932231));
#49685=CARTESIAN_POINT('Ctrl Pts',(19.8774616414621,0.192125465874728,35.7383757165539));
#49686=CARTESIAN_POINT('Ctrl Pts',(19.9567860404826,0.187897529459016,35.7369250975471));
#49687=CARTESIAN_POINT('Ctrl Pts',(20.036110751376,0.183669576420693,35.735474472837));
#49688=CARTESIAN_POINT('Ctrl Pts',(20.1155059368129,0.179441623382369,35.7380224440605));
#49689=CARTESIAN_POINT('Ctrl Pts',(20.1945410240051,0.175213670344046,35.7445501001127));
#49690=CARTESIAN_POINT('Ctrl Pts',(20.2736554109043,0.170981475196947,35.7510843056764));
#49691=CARTESIAN_POINT('Ctrl Pts',(20.3524085109971,0.166749280049848,35.7616061333742));
#49692=CARTESIAN_POINT('Ctrl Pts',(20.4303746581921,0.162517084902749,35.7760447305325));
#49693=CARTESIAN_POINT('Ctrl Pts',(20.5083791304018,0.158282809379141,35.7904904251229));
#49694=CARTESIAN_POINT('Ctrl Pts',(20.5855954237906,0.154048533855532,35.808856616531));
#49695=CARTESIAN_POINT('Ctrl Pts',(20.6616103489271,0.149814258331924,35.8310217746544));
#49696=CARTESIAN_POINT('Ctrl Pts',(20.7377615202967,0.145572393455453,35.8532266607561));
#49697=CARTESIAN_POINT('Ctrl Pts',(20.8127065783469,0.141330528578983,35.8792439652926));
#49698=CARTESIAN_POINT('Ctrl Pts',(20.8860499319902,0.137088663702512,35.908903023844));
#49699=CARTESIAN_POINT('Ctrl Pts',(20.951807402204,0.133285533774455,35.9354944539106));
#49700=CARTESIAN_POINT('Ctrl Pts',(21.0162774292693,0.129482403846397,35.9650124980401));
#49701=CARTESIAN_POINT('Ctrl Pts',(21.0791925799285,0.125679273918339,35.9973032039005));
#49702=CARTESIAN_POINT('Ctrl Pts',(21.0829383210873,0.125452849278894,35.9992256760669));
#49703=CARTESIAN_POINT('Ctrl Pts',(21.0866789488293,0.125226424639448,36.0011581693281));
#49704=CARTESIAN_POINT('Ctrl Pts',(21.0904144288932,0.125000000000002,36.0031006666601));
#49705=CARTESIAN_POINT('',(18.9094067387628,0.125,36.0031936714508));
#49706=CARTESIAN_POINT('Origin',(20.,0.125,38.1));
#49707=CARTESIAN_POINT('',(17.6361271868254,0.262848150271721,38.0978834451601));
#49708=CARTESIAN_POINT('Ctrl Pts',(18.9094067387628,0.124999999999998,36.0031936714508));
#49709=CARTESIAN_POINT('Ctrl Pts',(18.2138265225729,0.166907598306358,36.3649796342733));
#49710=CARTESIAN_POINT('Ctrl Pts',(17.6705484964577,0.212856981730266,37.1675355659372));
#49711=CARTESIAN_POINT('Ctrl Pts',(17.6334287363114,0.258806365154173,38.0226003826317));
#49712=CARTESIAN_POINT('Ctrl Pts',(17.6339392807276,0.262848150271721,38.0978814861616));
#49713=CARTESIAN_POINT('',(17.6365302632328,1.05659815022249,38.098884524413));
#49714=CARTESIAN_POINT('Ctrl Pts',(17.6365309473941,0.262848150271721,38.0978838066776));
#49715=CARTESIAN_POINT('Ctrl Pts',(17.6364618825206,0.26699404237924,38.175018863043));
#49716=CARTESIAN_POINT('Ctrl Pts',(17.6401730751359,0.271139934486759,38.2523306584864));
#49717=CARTESIAN_POINT('Ctrl Pts',(17.647689911148,0.275285826594278,38.3294072509425));
#49718=CARTESIAN_POINT('Ctrl Pts',(17.6553320274445,0.279500816729439,38.4077684500353));
#49719=CARTESIAN_POINT('Ctrl Pts',(17.6669078983962,0.283715806864601,38.4858860293951));
#49720=CARTESIAN_POINT('Ctrl Pts',(17.682388929481,0.287930796999763,38.5633242565501));
#49721=CARTESIAN_POINT('Ctrl Pts',(17.6975783227697,0.292066383481074,38.6393036717064));
#49722=CARTESIAN_POINT('Ctrl Pts',(17.7165269305249,0.296201969962385,38.7146286024622));
#49723=CARTESIAN_POINT('Ctrl Pts',(17.7391554804501,0.300337556443697,38.7888922262019));
#49724=CARTESIAN_POINT('Ctrl Pts',(17.7617717581082,0.304470900049416,38.8631155741379));
#49725=CARTESIAN_POINT('Ctrl Pts',(17.7880638787022,0.308604243655135,38.9362782884214));
#49726=CARTESIAN_POINT('Ctrl Pts',(17.8179020386913,0.312737587260854,39.0079861938116));
#49727=CARTESIAN_POINT('Ctrl Pts',(17.8477341671462,0.316870095345768,39.0796796040492));
#49728=CARTESIAN_POINT('Ctrl Pts',(17.8811107239061,0.321002603430683,39.1499183368414));
#49729=CARTESIAN_POINT('Ctrl Pts',(17.9178534771978,0.325135111515597,39.2183274558388));
#49730=CARTESIAN_POINT('Ctrl Pts',(17.955870911315,0.329410984709144,39.2891098262793));
#49731=CARTESIAN_POINT('Ctrl Pts',(17.9974921636746,0.333686857902691,39.3579327945156));
#49732=CARTESIAN_POINT('Ctrl Pts',(18.0424687398505,0.337962731096238,39.4244099842713));
#49733=CARTESIAN_POINT('Ctrl Pts',(18.085990774814,0.342100322670602,39.4887373035743));
#49734=CARTESIAN_POINT('Ctrl Pts',(18.1326540628943,0.346237914244966,39.5508678940322));
#49735=CARTESIAN_POINT('Ctrl Pts',(18.1821914387838,0.350375505819329,39.6104841858388));
#49736=CARTESIAN_POINT('Ctrl Pts',(18.234212182748,0.354720519822468,39.6730891138649));
#49737=CARTESIAN_POINT('Ctrl Pts',(18.2894023108564,0.359065533825606,39.7329205901025));
#49738=CARTESIAN_POINT('Ctrl Pts',(18.3474095171519,0.363410547828744,39.7896553307997));
#49739=CARTESIAN_POINT('Ctrl Pts',(18.4054167234473,0.367755561831882,39.8463900714969));
#49740=CARTESIAN_POINT('Ctrl Pts',(18.466240487423,0.372100575835021,39.9000277367094));
#49741=CARTESIAN_POINT('Ctrl Pts',(18.5294918301591,0.376445589838159,39.9502962366419));
#49742=CARTESIAN_POINT('Ctrl Pts',(18.5912586311502,0.380688624114211,39.9993849088683));
#49743=CARTESIAN_POINT('Ctrl Pts',(18.6556004960446,0.384931658390263,40.0454682312156));
#49744=CARTESIAN_POINT('Ctrl Pts',(18.7221932971537,0.389174692666315,40.0882656942826));
#49745=CARTESIAN_POINT('Ctrl Pts',(18.788690404912,0.39341162973425,40.1310016577194));
#49746=CARTESIAN_POINT('Ctrl Pts',(18.857431634827,0.397648566802186,40.1704608889279));
#49747=CARTESIAN_POINT('Ctrl Pts',(18.9280605298275,0.401885503870121,40.2064036206735));
#49748=CARTESIAN_POINT('Ctrl Pts',(18.9986074118953,0.406117521087132,40.2423046164009));
#49749=CARTESIAN_POINT('Ctrl Pts',(19.0710371882806,0.410349538304143,40.2746970170407));
#49750=CARTESIAN_POINT('Ctrl Pts',(19.1449665116178,0.414581555521154,40.3033856164196));
#49751=CARTESIAN_POINT('Ctrl Pts',(19.2188488338598,0.418810882203,40.3320559768166));
#49752=CARTESIAN_POINT('Ctrl Pts',(19.2942283760049,0.423040208884845,40.3570270416089));
#49753=CARTESIAN_POINT('Ctrl Pts',(19.3707004875316,0.427269535566691,40.3781511285486));
#49754=CARTESIAN_POINT('Ctrl Pts',(19.4471476170331,0.431497480605695,40.3992683146395));
#49755=CARTESIAN_POINT('Ctrl Pts',(19.5246861569039,0.435725425644699,40.416540894387));
#49756=CARTESIAN_POINT('Ctrl Pts',(19.6028963277898,0.439953370683703,40.4298710510278));
#49757=CARTESIAN_POINT('Ctrl Pts',(19.6811051208929,0.444181241241473,40.443200972839));
#49758=CARTESIAN_POINT('Ctrl Pts',(19.7599850605302,0.448409111799243,40.4525885324591));
#49759=CARTESIAN_POINT('Ctrl Pts',(19.8391076657526,0.452636982357013,40.457987298032));
#49760=CARTESIAN_POINT('Ctrl Pts',(19.9183070009431,0.456868952936158,40.4633912991139));
#49761=CARTESIAN_POINT('Ctrl Pts',(19.9977490044459,0.461100923515304,40.4647987472846));
#49762=CARTESIAN_POINT('Ctrl Pts',(20.077002187465,0.465332894094449,40.4622152958665));
#49763=CARTESIAN_POINT('Ctrl Pts',(20.1562928650638,0.469566866813471,40.4596306222208));
#49764=CARTESIAN_POINT('Ctrl Pts',(20.2353940777908,0.473800839532493,40.4530513257599));
#49765=CARTESIAN_POINT('Ctrl Pts',(20.3138789833638,0.478034812251516,40.4425350423638));
#49766=CARTESIAN_POINT('Ctrl Pts',(20.3925021979024,0.482276246231814,40.4320002267893));
#49767=CARTESIAN_POINT('Ctrl Pts',(20.4705064744765,0.486517680212112,40.4175146466936));
#49768=CARTESIAN_POINT('Ctrl Pts',(20.5474749282159,0.49075911419241,40.3991871702571));
#49769=CARTESIAN_POINT('Ctrl Pts',(20.616488844873,0.494562204380686,40.382753802171));
#49770=CARTESIAN_POINT('Ctrl Pts',(20.6846699260661,0.498365294568962,40.3632323758914));
#49771=CARTESIAN_POINT('Ctrl Pts',(20.7517303997312,0.502168384757237,40.3407346668046));
#49772=CARTESIAN_POINT('Ctrl Pts',(20.826578481796,0.506413120753787,40.3156243404981));
#49773=CARTESIAN_POINT('Ctrl Pts',(20.9003021434443,0.510657856750337,40.286714333335));
#49774=CARTESIAN_POINT('Ctrl Pts',(20.9724895378996,0.514902592746886,40.2541250055593));
#49775=CARTESIAN_POINT('Ctrl Pts',(21.0445757922291,0.51914138153983,40.2215813379537));
#49776=CARTESIAN_POINT('Ctrl Pts',(21.1151296321602,0.523380170332774,40.1853687790023));
#49777=CARTESIAN_POINT('Ctrl Pts',(21.1837559386883,0.527618959125719,40.1456569405744));
#49778=CARTESIAN_POINT('Ctrl Pts',(21.2523061311334,0.531853046638082,40.1059891469206));
#49779=CARTESIAN_POINT('Ctrl Pts',(21.3189326366379,0.536087134150445,40.0628300196778));
#49780=CARTESIAN_POINT('Ctrl Pts',(21.3832631957482,0.540321221662809,40.0163959330442));
#49781=CARTESIAN_POINT('Ctrl Pts',(21.4475548872188,0.544552750997682,39.9699899012477));
#49782=CARTESIAN_POINT('Ctrl Pts',(21.5095530083465,0.548784280332555,39.9203131106354));
#49783=CARTESIAN_POINT('Ctrl Pts',(21.5689136943686,0.553015809667429,39.8676255996456));
#49784=CARTESIAN_POINT('Ctrl Pts',(21.6282568153375,0.557246086876645,39.8149536790911));
#49785=CARTESIAN_POINT('Ctrl Pts',(21.6849637021973,0.561476364085862,39.7592731172668));
#49786=CARTESIAN_POINT('Ctrl Pts',(21.738724193471,0.565706641295079,39.7008836996918));
#49787=CARTESIAN_POINT('Ctrl Pts',(21.7924853496532,0.569936970824267,39.6424935599577));
#49788=CARTESIAN_POINT('Ctrl Pts',(21.8432997227037,0.574167300353455,39.5813948424348));
#49789=CARTESIAN_POINT('Ctrl Pts',(21.8908956101143,0.578397629882643,39.5179225058339));
#49790=CARTESIAN_POINT('Ctrl Pts',(21.9385396920706,0.582632242950196,39.4543858985452));
#49791=CARTESIAN_POINT('Ctrl Pts',(21.982958498106,0.586866856017749,39.3884712458543));
#49792=CARTESIAN_POINT('Ctrl Pts',(22.0239224456132,0.591101469085302,39.3205442945847));
#49793=CARTESIAN_POINT('Ctrl Pts',(22.0649067739001,0.595338188998541,39.2525835476406));
#49794=CARTESIAN_POINT('Ctrl Pts',(22.1024325983729,0.59957490891178,39.1826089195754));
#49795=CARTESIAN_POINT('Ctrl Pts',(22.1363165313248,0.603811628825019,39.1110104445001));
#49796=CARTESIAN_POINT('Ctrl Pts',(22.1702613067429,0.608055956252082,39.0392834061967));
#49797=CARTESIAN_POINT('Ctrl Pts',(22.2005509456261,0.612300283679145,38.9659271274026));
#49798=CARTESIAN_POINT('Ctrl Pts',(22.2270504962148,0.616544611106208,38.8913510777206));
#49799=CARTESIAN_POINT('Ctrl Pts',(22.250664678752,0.620326800629578,38.8248951412623));
#49800=CARTESIAN_POINT('Ctrl Pts',(22.2712698413409,0.624108990152948,38.7574710555183));
#49801=CARTESIAN_POINT('Ctrl Pts',(22.2888046377453,0.627891179676317,38.6893757469861));
#49802=CARTESIAN_POINT('Ctrl Pts',(22.3084266942537,0.632123583340497,38.6131746916016));
#49803=CARTESIAN_POINT('Ctrl Pts',(22.324276863283,0.636355987004676,38.5358461616176));
#49804=CARTESIAN_POINT('Ctrl Pts',(22.3362300683726,0.640588390668856,38.4577981393634));
#49805=CARTESIAN_POINT('Ctrl Pts',(22.348165852922,0.644814626049535,38.3798638638985));
#49806=CARTESIAN_POINT('Ctrl Pts',(22.3562158807938,0.649040861430213,38.3012126390911));
#49807=CARTESIAN_POINT('Ctrl Pts',(22.3603053973195,0.653267096810892,38.2222655809483));
#49808=CARTESIAN_POINT('Ctrl Pts',(22.3643901000154,0.657488357428077,38.1434114525425));
#49809=CARTESIAN_POINT('Ctrl Pts',(22.364523531154,0.661709618045262,38.0642626498012));
#49810=CARTESIAN_POINT('Ctrl Pts',(22.3606825622673,0.665930878662447,37.9852468688568));
#49811=CARTESIAN_POINT('Ctrl Pts',(22.3568440671912,0.670149420538699,37.906281978738));
#49812=CARTESIAN_POINT('Ctrl Pts',(22.349036275205,0.674367962414951,37.8274504086583));
#49813=CARTESIAN_POINT('Ctrl Pts',(22.3372881366587,0.678586504291203,37.7491800930187));
#49814=CARTESIAN_POINT('Ctrl Pts',(22.3255438813021,0.682803651785012,37.6709356485823));
#49815=CARTESIAN_POINT('Ctrl Pts',(22.309861935233,0.68702079927882,37.5932525547799));
#49816=CARTESIAN_POINT('Ctrl Pts',(22.2903229652327,0.691237946772629,37.5165523538245));
#49817=CARTESIAN_POINT('Ctrl Pts',(22.2707843277844,0.695455022490872,37.4398534583013));
#49818=CARTESIAN_POINT('Ctrl Pts',(22.2473889142856,0.699672098209116,37.3641378776005));
#49819=CARTESIAN_POINT('Ctrl Pts',(22.2202678816469,0.703889173927359,37.289814234495));
#49820=CARTESIAN_POINT('Ctrl Pts',(22.1931199610293,0.708110430483589,37.2154169064164));
#49821=CARTESIAN_POINT('Ctrl Pts',(22.1622392046997,0.71233168703982,37.1424147151563));
#49822=CARTESIAN_POINT('Ctrl Pts',(22.1278055815535,0.71655294359605,37.0711978576958));
#49823=CARTESIAN_POINT('Ctrl Pts',(22.0933554042309,0.720776229547382,36.9999467622923));
#49824=CARTESIAN_POINT('Ctrl Pts',(22.0553491836034,0.724999515498714,36.9304831233829));
#49825=CARTESIAN_POINT('Ctrl Pts',(22.0140124684469,0.729222801450046,36.8631717104463));
#49826=CARTESIAN_POINT('Ctrl Pts',(21.9726010402798,0.733453720673798,36.7957386371821));
#49827=CARTESIAN_POINT('Ctrl Pts',(21.9278473563894,0.737684639897551,36.7304659510557));
#49828=CARTESIAN_POINT('Ctrl Pts',(21.8800196967714,0.741915559121303,36.6676884484681));
#49829=CARTESIAN_POINT('Ctrl Pts',(21.8359388242095,0.745815030946001,36.6098288936955));
#49830=CARTESIAN_POINT('Ctrl Pts',(21.7892473922436,0.749714502770699,36.5540887381423));
#49831=CARTESIAN_POINT('Ctrl Pts',(21.7401831006425,0.753613974595397,36.5007022737657));
#49832=CARTESIAN_POINT('Ctrl Pts',(21.6868504876868,0.757852678849993,36.4426714829653));
#49833=CARTESIAN_POINT('Ctrl Pts',(21.6305121517996,0.762091383104589,36.3872028090615));
#49834=CARTESIAN_POINT('Ctrl Pts',(21.5714438914437,0.766330087359185,36.3346234008167));
#49835=CARTESIAN_POINT('Ctrl Pts',(21.5124604928476,0.770562701982907,36.2821195319746));
#49836=CARTESIAN_POINT('Ctrl Pts',(21.4507553057172,0.774795316606628,36.2324969942412));
#49837=CARTESIAN_POINT('Ctrl Pts',(21.3866424318643,0.779027931230349,36.1860477521491));
#49838=CARTESIAN_POINT('Ctrl Pts',(21.3226035729714,0.783255659521835,36.1396521332779));
#49839=CARTESIAN_POINT('Ctrl Pts',(21.2561629285916,0.787483387813321,36.096422803308));
#49840=CARTESIAN_POINT('Ctrl Pts',(21.1876681226633,0.791711116104807,36.0566119136812));
#49841=CARTESIAN_POINT('Ctrl Pts',(21.1192165382217,0.79593617662171,36.0168261454606));
#49842=CARTESIAN_POINT('Ctrl Pts',(21.0487137691173,0.800161237138613,35.980454770714));
#49843=CARTESIAN_POINT('Ctrl Pts',(20.9765358888945,0.804386297655516,35.9477063168329));
#49844=CARTESIAN_POINT('Ctrl Pts',(20.9043811128216,0.808610005729933,35.9149683457366));
#49845=CARTESIAN_POINT('Ctrl Pts',(20.8305527167774,0.81283371380435,35.8858511859687));
#49846=CARTESIAN_POINT('Ctrl Pts',(20.7554494762376,0.817057421878768,35.8605164591468));
#49847=CARTESIAN_POINT('Ctrl Pts',(20.6803469258958,0.82128109113735,35.8351819651508));
#49848=CARTESIAN_POINT('Ctrl Pts',(20.603969998732,0.825504760395932,35.8136299833845));
#49849=CARTESIAN_POINT('Ctrl Pts',(20.5267340449842,0.829728429654514,35.7959727243901));
#49850=CARTESIAN_POINT('Ctrl Pts',(20.4494215288891,0.833956285746006,35.7782979621328));
#49851=CARTESIAN_POINT('Ctrl Pts',(20.3712487430369,0.838184141837497,35.7645257392072));
#49852=CARTESIAN_POINT('Ctrl Pts',(20.292642094316,0.842411997928989,35.7547172781231));
#49853=CARTESIAN_POINT('Ctrl Pts',(20.2139974548782,0.846641897349977,35.7449040765943));
#49854=CARTESIAN_POINT('Ctrl Pts',(20.1349190026683,0.850871796770964,35.7390584878856));
#49855=CARTESIAN_POINT('Ctrl Pts',(20.0558365932587,0.855101696191952,35.7371896572612));
#49856=CARTESIAN_POINT('Ctrl Pts',(19.9766124765105,0.85933917514667,35.7353174778894));
#49857=CARTESIAN_POINT('Ctrl Pts',(19.8973848578431,0.863576654101389,35.7374362824276));
#49858=CARTESIAN_POINT('Ctrl Pts',(19.8185816833028,0.867814133056107,35.7435030585068));
#49859=CARTESIAN_POINT('Ctrl Pts',(19.7471539671461,0.871655011875563,35.749002024282));
#49860=CARTESIAN_POINT('Ctrl Pts',(19.6760751522037,0.87549589069502,35.7577438284633));
#49861=CARTESIAN_POINT('Ctrl Pts',(19.6056561338333,0.879336769514476,35.7696602487799));
#49862=CARTESIAN_POINT('Ctrl Pts',(19.5279481238012,0.883575213286357,35.7828101240683));
#49863=CARTESIAN_POINT('Ctrl Pts',(19.450753377928,0.887813657058239,35.7998757220939));
#49864=CARTESIAN_POINT('Ctrl Pts',(19.3744964180902,0.89205210083012,35.8208037140435));
#49865=CARTESIAN_POINT('Ctrl Pts',(19.2983487787586,0.896284468450797,35.8417017040277));
#49866=CARTESIAN_POINT('Ctrl Pts',(19.223136703738,0.900516836071473,35.8664509687147));
#49867=CARTESIAN_POINT('Ctrl Pts',(19.1492760415994,0.904749203692149,35.8949468968972));
#49868=CARTESIAN_POINT('Ctrl Pts',(19.0755002743758,0.908976706659862,35.9234100720644));
#49869=CARTESIAN_POINT('Ctrl Pts',(19.003073268172,0.913204209627575,35.9556111849861));
#49870=CARTESIAN_POINT('Ctrl Pts',(18.9323957143926,0.917431712595288,35.9913958336728));
#49871=CARTESIAN_POINT('Ctrl Pts',(18.8617625388377,0.92165656112653,36.0271580132855));
#49872=CARTESIAN_POINT('Ctrl Pts',(18.7928770522779,0.925881409657772,36.0664990513099));
#49873=CARTESIAN_POINT('Ctrl Pts',(18.7261188279924,0.930106258189014,36.1092169378598));
#49874=CARTESIAN_POINT('Ctrl Pts',(18.6593817580276,0.93432976795186,36.151921287982));
#49875=CARTESIAN_POINT('Ctrl Pts',(18.5947710061138,0.938553277714706,36.1980001093094));
#49876=CARTESIAN_POINT('Ctrl Pts',(18.532639145738,0.942776787477552,36.2472068209648));
#49877=CARTESIAN_POINT('Ctrl Pts',(18.4705076500873,0.947000272447639,36.296413243768));
#49878=CARTESIAN_POINT('Ctrl Pts',(18.4108553834613,0.951223757417726,36.3487472283445));
#49879=CARTESIAN_POINT('Ctrl Pts',(18.354002482924,0.955447242387812,36.4039214007954));
#49880=CARTESIAN_POINT('Ctrl Pts',(18.2970929061349,0.959674937720001,36.4591505759862));
#49881=CARTESIAN_POINT('Ctrl Pts',(18.2429886068065,0.96390263305219,36.5172252675961));
#49882=CARTESIAN_POINT('Ctrl Pts',(18.1919729611805,0.968130328384379,36.5778210789143));
#49883=CARTESIAN_POINT('Ctrl Pts',(18.1409325062355,0.97236007967883,36.6384463584632));
#49884=CARTESIAN_POINT('Ctrl Pts',(18.0929839809455,0.976589830973282,36.7015948264862));
#49885=CARTESIAN_POINT('Ctrl Pts',(18.0483689442624,0.980819582267733,36.7669108570016));
#49886=CARTESIAN_POINT('Ctrl Pts',(18.0036737137948,0.985056936374789,36.8323442905284));
#49887=CARTESIAN_POINT('Ctrl Pts',(17.9623241892086,0.989294290481844,36.8999526706709));
#49888=CARTESIAN_POINT('Ctrl Pts',(17.9245171304773,0.9935316445889,36.969353592312));
#49889=CARTESIAN_POINT('Ctrl Pts',(17.8902318405216,0.997374284537119,37.0322897423725));
#49890=CARTESIAN_POINT('Ctrl Pts',(17.8588592969497,1.00121692448534,37.0966994897598));
#49891=CARTESIAN_POINT('Ctrl Pts',(17.830511574449,1.00505956443356,37.1622844715479));
#49892=CARTESIAN_POINT('Ctrl Pts',(17.7960497203405,1.00973099781886,37.2420150415799));
#49893=CARTESIAN_POINT('Ctrl Pts',(17.7659475077993,1.01440243120416,37.3237385639075));
#49894=CARTESIAN_POINT('Ctrl Pts',(17.7404156919232,1.01907386458946,37.4069854290183));
#49895=CARTESIAN_POINT('Ctrl Pts',(17.7149582744737,1.02373168565296,37.4899897169534));
#49896=CARTESIAN_POINT('Ctrl Pts',(17.6940448157563,1.02838950671645,37.5745082191302));
#49897=CARTESIAN_POINT('Ctrl Pts',(17.6778379434104,1.03304732777995,37.6600524760432));
#49898=CARTESIAN_POINT('Ctrl Pts',(17.6617109571308,1.03768218975585,37.7451750726861));
#49899=CARTESIAN_POINT('Ctrl Pts',(17.6502443976019,1.04231705173175,37.8313130549651));
#49900=CARTESIAN_POINT('Ctrl Pts',(17.6435505015056,1.04695191370765,37.9179664812586));
#49901=CARTESIAN_POINT('Ctrl Pts',(17.6389066447746,1.05016732587926,37.9780818596809));
#49902=CARTESIAN_POINT('Ctrl Pts',(17.6365587886261,1.05338273805088,38.0384449196041));
#49903=CARTESIAN_POINT('Ctrl Pts',(17.6365302632328,1.05659815022249,38.098884524413));
#49904=CARTESIAN_POINT('',(17.6365309191062,1.85034815030119,38.102084360615));
#49905=CARTESIAN_POINT('Ctrl Pts',(17.6365302632324,1.05659815027172,38.0988845253384));
#49906=CARTESIAN_POINT('Ctrl Pts',(17.6364922090284,1.06088766352129,38.1795138418281));
#49907=CARTESIAN_POINT('Ctrl Pts',(17.6405844802438,1.06517717677086,38.2601328060387));
#49908=CARTESIAN_POINT('Ctrl Pts',(17.6487775398017,1.06946669002043,38.3402985300805));
#49909=CARTESIAN_POINT('Ctrl Pts',(17.656974087378,1.07375802943784,38.4204983829519));
#49910=CARTESIAN_POINT('Ctrl Pts',(17.6692748484675,1.07804936885525,38.5002441667311));
#49911=CARTESIAN_POINT('Ctrl Pts',(17.6855986141635,1.08234070827266,38.5790998498624));
#49912=CARTESIAN_POINT('Ctrl Pts',(17.7019469595511,1.08663850942208,38.6580742708148));
#49913=CARTESIAN_POINT('Ctrl Pts',(17.7223303146537,1.0909363105715,38.7361554754159));
#49914=CARTESIAN_POINT('Ctrl Pts',(17.7466167131606,1.09523411172092,38.8129194929954));
#49915=CARTESIAN_POINT('Ctrl Pts',(17.770922240334,1.09953529794223,38.8897439721246));
#49916=CARTESIAN_POINT('Ctrl Pts',(17.7991367774029,1.10383648416353,38.9652487783743));
#49917=CARTESIAN_POINT('Ctrl Pts',(17.8310799063504,1.10813767038484,39.0390293223658));
#49918=CARTESIAN_POINT('Ctrl Pts',(17.8630887408235,1.1124477039455,39.1129616294936));
#49919=CARTESIAN_POINT('Ctrl Pts',(17.8988412914902,1.11675773750616,39.1851621864708));
#49920=CARTESIAN_POINT('Ctrl Pts',(17.9381108110437,1.12106777106683,39.2552503682601));
#49921=CARTESIAN_POINT('Ctrl Pts',(17.967614619562,1.1243059671621,39.3079087230966));
#49922=CARTESIAN_POINT('Ctrl Pts',(17.999102709071,1.12754416325737,39.359375209935));
#49923=CARTESIAN_POINT('Ctrl Pts',(18.0324634928686,1.13078235935264,39.4095001084404));
#49924=CARTESIAN_POINT('Ctrl Pts',(18.0761228872686,1.135020199846,39.4750987684232));
#49925=CARTESIAN_POINT('Ctrl Pts',(18.1231484012448,1.13925804033936,39.5386346470832));
#49926=CARTESIAN_POINT('Ctrl Pts',(18.173318584529,1.14349588083273,39.5997417935341));
#49927=CARTESIAN_POINT('Ctrl Pts',(18.2234166423239,1.14772762893617,39.6607610913357));
#49928=CARTESIAN_POINT('Ctrl Pts',(18.2766500964784,1.15195937703962,39.7193582316383));
#49929=CARTESIAN_POINT('Ctrl Pts',(18.3327541842083,1.15619112514307,39.7751960573691));
#49930=CARTESIAN_POINT('Ctrl Pts',(18.3887934905289,1.16041798699639,39.8309694091341));
#49931=CARTESIAN_POINT('Ctrl Pts',(18.44769651288,1.16464484884972,39.8839894489175));
#49932=CARTESIAN_POINT('Ctrl Pts',(18.5091591799931,1.16887171070304,39.9339531319805));
#49933=CARTESIAN_POINT('Ctrl Pts',(18.5705830619685,1.17309590525559,39.9838852861754));
#49934=CARTESIAN_POINT('Ctrl Pts',(18.6345630198887,1.17732009980815,40.0307646169701));
#49935=CARTESIAN_POINT('Ctrl Pts',(18.7007600941331,1.1815442943607,40.0743267480088));
#49936=CARTESIAN_POINT('Ctrl Pts',(18.7669360012338,1.18576713818689,40.117874949642));
#49937=CARTESIAN_POINT('Ctrl Pts',(18.8353272255652,1.18998998201307,40.1581078004002));
#49938=CARTESIAN_POINT('Ctrl Pts',(18.9055650888976,1.19421282583926,40.1948037297705));
#49939=CARTESIAN_POINT('Ctrl Pts',(18.9758023558371,1.19843563380909,40.2314993475539));
#49940=CARTESIAN_POINT('Ctrl Pts',(19.0478858144988,1.20265844177892,40.2646578878824));
#49941=CARTESIAN_POINT('Ctrl Pts',(19.1214227338433,1.20688124974875,40.294104014921));
#49942=CARTESIAN_POINT('Ctrl Pts',(19.1950327513745,1.21110825533262,40.3235794124066));
#49943=CARTESIAN_POINT('Ctrl Pts',(19.2700986794169,1.2153352609165,40.3493348506362));
#49944=CARTESIAN_POINT('Ctrl Pts',(19.346208941088,1.21956226650037,40.3712436443911));
#49945=CARTESIAN_POINT('Ctrl Pts',(19.4223560763857,1.22379131996875,40.3931630524397));
#49946=CARTESIAN_POINT('Ctrl Pts',(19.4995480962676,1.22802037343713,40.4112319965042));
#49947=CARTESIAN_POINT('Ctrl Pts',(19.5773619293001,1.23224942690551,40.4253747014396));
#49948=CARTESIAN_POINT('Ctrl Pts',(19.6553155498996,1.23648607759758,40.4395428128385));
#49949=CARTESIAN_POINT('Ctrl Pts',(19.7338927497158,1.24072272828964,40.4497705314025));
#49950=CARTESIAN_POINT('Ctrl Pts',(19.8126642430962,1.24495937898171,40.4560339036366));
#49951=CARTESIAN_POINT('Ctrl Pts',(19.8842206074614,1.24880797074504,40.4617235779911));
#49952=CARTESIAN_POINT('Ctrl Pts',(19.9559370023904,1.25265656250838,40.4641425402918));
#49953=CARTESIAN_POINT('Ctrl Pts',(20.0274937259456,1.25650515427172,40.4633100803605));
#49954=CARTESIAN_POINT('Ctrl Pts',(20.1062856091861,1.26074288034121,40.462393449715));
#49955=CARTESIAN_POINT('Ctrl Pts',(20.1851794264319,1.2649806064107,40.4575304519096));
#49956=CARTESIAN_POINT('Ctrl Pts',(20.2637476697309,1.26921833248019,40.4487076462624));
#49957=CARTESIAN_POINT('Ctrl Pts',(20.3422029700115,1.27344996675542,40.4398975235296));
#49958=CARTESIAN_POINT('Ctrl Pts',(20.4203331638077,1.27768160103065,40.4271389491961));
#49959=CARTESIAN_POINT('Ctrl Pts',(20.4977113197383,1.28191323530589,40.410470489555));
#49960=CARTESIAN_POINT('Ctrl Pts',(20.5750001542058,1.28613998479471,40.3938212711478));
#49961=CARTESIAN_POINT('Ctrl Pts',(20.6515382200484,1.29036673428353,40.3732712348634));
#49962=CARTESIAN_POINT('Ctrl Pts',(20.7269058037042,1.29459348377236,40.3489104903133));
#49963=CARTESIAN_POINT('Ctrl Pts',(20.8022258433493,1.29881756690765,40.3245651132122));
#49964=CARTESIAN_POINT('Ctrl Pts',(20.8763764215342,1.30304165004293,40.2964139431262));
#49965=CARTESIAN_POINT('Ctrl Pts',(20.9489512710763,1.30726573317822,40.264597405067));
#49966=CARTESIAN_POINT('Ctrl Pts',(21.0215029325541,1.31148846669568,40.232791032567));
#49967=CARTESIAN_POINT('Ctrl Pts',(21.0924794361512,1.31571120021313,40.1973218057531));
#49968=CARTESIAN_POINT('Ctrl Pts',(21.1614942462938,1.31993393373059,40.1583783803583));
#49969=CARTESIAN_POINT('Ctrl Pts',(21.2305084911823,1.32415663266246,40.119435273923));
#49970=CARTESIAN_POINT('Ctrl Pts',(21.2975606670246,1.32837933159433,40.0770182570923));
#49971=CARTESIAN_POINT('Ctrl Pts',(21.362289930623,1.3326020305262,40.0313613296903));
#49972=CARTESIAN_POINT('Ctrl Pts',(21.4270835816442,1.33682892985657,39.9856589864791));
#49973=CARTESIAN_POINT('Ctrl Pts',(21.4895493209607,1.34105582918694,39.9367105659571));
#49974=CARTESIAN_POINT('Ctrl Pts',(21.5493568587223,1.34528272851731,39.884792359136));
#49975=CARTESIAN_POINT('Ctrl Pts',(21.6091933917337,1.34951167708774,39.832848981886));
#49976=CARTESIAN_POINT('Ctrl Pts',(21.6663688174055,1.35374062565816,39.777933275252));
#49977=CARTESIAN_POINT('Ctrl Pts',(21.7205892967737,1.35796957422859,39.720358883929));
#49978=CARTESIAN_POINT('Ctrl Pts',(21.7749072275994,1.36220612356548,39.6626810131014));
#49979=CARTESIAN_POINT('Ctrl Pts',(21.8262592957658,1.36644267290238,39.6023352675118));
#49980=CARTESIAN_POINT('Ctrl Pts',(21.8743917519422,1.37067922223927,39.5396687122915));
#49981=CARTESIAN_POINT('Ctrl Pts',(21.9181277069757,1.37452879788978,39.4827262277615));
#49982=CARTESIAN_POINT('Ctrl Pts',(21.9592057467301,1.37837837354028,39.4238681546416));
#49983=CARTESIAN_POINT('Ctrl Pts',(21.9974679156332,1.38222794919079,39.3633734075545));
#49984=CARTESIAN_POINT('Ctrl Pts',(22.0395862130507,1.38646549182956,39.2967818937159));
#49985=CARTESIAN_POINT('Ctrl Pts',(22.0784499280056,1.39070303446833,39.2279568106674));
#49986=CARTESIAN_POINT('Ctrl Pts',(22.1138150633832,1.3949405771071,39.1572494117824));
#49987=CARTESIAN_POINT('Ctrl Pts',(22.1491293279213,1.39917202426938,39.0866437216765));
#49988=CARTESIAN_POINT('Ctrl Pts',(22.1809547990065,1.40340347143165,39.0141615086005));
#49989=CARTESIAN_POINT('Ctrl Pts',(22.209091417091,1.40763491859393,38.9401818564066));
#49990=CARTESIAN_POINT('Ctrl Pts',(22.2371955231821,1.41186147629926,38.8662876880461));
#49991=CARTESIAN_POINT('Ctrl Pts',(22.2616190810898,1.41608803400459,38.7908999550597));
#49992=CARTESIAN_POINT('Ctrl Pts',(22.2822091960486,1.42031459170992,38.714419747706));
#49993=CARTESIAN_POINT('Ctrl Pts',(22.3027863081582,1.42453848030471,38.6379878383152));
#49994=CARTESIAN_POINT('Ctrl Pts',(22.3195346608879,1.4287623688995,38.5604652754409));
#49995=CARTESIAN_POINT('Ctrl Pts',(22.3323508852338,1.43298625749429,38.4822692624957));
#49996=CARTESIAN_POINT('Ctrl Pts',(22.3451630069937,1.43720879398521,38.4040982807816));
#49997=CARTESIAN_POINT('Ctrl Pts',(22.3540454241433,1.44143133047612,38.3252547393824));
#49998=CARTESIAN_POINT('Ctrl Pts',(22.3589459666818,1.44565386696704,38.2461655471566));
#49999=CARTESIAN_POINT('Ctrl Pts',(22.3638464665078,1.4498763666548,38.1670770442634));
#50000=CARTESIAN_POINT('Ctrl Pts',(22.3647651331607,1.45409886634255,38.0877433627901));
#50001=CARTESIAN_POINT('Ctrl Pts',(22.3617018193823,1.45832136603031,38.0085945448767));
#50002=CARTESIAN_POINT('Ctrl Pts',(22.3586354598535,1.46254806400814,37.9293670319435));
#50003=CARTESIAN_POINT('Ctrl Pts',(22.3515792296434,1.46677476198598,37.8503252192567));
#50004=CARTESIAN_POINT('Ctrl Pts',(22.3405850896208,1.47100145996381,37.7718965420103));
#50005=CARTESIAN_POINT('Ctrl Pts',(22.3295856231211,1.47523020570618,37.6934298673803));
#50006=CARTESIAN_POINT('Ctrl Pts',(22.31464453462,1.47945895144855,37.6155773809426));
#50007=CARTESIAN_POINT('Ctrl Pts',(22.2958649617504,1.48368769719093,37.5387562754857));
#50008=CARTESIAN_POINT('Ctrl Pts',(22.2770516350047,1.48792404356196,37.4617970939344));
#50009=CARTESIAN_POINT('Ctrl Pts',(22.2543861730742,1.492160389933,37.3858734476615));
#50010=CARTESIAN_POINT('Ctrl Pts',(22.228021571741,1.49639673630403,37.3113870932095));
#50011=CARTESIAN_POINT('Ctrl Pts',(22.2040530555621,1.50024807223931,37.2436702569397));
#50012=CARTESIAN_POINT('Ctrl Pts',(22.1770279440483,1.50409940817459,37.1771413418693));
#50013=CARTESIAN_POINT('Ctrl Pts',(22.1470944454545,1.50795074410987,37.1120850830167));
#50014=CARTESIAN_POINT('Ctrl Pts',(22.1141582190445,1.51218842023544,37.0405028166052));
#50015=CARTESIAN_POINT('Ctrl Pts',(22.0775765256762,1.51642609636102,36.9704351006756));
#50016=CARTESIAN_POINT('Ctrl Pts',(22.0375112375595,1.52066377248659,36.9022778294952));
#50017=CARTESIAN_POINT('Ctrl Pts',(21.9975035613329,1.52489535504482,36.8342185650784));
#50018=CARTESIAN_POINT('Ctrl Pts',(21.9540224738326,1.52912693760305,36.76806469065));
#50019=CARTESIAN_POINT('Ctrl Pts',(21.9072771086963,1.53335852016128,36.7041903885046));
#50020=CARTESIAN_POINT('Ctrl Pts',(21.8605857316504,1.53758521549571,36.6403898573435));
#50021=CARTESIAN_POINT('Ctrl Pts',(21.8106378444394,1.54181191083013,36.5788640428588));
#50022=CARTESIAN_POINT('Ctrl Pts',(21.7576867131067,1.54603860616456,36.5199595386611));
#50023=CARTESIAN_POINT('Ctrl Pts',(21.7047690035798,1.55026263368459,36.4610922139315));
#50024=CARTESIAN_POINT('Ctrl Pts',(21.6488521250394,1.55448666120462,36.4048432631426));
#50025=CARTESIAN_POINT('Ctrl Pts',(21.5902298172869,1.55871068872465,36.3515265031715));
#50026=CARTESIAN_POINT('Ctrl Pts',(21.5316262591519,1.56293336524191,36.2982267959044));
#50027=CARTESIAN_POINT('Ctrl Pts',(21.4703193366545,1.56715604175917,36.2478577322939));
#50028=CARTESIAN_POINT('Ctrl Pts',(21.4066387990038,1.57137871827643,36.2006954614815));
#50029=CARTESIAN_POINT('Ctrl Pts',(21.3429588026859,1.57560135889775,36.153533591584));
#50030=CARTESIAN_POINT('Ctrl Pts',(21.2769056088874,1.57982399951907,36.109578738123));
#50031=CARTESIAN_POINT('Ctrl Pts',(21.2088399116202,1.58404664014039,36.0690651145411));
#50032=CARTESIAN_POINT('Ctrl Pts',(21.1407065340248,1.58827347949492,36.0285112067125));
#50033=CARTESIAN_POINT('Ctrl Pts',(21.0705570594829,1.59250031884945,35.9914056040329));
#50034=CARTESIAN_POINT('Ctrl Pts',(20.9987783582249,1.59672715820398,35.9579373883937));
#50035=CARTESIAN_POINT('Ctrl Pts',(20.9269648746004,1.6009560457911,35.9244529547995));
#50036=CARTESIAN_POINT('Ctrl Pts',(20.8535210263446,1.60518493337822,35.89460959624));
#50037=CARTESIAN_POINT('Ctrl Pts',(20.7788529481758,1.60941382096534,35.8685478884776));
#50038=CARTESIAN_POINT('Ctrl Pts',(20.704050683485,1.61365030831573,35.8424393450391));
#50039=CARTESIAN_POINT('Ctrl Pts',(20.6280202437852,1.61788679566611,35.8201261638457));
#50040=CARTESIAN_POINT('Ctrl Pts',(20.5511819536775,1.62212328301649,35.8016986936348));
#50041=CARTESIAN_POINT('Ctrl Pts',(20.4813519389428,1.62597336835398,35.7849519581914));
#50042=CARTESIAN_POINT('Ctrl Pts',(20.4108551177745,1.62982345369147,35.7714138383846));
#50043=CARTESIAN_POINT('Ctrl Pts',(20.340010694254,1.63367353902895,35.7611149731778));
#50044=CARTESIAN_POINT('Ctrl Pts',(20.2620347941965,1.63791118900294,35.7497793839507));
#50045=CARTESIAN_POINT('Ctrl Pts',(20.1833450394548,1.64214883897692,35.7423262308307));
#50046=CARTESIAN_POINT('Ctrl Pts',(20.1043616405112,1.64638648895091,35.7388352262305));
#50047=CARTESIAN_POINT('Ctrl Pts',(20.0254918181876,1.65061804526513,35.7353492416284));
#50048=CARTESIAN_POINT('Ctrl Pts',(19.9463296546664,1.65484960157934,35.7358141113773));
#50049=CARTESIAN_POINT('Ctrl Pts',(19.8673028734806,1.65908115789356,35.7402580832825));
#50050=CARTESIAN_POINT('Ctrl Pts',(19.7883673642613,1.66330782697259,35.7446969226232));
#50051=CARTESIAN_POINT('Ctrl Pts',(19.7095673923144,1.66753449605162,35.7531057051948));
#50052=CARTESIAN_POINT('Ctrl Pts',(19.6313315611324,1.67176116513065,35.7654606400656));
#50053=CARTESIAN_POINT('Ctrl Pts',(19.553145111207,1.67598516640098,35.7778077766911));
#50054=CARTESIAN_POINT('Ctrl Pts',(19.4755225570951,1.68020916767132,35.7940960488192));
#50055=CARTESIAN_POINT('Ctrl Pts',(19.3988870385322,1.68443316894165,35.8142498718243));
#50056=CARTESIAN_POINT('Ctrl Pts',(19.3222760302581,1.68865581925237,35.834397249045));
#50057=CARTESIAN_POINT('Ctrl Pts',(19.2466518836787,1.69287846956309,35.8584076029226));
#50058=CARTESIAN_POINT('Ctrl Pts',(19.172425741671,1.69710111987381,35.8861546377736));
#50059=CARTESIAN_POINT('Ctrl Pts',(19.098200229228,1.70132373436923,35.9139014372824));
#50060=CARTESIAN_POINT('Ctrl Pts',(19.0253731363741,1.70554634886465,35.945384689268));
#50061=CARTESIAN_POINT('Ctrl Pts',(18.9543372719364,1.70976896336007,35.980429312328));
#50062=CARTESIAN_POINT('Ctrl Pts',(18.8832307681291,1.71399577690097,36.0155087844053));
#50063=CARTESIAN_POINT('Ctrl Pts',(18.8139194721272,1.71822259044188,36.054156493825));
#50064=CARTESIAN_POINT('Ctrl Pts',(18.7467725820626,1.72244940398278,36.0961508340621));
#50065=CARTESIAN_POINT('Ctrl Pts',(18.6795931518429,1.72667826588613,36.1381655252394));
#50066=CARTESIAN_POINT('Ctrl Pts',(18.614580602009,1.73090712778948,36.1835298094884));
#50067=CARTESIAN_POINT('Ctrl Pts',(18.552073926742,1.73513598969284,36.2319795163651));
#50068=CARTESIAN_POINT('Ctrl Pts',(18.489454911885,1.73937245188225,36.280516299065));
#50069=CARTESIAN_POINT('Ctrl Pts',(18.4293511267712,1.74360891407166,36.3321492781482));
#50070=CARTESIAN_POINT('Ctrl Pts',(18.3720671557503,1.74784537626107,36.3865750394274));
#50071=CARTESIAN_POINT('Ctrl Pts',(18.3200044757893,1.75169569549006,36.4360400283347));
#50072=CARTESIAN_POINT('Ctrl Pts',(18.2702707099253,1.75554601471904,36.4878112278055));
#50073=CARTESIAN_POINT('Ctrl Pts',(18.2230653501685,1.75939633394803,36.5416374968807));
#50074=CARTESIAN_POINT('Ctrl Pts',(18.1715836395797,1.76359545500637,36.6003399073884));
#50075=CARTESIAN_POINT('Ctrl Pts',(18.1229080755859,1.76779457606471,36.6617171330744));
#50076=CARTESIAN_POINT('Ctrl Pts',(18.0773323538624,1.77199369712305,36.7254675109712));
#50077=CARTESIAN_POINT('Ctrl Pts',(18.0318175156023,1.77618720868092,36.7891327263375));
#50078=CARTESIAN_POINT('Ctrl Pts',(17.989394580521,1.78038072023878,36.8551644206018));
#50079=CARTESIAN_POINT('Ctrl Pts',(17.9503186160587,1.78457423179664,36.923226162245));
#50080=CARTESIAN_POINT('Ctrl Pts',(17.911282140254,1.78876350555401,36.9912191233261));
#50081=CARTESIAN_POINT('Ctrl Pts',(17.8755861597843,1.79295277931138,37.0612376488103));
#50082=CARTESIAN_POINT('Ctrl Pts',(17.8434428890811,1.79714205306875,37.1329157905098));
#50083=CARTESIAN_POINT('Ctrl Pts',(17.8113216485129,1.80132845561033,37.204544805935));
#50084=CARTESIAN_POINT('Ctrl Pts',(17.7827484780239,1.80551485815192,37.27783074427));
#50085=CARTESIAN_POINT('Ctrl Pts',(17.7578892482021,1.80970126069351,37.3523839103041));
#50086=CARTESIAN_POINT('Ctrl Pts',(17.7330335636422,1.81388706619755,37.4269264440499));
#50087=CARTESIAN_POINT('Ctrl Pts',(17.7118909287193,1.8180728717016,37.5027353967955));
#50088=CARTESIAN_POINT('Ctrl Pts',(17.6945782475928,1.82225867720565,37.5794032420121));
#50089=CARTESIAN_POINT('Ctrl Pts',(17.6772666835378,1.82644421262763,37.6560661403648));
#50090=CARTESIAN_POINT('Ctrl Pts',(17.6637846795615,1.83062974804961,37.7335873531143));
#50091=CARTESIAN_POINT('Ctrl Pts',(17.6541982053108,1.8348152834716,37.8115483039864));
#50092=CARTESIAN_POINT('Ctrl Pts',(17.6446061767769,1.83900324394048,37.8895544244588));
#50093=CARTESIAN_POINT('Ctrl Pts',(17.638914228829,1.84319120440936,37.9680003158431));
#50094=CARTESIAN_POINT('Ctrl Pts',(17.6371364426992,1.84737916487824,38.0464626253931));
#50095=CARTESIAN_POINT('Ctrl Pts',(17.636716331996,1.84836882667607,38.0650041448052));
#50096=CARTESIAN_POINT('Ctrl Pts',(17.6365145705078,1.84935848847389,38.0835465812456));
#50097=CARTESIAN_POINT('Ctrl Pts',(17.6365309191057,1.85034815027172,38.1020843600629));
#50098=CARTESIAN_POINT('',(17.6365300584559,2.64409815030312,38.0994743406844));
#50099=CARTESIAN_POINT('Ctrl Pts',(17.6365309191062,1.85034815030119,38.102084360615));
#50100=CARTESIAN_POINT('Ctrl Pts',(17.6366171557615,1.8555684817835,38.1998686244756));
#50101=CARTESIAN_POINT('Ctrl Pts',(17.6427755898215,1.86078881326582,38.2973860103044));
#50102=CARTESIAN_POINT('Ctrl Pts',(17.6548850483977,1.86600914474813,38.3939835108835));
#50103=CARTESIAN_POINT('Ctrl Pts',(17.6672029815152,1.87131934863924,38.4922440188962));
#50104=CARTESIAN_POINT('Ctrl Pts',(17.6856785644927,1.87662955253035,38.5895528165203));
#50105=CARTESIAN_POINT('Ctrl Pts',(17.7101357563283,1.88193975642146,38.6852454070336));
#50106=CARTESIAN_POINT('Ctrl Pts',(17.7150168320469,1.88299954723668,38.704343379652));
#50107=CARTESIAN_POINT('Ctrl Pts',(17.7201360078384,1.8840593380519,38.7233770457282));
#50108=CARTESIAN_POINT('Ctrl Pts',(17.7254916586676,1.88511912886712,38.7423412224896));
#50109=CARTESIAN_POINT('Ctrl Pts',(17.7469066035976,1.88935677666546,38.8181708114481));
#50110=CARTESIAN_POINT('Ctrl Pts',(17.7721580043752,1.8935944244638,38.8930706393473));
#50111=CARTESIAN_POINT('Ctrl Pts',(17.8011474670498,1.89783207226214,38.9666244741747));
#50112=CARTESIAN_POINT('Ctrl Pts',(17.8300952422087,1.90206362622524,39.0400725368917));
#50113=CARTESIAN_POINT('Ctrl Pts',(17.8627702337122,1.90629518018834,39.1121780178797));
#50114=CARTESIAN_POINT('Ctrl Pts',(17.899023986667,1.91052673415144,39.1825387902054));
#50115=CARTESIAN_POINT('Ctrl Pts',(17.9352358661502,1.91475340062454,39.2528182950881));
#50116=CARTESIAN_POINT('Ctrl Pts',(17.9750180791399,1.91898006709764,39.3213566813332));
#50117=CARTESIAN_POINT('Ctrl Pts',(18.018174287773,1.92320673357075,39.3877722187002));
#50118=CARTESIAN_POINT('Ctrl Pts',(18.0613032552779,1.92743073208096,39.4541458331499));
#50119=CARTESIAN_POINT('Ctrl Pts',(18.1078017363803,1.93165473059118,39.5183988664016));
#50120=CARTESIAN_POINT('Ctrl Pts',(18.1574283184202,1.93587872910139,39.580175678472));
#50121=CARTESIAN_POINT('Ctrl Pts',(18.2070390266422,1.94010137650138,39.6419327302885));
#50122=CARTESIAN_POINT('Ctrl Pts',(18.2597755554984,1.94432402390136,39.7012147685995));
#50123=CARTESIAN_POINT('Ctrl Pts',(18.3153550678058,1.94854667130134,39.7576977689955));
#50124=CARTESIAN_POINT('Ctrl Pts',(18.3709341067662,1.95276928273883,39.8141802883497));
#50125=CARTESIAN_POINT('Ctrl Pts',(18.4293557512288,1.95699189417632,39.8678634840564));
#50126=CARTESIAN_POINT('Ctrl Pts',(18.49030007955,1.9612145056138,39.9184599503682));
#50127=CARTESIAN_POINT('Ctrl Pts',(18.5513050090197,1.96544131588506,39.9691067282359));
#50128=CARTESIAN_POINT('Ctrl Pts',(18.6148372715323,1.96966812615631,40.0166603455416));
#50129=CARTESIAN_POINT('Ctrl Pts',(18.6805440751784,1.97389493642756,40.0608739131707));
#50130=CARTESIAN_POINT('Ctrl Pts',(18.7462827192386,1.97812379494011,40.1051089059524));
#50131=CARTESIAN_POINT('Ctrl Pts',(18.814197601508,1.98235265345266,40.146000382642));
#50132=CARTESIAN_POINT('Ctrl Pts',(18.8839093634339,1.98658151196521,40.1833463782745));
#50133=CARTESIAN_POINT('Ctrl Pts',(18.9537464115799,1.99081797059693,40.2207594922598));
#50134=CARTESIAN_POINT('Ctrl Pts',(19.0253863671182,1.99505442922866,40.2546141926485));
#50135=CARTESIAN_POINT('Ctrl Pts',(19.0984280504848,1.99929088786038,40.2847559270425));
#50136=CARTESIAN_POINT('Ctrl Pts',(19.164812672012,2.00314123316898,40.3121505260946));
#50137=CARTESIAN_POINT('Ctrl Pts',(19.2323546680652,2.00699157847758,40.336478654606));
#50138=CARTESIAN_POINT('Ctrl Pts',(19.3007434046261,2.01084192378618,40.3576604383136));
#50139=CARTESIAN_POINT('Ctrl Pts',(19.3760112099709,2.01507956664628,40.3809728498762));
#50140=CARTESIAN_POINT('Ctrl Pts',(19.4525873877916,2.01931720950637,40.400560891116));
#50141=CARTESIAN_POINT('Ctrl Pts',(19.5300692163137,2.02355485236646,40.4162805312492));
#50142=CARTESIAN_POINT('Ctrl Pts',(19.607439623386,2.02778640135498,40.4319775660164));
#50143=CARTESIAN_POINT('Ctrl Pts',(19.6857126391836,2.03201795034351,40.4438171546242));
#50144=CARTESIAN_POINT('Ctrl Pts',(19.764470124179,2.03624949933204,40.4517049386553));
#50145=CARTESIAN_POINT('Ctrl Pts',(19.8431366427601,2.04047616079987,40.4595836121437));
#50146=CARTESIAN_POINT('Ctrl Pts',(19.9222860544513,2.0447028222677,40.4635195052084));
#50147=CARTESIAN_POINT('Ctrl Pts',(20.0014912653639,2.04892948373553,40.4634695295323));
#50148=CARTESIAN_POINT('Ctrl Pts',(20.0806464798769,2.05315347722415,40.4634195854022));
#50149=CARTESIAN_POINT('Ctrl Pts',(20.159856956153,2.05737747071278,40.4593887667777));
#50150=CARTESIAN_POINT('Ctrl Pts',(20.2386929506919,2.0616014642014,40.4513859989781));
#50151=CARTESIAN_POINT('Ctrl Pts',(20.317503728136,2.0658241065706,40.443385791006));
#50152=CARTESIAN_POINT('Ctrl Pts',(20.3959397956713,2.07004674893979,40.4314162041263));
#50153=CARTESIAN_POINT('Ctrl Pts',(20.4735753821855,2.07426939130899,40.4155381228319));
#50154=CARTESIAN_POINT('Ctrl Pts',(20.5512103074713,2.0784919977136,40.3996601767723));
#50155=CARTESIAN_POINT('Ctrl Pts',(20.6280443063126,2.08271460411822,40.3798738978164));
#50156=CARTESIAN_POINT('Ctrl Pts',(20.7036621393815,2.08693721052283,40.3562912122554));
#50157=CARTESIAN_POINT('Ctrl Pts',(20.7793551651435,2.09116401579344,40.3326850765959));
#50158=CARTESIAN_POINT('Ctrl Pts',(20.853829160939,2.09539082106404,40.3052751335167));
#50159=CARTESIAN_POINT('Ctrl Pts',(20.9266849830521,2.09961762633465,40.2742229377609));
#50160=CARTESIAN_POINT('Ctrl Pts',(20.999576110082,2.10384647985623,40.2431556945435));
#50161=CARTESIAN_POINT('Ctrl Pts',(21.0708470793397,2.10807533337781,40.2084428881213));
#50162=CARTESIAN_POINT('Ctrl Pts',(21.1401219713545,2.11230418689939,40.1702928129458));
#50163=CARTESIAN_POINT('Ctrl Pts',(21.2095213658217,2.1165406406152,40.1320741735649));
#50164=CARTESIAN_POINT('Ctrl Pts',(21.2769171154113,2.120777094331,40.0904061692058));
#50165=CARTESIAN_POINT('Ctrl Pts',(21.3419611955674,2.12501354804681,40.0455412076055));
#50166=CARTESIAN_POINT('Ctrl Pts',(21.4010778782623,2.1288639382663,40.0047647419737));
#50167=CARTESIAN_POINT('Ctrl Pts',(21.458252154305,2.13271432848578,39.961348140781));
#50168=CARTESIAN_POINT('Ctrl Pts',(21.5132479222866,2.13656471870527,39.9155085146028));
#50169=CARTESIAN_POINT('Ctrl Pts',(21.5737748531757,2.14080235936861,39.8650585984093));
#50170=CARTESIAN_POINT('Ctrl Pts',(21.6318897287454,2.14504000003196,39.8114838263428));
#50171=CARTESIAN_POINT('Ctrl Pts',(21.6872525104689,2.1492776406953,39.755043626862));
#50172=CARTESIAN_POINT('Ctrl Pts',(21.7425356779164,2.15350918743267,39.6986845910344));
#50173=CARTESIAN_POINT('Ctrl Pts',(21.7950742854727,2.15774073417004,39.6394686428468));
#50174=CARTESIAN_POINT('Ctrl Pts',(21.8445615706559,2.16197228090742,39.5776951826948));
#50175=CARTESIAN_POINT('Ctrl Pts',(21.8939916962034,2.16619894005258,39.5159930731628));
#50176=CARTESIAN_POINT('Ctrl Pts',(21.940377211622,2.17042559919773,39.4517396860489));
#50177=CARTESIAN_POINT('Ctrl Pts',(21.9834494890326,2.17465225834289,39.3852698414561));
#50178=CARTESIAN_POINT('Ctrl Pts',(22.0264945776475,2.17887624946633,39.3188419550583));
#50179=CARTESIAN_POINT('Ctrl Pts',(22.0662303252704,2.18310024058977,39.2502007806291));
#50180=CARTESIAN_POINT('Ctrl Pts',(22.1024302942585,2.18732423171321,39.1797116738668));
#50181=CARTESIAN_POINT('Ctrl Pts',(22.1386186837,2.19154687167797,39.1092451149662));
#50182=CARTESIAN_POINT('Ctrl Pts',(22.171273326482,2.19576951164274,39.0369322142614));
#50183=CARTESIAN_POINT('Ctrl Pts',(22.2002135341123,2.19999215160751,38.9631632784179));
#50184=CARTESIAN_POINT('Ctrl Pts',(22.2291534950096,2.20421475557169,38.8893949714997));
#50185=CARTESIAN_POINT('Ctrl Pts',(22.2543789138503,2.20843735953587,38.8141710910394));
#50186=CARTESIAN_POINT('Ctrl Pts',(22.2757576522585,2.21265996350005,38.7379008928407));
#50187=CARTESIAN_POINT('Ctrl Pts',(22.2971576490197,2.21688676629038,38.6615548539273));
#50188=CARTESIAN_POINT('Ctrl Pts',(22.3147031980385,2.22111356908071,38.5841608714462));
#50189=CARTESIAN_POINT('Ctrl Pts',(22.3283125540416,2.22534037187103,38.5061417136818));
#50190=CARTESIAN_POINT('Ctrl Pts',(22.34192850487,2.22956922288656,38.4280847493735));
#50191=CARTESIAN_POINT('Ctrl Pts',(22.3516044056267,2.23379807390209,38.349402472139));
#50192=CARTESIAN_POINT('Ctrl Pts',(22.3573103612433,2.23802692491762,38.2705236103154));
#50193=CARTESIAN_POINT('Ctrl Pts',(22.3630265717229,2.24226337611281,38.1915029857483));
#50194=CARTESIAN_POINT('Ctrl Pts',(22.3647585706317,2.24649982730801,38.1122855404265));
#50195=CARTESIAN_POINT('Ctrl Pts',(22.3625286523006,2.2507362785032,38.0333006150055));
#50196=CARTESIAN_POINT('Ctrl Pts',(22.3605019315261,2.25458669021025,37.9615130580364));
#50197=CARTESIAN_POINT('Ctrl Pts',(22.3552031283345,2.2584371019173,37.8899178042344));
#50198=CARTESIAN_POINT('Ctrl Pts',(22.3466858523132,2.26228751362435,37.8188310979975));
#50199=CARTESIAN_POINT('Ctrl Pts',(22.3373120035765,2.26652515683622,37.740595282958));
#50200=CARTESIAN_POINT('Ctrl Pts',(22.324003842043,2.27076280004809,37.6626818952908));
#50201=CARTESIAN_POINT('Ctrl Pts',(22.3067938993386,2.27500044325996,37.5855173988616));
#50202=CARTESIAN_POINT('Ctrl Pts',(22.2896087051605,2.27923199258609,37.5084638677971));
#50203=CARTESIAN_POINT('Ctrl Pts',(22.2685329737471,2.28346354191222,37.4321575430333));
#50204=CARTESIAN_POINT('Ctrl Pts',(22.2436508812131,2.28769509123835,37.3570187323144));
#50205=CARTESIAN_POINT('Ctrl Pts',(22.2187975281099,2.29192175302061,37.2819667087757));
#50206=CARTESIAN_POINT('Ctrl Pts',(22.1901466973382,2.29614841480287,37.2080799622139));
#50207=CARTESIAN_POINT('Ctrl Pts',(22.1578330354633,2.30037507658513,37.1357660906381));
#50208=CARTESIAN_POINT('Ctrl Pts',(22.1255397709241,2.30459907037389,37.0634978657096));
#50209=CARTESIAN_POINT('Ctrl Pts',(22.0895884552659,2.30882306416266,36.9928009719466));
#50210=CARTESIAN_POINT('Ctrl Pts',(22.0501623160007,2.31304705795142,36.9240642368945));
#50211=CARTESIAN_POINT('Ctrl Pts',(22.0107487880241,2.31726970060601,36.8553494887479));
#50212=CARTESIAN_POINT('Ctrl Pts',(21.9678628767205,2.32149234326059,36.7885940605554));
#50213=CARTESIAN_POINT('Ctrl Pts',(21.9217336430263,2.32571498591517,36.7241619840399));
#50214=CARTESIAN_POINT('Ctrl Pts',(21.8756048023846,2.32993759258995,36.6597304565298));
#50215=CARTESIAN_POINT('Ctrl Pts',(21.8262329683468,2.33416019926473,36.5976226216611));
#50216=CARTESIAN_POINT('Ctrl Pts',(21.7738895251984,2.33838280593951,36.5381720986961));
#50217=CARTESIAN_POINT('Ctrl Pts',(21.7214940332192,2.34260961145423,36.4786624598224));
#50218=CARTESIAN_POINT('Ctrl Pts',(21.6661213402309,2.34683641696896,36.4218157636223));
#50219=CARTESIAN_POINT('Ctrl Pts',(21.6080815964379,2.35106322248368,36.3679307115194));
#50220=CARTESIAN_POINT('Ctrl Pts',(21.5500137275854,2.35529207623551,36.314019547649));
#50221=CARTESIAN_POINT('Ctrl Pts',(21.4892765929159,2.35952092998734,36.2630731885298));
#50222=CARTESIAN_POINT('Ctrl Pts',(21.4262135662216,2.36374978373917,36.2153500843856));
#50223=CARTESIAN_POINT('Ctrl Pts',(21.3630372015836,2.36798623765886,36.1675412114672));
#50224=CARTESIAN_POINT('Ctrl Pts',(21.297526981097,2.37222269157856,36.1229674326072));
#50225=CARTESIAN_POINT('Ctrl Pts',(21.2300552007382,2.37645914549825,36.0818437513322));
#50226=CARTESIAN_POINT('Ctrl Pts',(21.1687320949326,2.38030953317998,36.0444676535839));
#50227=CARTESIAN_POINT('Ctrl Pts',(21.1057892168215,2.3841599208617,36.0099410418537));
#50228=CARTESIAN_POINT('Ctrl Pts',(21.0415210293745,2.38801030854343,35.9783910854565));
#50229=CARTESIAN_POINT('Ctrl Pts',(20.970789036555,2.39224795090858,35.9436679762793));
#50230=CARTESIAN_POINT('Ctrl Pts',(20.8981859316676,2.39648559327372,35.9124207415185));
#50231=CARTESIAN_POINT('Ctrl Pts',(20.8240871693434,2.40072323563887,35.8848542309312));
#50232=CARTESIAN_POINT('Ctrl Pts',(20.7500949639096,2.40495478411016,35.8573273620538));
#50233=CARTESIAN_POINT('Ctrl Pts',(20.6746118080797,2.40918633258145,35.8334708679945));
#50234=CARTESIAN_POINT('Ctrl Pts',(20.5980361042617,2.41341788105274,35.8134429246355));
#50235=CARTESIAN_POINT('Ctrl Pts',(20.5215488474356,2.41764454197204,35.7934381140883));
#50236=CARTESIAN_POINT('Ctrl Pts',(20.4439720016012,2.42187120289134,35.7772531844735));
#50237=CARTESIAN_POINT('Ctrl Pts',(20.3657207802558,2.42609786381065,35.7649970552933));
#50238=CARTESIAN_POINT('Ctrl Pts',(20.2875189534818,2.43032185673192,35.7527486625578));
#50239=CARTESIAN_POINT('Ctrl Pts',(20.2086440580531,2.43454584965319,35.7444242201197));
#50240=CARTESIAN_POINT('Ctrl Pts',(20.1295220058824,2.43876984257446,35.7400816770718));
#50241=CARTESIAN_POINT('Ctrl Pts',(20.0504252626488,2.44299248435824,35.7357405230824));
#50242=CARTESIAN_POINT('Ctrl Pts',(19.9710819873992,2.44721512614202,35.7353787648406));
#50243=CARTESIAN_POINT('Ctrl Pts',(19.8919222404062,2.4514377679258,35.7390024060196));
#50244=CARTESIAN_POINT('Ctrl Pts',(19.8127631679478,2.45566037372769,35.7426260163209));
#50245=CARTESIAN_POINT('Ctrl Pts',(19.7337880888534,2.45988297952957,35.7502349356552));
#50246=CARTESIAN_POINT('Ctrl Pts',(19.6554245894791,2.46410558533146,35.7617831094263));
#50247=CARTESIAN_POINT('Ctrl Pts',(19.5769831676012,2.46833238997615,35.773342766383));
#50248=CARTESIAN_POINT('Ctrl Pts',(19.4991550050446,2.47255919462084,35.7888494336711));
#50249=CARTESIAN_POINT('Ctrl Pts',(19.4223594983946,2.47678599926553,35.8082055302002));
#50250=CARTESIAN_POINT('Ctrl Pts',(19.3455267779548,2.4810148521475,35.8275710063628));
#50251=CARTESIAN_POINT('Ctrl Pts',(19.2697281590817,2.48524370502947,35.8507894903244));
#50252=CARTESIAN_POINT('Ctrl Pts',(19.1953673577147,2.48947255791144,35.8777136206445));
#50253=CARTESIAN_POINT('Ctrl Pts',(19.1208729136391,2.49370901097178,35.9046861395462));
#50254=CARTESIAN_POINT('Ctrl Pts',(19.0478218835058,2.49794546403211,35.9353774298504));
#50255=CARTESIAN_POINT('Ctrl Pts',(18.9765972806018,2.50218191709245,35.9695922186519));
#50256=CARTESIAN_POINT('Ctrl Pts',(18.911863201522,2.50603231254914,36.0006890974505));
#50257=CARTESIAN_POINT('Ctrl Pts',(18.8486377701117,2.50988270800582,36.03469583917));
#50258=CARTESIAN_POINT('Ctrl Pts',(18.7871879528988,2.51373310346251,36.0714346499789));
#50259=CARTESIAN_POINT('Ctrl Pts',(18.7195579291215,2.51797074562482,36.1118684016359));
#50260=CARTESIAN_POINT('Ctrl Pts',(18.6538251905401,2.52220838778714,36.155763810211));
#50261=CARTESIAN_POINT('Ctrl Pts',(18.590365952264,2.52644602994945,36.2029174260556));
#50262=CARTESIAN_POINT('Ctrl Pts',(18.5269979709271,2.53067757821175,36.2500032331026));
#50263=CARTESIAN_POINT('Ctrl Pts',(18.4658973703607,2.53490912647406,36.3003376653042));
#50264=CARTESIAN_POINT('Ctrl Pts',(18.4074137037711,2.53914067473636,36.353672616614));
#50265=CARTESIAN_POINT('Ctrl Pts',(18.3489975875033,2.54336733543837,36.4069459645166));
#50266=CARTESIAN_POINT('Ctrl Pts',(18.2931927430933,2.54759399614038,36.4632126300605));
#50267=CARTESIAN_POINT('Ctrl Pts',(18.2403165550457,2.55182065684239,36.5221835929191));
#50268=CARTESIAN_POINT('Ctrl Pts',(18.187473744134,2.5560446495414,36.5811173314256));
#50269=CARTESIAN_POINT('Ctrl Pts',(18.1375562323235,2.56026864224041,36.6427516308589));
#50270=CARTESIAN_POINT('Ctrl Pts',(18.0908444702271,2.56449263493942,36.7067607513289));
#50271=CARTESIAN_POINT('Ctrl Pts',(18.0441476499725,2.56871527649628,36.7707493969954));
#50272=CARTESIAN_POINT('Ctrl Pts',(18.0006548192613,2.57293791805314,36.8371109768091));
#50273=CARTESIAN_POINT('Ctrl Pts',(17.9606051114807,2.57716055961,36.9054879952125));
#50274=CARTESIAN_POINT('Ctrl Pts',(17.9205557450123,2.58138316518061,36.9738644308923));
#50275=CARTESIAN_POINT('Ctrl Pts',(17.8839496788187,2.58560577075122,37.0442558657929));
#50276=CARTESIAN_POINT('Ctrl Pts',(17.8509810296547,2.58982837632183,37.1162785424746));
#50277=CARTESIAN_POINT('Ctrl Pts',(17.8179795974141,2.59405518072996,37.1883728364345));
#50278=CARTESIAN_POINT('Ctrl Pts',(17.7886230026289,2.5982819851381,37.2621011850176));
#50279=CARTESIAN_POINT('Ctrl Pts',(17.7630576801667,2.60250878954623,37.3370586532119));
#50280=CARTESIAN_POINT('Ctrl Pts',(17.7374799692052,2.60673764218838,37.4120524444582));
#50281=CARTESIAN_POINT('Ctrl Pts',(17.7156973194211,2.61096649483052,37.4882760905327));
#50282=CARTESIAN_POINT('Ctrl Pts',(17.6978058710282,2.61519534747267,37.5653107131916));
#50283=CARTESIAN_POINT('Ctrl Pts',(17.6798822677788,2.61943180029042,37.6424837839614));
#50284=CARTESIAN_POINT('Ctrl Pts',(17.665863922428,2.62366825310818,37.720470281074));
#50285=CARTESIAN_POINT('Ctrl Pts',(17.655795514626,2.62790470592593,37.7988426131532));
#50286=CARTESIAN_POINT('Ctrl Pts',(17.6466446108514,2.63175510341115,37.8700731079398));
#50287=CARTESIAN_POINT('Ctrl Pts',(17.6407559108034,2.63560550089637,37.941621989365));
#50288=CARTESIAN_POINT('Ctrl Pts',(17.6381255883642,2.63945589838159,38.0131685278254));
#50289=CARTESIAN_POINT('Ctrl Pts',(17.6370685010235,2.6410033156783,38.0419220140714));
#50290=CARTESIAN_POINT('Ctrl Pts',(17.6365364592934,2.64255073297501,38.0706949209532));
#50291=CARTESIAN_POINT('Ctrl Pts',(17.6365300584561,2.64409815027172,38.0994743401003));
#50292=CARTESIAN_POINT('',(17.6365305931584,3.43784812059947,38.0983255377209));
#50293=CARTESIAN_POINT('Ctrl Pts',(17.6365300584559,2.64409815030312,38.0994743406844));
#50294=CARTESIAN_POINT('Ctrl Pts',(17.6365126342479,2.64831049778694,38.1778170825479));
#50295=CARTESIAN_POINT('Ctrl Pts',(17.640394763803,2.65252284527075,38.2563144725919));
#50296=CARTESIAN_POINT('Ctrl Pts',(17.6481964798018,2.65673519275457,38.3345434784501));
#50297=CARTESIAN_POINT('Ctrl Pts',(17.6559871178273,2.66094155895511,38.4126614037658));
#50298=CARTESIAN_POINT('Ctrl Pts',(17.6676862462287,2.66514792515566,38.4905112328437));
#50299=CARTESIAN_POINT('Ctrl Pts',(17.6832618833385,2.66935429135621,38.5676696908159));
#50300=CARTESIAN_POINT('Ctrl Pts',(17.698820203847,2.67355598102465,38.6447423659561));
#50301=CARTESIAN_POINT('Ctrl Pts',(17.7182463777624,2.67775767069309,38.7211247337187));
#50302=CARTESIAN_POINT('Ctrl Pts',(17.7414567754773,2.68195936036154,38.7963999884138));
#50303=CARTESIAN_POINT('Ctrl Pts',(17.7646533659365,2.68615855055519,38.8716304638376));
#50304=CARTESIAN_POINT('Ctrl Pts',(17.7916295736728,2.69035774074883,38.9457546802339));
#50305=CARTESIAN_POINT('Ctrl Pts',(17.8222512861565,2.69455693094248,39.0183686516063));
#50306=CARTESIAN_POINT('Ctrl Pts',(17.8528646098222,2.698754970768,39.0909627303815));
#50307=CARTESIAN_POINT('Ctrl Pts',(17.8871212708334,2.70295301059351,39.1620469482083));
#50308=CARTESIAN_POINT('Ctrl Pts',(17.9248387147748,2.70715105041902,39.2312365275231));
#50309=CARTESIAN_POINT('Ctrl Pts',(17.9625579303584,2.71134928743246,39.3004293567713));
#50310=CARTESIAN_POINT('Ctrl Pts',(18.0037380224241,2.7155475244459,39.3677269548083));
#50311=CARTESIAN_POINT('Ctrl Pts',(18.0481508620189,2.71974576145934,39.4327698163834));
#50312=CARTESIAN_POINT('Ctrl Pts',(18.0926089584444,2.7239482764902,39.4978789568498));
#50313=CARTESIAN_POINT('Ctrl Pts',(18.1403061098576,2.72815079152106,39.5607283814506));
#50314=CARTESIAN_POINT('Ctrl Pts',(18.1909717149057,2.73235330655192,39.6209888574966));
#50315=CARTESIAN_POINT('Ctrl Pts',(18.2416652800875,2.7365581407672,39.6812825886664));
#50316=CARTESIAN_POINT('Ctrl Pts',(18.2953302355493,2.74076297498247,39.7389841801321));
#50317=CARTESIAN_POINT('Ctrl Pts',(18.3516584349362,2.74496780919775,39.793800615711));
#50318=CARTESIAN_POINT('Ctrl Pts',(18.4080820901582,2.74917976907949,39.8487099452346));
#50319=CARTESIAN_POINT('Ctrl Pts',(18.4671776426322,2.75339172896124,39.9007240446893));
#50320=CARTESIAN_POINT('Ctrl Pts',(18.5286035805689,2.75760368884298,39.9495899593654));
#50321=CARTESIAN_POINT('Ctrl Pts',(18.5654274319154,2.76012869032888,39.9788842809239));
#50322=CARTESIAN_POINT('Ctrl Pts',(18.6030881936985,2.76265369181477,40.0070480259098));
#50323=CARTESIAN_POINT('Ctrl Pts',(18.6415077282651,2.76517869330067,40.0340344331311));
#50324=CARTESIAN_POINT('Ctrl Pts',(18.7059862041131,2.76941633566571,40.0793249975762));
#50325=CARTESIAN_POINT('Ctrl Pts',(18.7728530917134,2.77365397803075,40.1214725932932));
#50326=CARTESIAN_POINT('Ctrl Pts',(18.8417693212833,2.77789162039579,40.160216526431));
#50327=CARTESIAN_POINT('Ctrl Pts',(18.9105864466124,2.78212316886492,40.1989047442735));
#50328=CARTESIAN_POINT('Ctrl Pts',(18.9814466561246,2.78635471733404,40.2341987919326));
#50329=CARTESIAN_POINT('Ctrl Pts',(19.0539809595455,2.79058626580317,40.2658805174796));
#50330=CARTESIAN_POINT('Ctrl Pts',(19.1264314838471,2.79481292671721,40.2975256497605));
#50331=CARTESIAN_POINT('Ctrl Pts',(19.2005518320499,2.79903958763125,40.3255665647168));
#50332=CARTESIAN_POINT('Ctrl Pts',(19.2759487543359,2.80326624854529,40.3498311568987));
#50333=CARTESIAN_POINT('Ctrl Pts',(19.3512980837379,2.8074902414594,40.3740804325149));
#50334=CARTESIAN_POINT('Ctrl Pts',(19.427921942706,2.81171423437352,40.394557973569));
#50335=CARTESIAN_POINT('Ctrl Pts',(19.5054085940351,2.81593822728763,40.4111403639861));
#50336=CARTESIAN_POINT('Ctrl Pts',(19.5828704595116,2.82016086906237,40.4277174501517));
#50337=CARTESIAN_POINT('Ctrl Pts',(19.6611941112365,2.82438351083711,40.4404017618673));
#50338=CARTESIAN_POINT('Ctrl Pts',(19.739955643659,2.82860615261186,40.4491205532359));
#50339=CARTESIAN_POINT('Ctrl Pts',(19.818716504905,2.83282875840281,40.4578392703061));
#50340=CARTESIAN_POINT('Ctrl Pts',(19.8979147733456,2.83705136419377,40.4625924840629));
#50341=CARTESIAN_POINT('Ctrl Pts',(19.9771208994181,2.84127396998473,40.4633592591175));
#50342=CARTESIAN_POINT('Ctrl Pts',(20.0564057858247,2.84550077461559,40.4641267966317));
#50343=CARTESIAN_POINT('Ctrl Pts',(20.1356980756293,2.84972757924645,40.4608999727833));
#50344=CARTESIAN_POINT('Ctrl Pts',(20.2145683043251,2.8539543838773,40.4537100254023));
#50345=CARTESIAN_POINT('Ctrl Pts',(20.2934767521556,2.85818323674383,40.4465165938983));
#50346=CARTESIAN_POINT('Ctrl Pts',(20.3719622667441,2.86241208961035,40.435356279158));
#50347=CARTESIAN_POINT('Ctrl Pts',(20.4496031398418,2.86664094247688,40.420311931087));
#50348=CARTESIAN_POINT('Ctrl Pts',(20.5273835506115,2.87087739551919,40.4052405450239));
#50349=CARTESIAN_POINT('Ctrl Pts',(20.6043158305455,2.87511384856151,40.3862712904857));
#50350=CARTESIAN_POINT('Ctrl Pts',(20.6799912790346,2.87935030160383,40.3635375634915));
#50351=CARTESIAN_POINT('Ctrl Pts',(20.7487706107861,2.88320069714247,40.3428755048965));
#50352=CARTESIAN_POINT('Ctrl Pts',(20.8165116962031,2.88705109268111,40.3191045291742));
#50353=CARTESIAN_POINT('Ctrl Pts',(20.882923187911,2.89090148821975,40.2923587948028));
#50354=CARTESIAN_POINT('Ctrl Pts',(20.956013899517,2.89513913057119,40.2629231548652));
#50355=CARTESIAN_POINT('Ctrl Pts',(21.0277681739357,2.89937677292263,40.2297731241964));
#50356=CARTESIAN_POINT('Ctrl Pts',(21.0977827558158,2.90361441527406,40.1930512325152));
#50357=CARTESIAN_POINT('Ctrl Pts',(21.1676966539706,2.90784596372896,40.1563821483601));
#50358=CARTESIAN_POINT('Ctrl Pts',(21.235875416115,2.91207751218385,40.1161516196961));
#50359=CARTESIAN_POINT('Ctrl Pts',(21.30193518715,2.91630906063874,40.0725504326533));
#50360=CARTESIAN_POINT('Ctrl Pts',(21.3679186573145,2.92053572153763,40.0289996061926));
#50361=CARTESIAN_POINT('Ctrl Pts',(21.4317876108973,2.92476238243652,39.9820861150492));
#50362=CARTESIAN_POINT('Ctrl Pts',(21.4931836143664,2.92898904333542,39.9320461606324));
#50363=CARTESIAN_POINT('Ctrl Pts',(21.554540862759,2.93321303623384,39.8820377929988));
#50364=CARTESIAN_POINT('Ctrl Pts',(21.6134278970377,2.93743702913226,39.8289071746988));
#50365=CARTESIAN_POINT('Ctrl Pts',(21.6695170642665,2.94166102203068,39.7729325189687));
#50366=CARTESIAN_POINT('Ctrl Pts',(21.7255882901034,2.9458836637892,39.7169757680014));
#50367=CARTESIAN_POINT('Ctrl Pts',(21.7788630945344,2.95010630554772,39.658177117043));
#50368=CARTESIAN_POINT('Ctrl Pts',(21.8290497065301,2.95432894730624,39.5968525685391));
#50369=CARTESIAN_POINT('Ctrl Pts',(21.8792358908482,2.95855155308047,39.5355285426276));
#50370=CARTESIAN_POINT('Ctrl Pts',(21.926333639276,2.96277415885471,39.4716790256496));
#50371=CARTESIAN_POINT('Ctrl Pts',(21.9700915707039,2.96699676462894,39.4056529569305));
#50372=CARTESIAN_POINT('Ctrl Pts',(22.0138930137757,2.97122356924239,39.3395612337644));
#50373=CARTESIAN_POINT('Ctrl Pts',(22.0543477465301,2.97545037385585,39.2712890273145));
#50374=CARTESIAN_POINT('Ctrl Pts',(22.0912482005776,2.9796771784693,39.2012136052923));
#50375=CARTESIAN_POINT('Ctrl Pts',(22.128166535937,2.98390603131803,39.1311042259516));
#50376=CARTESIAN_POINT('Ctrl Pts',(22.1615269639637,2.98813488416676,39.0591903161031));
#50377=CARTESIAN_POINT('Ctrl Pts',(22.1911694339725,2.99236373701548,38.9858707312722));
#50378=CARTESIAN_POINT('Ctrl Pts',(22.220865177996,2.99660019003953,38.9124193750795));
#50379=CARTESIAN_POINT('Ctrl Pts',(22.2468294587741,3.00083664306357,38.8375577400424));
#50380=CARTESIAN_POINT('Ctrl Pts',(22.268951707638,3.00507309608762,38.7617012840448));
#50381=CARTESIAN_POINT('Ctrl Pts',(22.289058011439,3.00892349177136,38.6927574366568));
#50382=CARTESIAN_POINT('Ctrl Pts',(22.3059911908141,3.01277388745509,38.6229922463347));
#50383=CARTESIAN_POINT('Ctrl Pts',(22.3197051962276,3.01662428313883,38.5527231422126));
#50384=CARTESIAN_POINT('Ctrl Pts',(22.3347984633941,3.02086192553427,38.4753868476661));
#50385=CARTESIAN_POINT('Ctrl Pts',(22.3460483782244,3.02509956792971,38.3971497721236));
#50386=CARTESIAN_POINT('Ctrl Pts',(22.3533549980713,3.02933721032515,38.3184277774291));
#50387=CARTESIAN_POINT('Ctrl Pts',(22.3606511107127,3.03356875882481,38.2398189880471));
#50388=CARTESIAN_POINT('Ctrl Pts',(22.3640151467171,3.03780030732446,38.160727127262));
#50389=CARTESIAN_POINT('Ctrl Pts',(22.3633982044233,3.04203185582412,38.0815780503533));
#50390=CARTESIAN_POINT('Ctrl Pts',(22.3627819747148,3.04625851676872,38.0025203928082));
#50391=CARTESIAN_POINT('Ctrl Pts',(22.3581939080036,3.05048517771332,37.9234061168559));
#50392=CARTESIAN_POINT('Ctrl Pts',(22.3496370378967,3.05471183865792,37.8446644735964));
#50393=CARTESIAN_POINT('Ctrl Pts',(22.3410855691526,3.0589358316026,37.7659725345124));
#50394=CARTESIAN_POINT('Ctrl Pts',(22.3285703201331,3.06315982454729,37.6876532260512));
#50395=CARTESIAN_POINT('Ctrl Pts',(22.3121463217775,3.06738381749197,37.6101328469975));
#50396=CARTESIAN_POINT('Ctrl Pts',(22.2957275770082,3.07160645929725,37.5326372645854));
#50397=CARTESIAN_POINT('Ctrl Pts',(22.2754026628456,3.07582910110253,37.455940562361));
#50398=CARTESIAN_POINT('Ctrl Pts',(22.2512778421683,3.0800517429078,37.3804595089489));
#50399=CARTESIAN_POINT('Ctrl Pts',(22.2271532270742,3.08427434872922,37.3049790987599));
#50400=CARTESIAN_POINT('Ctrl Pts',(22.1992289139255,3.08849695455063,37.2307147628709));
#50401=CARTESIAN_POINT('Ctrl Pts',(22.1676607809497,3.09271956037204,37.1580673168254));
#50402=CARTESIAN_POINT('Ctrl Pts',(22.1360612575172,3.09694636503301,37.0853476322185));
#50403=CARTESIAN_POINT('Ctrl Pts',(22.1008108639355,3.10117316969397,37.0142484799576));
#50404=CARTESIAN_POINT('Ctrl Pts',(22.0621130910175,3.10539997435494,36.9451493426618));
#50405=CARTESIAN_POINT('Ctrl Pts',(22.0233965658362,3.10962882725143,36.876016721134));
#50406=CARTESIAN_POINT('Ctrl Pts',(21.9812295830714,3.11385768014793,36.8088864427421));
#50407=CARTESIAN_POINT('Ctrl Pts',(21.9358596084275,3.11808653304443,36.744109880057));
#50408=CARTESIAN_POINT('Ctrl Pts',(21.8904080939984,3.12232298611613,36.6792168996961));
#50409=CARTESIAN_POINT('Ctrl Pts',(21.8417423742846,3.12655943918783,36.6166864580939));
#50410=CARTESIAN_POINT('Ctrl Pts',(21.7901507769903,3.13079589225953,36.556837456215));
#50411=CARTESIAN_POINT('Ctrl Pts',(21.7432605981942,3.13464628752565,36.5024423503053));
#50412=CARTESIAN_POINT('Ctrl Pts',(21.6939541776096,3.13849668279178,36.4502619890175));
#50413=CARTESIAN_POINT('Ctrl Pts',(21.642472729767,3.14234707805791,36.4005077896996));
#50414=CARTESIAN_POINT('Ctrl Pts',(21.5858136208204,3.14658472043226,36.3457496444291));
#50415=CARTESIAN_POINT('Ctrl Pts',(21.5263068026791,3.1508223628066,36.2937252357204));
#50416=CARTESIAN_POINT('Ctrl Pts',(21.4642467260256,3.15506000518095,36.244744770598));
#50417=CARTESIAN_POINT('Ctrl Pts',(21.402275894198,3.15929155365925,36.1958347413069));
#50418=CARTESIAN_POINT('Ctrl Pts',(21.3377594604198,3.16352310213755,36.1499602506902));
#50419=CARTESIAN_POINT('Ctrl Pts',(21.2710280419653,3.16775465061585,36.1073941289262));
#50420=CARTESIAN_POINT('Ctrl Pts',(21.2043737001417,3.17198131153881,36.0648771722082));
#50421=CARTESIAN_POINT('Ctrl Pts',(21.135509850979,3.17620797246177,36.0256612413644));
#50422=CARTESIAN_POINT('Ctrl Pts',(21.0647982306072,3.18043463338473,35.9899774482258));
#50423=CARTESIAN_POINT('Ctrl Pts',(20.9941312456137,3.18465862630761,35.9543161798094));
#50424=CARTESIAN_POINT('Ctrl Pts',(20.9216192219379,3.18888261923048,35.9221828342385));
#50425=CARTESIAN_POINT('Ctrl Pts',(20.8476497231039,3.19310661215335,35.8937632974176));
#50426=CARTESIAN_POINT('Ctrl Pts',(20.773703885085,3.19732925393668,35.8653528512274));
#50427=CARTESIAN_POINT('Ctrl Pts',(20.6983019349738,3.20155189572001,35.8406540227646));
#50428=CARTESIAN_POINT('Ctrl Pts',(20.6218513291174,3.20577453750334,35.8198045335158));
#50429=CARTESIAN_POINT('Ctrl Pts',(20.545401374748,3.2099971433027,35.7989552219395));
#50430=CARTESIAN_POINT('Ctrl Pts',(20.4679032350335,3.21421974910206,35.7819553063147));
#50431=CARTESIAN_POINT('Ctrl Pts',(20.3897779911959,3.21844235490142,35.7688922035909));
#50432=CARTESIAN_POINT('Ctrl Pts',(20.3115750618297,3.22266915954033,35.7558161112879));
#50433=CARTESIAN_POINT('Ctrl Pts',(20.2327442461769,3.22689596417925,35.7466847289162));
#50434=CARTESIAN_POINT('Ctrl Pts',(20.1537146471826,3.23112276881816,35.7415339205022));
#50435=CARTESIAN_POINT('Ctrl Pts',(20.0746467518291,3.23535162169255,35.7363806160967));
#50436=CARTESIAN_POINT('Ctrl Pts',(19.9953803505619,3.23958047456695,35.7352117351967));
#50437=CARTESIAN_POINT('Ctrl Pts',(19.9163449028138,3.24380932744135,35.7380109514194));
#50438=CARTESIAN_POINT('Ctrl Pts',(19.8371674110449,3.24804578049114,35.7408151984471));
#50439=CARTESIAN_POINT('Ctrl Pts',(19.7582221703125,3.25228223354094,35.747601751861));
#50440=CARTESIAN_POINT('Ctrl Pts',(19.6799336433097,3.25651868659074,35.7583023320217));
#50441=CARTESIAN_POINT('Ctrl Pts',(19.6087793579768,3.26036908205282,35.7680277945273));
#50442=CARTESIAN_POINT('Ctrl Pts',(19.5381677039131,3.26421947751491,35.7809857284757));
#50443=CARTESIAN_POINT('Ctrl Pts',(19.4684073339674,3.26806987297699,35.7970888687749));
#50444=CARTESIAN_POINT('Ctrl Pts',(19.3916309345943,3.27230751535147,35.8148115547604));
#50445=CARTESIAN_POINT('Ctrl Pts',(19.3155976689195,3.27654515772595,35.836411161631));
#50446=CARTESIAN_POINT('Ctrl Pts',(19.2407280395302,3.28078280010044,35.8618095409585));
#50447=CARTESIAN_POINT('Ctrl Pts',(19.1659660756073,3.28501434857882,35.8871713964195));
#50448=CARTESIAN_POINT('Ctrl Pts',(19.0923648651002,3.2892458970572,35.9163210264038));
#50449=CARTESIAN_POINT('Ctrl Pts',(19.020333243132,3.29347744553558,35.9491295979563));
#50450=CARTESIAN_POINT('Ctrl Pts',(18.9483848196777,3.29770410645853,35.981900274702));
#50451=CARTESIAN_POINT('Ctrl Pts',(18.8780028064846,3.30193076738147,36.018321301211));
#50452=CARTESIAN_POINT('Ctrl Pts',(18.8095779816057,3.30615742830442,36.05821503115));
#50453=CARTESIAN_POINT('Ctrl Pts',(18.7411963486092,3.31038142122723,36.0980835789229));
#50454=CARTESIAN_POINT('Ctrl Pts',(18.6747698556288,3.31460541415005,36.1414202435998));
#50455=CARTESIAN_POINT('Ctrl Pts',(18.6106654009218,3.31882940707286,36.1880010950044));
#50456=CARTESIAN_POINT('Ctrl Pts',(18.5465814514735,3.32305204885607,36.234567046471));
#50457=CARTESIAN_POINT('Ctrl Pts',(18.4848184442857,3.32727469063928,36.2843748485822));
#50458=CARTESIAN_POINT('Ctrl Pts',(18.4257137024169,3.33149733242249,36.3371576661136));
#50459=CARTESIAN_POINT('Ctrl Pts',(18.3666094642199,3.33571993822169,36.3899400338466));
#50460=CARTESIAN_POINT('Ctrl Pts',(18.3101637949927,3.33994254402088,36.4456970532807));
#50461=CARTESIAN_POINT('Ctrl Pts',(18.2566792354514,3.34416514982008,36.5041230771787));
#50462=CARTESIAN_POINT('Ctrl Pts',(18.2031414923808,3.34839195445873,36.562607198258));
#50463=CARTESIAN_POINT('Ctrl Pts',(18.1525710577994,3.35261875909739,36.623765278567));
#50464=CARTESIAN_POINT('Ctrl Pts',(18.1052315928562,3.35684556373604,36.687256879617));
#50465=CARTESIAN_POINT('Ctrl Pts',(18.0578691880381,3.36107441661013,36.7507792475839));
#50466=CARTESIAN_POINT('Ctrl Pts',(18.0137411331327,3.36530326948422,36.8166369990124));
#50467=CARTESIAN_POINT('Ctrl Pts',(17.9730675024953,3.36953212235831,36.8844609872738));
#50468=CARTESIAN_POINT('Ctrl Pts',(17.9323207724304,3.37376857540772,36.9524068701051));
#50469=CARTESIAN_POINT('Ctrl Pts',(17.8950410926088,3.37800502845714,37.0223256359311));
#50470=CARTESIAN_POINT('Ctrl Pts',(17.8614022355798,3.38224148150655,37.0938240497224));
#50471=CARTESIAN_POINT('Ctrl Pts',(17.83082880517,3.38609187696972,37.1588069882503));
#50472=CARTESIAN_POINT('Ctrl Pts',(17.8032623637644,3.3899422724329,37.2250942800547));
#50473=CARTESIAN_POINT('Ctrl Pts',(17.7787977182185,3.39379266789607,37.2923795047743));
#50474=CARTESIAN_POINT('Ctrl Pts',(17.747710668165,3.398685337862,37.3778783584077));
#50475=CARTESIAN_POINT('Ctrl Pts',(17.7215354524299,3.40357800782793,37.4652526455507));
#50476=CARTESIAN_POINT('Ctrl Pts',(17.7004693699155,3.40847067779385,37.5539694860147));
#50477=CARTESIAN_POINT('Ctrl Pts',(17.6793879141012,3.41336691826146,37.6427510689668));
#50478=CARTESIAN_POINT('Ctrl Pts',(17.6634232143288,3.41826315872906,37.7328770278252));
#50479=CARTESIAN_POINT('Ctrl Pts',(17.6527251187551,3.42315939919666,37.823791613493));
#50480=CARTESIAN_POINT('Ctrl Pts',(17.6420270231814,3.42805563966427,37.9147061991608));
#50481=CARTESIAN_POINT('Ctrl Pts',(17.6365957136741,3.43295188013187,38.0064092559421));
#50482=CARTESIAN_POINT('Ctrl Pts',(17.6365305931584,3.43784812059947,38.0983255377209));
#50483=CARTESIAN_POINT('',(17.6387453353606,4.23159815027171,38.101781203975));
#50484=CARTESIAN_POINT('Ctrl Pts',(17.6390002039829,3.43784815027172,38.0983278438321));
#50485=CARTESIAN_POINT('Ctrl Pts',(17.6423555560034,3.4650705877862,38.6088386346336));
#50486=CARTESIAN_POINT('Ctrl Pts',(18.0552834653053,3.53420062360702,39.910202051485));
#50487=CARTESIAN_POINT('Ctrl Pts',(20.1976448724621,3.64523825773423,40.8842741316918));
#50488=CARTESIAN_POINT('Ctrl Pts',(22.4432224513611,3.77096105265329,39.4497814596623));
#50489=CARTESIAN_POINT('Ctrl Pts',(22.4622207069824,3.89668384757238,36.7851938828303));
#50490=CARTESIAN_POINT('Ctrl Pts',(20.2373259792565,4.02240664249146,35.3188271691023));
#50491=CARTESIAN_POINT('Ctrl Pts',(18.0696336552147,4.13404474339124,36.2673539383482));
#50492=CARTESIAN_POINT('Ctrl Pts',(17.6424244891864,4.20377524598466,37.5801514847896));
#50493=CARTESIAN_POINT('Ctrl Pts',(17.6387453353606,4.23159815027171,38.101781203975));
#50494=CARTESIAN_POINT('',(17.6327380335352,5.02534815027172,38.1003247073934));
#50495=CARTESIAN_POINT('Ctrl Pts',(17.6387453353606,4.23159815027171,38.101781203975));
#50496=CARTESIAN_POINT('Ctrl Pts',(17.6368828498576,4.24568284429102,38.3658440390514));
#50497=CARTESIAN_POINT('Ctrl Pts',(17.7993870304845,4.30167513661668,39.4133737818963));
#50498=CARTESIAN_POINT('Ctrl Pts',(19.3334665954578,4.3995750272487,40.8105311576044));
#50499=CARTESIAN_POINT('Ctrl Pts',(21.9109589195357,4.52529782216778,40.1345716855284));
#50500=CARTESIAN_POINT('Ctrl Pts',(22.7469390798614,4.65102061708686,37.60444815888));
#50501=CARTESIAN_POINT('Ctrl Pts',(21.0795541642787,4.77674341200594,35.5259353655944));
#50502=CARTESIAN_POINT('Ctrl Pts',(18.4483093765511,4.9015192564009,35.791228794861));
#50503=CARTESIAN_POINT('Ctrl Pts',(17.6342141099641,4.98438750248949,37.3374076479298));
#50504=CARTESIAN_POINT('Ctrl Pts',(17.6327380335352,5.02534815027172,38.1003247073934));
#50505=CARTESIAN_POINT('',(17.6378382696348,5.81909815027172,38.0979654557371));
#50506=CARTESIAN_POINT('Ctrl Pts',(17.6327380335352,5.02534815027172,38.1003247073934));
#50507=CARTESIAN_POINT('Ctrl Pts',(17.6327039087979,5.02629510079585,38.1179622387422));
#50508=CARTESIAN_POINT('Ctrl Pts',(17.6408568301016,5.06914964962618,38.9161219948285));
#50509=CARTESIAN_POINT('Ctrl Pts',(18.5336418898511,5.15391179676333,40.4750873307105));
#50510=CARTESIAN_POINT('Ctrl Pts',(21.1941929599868,5.27963459168218,40.6229247135073));
#50511=CARTESIAN_POINT('Ctrl Pts',(22.7664414274776,5.40535738660137,38.4715477951031));
#50512=CARTESIAN_POINT('Ctrl Pts',(21.8175517653059,5.5310801815204,35.9815686189682));
#50513=CARTESIAN_POINT('Ctrl Pts',(19.2122745821007,5.65680297643949,35.4221772646974));
#50514=CARTESIAN_POINT('Ctrl Pts',(17.7709947773869,5.75280896602327,36.8585589655981));
#50515=CARTESIAN_POINT('Ctrl Pts',(17.6359459392263,5.80690735730068,37.8696316425113));
#50516=CARTESIAN_POINT('Ctrl Pts',(17.6378382696348,5.81909815027172,38.0979654557371));
#50517=CARTESIAN_POINT('',(17.6396768404944,6.61284815027172,38.1012519486375));
#50518=CARTESIAN_POINT('Ctrl Pts',(17.6378382696348,5.81909815027172,38.0979654557371));
#50519=CARTESIAN_POINT('Ctrl Pts',(17.6424510962582,5.84881495560703,38.654561855595));
#50520=CARTESIAN_POINT('Ctrl Pts',(18.1165213946417,5.9204393592487,40.0031607324733));
#50521=CARTESIAN_POINT('Ctrl Pts',(20.3621280800665,6.03397136119673,40.8676902264046));
#50522=CARTESIAN_POINT('Ctrl Pts',(22.5188448048673,6.15969415611581,39.3027746192458));
#50523=CARTESIAN_POINT('Ctrl Pts',(22.3800653672784,6.28541695103489,36.6417356950161));
#50524=CARTESIAN_POINT('Ctrl Pts',(20.0722634848505,6.41113974595397,35.3096552319713));
#50525=CARTESIAN_POINT('Ctrl Pts',(18.0116199776956,6.52028347903291,36.3608230696746));
#50526=CARTESIAN_POINT('Ctrl Pts',(17.641972639838,6.5875196138055,37.6259160691615));
#50527=CARTESIAN_POINT('Ctrl Pts',(17.6396768404944,6.61284815027172,38.1012519486375));
#50528=CARTESIAN_POINT('',(17.6333442921061,7.40659815027172,38.1011170196962));
#50529=CARTESIAN_POINT('Ctrl Pts',(17.6396768404944,6.61284815027172,38.1012519486375));
#50530=CARTESIAN_POINT('Ctrl Pts',(17.6381741007155,6.62942721211186,38.4123880836123));
#50531=CARTESIAN_POINT('Ctrl Pts',(17.8398734532478,6.68791387225836,39.5081257521821));
#50532=CARTESIAN_POINT('Ctrl Pts',(19.4950998583179,6.7883081307112,40.845236197969));
#50533=CARTESIAN_POINT('Ctrl Pts',(22.0280545809553,6.91403092563029,40.0178739667594));
#50534=CARTESIAN_POINT('Ctrl Pts',(22.7127844750115,7.03975372054937,37.4426976891526));
#50535=CARTESIAN_POINT('Ctrl Pts',(20.9252753729429,7.16547651546845,35.4665400287961));
#50536=CARTESIAN_POINT('Ctrl Pts',(18.3665453557022,7.28775799204257,35.8787305372433));
#50537=CARTESIAN_POINT('Ctrl Pts',(17.6375482172936,7.36813187031033,37.3841700502603));
#50538=CARTESIAN_POINT('Ctrl Pts',(17.6333442921061,7.40659815027172,38.1011170196962));
#50539=CARTESIAN_POINT('',(17.6364827852058,8.20034815027172,38.0978694718631));
#50540=CARTESIAN_POINT('Ctrl Pts',(17.6333442921061,7.40659815027172,38.1011170196962));
#50541=CARTESIAN_POINT('Ctrl Pts',(17.6329681953044,7.41003946861669,38.1652574242468));
#50542=CARTESIAN_POINT('Ctrl Pts',(17.6643665387496,7.45538838526801,39.010111409356));
#50543=CARTESIAN_POINT('Ctrl Pts',(18.6768195719384,7.54264490022567,40.5577305569364));
#50544=CARTESIAN_POINT('Ctrl Pts',(21.3414563833941,7.66836769514478,40.5478032411045));
#50545=CARTESIAN_POINT('Ctrl Pts',(22.7835851728612,7.79409049006385,38.3071219957784));
#50546=CARTESIAN_POINT('Ctrl Pts',(21.6889522413839,7.91981328498292,35.8776844818901));
#50547=CARTESIAN_POINT('Ctrl Pts',(19.0551282565062,8.04553607990202,35.4735074102416));
#50548=CARTESIAN_POINT('Ctrl Pts',(17.7365819503052,8.13904770166493,36.9532235056783));
#50549=CARTESIAN_POINT('Ctrl Pts',(17.6348288095622,8.19065172512151,37.9165204024922));
#50550=CARTESIAN_POINT('Ctrl Pts',(17.6364827852058,8.20034815027172,38.0978694718631));
#50551=CARTESIAN_POINT('',(17.6402258042432,8.99409815027172,38.1005671551939));
#50552=CARTESIAN_POINT('Ctrl Pts',(17.6364827852058,8.20034815027172,38.0978694718631));
#50553=CARTESIAN_POINT('Ctrl Pts',(17.6419772323887,8.23255932342787,38.700304512068));
#50554=CARTESIAN_POINT('Ctrl Pts',(18.1821171684312,8.30667809489039,40.0952851716237));
#50555=CARTESIAN_POINT('Ctrl Pts',(20.5253410324787,8.42270446465923,40.8413979527426));
#50556=CARTESIAN_POINT('Ctrl Pts',(22.5856316777532,8.54842725957834,39.1515487448081));
#50557=CARTESIAN_POINT('Ctrl Pts',(22.2895613506621,8.67415005449739,36.5033927354347));
#50558=CARTESIAN_POINT('Ctrl Pts',(19.9069475081291,8.79987284941649,35.3102711297575));
#50559=CARTESIAN_POINT('Ctrl Pts',(17.9577366623079,8.90652221467458,36.4548168564723));
#50560=CARTESIAN_POINT('Ctrl Pts',(17.6411507209954,8.97126398162633,37.6717931370567));
#50561=CARTESIAN_POINT('Ctrl Pts',(17.6402258042432,8.99409815027172,38.1005671551939));
#50562=CARTESIAN_POINT('',(17.6365306272256,9.78784815027173,38.1017218761687));
#50563=CARTESIAN_POINT('Ctrl Pts',(17.6402258042432,8.99409815027172,38.1005671551939));
#50564=CARTESIAN_POINT('Ctrl Pts',(17.6394532193119,9.0131715799327,38.4587230049819));
#50565=CARTESIAN_POINT('Ctrl Pts',(17.8840036200799,9.07415260790002,39.6028076270516));
#50566=CARTESIAN_POINT('Ctrl Pts',(19.6585041852042,9.17704123417373,40.8703116330452));
#50567=CARTESIAN_POINT('Ctrl Pts',(22.1380363316913,9.3027640290928,39.8944488234764));
#50568=CARTESIAN_POINT('Ctrl Pts',(22.6691140974391,9.42848682401188,37.2832528723284));
#50569=CARTESIAN_POINT('Ctrl Pts',(20.7677509459015,9.55420961893096,35.4163822141042));
#50570=CARTESIAN_POINT('Ctrl Pts',(18.2895222809352,9.67399640298303,35.9678425920262));
#50571=CARTESIAN_POINT('Ctrl Pts',(17.6399433145644,9.75187558872876,37.4304476506293));
#50572=CARTESIAN_POINT('Ctrl Pts',(17.6344290770428,9.78784717616812,38.1017052298117));
#50573=CARTESIAN_POINT('',(17.6365307901728,10.5815981503084,38.0980673595779));
#50574=CARTESIAN_POINT('Ctrl Pts',(17.6365306272256,9.78784815027173,38.1017218761687));
#50575=CARTESIAN_POINT('Ctrl Pts',(17.6366112510818,9.79378383643753,38.2123872180115));
#50576=CARTESIAN_POINT('Ctrl Pts',(17.6444651929882,9.79971952260332,38.3227723948623));
#50577=CARTESIAN_POINT('Ctrl Pts',(17.6599710750915,9.80565520876911,38.432046791118));
#50578=CARTESIAN_POINT('Ctrl Pts',(17.6710411319083,9.8098928511466,38.5100606549601));
#50579=CARTESIAN_POINT('Ctrl Pts',(17.6860375731455,9.81413049352408,38.5876667582401));
#50580=CARTESIAN_POINT('Ctrl Pts',(17.7049186169119,9.81836813590157,38.6644394439639));
#50581=CARTESIAN_POINT('Ctrl Pts',(17.7237725089964,9.82259968438302,38.7411017275527));
#50582=CARTESIAN_POINT('Ctrl Pts',(17.746499798886,9.82683123286447,38.8169325222216));
#50583=CARTESIAN_POINT('Ctrl Pts',(17.7730072060122,9.83106278134592,38.8915134467756));
#50584=CARTESIAN_POINT('Ctrl Pts',(17.7994839963513,9.83528944227202,38.9660082283023));
#50585=CARTESIAN_POINT('Ctrl Pts',(17.8297320711137,9.83951610319812,39.0392555691103));
#50586=CARTESIAN_POINT('Ctrl Pts',(17.8636079670862,9.84374276412422,39.1108508903901));
#50587=CARTESIAN_POINT('Ctrl Pts',(17.8974624795375,9.84796675705023,39.1824010184721));
#50588=CARTESIAN_POINT('Ctrl Pts',(17.9349400678453,9.85219074997625,39.2523007742551));
#50589=CARTESIAN_POINT('Ctrl Pts',(17.9758491067801,9.85641474290226,39.3201653995984));
#50590=CARTESIAN_POINT('Ctrl Pts',(18.0167450600346,9.86063738468872,39.3880083169082));
#50591=CARTESIAN_POINT('Ctrl Pts',(18.0610700424113,9.86486002647517,39.4538169953179));
#50592=CARTESIAN_POINT('Ctrl Pts',(18.1085871443441,9.86908266826163,39.5172324616518));
#50593=CARTESIAN_POINT('Ctrl Pts',(18.1561038413518,9.87330527406412,39.5806473875799));
#50594=CARTESIAN_POINT('Ctrl Pts',(18.2068123215903,9.8775278798666,39.6416687676949));
#50595=CARTESIAN_POINT('Ctrl Pts',(18.2604340223364,9.88175048566909,39.6999689529036));
#50596=CARTESIAN_POINT('Ctrl Pts',(18.3141090429816,9.88597729031107,39.7583271101636));
#50597=CARTESIAN_POINT('Ctrl Pts',(18.3707027524758,9.89020409495305,39.8139583216821));
#50598=CARTESIAN_POINT('Ctrl Pts',(18.4298985893385,9.89443089959503,39.8665706895392));
#50599=CARTESIAN_POINT('Ctrl Pts',(18.4891231114666,9.89865975247248,39.9192085524278));
#50600=CARTESIAN_POINT('Ctrl Pts',(18.5509519068367,9.90288860534993,39.9688243636632));
#50601=CARTESIAN_POINT('Ctrl Pts',(18.6150360720197,9.90711745822738,40.0151671882876));
#50602=CARTESIAN_POINT('Ctrl Pts',(18.6792354104909,9.91135391128016,40.0615933011234));
#50603=CARTESIAN_POINT('Ctrl Pts',(18.7456978237154,9.91559036433293,40.1047344181595));
#50604=CARTESIAN_POINT('Ctrl Pts',(18.8140464360769,9.91982681738571,40.1443836687662));
#50605=CARTESIAN_POINT('Ctrl Pts',(18.8761666063443,9.92367721281988,40.1804197800137));
#50606=CARTESIAN_POINT('Ctrl Pts',(18.9398443143707,9.92752760825404,40.2135719016388));
#50607=CARTESIAN_POINT('Ctrl Pts',(19.0047824039744,9.93137800368821,40.2437192860683));
#50608=CARTESIAN_POINT('Ctrl Pts',(19.0762515310092,9.93561564606571,40.2768986921873));
#50609=CARTESIAN_POINT('Ctrl Pts',(19.1495158714723,9.93985328844322,40.3065624231164));
#50610=CARTESIAN_POINT('Ctrl Pts',(19.2241956121396,9.94409093082072,40.3325138281042));
#50611=CARTESIAN_POINT('Ctrl Pts',(19.2987679604092,9.94832247930218,40.3584279139532));
#50612=CARTESIAN_POINT('Ctrl Pts',(19.3747512276241,9.95255402778364,40.380640122966));
#50613=CARTESIAN_POINT('Ctrl Pts',(19.4517436714328,9.95678557626511,40.3990009654383));
#50614=CARTESIAN_POINT('Ctrl Pts',(19.5286471868427,9.96101223719122,40.4173406006304));
#50615=CARTESIAN_POINT('Ctrl Pts',(19.6065571087742,9.96523889811733,40.4318376012495));
#50616=CARTESIAN_POINT('Ctrl Pts',(19.6850559570527,9.96946555904344,40.4423920873142));
#50617=CARTESIAN_POINT('Ctrl Pts',(19.7635052544119,9.97368955196946,40.4529399110583));
#50618=CARTESIAN_POINT('Ctrl Pts',(19.8425422768608,9.97791354489548,40.4595500976168));
#50619=CARTESIAN_POINT('Ctrl Pts',(19.9217399548449,9.98213753782151,40.4621739576569));
#50620=CARTESIAN_POINT('Ctrl Pts',(20.0009122996626,9.98636017960797,40.4647969783961));
#50621=CARTESIAN_POINT('Ctrl Pts',(20.0802447297881,9.99058282139444,40.4634361892354));
#50622=CARTESIAN_POINT('Ctrl Pts',(20.159307155965,9.9948054631809,40.4580949240771));
#50623=CARTESIAN_POINT('Ctrl Pts',(20.2383689083978,9.99902806898339,40.4527537044354));
#50624=CARTESIAN_POINT('Ctrl Pts',(20.3171601938467,10.0032506747859,40.4434321092631));
#50625=CARTESIAN_POINT('Ctrl Pts',(20.3952545265196,10.0074732805884,40.4301854647572));
#50626=CARTESIAN_POINT('Ctrl Pts',(20.4734265139831,10.0117000852304,40.4169256481635));
#50627=CARTESIAN_POINT('Ctrl Pts',(20.5508997010936,10.0159268898723,40.3997330646378));
#50628=CARTESIAN_POINT('Ctrl Pts',(20.6272569084859,10.0201536945143,40.3787143769364));
#50629=CARTESIAN_POINT('Ctrl Pts',(20.703651117243,10.0243825473918,40.3576855039472));
#50630=CARTESIAN_POINT('Ctrl Pts',(20.7789278232766,10.0286114002692,40.3328269804548));
#50631=CARTESIAN_POINT('Ctrl Pts',(20.8526866048507,10.0328402531467,40.3042948974237));
#50632=CARTESIAN_POINT('Ctrl Pts',(20.9265779471188,10.0370767061995,40.2757115359869));
#50633=CARTESIAN_POINT('Ctrl Pts',(20.9989454848812,10.0413131592523,40.2434416145585));
#50634=CARTESIAN_POINT('Ctrl Pts',(21.069410534283,10.0455496123051,40.2076886748437));
#50635=CARTESIAN_POINT('Ctrl Pts',(21.1334542758511,10.0494000077391,40.1751938131949));
#50636=CARTESIAN_POINT('Ctrl Pts',(21.1959265551441,10.0532504031732,40.1398225255816));
#50637=CARTESIAN_POINT('Ctrl Pts',(21.2565643282684,10.0571007986073,40.1017583594988));
#50638=CARTESIAN_POINT('Ctrl Pts',(21.3233006418414,10.0613384409847,40.0598659549346));
#50639=CARTESIAN_POINT('Ctrl Pts',(21.3880649679024,10.0655760833622,40.0145538970917));
#50640=CARTESIAN_POINT('Ctrl Pts',(21.4504855966769,10.0698137257397,39.9660337549821));
#50641=CARTESIAN_POINT('Ctrl Pts',(21.5128164621377,10.0740452742212,39.917583386741));
#50642=CARTESIAN_POINT('Ctrl Pts',(21.5728099564192,10.0782768227026,39.8659343812352));
#50643=CARTESIAN_POINT('Ctrl Pts',(21.6301219948177,10.0825083711841,39.8113423745445));
#50644=CARTESIAN_POINT('Ctrl Pts',(21.6873678362291,10.0867350321102,39.7568134231291));
#50645=CARTESIAN_POINT('Ctrl Pts',(21.7419380388731,10.0909616930363,39.6993485473729));
#50646=CARTESIAN_POINT('Ctrl Pts',(21.7935215673784,10.0951883539624,39.6392435896402));
#50647=CARTESIAN_POINT('Ctrl Pts',(21.845072534753,10.0994123468884,39.5791765720298));
#50648=CARTESIAN_POINT('Ctrl Pts',(21.8936402655684,10.1036363398144,39.5164731350639));
#50649=CARTESIAN_POINT('Ctrl Pts',(21.9389514467888,10.1078603327404,39.4514650302156));
#50650=CARTESIAN_POINT('Ctrl Pts',(21.9842481342043,10.1120829745269,39.3864777196782));
#50651=CARTESIAN_POINT('Ctrl Pts',(22.0262900727396,10.1163056163134,39.3191875894887));
#50652=CARTESIAN_POINT('Ctrl Pts',(22.0648459462335,10.1205282580998,39.2499572423455));
#50653=CARTESIAN_POINT('Ctrl Pts',(22.1034014911669,10.1247508639023,39.1807274851607));
#50654=CARTESIAN_POINT('Ctrl Pts',(22.1384708032911,10.1289734697048,39.1095579541354));
#50655=CARTESIAN_POINT('Ctrl Pts',(22.1698681425892,10.1331960755073,39.0368365303919));
#50656=CARTESIAN_POINT('Ctrl Pts',(22.2012967025113,10.1374228801492,38.9640427945263));
#50657=CARTESIAN_POINT('Ctrl Pts',(22.2290458098626,10.1416496847912,38.889694514852));
#50658=CARTESIAN_POINT('Ctrl Pts',(22.2529778550209,10.1458764894332,38.8141997099449));
#50659=CARTESIAN_POINT('Ctrl Pts',(22.2769214972289,10.1501053423107,38.7386683215783));
#50660=CARTESIAN_POINT('Ctrl Pts',(22.2970442733188,10.1543341951881,38.6619897551865));
#50661=CARTESIAN_POINT('Ctrl Pts',(22.3132591591634,10.1585630480656,38.5845848774434));
#50662=CARTESIAN_POINT('Ctrl Pts',(22.3295031867111,10.1627995011183,38.5070408861726));
#50663=CARTESIAN_POINT('Ctrl Pts',(22.3418252176368,10.1670359541711,38.4287684395224));
#50664=CARTESIAN_POINT('Ctrl Pts',(22.3501898654027,10.1712724072239,38.3501959980866));
#50665=CARTESIAN_POINT('Ctrl Pts',(22.3577922632494,10.175122802658,38.2787836713156));
#50666=CARTESIAN_POINT('Ctrl Pts',(22.3621263178339,10.1789731980922,38.2071238524588));
#50667=CARTESIAN_POINT('Ctrl Pts',(22.3632028170632,10.1828235935264,38.1355371119357));
#50668=CARTESIAN_POINT('Ctrl Pts',(22.3643875833634,10.1870612359039,38.0567506572731));
#50669=CARTESIAN_POINT('Ctrl Pts',(22.3616302904976,10.1912988782814,37.9777570002356));
#50670=CARTESIAN_POINT('Ctrl Pts',(22.3549060820149,10.1955365206589,37.8989831206356));
#50671=CARTESIAN_POINT('Ctrl Pts',(22.3481915432079,10.1997680691403,37.8203225209658));
#50672=CARTESIAN_POINT('Ctrl Pts',(22.3375214570927,10.2039996176218,37.7418815343062));
#50673=CARTESIAN_POINT('Ctrl Pts',(22.3229229709614,10.2082311661032,37.6640879539632));
#50674=CARTESIAN_POINT('Ctrl Pts',(22.3083413464846,10.2124578270293,37.5863842273538));
#50675=CARTESIAN_POINT('Ctrl Pts',(22.2898404249894,10.2166844879554,37.509326879449));
#50676=CARTESIAN_POINT('Ctrl Pts',(22.2674990714423,10.2209111488815,37.4333378652509));
#50677=CARTESIAN_POINT('Ctrl Pts',(22.2451718204538,10.2251351418075,37.3573968176866));
#50678=CARTESIAN_POINT('Ctrl Pts',(22.2190090810641,10.2293591347336,37.2825232138497));
#50679=CARTESIAN_POINT('Ctrl Pts',(22.189140374835,10.2335831276596,37.2091269113014));
#50680=CARTESIAN_POINT('Ctrl Pts',(22.1592812227863,10.237805769446,37.1357540862185));
#50681=CARTESIAN_POINT('Ctrl Pts',(22.1257186345117,10.2420284112325,37.0638580579205));
#50682=CARTESIAN_POINT('Ctrl Pts',(22.0886308720566,10.246251053019,36.9938302475696));
#50683=CARTESIAN_POINT('Ctrl Pts',(22.0515434256514,10.2504736588214,36.9238030339729));
#50684=CARTESIAN_POINT('Ctrl Pts',(22.0109310854571,10.2546962646239,36.8556444202606));
#50685=CARTESIAN_POINT('Ctrl Pts',(21.9670181274846,10.2589188704264,36.7897213551894));
#50686=CARTESIAN_POINT('Ctrl Pts',(21.9230615037117,10.2631456750684,36.7237327380911));
#50687=CARTESIAN_POINT('Ctrl Pts',(21.8757979667557,10.2673724797104,36.6599845010665));
#50688=CARTESIAN_POINT('Ctrl Pts',(21.8254948843686,10.2715992843524,36.5988141793755));
#50689=CARTESIAN_POINT('Ctrl Pts',(21.7751674259893,10.2758281372298,36.5376142156185));
#50690=CARTESIAN_POINT('Ctrl Pts',(21.7217978039609,10.2800569901073,36.4789950028464));
#50691=CARTESIAN_POINT('Ctrl Pts',(21.6656916993704,10.2842858429847,36.4232586354633));
#50692=CARTESIAN_POINT('Ctrl Pts',(21.609484759815,10.2885222960375,36.367422097614));
#50693=CARTESIAN_POINT('Ctrl Pts',(21.5505318605398,10.2927587490903,36.314479071465));
#50694=CARTESIAN_POINT('Ctrl Pts',(21.4891731611,10.296995202143,36.2646924679609));
#50695=CARTESIAN_POINT('Ctrl Pts',(21.4334059300638,10.3008455975772,36.2194427960241));
#50696=CARTESIAN_POINT('Ctrl Pts',(21.3756520105745,10.3046959930113,36.1768001125802));
#50697=CARTESIAN_POINT('Ctrl Pts',(21.3161861910076,10.3085463884455,36.1369298658731));
#50698=CARTESIAN_POINT('Ctrl Pts',(21.2507396982202,10.312784030823,36.0930497372118));
#50699=CARTESIAN_POINT('Ctrl Pts',(21.1829735872081,10.3170216732005,36.0523636865999));
#50700=CARTESIAN_POINT('Ctrl Pts',(21.1132325072472,10.3212593155779,36.0151249855907));
#50701=CARTESIAN_POINT('Ctrl Pts',(21.0435917176962,10.3254908640594,35.977939835295));
#50702=CARTESIAN_POINT('Ctrl Pts',(20.9719820094379,10.3297224125409,35.9441924085928));
#50703=CARTESIAN_POINT('Ctrl Pts',(20.8987770216472,10.3339539610223,35.9140927955975));
#50704=CARTESIAN_POINT('Ctrl Pts',(20.825656587639,10.3381806219484,35.8840279484863));
#50705=CARTESIAN_POINT('Ctrl Pts',(20.7509449671529,10.3424072828745,35.8576027195065));
#50706=CARTESIAN_POINT('Ctrl Pts',(20.6750390535672,10.3466339438006,35.8349806364936));
#50707=CARTESIAN_POINT('Ctrl Pts',(20.5991810541596,10.3508579367267,35.8123728332445));
#50708=CARTESIAN_POINT('Ctrl Pts',(20.5221307060824,10.3550819296527,35.7935635444467));
#50709=CARTESIAN_POINT('Ctrl Pts',(20.4443023287473,10.3593059225787,35.7786672186932));
#50710=CARTESIAN_POINT('Ctrl Pts',(20.3664988465768,10.3635285643652,35.763775657866));
#50711=CARTESIAN_POINT('Ctrl Pts',(20.2879182894395,10.3677512061516,35.7527946626141));
#50712=CARTESIAN_POINT('Ctrl Pts',(20.2089860422268,10.3719738479381,35.7457877591317));
#50713=CARTESIAN_POINT('Ctrl Pts',(20.1300544676489,10.3761964537406,35.7387809153597));
#50714=CARTESIAN_POINT('Ctrl Pts',(20.0507716760174,10.380419059543,35.735748136048));
#50715=CARTESIAN_POINT('Ctrl Pts',(19.9715675701519,10.3846416653455,35.7367010265663));
#50716=CARTESIAN_POINT('Ctrl Pts',(19.892284705969,10.3888684699875,35.7376548646119));
#50717=CARTESIAN_POINT('Ctrl Pts',(19.8130811536719,10.3930952746295,35.7426022834191));
#50718=CARTESIAN_POINT('Ctrl Pts',(19.734385598417,10.3973220792715,35.7515027292816));
#50719=CARTESIAN_POINT('Ctrl Pts',(19.655651908675,10.4015509321489,35.7604074881442));
#50720=CARTESIAN_POINT('Ctrl Pts',(19.5774271695223,10.4057797850264,35.7732690139461));
#50721=CARTESIAN_POINT('Ctrl Pts',(19.5001311912394,10.4100086379038,35.7899953214488));
#50722=CARTESIAN_POINT('Ctrl Pts',(19.422696295145,10.4142450909566,35.8067516897916));
#50723=CARTESIAN_POINT('Ctrl Pts',(19.3461939487898,10.4184815440094,35.8273865959679));
#50724=CARTESIAN_POINT('Ctrl Pts',(19.2710298605755,10.4227179970622,35.8517578029208));
#50725=CARTESIAN_POINT('Ctrl Pts',(19.2027152921228,10.4265683924963,35.8739081213137));
#50726=CARTESIAN_POINT('Ctrl Pts',(19.1355062167052,10.4304187879304,35.8991440847221));
#50727=CARTESIAN_POINT('Ctrl Pts',(19.0696910005683,10.4342691833645,35.9273252414417));
#50728=CARTESIAN_POINT('Ctrl Pts',(18.9972565314969,10.438506825742,35.9583406698581));
#50729=CARTESIAN_POINT('Ctrl Pts',(18.9262388203568,10.4427444681195,35.9930406009896));
#50730=CARTESIAN_POINT('Ctrl Pts',(18.8570379332917,10.446982110497,36.031273784435));
#50731=CARTESIAN_POINT('Ctrl Pts',(18.7879365598179,10.4512136589785,36.0694519870622));
#50732=CARTESIAN_POINT('Ctrl Pts',(18.7206472288333,10.4554452074599,36.1111531268728));
#50733=CARTESIAN_POINT('Ctrl Pts',(18.655549563203,10.4596767559414,36.1561781295869));
#50734=CARTESIAN_POINT('Ctrl Pts',(18.5905270871742,10.4639034168675,36.2011511271795));
#50735=CARTESIAN_POINT('Ctrl Pts',(18.5276916294922,10.4681300777936,36.2494400930017));
#50736=CARTESIAN_POINT('Ctrl Pts',(18.4673964115256,10.4723567387197,36.3008011000739));
#50737=CARTESIAN_POINT('Ctrl Pts',(18.4071392537795,10.4765807316457,36.352129686478));
#50738=CARTESIAN_POINT('Ctrl Pts',(18.3494195089428,10.4808047245717,36.4065261619143));
#50739=CARTESIAN_POINT('Ctrl Pts',(18.2945587130075,10.4850287174977,36.4637052656928));
#50740=CARTESIAN_POINT('Ctrl Pts',(18.2397154655372,10.4892513592842,36.5208660794433));
#50741=CARTESIAN_POINT('Ctrl Pts',(18.1877296752638,10.4934740010706,36.5808074159847));
#50742=CARTESIAN_POINT('Ctrl Pts',(18.1388861843631,10.4976966428571,36.6432070132838));
#50743=CARTESIAN_POINT('Ctrl Pts',(18.0900431096907,10.5019192486596,36.7056060788339));
#50744=CARTESIAN_POINT('Ctrl Pts',(18.0443425689648,10.5061418544621,36.7704629934736));
#50745=CARTESIAN_POINT('Ctrl Pts',(18.0020283089336,10.5103644602645,36.8374234428768));
#50746=CARTESIAN_POINT('Ctrl Pts',(17.9596719728017,10.5145912649065,36.9044504758526));
#50747=CARTESIAN_POINT('Ctrl Pts',(17.9207088944077,10.5188180695485,36.9735848245615));
#50748=CARTESIAN_POINT('Ctrl Pts',(17.885338403124,10.5230448741905,37.044444804097));
#50749=CARTESIAN_POINT('Ctrl Pts',(17.84995077192,10.5272737270679,37.1153391211369));
#50750=CARTESIAN_POINT('Ctrl Pts',(17.8181593841433,10.5315025799454,37.1879603048555));
#50751=CARTESIAN_POINT('Ctrl Pts',(17.7901155940106,10.5357314328228,37.2619061191818));
#50752=CARTESIAN_POINT('Ctrl Pts',(17.7620214030416,10.5399678858756,37.3359848303409));
#50753=CARTESIAN_POINT('Ctrl Pts',(17.7376884117068,10.5442043389284,37.4113924816997));
#50754=CARTESIAN_POINT('Ctrl Pts',(17.7172181434474,10.5484407919811,37.4877113129461));
#50755=CARTESIAN_POINT('Ctrl Pts',(17.6986132807333,10.5522911874153,37.5570753955191));
#50756=CARTESIAN_POINT('Ctrl Pts',(17.6831986247484,10.5561415828494,37.6271917420335));
#50757=CARTESIAN_POINT('Ctrl Pts',(17.6710133231036,10.5599919782835,37.6977419985394));
#50758=CARTESIAN_POINT('Ctrl Pts',(17.6502336907217,10.5665580694628,37.8180515680009));
#50759=CARTESIAN_POINT('Ctrl Pts',(17.6387726117503,10.573124160642,37.9400146317809));
#50760=CARTESIAN_POINT('Ctrl Pts',(17.6368279557372,10.5796902518213,38.0624722753877));
#50761=CARTESIAN_POINT('Ctrl Pts',(17.6366396038906,10.5803262179714,38.0743330482635));
#50762=CARTESIAN_POINT('Ctrl Pts',(17.6365404955559,10.5809621841216,38.0861984337401));
#50763=CARTESIAN_POINT('Ctrl Pts',(17.6365307901734,10.5815981502717,38.0980673588938));
#50764=CARTESIAN_POINT('',(17.6365300074329,11.3753481502331,38.0998125575523));
#50765=CARTESIAN_POINT('Ctrl Pts',(17.6365307901728,10.5815981503084,38.0980673595779));
#50766=CARTESIAN_POINT('Ctrl Pts',(17.6364645857,10.585936342929,38.1790302905545));
#50767=CARTESIAN_POINT('Ctrl Pts',(17.640563531315,10.5902745355496,38.2601393309714));
#50768=CARTESIAN_POINT('Ctrl Pts',(17.6488415013264,10.5946127281702,38.3409235459956));
#50769=CARTESIAN_POINT('Ctrl Pts',(17.656787108768,10.5987767412702,38.4184642545474));
#50770=CARTESIAN_POINT('Ctrl Pts',(17.6685825490526,10.6029407543702,38.4957051822));
#50771=CARTESIAN_POINT('Ctrl Pts',(17.6841870367672,10.6071047674702,38.5722295630548));
#50772=CARTESIAN_POINT('Ctrl Pts',(17.6997824680218,10.6112663638797,38.6487095310455));
#50773=CARTESIAN_POINT('Ctrl Pts',(17.7191824658297,10.6154279602891,38.7244733038589));
#50774=CARTESIAN_POINT('Ctrl Pts',(17.7422947371148,10.6195895566986,38.7991118557431));
#50775=CARTESIAN_POINT('Ctrl Pts',(17.7654012946875,10.6237501242968,38.873731955818));
#50776=CARTESIAN_POINT('Ctrl Pts',(17.7922181608439,10.627910691895,38.9472269249856));
#50777=CARTESIAN_POINT('Ctrl Pts',(17.822602968645,10.6320712594932,39.0192021588021));
#50778=CARTESIAN_POINT('Ctrl Pts',(17.8529903875591,10.636232184629,39.0911835777974));
#50779=CARTESIAN_POINT('Ctrl Pts',(17.8869461655744,10.6403931097648,39.1616445575498));
#50780=CARTESIAN_POINT('Ctrl Pts',(17.9242801823507,10.6445540349007,39.230211342855));
#50781=CARTESIAN_POINT('Ctrl Pts',(17.9616524192876,10.6487192197235,39.2988483224164));
#50782=CARTESIAN_POINT('Ctrl Pts',(18.0024095615276,10.6528844045463,39.3655868139426));
#50783=CARTESIAN_POINT('Ctrl Pts',(18.0463164606769,10.6570495893692,39.4300793469105));
#50784=CARTESIAN_POINT('Ctrl Pts',(18.0902500971362,10.6612173106007,39.4946111529058));
#50785=CARTESIAN_POINT('Ctrl Pts',(18.1373370118005,10.6653850318321,39.5568938960868));
#50786=CARTESIAN_POINT('Ctrl Pts',(18.1873014405384,10.6695527530636,39.6166127961434));
#50787=CARTESIAN_POINT('Ctrl Pts',(18.2373451387713,10.6737270864623,39.6764264413451));
#50788=CARTESIAN_POINT('Ctrl Pts',(18.2902751262759,10.677901419861,39.7336677789488));
#50789=CARTESIAN_POINT('Ctrl Pts',(18.3457791175477,10.6820757532597,39.7880591556456));
#50790=CARTESIAN_POINT('Ctrl Pts',(18.3619078509177,10.6832887599073,39.8038645777831));
#50791=CARTESIAN_POINT('Ctrl Pts',(18.3782537283861,10.684501766555,39.8194296123154));
#50792=CARTESIAN_POINT('Ctrl Pts',(18.3948086017898,10.6857147732027,39.8347481131311));
#50793=CARTESIAN_POINT('Ctrl Pts',(18.4526431018926,10.6899524155802,39.8882633418736));
#50794=CARTESIAN_POINT('Ctrl Pts',(18.5132652934297,10.6941900579577,39.9389836574223));
#50795=CARTESIAN_POINT('Ctrl Pts',(18.5763740608301,10.6984277003352,39.9866053180839));
#50796=CARTESIAN_POINT('Ctrl Pts',(18.6393920753463,10.7026592488166,40.0341584969287));
#50797=CARTESIAN_POINT('Ctrl Pts',(18.7048891934309,10.7068907972981,40.0786215900338));
#50798=CARTESIAN_POINT('Ctrl Pts',(18.7725289528581,10.7111223457796,40.1197290088842));
#50799=CARTESIAN_POINT('Ctrl Pts',(18.8400905864953,10.7153490067057,40.1607889475307));
#50800=CARTESIAN_POINT('Ctrl Pts',(18.9097895448374,10.7195756676318,40.1985006720779));
#50801=CARTESIAN_POINT('Ctrl Pts',(18.9812591597996,10.7238023285579,40.2326409780851));
#50802=CARTESIAN_POINT('Ctrl Pts',(19.0526836609138,10.7280263214839,40.2667597336673));
#50803=CARTESIAN_POINT('Ctrl Pts',(19.1258761782657,10.7322503144099,40.2973113438965));
#50804=CARTESIAN_POINT('Ctrl Pts',(19.2004452042721,10.7364743073359,40.3241183802866));
#50805=CARTESIAN_POINT('Ctrl Pts',(19.274990377691,10.7406969491224,40.3509168418405));
#50806=CARTESIAN_POINT('Ctrl Pts',(19.3509107445848,10.7449195909088,40.3739729496525));
#50807=CARTESIAN_POINT('Ctrl Pts',(19.4277959548363,10.7491422326953,40.3931578601567));
#50808=CARTESIAN_POINT('Ctrl Pts',(19.5046805098969,10.7533648384978,40.4123426071733));
#50809=CARTESIAN_POINT('Ctrl Pts',(19.5825294367942,10.7575874443003,40.42765611037));
#50810=CARTESIAN_POINT('Ctrl Pts',(19.6609198558077,10.7618100501027,40.4390201146451));
#50811=CARTESIAN_POINT('Ctrl Pts',(19.7393882240316,10.7660368547447,40.4503954189639));
#50812=CARTESIAN_POINT('Ctrl Pts',(19.8183986949142,10.7702636593867,40.4578133122121));
#50813=CARTESIAN_POINT('Ctrl Pts',(19.8975214880639,10.7744904640287,40.4612472542052));
#50814=CARTESIAN_POINT('Ctrl Pts',(19.9766826227329,10.7787193169061,40.4646828602263));
#50815=CARTESIAN_POINT('Ctrl Pts',(20.0559557187369,10.7829481697836,40.4641306723745));
#50816=CARTESIAN_POINT('Ctrl Pts',(20.1349117722814,10.7871770226611,40.459616336314));
#50817=CARTESIAN_POINT('Ctrl Pts',(20.2140097271565,10.7914134757138,40.4550938870023));
#50818=CARTESIAN_POINT('Ctrl Pts',(20.2927890338919,10.7956499287666,40.4465951117349));
#50819=CARTESIAN_POINT('Ctrl Pts',(20.3708268121079,10.7998863818194,40.4341974887147));
#50820=CARTESIAN_POINT('Ctrl Pts',(20.4417531982116,10.8037367772535,40.4229296307976));
#50821=CARTESIAN_POINT('Ctrl Pts',(20.5120669072558,10.8075871726876,40.408441843249));
#50822=CARTESIAN_POINT('Ctrl Pts',(20.5814612535748,10.8114375681218,40.3908280711331));
#50823=CARTESIAN_POINT('Ctrl Pts',(20.6578348177323,10.8156752104993,40.3714428239752));
#50824=CARTESIAN_POINT('Ctrl Pts',(20.733381259297,10.8199128528767,40.3481977022715));
#50825=CARTESIAN_POINT('Ctrl Pts',(20.8076818713031,10.8241504952542,40.3211799647188));
#50826=CARTESIAN_POINT('Ctrl Pts',(20.8818756361132,10.8283820437357,40.294201079733));
#50827=CARTESIAN_POINT('Ctrl Pts',(20.9548266923092,10.8326135922171,40.2634605116557));
#50828=CARTESIAN_POINT('Ctrl Pts',(21.0261290979499,10.8368451406986,40.2290959384773));
#50829=CARTESIAN_POINT('Ctrl Pts',(21.0973491473432,10.8410718016247,40.1947710573298));
#50830=CARTESIAN_POINT('Ctrl Pts',(21.1669239102289,10.8452984625508,40.1568306918639));
#50831=CARTESIAN_POINT('Ctrl Pts',(21.2344665571698,10.8495251234769,40.1154609299437));
#50832=CARTESIAN_POINT('Ctrl Pts',(21.3019665690871,10.8537491164029,40.0741172819064));
#50833=CARTESIAN_POINT('Ctrl Pts',(21.3674366124437,10.8579731093289,40.0293487783934));
#50834=CARTESIAN_POINT('Ctrl Pts',(21.4305147367452,10.8621971022549,39.9813872617977));
#50835=CARTESIAN_POINT('Ctrl Pts',(21.4935726840838,10.8664197440414,39.9334410867765));
#50836=CARTESIAN_POINT('Ctrl Pts',(21.5542398588359,10.8706423858279,39.8823042104119));
#50837=CARTESIAN_POINT('Ctrl Pts',(21.6121848101614,10.8748650276143,39.8282507279862));
#50838=CARTESIAN_POINT('Ctrl Pts',(21.6701292676988,10.8790876334168,39.7741977061867));
#50839=CARTESIAN_POINT('Ctrl Pts',(21.7253512061264,10.8833102392193,39.7172284485515));
#50840=CARTESIAN_POINT('Ctrl Pts',(21.7775547913187,10.8875328450218,39.6576550981395));
#50841=CARTESIAN_POINT('Ctrl Pts',(21.8298102862763,10.8917596496637,39.5980225096765));
#50842=CARTESIAN_POINT('Ctrl Pts',(21.8790411230933,10.8959864543057,39.5357810094083));
#50843=CARTESIAN_POINT('Ctrl Pts',(21.9249910933316,10.9002132589477,39.4712766794101));
#50844=CARTESIAN_POINT('Ctrl Pts',(21.9709633301203,10.9044421118252,39.4067410917438));
#50845=CARTESIAN_POINT('Ctrl Pts',(22.0136512804146,10.9086709647026,39.3399408854482));
#50846=CARTESIAN_POINT('Ctrl Pts',(22.0528429355228,10.9128998175801,39.2712498977478));
#50847=CARTESIAN_POINT('Ctrl Pts',(22.0921050266236,10.9171362706328,39.2024354572896));
#50848=CARTESIAN_POINT('Ctrl Pts',(22.1278580552572,10.9213727236856,39.1317238649282));
#50849=CARTESIAN_POINT('Ctrl Pts',(22.1599368265607,10.9256091767384,39.0595120354465));
#50850=CARTESIAN_POINT('Ctrl Pts',(22.1890923377918,10.9294595721726,38.993880693599));
#50851=CARTESIAN_POINT('Ctrl Pts',(22.2152132525274,10.9333099676067,38.9270105845734));
#50852=CARTESIAN_POINT('Ctrl Pts',(22.2382114383322,10.9371603630409,38.8592101146711));
#50853=CARTESIAN_POINT('Ctrl Pts',(22.2635226273876,10.9413980054184,38.7845907283287));
#50854=CARTESIAN_POINT('Ctrl Pts',(22.2851456605777,10.9456356477959,38.7085641214613));
#50855=CARTESIAN_POINT('Ctrl Pts',(22.3029258193166,10.9498732901734,38.6315290317802));
#50856=CARTESIAN_POINT('Ctrl Pts',(22.3206804094894,10.9541048386548,38.5546047215811));
#50857=CARTESIAN_POINT('Ctrl Pts',(22.3346029951879,10.9583363871363,38.4766752615975));
#50858=CARTESIAN_POINT('Ctrl Pts',(22.3445881013937,10.9625679356177,38.3981561263885));
#50859=CARTESIAN_POINT('Ctrl Pts',(22.3545616745261,10.9667945965438,38.319727682949));
#50860=CARTESIAN_POINT('Ctrl Pts',(22.360606747145,10.9710212574699,38.2407113804582));
#50861=CARTESIAN_POINT('Ctrl Pts',(22.3626688573211,10.975247918396,38.1615330118293));
#50862=CARTESIAN_POINT('Ctrl Pts',(22.3647296658291,10.9794719113221,38.0824046230541));
#50863=CARTESIAN_POINT('Ctrl Pts',(22.3628124900714,10.9836959042481,38.0031148385859));
#50864=CARTESIAN_POINT('Ctrl Pts',(22.3569147926027,10.9879198971741,37.9240934870149));
#50865=CARTESIAN_POINT('Ctrl Pts',(22.3510189816458,10.9921425389605,37.8450974122081));
#50866=CARTESIAN_POINT('Ctrl Pts',(22.3411452122845,10.996365180747,37.766370066925));
#50867=CARTESIAN_POINT('Ctrl Pts',(22.3273429936983,11.0005878225335,37.6883386943332));
#50868=CARTESIAN_POINT('Ctrl Pts',(22.3135408927301,11.004810428336,37.6103079866992));
#50869=CARTESIAN_POINT('Ctrl Pts',(22.2958104921561,11.0090330341384,37.5329737013224));
#50870=CARTESIAN_POINT('Ctrl Pts',(22.2742526056455,11.0132556399409,37.4567539144196));
#50871=CARTESIAN_POINT('Ctrl Pts',(22.2526732825838,11.0174824445829,37.3804583367218));
#50872=CARTESIAN_POINT('Ctrl Pts',(22.2272589990749,11.0217092492249,37.3052799233104));
#50873=CARTESIAN_POINT('Ctrl Pts',(22.1981606087981,11.0259360538669,37.23162198391));
#50874=CARTESIAN_POINT('Ctrl Pts',(22.1690481179513,11.0301649067443,37.1579283511628));
#50875=CARTESIAN_POINT('Ctrl Pts',(22.1362481581054,11.0343937596218,37.0857570875216));
#50876=CARTESIAN_POINT('Ctrl Pts',(22.0999589253276,11.0386226124992,37.0154895330901));
#50877=CARTESIAN_POINT('Ctrl Pts',(22.063604472846,11.042859065552,36.945095692465));
#50878=CARTESIAN_POINT('Ctrl Pts',(22.0237484537432,11.0470955186048,36.8766128034194));
#50879=CARTESIAN_POINT('Ctrl Pts',(21.9806339055323,11.0513319716575,36.8103954973885));
#50880=CARTESIAN_POINT('Ctrl Pts',(21.9414482807872,11.0551823670917,36.7502124127122));
#50881=CARTESIAN_POINT('Ctrl Pts',(21.8995716557137,11.0590327625258,36.6919006476892));
#50882=CARTESIAN_POINT('Ctrl Pts',(21.8552147687459,11.0628831579599,36.6357020102701));
#50883=CARTESIAN_POINT('Ctrl Pts',(21.8063967636439,11.0671208003374,36.5738512908939));
#50884=CARTESIAN_POINT('Ctrl Pts',(21.754390692574,11.0713584427149,36.5143284458008));
#50885=CARTESIAN_POINT('Ctrl Pts',(21.6994468248549,11.0755960850924,36.4574803105014));
#50886=CARTESIAN_POINT('Ctrl Pts',(21.6445819685736,11.0798276335739,36.4007139250514));
#50887=CARTESIAN_POINT('Ctrl Pts',(21.5867880285279,11.0840591820553,36.3466149452102));
#50888=CARTESIAN_POINT('Ctrl Pts',(21.5263561190588,11.0882907305368,36.2954980081164));
#50889=CARTESIAN_POINT('Ctrl Pts',(21.465994010114,11.0925173914629,36.2444401124967));
#50890=CARTESIAN_POINT('Ctrl Pts',(21.4030003428528,11.096744052389,36.196357716058));
#50891=CARTESIAN_POINT('Ctrl Pts',(21.3377026555861,11.1009707133151,36.151528279359));
#50892=CARTESIAN_POINT('Ctrl Pts',(21.2724461862546,11.1051947062411,36.1067271403975));
#50893=CARTESIAN_POINT('Ctrl Pts',(21.204888969131,11.1094186991671,36.0651751500913));
#50894=CARTESIAN_POINT('Ctrl Pts',(21.1353901922661,11.1136426920931,36.0271084079948));
#50895=CARTESIAN_POINT('Ctrl Pts',(21.065913646155,11.1178653338796,35.9890538424057));
#50896=CARTESIAN_POINT('Ctrl Pts',(20.994497184432,11.122087975666,35.9544825362157));
#50897=CARTESIAN_POINT('Ctrl Pts',(20.921526157148,11.1263106174525,35.9235855214155));
#50898=CARTESIAN_POINT('Ctrl Pts',(20.8485557516991,11.130533223255,35.8926887699096));
#50899=CARTESIAN_POINT('Ctrl Pts',(20.7740312392585,11.1347558290575,35.8654664289973));
#50900=CARTESIAN_POINT('Ctrl Pts',(20.6983582068759,11.13897843486,35.8420615030987));
#50901=CARTESIAN_POINT('Ctrl Pts',(20.6226099273753,11.1432052395019,35.8186333040053));
#50902=CARTESIAN_POINT('Ctrl Pts',(20.5457112955545,11.1474320441439,35.7990302411467));
#50903=CARTESIAN_POINT('Ctrl Pts',(20.4680827498871,11.1516588487859,35.7833453040735));
#50904=CARTESIAN_POINT('Ctrl Pts',(20.3904165867866,11.1558877016634,35.7676527663548));
#50905=CARTESIAN_POINT('Ctrl Pts',(20.3120202693913,11.1601165545408,35.7558822064558));
#50906=CARTESIAN_POINT('Ctrl Pts',(20.2333215767156,11.1643454074183,35.7480749410879));
#50907=CARTESIAN_POINT('Ctrl Pts',(20.1544814452432,11.1685818604711,35.7402536443531));
#50908=CARTESIAN_POINT('Ctrl Pts',(20.0753383219877,11.1728183135238,35.7364098972061));
#50909=CARTESIAN_POINT('Ctrl Pts',(19.9963219897195,11.1770547665766,35.7365328618446));
#50910=CARTESIAN_POINT('Ctrl Pts',(19.9245062228041,11.1809051620107,35.736644621016));
#50911=CARTESIAN_POINT('Ctrl Pts',(19.8527954382003,11.1847555574448,35.7400323989185));
#50912=CARTESIAN_POINT('Ctrl Pts',(19.781507193178,11.188605952879,35.7466510385693));
#50913=CARTESIAN_POINT('Ctrl Pts',(19.7030492546903,11.1928435952564,35.7539353365967));
#50914=CARTESIAN_POINT('Ctrl Pts',(19.6248087169068,11.1970812376339,35.765161144516));
#50915=CARTESIAN_POINT('Ctrl Pts',(19.547212759378,11.2013188800114,35.7803073143992));
#50916=CARTESIAN_POINT('Ctrl Pts',(19.4697283878813,11.2055504284929,35.7954317034957));
#50917=CARTESIAN_POINT('Ctrl Pts',(19.3928872121281,11.2097819769743,35.814465169672));
#50918=CARTESIAN_POINT('Ctrl Pts',(19.3171116348953,11.2140135254558,35.8373347747171));
#50919=CARTESIAN_POINT('Ctrl Pts',(19.2414235805467,11.2182401863819,35.8601779647368));
#50920=CARTESIAN_POINT('Ctrl Pts',(19.1667991253259,11.222466847308,35.8868483536596));
#50921=CARTESIAN_POINT('Ctrl Pts',(19.093649312643,11.2266935082341,35.9172222118531));
#50922=CARTESIAN_POINT('Ctrl Pts',(19.0205456744013,11.2309175011601,35.9475768971209));
#50923=CARTESIAN_POINT('Ctrl Pts',(18.9489152628844,11.2351414940861,35.9816302321969));
#50924=CARTESIAN_POINT('Ctrl Pts',(18.879151653174,11.2393654870121,36.0192094232438));
#50925=CARTESIAN_POINT('Ctrl Pts',(18.8094103589302,11.2435881287986,36.0567765937375));
#50926=CARTESIAN_POINT('Ctrl Pts',(18.7415350931024,11.247810770585,36.0978671584149));
#50927=CARTESIAN_POINT('Ctrl Pts',(18.6758958659601,11.2520334123715,36.1422618451084));
#50928=CARTESIAN_POINT('Ctrl Pts',(18.6102571981736,11.256256018174,36.186656153485));
#50929=CARTESIAN_POINT('Ctrl Pts',(18.5468549186846,11.2604786239765,36.2343542640857));
#50930=CARTESIAN_POINT('Ctrl Pts',(18.4860297647078,11.264701229779,36.2850937854674));
#50931=CARTESIAN_POINT('Ctrl Pts',(18.4251441279225,11.268928034421,36.3358837607904));
#50932=CARTESIAN_POINT('Ctrl Pts',(18.3668410963031,11.273154839063,36.3897208869518));
#50933=CARTESIAN_POINT('Ctrl Pts',(18.3114275353693,11.2773816437049,36.44630308926));
#50934=CARTESIAN_POINT('Ctrl Pts',(18.2559871219948,11.2816104965824,36.5029127103121));
#50935=CARTESIAN_POINT('Ctrl Pts',(18.2034392797682,11.2858393494599,36.5622697060143));
#50936=CARTESIAN_POINT('Ctrl Pts',(18.154051523256,11.2900682023373,36.6240377165705));
#50937=CARTESIAN_POINT('Ctrl Pts',(18.1045750061226,11.2943046553901,36.6859167377775));
#50938=CARTESIAN_POINT('Ctrl Pts',(18.0582701972243,11.2985411084429,36.7502150505365));
#50939=CARTESIAN_POINT('Ctrl Pts',(18.0153619511129,11.3027775614956,36.8165662246109));
#50940=CARTESIAN_POINT('Ctrl Pts',(17.9763638286608,11.3066279569298,36.876870978263));
#50941=CARTESIAN_POINT('Ctrl Pts',(17.9401709977417,11.3104783523639,36.9388709190513));
#50942=CARTESIAN_POINT('Ctrl Pts',(17.9069184353317,11.3143287477981,37.0022750779245));
#50943=CARTESIAN_POINT('Ctrl Pts',(17.8681932052737,11.3188128367884,37.076114218762));
#50944=CARTESIAN_POINT('Ctrl Pts',(17.8333244380349,11.3232969257787,37.1521088126688));
#50945=CARTESIAN_POINT('Ctrl Pts',(17.8025426710631,11.3277810147689,37.2298438482654));
#50946=CARTESIAN_POINT('Ctrl Pts',(17.7718532744003,11.3322516478492,37.3073456156009));
#50947=CARTESIAN_POINT('Ctrl Pts',(17.7452265869857,11.3367222809295,37.3865770613249));
#50948=CARTESIAN_POINT('Ctrl Pts',(17.7228462170966,11.3411929140099,37.4671010428919));
#50949=CARTESIAN_POINT('Ctrl Pts',(17.7005069260382,11.3456553413107,37.5474772239072));
#50950=CARTESIAN_POINT('Ctrl Pts',(17.6823985487696,11.3501177686115,37.6291408496797));
#50951=CARTESIAN_POINT('Ctrl Pts',(17.6686561326386,11.3545801959123,37.711636493712));
#50952=CARTESIAN_POINT('Ctrl Pts',(17.6549469886206,11.359031819117,37.7939324054432));
#50953=CARTESIAN_POINT('Ctrl Pts',(17.6455828135995,11.3634834423216,37.8770559423081));
#50954=CARTESIAN_POINT('Ctrl Pts',(17.6406481221886,11.3679350655263,37.9605397634879));
#50955=CARTESIAN_POINT('Ctrl Pts',(17.6379089501496,11.3704060937619,38.006880361034));
#50956=CARTESIAN_POINT('Ctrl Pts',(17.6365336937416,11.3728771219975,38.0533317298038));
#50957=CARTESIAN_POINT('Ctrl Pts',(17.6365300074329,11.3753481502331,38.0998125575523));
#50958=CARTESIAN_POINT('',(17.636530903764,12.1690981502314,38.10206689074));
#50959=CARTESIAN_POINT('Ctrl Pts',(17.6365300074328,11.3753481502717,38.0998125582779));
#50960=CARTESIAN_POINT('Ctrl Pts',(17.6365234494525,11.3797441513659,38.1825027382993));
#50961=CARTESIAN_POINT('Ctrl Pts',(17.6408608001244,11.3841401524601,38.2651212912942));
#50962=CARTESIAN_POINT('Ctrl Pts',(17.6494937094782,11.3885361535542,38.3472056211282));
#50963=CARTESIAN_POINT('Ctrl Pts',(17.6581476503877,11.3929428642178,38.4294899253955));
#50964=CARTESIAN_POINT('Ctrl Pts',(17.6711180189738,11.3973495748814,38.5112369962023));
#50965=CARTESIAN_POINT('Ctrl Pts',(17.688304818639,11.401756285545,38.5919916964463));
#50966=CARTESIAN_POINT('Ctrl Pts',(17.7055127065732,11.4061684032594,38.6728454830171));
#50967=CARTESIAN_POINT('Ctrl Pts',(17.7269472330067,11.4105805209739,38.7527040752355));
#50968=CARTESIAN_POINT('Ctrl Pts',(17.7524584399641,11.4149926386884,38.8311274696054));
#50969=CARTESIAN_POINT('Ctrl Pts',(17.7780370260216,11.4194164094979,38.9097579924635));
#50970=CARTESIAN_POINT('Ctrl Pts',(17.8077136725913,11.4238401803075,38.9869453542417));
#50971=CARTESIAN_POINT('Ctrl Pts',(17.8412898630427,11.428263951117,39.0622686659649));
#50972=CARTESIAN_POINT('Ctrl Pts',(17.8711122655108,11.4321931483171,39.1291708989829));
#50973=CARTESIAN_POINT('Ctrl Pts',(17.9040102459344,11.4361223455171,39.1946027443427));
#50974=CARTESIAN_POINT('Ctrl Pts',(17.9398154781111,11.4400515427171,39.2582876053336));
#50975=CARTESIAN_POINT('Ctrl Pts',(17.9784314501492,11.4442891850946,39.3269717797339));
#50976=CARTESIAN_POINT('Ctrl Pts',(18.0205584409762,11.4485268274721,39.3938516508459));
#50977=CARTESIAN_POINT('Ctrl Pts',(18.0660031052796,11.4527644698496,39.4585457121908));
#50978=CARTESIAN_POINT('Ctrl Pts',(18.1113824183724,11.456996018331,39.5231467409367));
#50979=CARTESIAN_POINT('Ctrl Pts',(18.1600696630579,11.4612275668125,39.585567821757));
#50980=CARTESIAN_POINT('Ctrl Pts',(18.2118261425487,11.465459115294,39.6454529098059));
#50981=CARTESIAN_POINT('Ctrl Pts',(18.2635228418764,11.4696857762201,39.7052688289244));
#50982=CARTESIAN_POINT('Ctrl Pts',(18.3182814261258,11.4739124371462,39.7625542233394));
#50983=CARTESIAN_POINT('Ctrl Pts',(18.3758214409796,11.4781390980723,39.816984114463));
#50984=CARTESIAN_POINT('Ctrl Pts',(18.4333251347829,11.4823630909983,39.8713796477432));
#50985=CARTESIAN_POINT('Ctrl Pts',(18.4936064346114,11.4865870839243,39.9229229341624));
#50986=CARTESIAN_POINT('Ctrl Pts',(18.5563471947755,11.4908110768503,39.9713249367407));
#50987=CARTESIAN_POINT('Ctrl Pts',(18.6190678858902,11.4950337186368,40.019711456845));
#50988=CARTESIAN_POINT('Ctrl Pts',(18.6842461041889,11.4992563604232,40.0649584023344));
#50989=CARTESIAN_POINT('Ctrl Pts',(18.7515308578564,11.5034790022097,40.1068171919772));
#50990=CARTESIAN_POINT('Ctrl Pts',(18.8188150381452,11.5077016080122,40.1486756249131));
#50991=CARTESIAN_POINT('Ctrl Pts',(18.8882053193212,11.5119242138147,40.1871457130015));
#50992=CARTESIAN_POINT('Ctrl Pts',(18.9593232566276,11.5161468196172,40.2220231753456));
#50993=CARTESIAN_POINT('Ctrl Pts',(19.0305119115947,11.5203736242591,40.2569353188495));
#50994=CARTESIAN_POINT('Ctrl Pts',(19.1034312324066,11.5246004289011,40.2882474938245));
#50995=CARTESIAN_POINT('Ctrl Pts',(19.1776803327944,11.5288272335431,40.3158025195913));
#50996=CARTESIAN_POINT('Ctrl Pts',(19.2519654129954,11.5330560864206,40.3433708980406));
#50997=CARTESIAN_POINT('Ctrl Pts',(19.3275811087614,11.537284939298,40.3671783593769));
#50998=CARTESIAN_POINT('Ctrl Pts',(19.4041112544086,11.5415137921755,40.387117627884));
#50999=CARTESIAN_POINT('Ctrl Pts',(19.4807789414983,11.5457502452283,40.407092731626));
#51000=CARTESIAN_POINT('Ctrl Pts',(19.5583639021829,11.549986698281,40.4231856563543));
#51001=CARTESIAN_POINT('Ctrl Pts',(19.6364398885131,11.5542231513338,40.4353403362756));
#51002=CARTESIAN_POINT('Ctrl Pts',(19.7074010009196,11.558073546768,40.446387389905));
#51003=CARTESIAN_POINT('Ctrl Pts',(19.7787673752423,11.5619239422021,40.4541818933362));
#51004=CARTESIAN_POINT('Ctrl Pts',(19.8502182944387,11.5657743376363,40.4587191188395));
#51005=CARTESIAN_POINT('Ctrl Pts',(19.9288552677771,11.5700119800138,40.4637126680471));
#51006=CARTESIAN_POINT('Ctrl Pts',(20.0078898418441,11.5742496223913,40.4647787910041));
#51007=CARTESIAN_POINT('Ctrl Pts',(20.0868967384967,11.5784872647688,40.461872011295));
#51008=CARTESIAN_POINT('Ctrl Pts',(20.1657900201316,11.5827188132502,40.4589694116492));
#51009=CARTESIAN_POINT('Ctrl Pts',(20.2446552388075,11.5869503617317,40.4521052722963));
#51010=CARTESIAN_POINT('Ctrl Pts',(20.3230637889011,11.5911819102132,40.4412860203745));
#51011=CARTESIAN_POINT('Ctrl Pts',(20.4013817749539,11.5954085711393,40.4304792649874));
#51012=CARTESIAN_POINT('Ctrl Pts',(20.4792436786066,11.5996352320654,40.4157265390742));
#51013=CARTESIAN_POINT('Ctrl Pts',(20.5562242246053,11.6038618929915,40.3970862092795));
#51014=CARTESIAN_POINT('Ctrl Pts',(20.6331561780845,11.6080858859175,40.3784576458419));
#51015=CARTESIAN_POINT('Ctrl Pts',(20.7092074237692,11.6123098788435,40.355946459429));
#51016=CARTESIAN_POINT('Ctrl Pts',(20.7839623199025,11.6165338717695,40.3296621990501));
#51017=CARTESIAN_POINT('Ctrl Pts',(20.8586933039937,11.620756513556,40.3033863462857));
#51018=CARTESIAN_POINT('Ctrl Pts',(20.9321283200646,11.6249791553424,40.2733399716059));
#51019=CARTESIAN_POINT('Ctrl Pts',(21.0038677840611,11.6292017971289,40.2396821990717));
#51020=CARTESIAN_POINT('Ctrl Pts',(21.0756066367174,11.6334244029314,40.206024713358));
#51021=CARTESIAN_POINT('Ctrl Pts',(21.1456495422488,11.6376470087339,40.1687560913823));
#51022=CARTESIAN_POINT('Ctrl Pts',(21.2136191351045,11.6418696145364,40.1280826008347));
#51023=CARTESIAN_POINT('Ctrl Pts',(21.2816563149963,11.6460964191784,40.0873686657211));
#51024=CARTESIAN_POINT('Ctrl Pts',(21.3476156608831,11.6503232238203,40.0432433403453));
#51025=CARTESIAN_POINT('Ctrl Pts',(21.4111471023474,11.6545500284623,39.9959573561757));
#51026=CARTESIAN_POINT('Ctrl Pts',(21.474709330035,11.6587788813398,39.9486484580467));
#51027=CARTESIAN_POINT('Ctrl Pts',(21.5358409475857,11.6630077342172,39.8981761488354));
#51028=CARTESIAN_POINT('Ctrl Pts',(21.5942254311096,11.6672365870947,39.8448311424615));
#51029=CARTESIAN_POINT('Ctrl Pts',(21.6527148443447,11.6714730401474,39.7913902634212));
#51030=CARTESIAN_POINT('Ctrl Pts',(21.708446928044,11.6757094932002,39.7350667053189));
#51031=CARTESIAN_POINT('Ctrl Pts',(21.7611426285269,11.679945946253,39.6761875151407));
#51032=CARTESIAN_POINT('Ctrl Pts',(21.8090362985402,11.6837963416871,39.6226738417441));
#51033=CARTESIAN_POINT('Ctrl Pts',(21.8544221080747,11.6876467371212,39.567049728623));
#51034=CARTESIAN_POINT('Ctrl Pts',(21.8971215135095,11.6914971325553,39.5095816414381));
#51035=CARTESIAN_POINT('Ctrl Pts',(21.944115338705,11.6957347749328,39.446333799554));
#51036=CARTESIAN_POINT('Ctrl Pts',(21.9880310015187,11.6999724173103,39.3806145856531));
#51037=CARTESIAN_POINT('Ctrl Pts',(22.0285988592561,11.7042100596878,39.3127559973569));
#51038=CARTESIAN_POINT('Ctrl Pts',(22.069108378822,11.7084416081693,39.2449949923734));
#51039=CARTESIAN_POINT('Ctrl Pts',(22.106279415464,11.7126731566507,39.1751011216777));
#51040=CARTESIAN_POINT('Ctrl Pts',(22.1398840554303,11.7169047051322,39.1034374271548));
#51041=CARTESIAN_POINT('Ctrl Pts',(22.1734498811094,11.7211313660583,39.0318565061783));
#51042=CARTESIAN_POINT('Ctrl Pts',(22.2034572981561,11.7253580269844,38.9585102459841));
#51043=CARTESIAN_POINT('Ctrl Pts',(22.2297237760258,11.7295846879105,38.883787167237));
#51044=CARTESIAN_POINT('Ctrl Pts',(22.255973673676,11.7338086808365,38.8091112560258));
#51045=CARTESIAN_POINT('Ctrl Pts',(22.2784871642117,11.7380326737625,38.7330606924001));
#51046=CARTESIAN_POINT('Ctrl Pts',(22.2971298961696,11.7422566666885,38.6560437761758));
#51047=CARTESIAN_POINT('Ctrl Pts',(22.3157666648286,11.746479308475,38.5790514955519));
#51048=CARTESIAN_POINT('Ctrl Pts',(22.3305350234233,11.7507019502615,38.5010939314472));
#51049=CARTESIAN_POINT('Ctrl Pts',(22.3413509481727,11.7549245920479,38.4225928988535));
#51050=CARTESIAN_POINT('Ctrl Pts',(22.3521667807523,11.7591471978504,38.34409253522));
#51051=CARTESIAN_POINT('Ctrl Pts',(22.3590301838881,11.7633698036529,38.2650491768866));
#51052=CARTESIAN_POINT('Ctrl Pts',(22.3619087753822,11.7675924094553,38.1858916624153));
#51053=CARTESIAN_POINT('Ctrl Pts',(22.3647902292661,11.7718192140973,38.1066554359555));
#51054=CARTESIAN_POINT('Ctrl Pts',(22.3636789395533,11.7760460187393,38.0273052961667));
#51055=CARTESIAN_POINT('Ctrl Pts',(22.3585946809799,11.7802728233813,37.9482713878224));
#51056=CARTESIAN_POINT('Ctrl Pts',(22.3535079586638,11.7845016762587,37.8691991810309));
#51057=CARTESIAN_POINT('Ctrl Pts',(22.3444444858648,11.7887305291362,37.7904439772517));
#51058=CARTESIAN_POINT('Ctrl Pts',(22.3314758378677,11.7929593820136,37.7124295440325));
#51059=CARTESIAN_POINT('Ctrl Pts',(22.3184838823684,11.7971958350664,37.6342749017808));
#51060=CARTESIAN_POINT('Ctrl Pts',(22.3015728284014,11.8014322881192,37.5568641492687));
#51061=CARTESIAN_POINT('Ctrl Pts',(22.2808651262499,11.805668741172,37.4806093988788));
#51062=CARTESIAN_POINT('Ctrl Pts',(22.2620444664143,11.8095191366061,37.4113035576305));
#51063=CARTESIAN_POINT('Ctrl Pts',(22.2400883095329,11.8133695320402,37.3429526919254));
#51064=CARTESIAN_POINT('Ctrl Pts',(22.2151229973752,11.8172199274744,37.2758516229467));
#51065=CARTESIAN_POINT('Ctrl Pts',(22.1876468415941,11.8214575698519,37.2020019785807));
#51066=CARTESIAN_POINT('Ctrl Pts',(22.1564219787768,11.8256952122293,37.1293892492687));
#51067=CARTESIAN_POINT('Ctrl Pts',(22.1215801348679,11.8299328546068,37.0584203476288));
#51068=CARTESIAN_POINT('Ctrl Pts',(22.0867883948979,11.8341644030883,36.9875535020545));
#51069=CARTESIAN_POINT('Ctrl Pts',(22.0483902081382,11.8383959515697,36.9183262070084));
#51070=CARTESIAN_POINT('Ctrl Pts',(22.0065660571066,11.8426275000512,36.8511272685467));
#51071=CARTESIAN_POINT('Ctrl Pts',(21.9647902141243,11.8468541609773,36.7840059467146));
#51072=CARTESIAN_POINT('Ctrl Pts',(21.9195965170393,11.8510808219034,36.7189087216886));
#51073=CARTESIAN_POINT('Ctrl Pts',(21.8712115253835,11.8553074828295,36.6562001980289));
#51074=CARTESIAN_POINT('Ctrl Pts',(21.8228570758423,11.8595314757555,36.5935312579434));
#51075=CARTESIAN_POINT('Ctrl Pts',(21.7713156157961,11.8637554686815,36.5332483965298));
#51076=CARTESIAN_POINT('Ctrl Pts',(21.7168565224518,11.8679794616076,36.475686568973));
#51077=CARTESIAN_POINT('Ctrl Pts',(21.6624148490787,11.872202103394,36.418143153867));
#51078=CARTESIAN_POINT('Ctrl Pts',(21.6050577176351,11.8764247451805,36.3633193844847));
#51079=CARTESIAN_POINT('Ctrl Pts',(21.5450932379161,11.8806473869669,36.3115153545401));
#51080=CARTESIAN_POINT('Ctrl Pts',(21.485129269195,11.8848699927694,36.2597117660526));
#51081=CARTESIAN_POINT('Ctrl Pts',(21.4225583520407,11.8890925985719,36.2109281712106));
#51082=CARTESIAN_POINT('Ctrl Pts',(21.3577225984424,11.8933152043744,36.1654251664568));
#51083=CARTESIAN_POINT('Ctrl Pts',(21.2928223740089,11.8975420090164,36.1198769148051));
#51084=CARTESIAN_POINT('Ctrl Pts',(21.2256531991711,11.9017688136584,36.0776160392707));
#51085=CARTESIAN_POINT('Ctrl Pts',(21.156586672529,11.9059956183003,36.0388600945524));
#51086=CARTESIAN_POINT('Ctrl Pts',(21.0874866774581,11.9102244711778,36.0000853693824));
#51087=CARTESIAN_POINT('Ctrl Pts',(21.0164879193549,11.9144533240553,35.9648191673006));
#51088=CARTESIAN_POINT('Ctrl Pts',(20.9439848440504,11.9186821769327,35.9332321178532));
#51089=CARTESIAN_POINT('Ctrl Pts',(20.8713514648315,11.9229186299855,35.901588299556));
#51090=CARTESIAN_POINT('Ctrl Pts',(20.7972088060598,11.9271550830383,35.8736370115531));
#51091=CARTESIAN_POINT('Ctrl Pts',(20.7219692294953,11.931391536091,35.8494998616836));
#51092=CARTESIAN_POINT('Ctrl Pts',(20.6535860517611,11.9352419315252,35.8275622713238));
#51093=CARTESIAN_POINT('Ctrl Pts',(20.5842972096088,11.9390923269593,35.8087747749266));
#51094=CARTESIAN_POINT('Ctrl Pts',(20.5144187912874,11.9429427223935,35.7931918701222));
#51095=CARTESIAN_POINT('Ctrl Pts',(20.437512470413,11.947180364771,35.7760417412865));
#51096=CARTESIAN_POINT('Ctrl Pts',(20.3596032030523,11.9514180071485,35.7627095780923));
#51097=CARTESIAN_POINT('Ctrl Pts',(20.2811040381236,11.955655649526,35.7533063769102));
#51098=CARTESIAN_POINT('Ctrl Pts',(20.2027177580751,11.9598871980074,35.7439166979004));
#51099=CARTESIAN_POINT('Ctrl Pts',(20.1237437266959,11.9641187464889,35.7384448158167));
#51100=CARTESIAN_POINT('Ctrl Pts',(20.0446063438319,11.9683502949703,35.7369509706758));
#51101=CARTESIAN_POINT('Ctrl Pts',(19.9655603668302,11.9725769558964,35.7354588509674));
#51102=CARTESIAN_POINT('Ctrl Pts',(19.886351879607,11.9768036168225,35.7379356460951));
#51103=CARTESIAN_POINT('Ctrl Pts',(19.8074100615131,11.9810302777486,35.7443897698274));
#51104=CARTESIAN_POINT('Ctrl Pts',(19.7285180739549,11.9852542706746,35.7508398195158));
#51105=CARTESIAN_POINT('Ctrl Pts',(19.6498928874021,11.9894782636006,35.7612621764191));
#51106=CARTESIAN_POINT('Ctrl Pts',(19.5719621164874,11.9937022565267,35.7756131967381));
#51107=CARTESIAN_POINT('Ctrl Pts',(19.4940562734901,11.9979248983131,35.7899596265591));
#51108=CARTESIAN_POINT('Ctrl Pts',(19.4168448657247,12.0021475400996,35.8082321394577));
#51109=CARTESIAN_POINT('Ctrl Pts',(19.3407473471902,12.0063701818861,35.8303356237842));
#51110=CARTESIAN_POINT('Ctrl Pts',(19.2646504771337,12.0105927876886,35.852438919752));
#51111=CARTESIAN_POINT('Ctrl Pts',(19.1896679272032,12.0148153934911,35.8783729901076));
#51112=CARTESIAN_POINT('Ctrl Pts',(19.116204527019,12.0190379992936,35.9079927000947));
#51113=CARTESIAN_POINT('Ctrl Pts',(19.0426680769127,12.0232648039355,35.9376418630814));
#51114=CARTESIAN_POINT('Ctrl Pts',(18.9706542297579,12.0274916085775,35.9709838106444));
#51115=CARTESIAN_POINT('Ctrl Pts',(18.9005477594611,12.0317184132195,36.0078252435148));
#51116=CARTESIAN_POINT('Ctrl Pts',(18.8304073167971,12.035947266097,36.044684529098));
#51117=CARTESIAN_POINT('Ctrl Pts',(18.7621764962502,12.0401761189744,36.0850464392235));
#51118=CARTESIAN_POINT('Ctrl Pts',(18.696213144297,12.0444049718519,36.1286729657928));
#51119=CARTESIAN_POINT('Ctrl Pts',(18.6301312417454,12.0486414249047,36.1723778987906));
#51120=CARTESIAN_POINT('Ctrl Pts',(18.5663253286885,12.0528778779574,36.2193588929237));
#51121=CARTESIAN_POINT('Ctrl Pts',(18.5051218811585,12.0571143310102,36.2693362267448));
#51122=CARTESIAN_POINT('Ctrl Pts',(18.4494957543052,12.0609647264443,36.3147592482104));
#51123=CARTESIAN_POINT('Ctrl Pts',(18.3960191538544,12.0648151218784,36.3626567102708));
#51124=CARTESIAN_POINT('Ctrl Pts',(18.344909854166,12.0686655173126,36.4127931217355));
#51125=CARTESIAN_POINT('Ctrl Pts',(18.2893631618179,12.0728502103508,36.4672824581194));
#51126=CARTESIAN_POINT('Ctrl Pts',(18.2363912731082,12.0770349033891,36.5246348089381));
#51127=CARTESIAN_POINT('Ctrl Pts',(18.1863097270532,12.0812195964274,36.5845733159542));
#51128=CARTESIAN_POINT('Ctrl Pts',(18.1364025412697,12.0853897203425,36.6443031454198));
#51129=CARTESIAN_POINT('Ctrl Pts',(18.089365962541,12.0895598442576,36.7066008259692));
#51130=CARTESIAN_POINT('Ctrl Pts',(18.0454776458662,12.0937299681727,36.7711535799457));
#51131=CARTESIAN_POINT('Ctrl Pts',(18.0016311623586,12.0978961172374,36.8356448039671));
#51132=CARTESIAN_POINT('Ctrl Pts',(17.9609272596224,12.1020622663021,36.9023864408502));
#51133=CARTESIAN_POINT('Ctrl Pts',(17.9236031437762,12.1062284153669,36.971032978177));
#51134=CARTESIAN_POINT('Ctrl Pts',(17.8863021886088,12.1103919792172,37.0396369183689));
#51135=CARTESIAN_POINT('Ctrl Pts',(17.8523770889213,12.1145555430676,37.1101429896707));
#51136=CARTESIAN_POINT('Ctrl Pts',(17.8220206330937,12.118719106918,37.1821784932622));
#51137=CARTESIAN_POINT('Ctrl Pts',(17.7914112549676,12.1229173605274,37.2548141784179));
#51138=CARTESIAN_POINT('Ctrl Pts',(17.7644305105462,12.1271156141369,37.3290044660351));
#51139=CARTESIAN_POINT('Ctrl Pts',(17.7412271533729,12.1313138677463,37.4043451515011));
#51140=CARTESIAN_POINT('Ctrl Pts',(17.7182126026396,12.1354779600354,37.479072787463));
#51141=CARTESIAN_POINT('Ctrl Pts',(17.6989142830347,12.1396420523245,37.5549316847391));
#51142=CARTESIAN_POINT('Ctrl Pts',(17.6834270820676,12.1438061446135,37.6315126930192));
#51143=CARTESIAN_POINT('Ctrl Pts',(17.6677493005859,12.1480214788832,37.7090360825593));
#51144=CARTESIAN_POINT('Ctrl Pts',(17.6559771855541,12.1522368131528,37.7872989801367));
#51145=CARTESIAN_POINT('Ctrl Pts',(17.648155372092,12.1564521474225,37.8658690813235));
#51146=CARTESIAN_POINT('Ctrl Pts',(17.6403335586299,12.1606674816921,37.9444391825103));
#51147=CARTESIAN_POINT('Ctrl Pts',(17.6364620348551,12.1648828159617,38.02331597533));
#51148=CARTESIAN_POINT('Ctrl Pts',(17.636530903764,12.1690981502314,38.10206689074));
#51149=CARTESIAN_POINT('',(17.6365304462654,12.9628481502994,38.0985475986668));
#51150=CARTESIAN_POINT('Ctrl Pts',(17.6365309037646,12.1690981502717,38.1020668914937));
#51151=CARTESIAN_POINT('Ctrl Pts',(17.6366294876699,12.175132280472,38.21479656999));
#51152=CARTESIAN_POINT('Ctrl Pts',(17.6447967865786,12.1811664106723,38.3271841533755));
#51153=CARTESIAN_POINT('Ctrl Pts',(17.660866537229,12.1872005408726,38.4382973311233));
#51154=CARTESIAN_POINT('Ctrl Pts',(17.6672472245105,12.1895964646589,38.4824161513517));
#51155=CARTESIAN_POINT('Ctrl Pts',(17.6748733071161,12.1919923884453,38.5263343998155));
#51156=CARTESIAN_POINT('Ctrl Pts',(17.6837324628504,12.1943883122316,38.5699948268302));
#51157=CARTESIAN_POINT('Ctrl Pts',(17.6994015479786,12.1986259546091,38.6472165134263));
#51158=CARTESIAN_POINT('Ctrl Pts',(17.7189659915919,12.2028635969866,38.7237987115027));
#51159=CARTESIAN_POINT('Ctrl Pts',(17.7423588860591,12.2071012393641,38.7993189841149));
#51160=CARTESIAN_POINT('Ctrl Pts',(17.765718140626,12.2113327878455,38.8747306556113));
#51161=CARTESIAN_POINT('Ctrl Pts',(17.7928947751503,12.215564336327,38.9490829902201));
#51162=CARTESIAN_POINT('Ctrl Pts',(17.8237709043756,12.2197958848084,39.0219638627723));
#51163=CARTESIAN_POINT('Ctrl Pts',(17.8546113708191,12.2240225457345,39.0947605559041));
#51164=CARTESIAN_POINT('Ctrl Pts',(17.8891426584629,12.2282492066606,39.1660887350197));
#51165=CARTESIAN_POINT('Ctrl Pts',(17.9271976045251,12.2324758675867,39.2355530239552));
#51166=CARTESIAN_POINT('Ctrl Pts',(17.9652285291196,12.2366998605127,39.3049734648668));
#51167=CARTESIAN_POINT('Ctrl Pts',(18.0067784726181,12.2409238534387,39.3725319408648));
#51168=CARTESIAN_POINT('Ctrl Pts',(18.0516333680824,12.2451478463648,39.4378557128965));
#51169=CARTESIAN_POINT('Ctrl Pts',(18.096473915695,12.2493704881512,39.5031585896441));
#51170=CARTESIAN_POINT('Ctrl Pts',(18.1446170507948,12.2535931299377,39.5662277957552));
#51171=CARTESIAN_POINT('Ctrl Pts',(18.1958050280076,12.2578157717241,39.6267190127648));
#51172=CARTESIAN_POINT('Ctrl Pts',(18.2469925690134,12.2620383775266,39.6872097142881));
#51173=CARTESIAN_POINT('Ctrl Pts',(18.3012245966393,12.2662609833291,39.7451221134685));
#51174=CARTESIAN_POINT('Ctrl Pts',(18.3582036398034,12.2704835891316,39.8001456268641));
#51175=CARTESIAN_POINT('Ctrl Pts',(18.4152393413126,12.2747103937736,39.8552238540815));
#51176=CARTESIAN_POINT('Ctrl Pts',(18.4750271766593,12.2789371984156,39.9074071310377));
#51177=CARTESIAN_POINT('Ctrl Pts',(18.5372338591295,12.2831640030576,39.9564228122986));
#51178=CARTESIAN_POINT('Ctrl Pts',(18.599470685868,12.287392855935,40.0054622456999));
#51179=CARTESIAN_POINT('Ctrl Pts',(18.6641283119256,12.2916217088125,40.0513307540042));
#51180=CARTESIAN_POINT('Ctrl Pts',(18.7308435903827,12.2958505616899,40.0937984975487));
#51181=CARTESIAN_POINT('Ctrl Pts',(18.7976787708152,12.3000870147427,40.1363425649347));
#51182=CARTESIAN_POINT('Ctrl Pts',(18.8665785841266,12.3043234677955,40.1754734233001));
#51183=CARTESIAN_POINT('Ctrl Pts',(18.937154568891,12.3085599208483,40.2110068759885));
#51184=CARTESIAN_POINT('Ctrl Pts',(19.0012991365544,12.3124103162824,40.2433022519283));
#51185=CARTESIAN_POINT('Ctrl Pts',(19.0668277772106,12.3162607117166,40.2726264897086));
#51186=CARTESIAN_POINT('Ctrl Pts',(19.133436707561,12.3201111071507,40.2988766452662));
#51187=CARTESIAN_POINT('Ctrl Pts',(19.2067447172969,12.3243487495282,40.3277668653774));
#51188=CARTESIAN_POINT('Ctrl Pts',(19.2816366628692,12.3285863919057,40.3530412991894));
#51189=CARTESIAN_POINT('Ctrl Pts',(19.3577217554161,12.3328240342832,40.3745261259072));
#51190=CARTESIAN_POINT('Ctrl Pts',(19.4336974346141,12.3370555827646,40.3959800566009));
#51191=CARTESIAN_POINT('Ctrl Pts',(19.5108624059776,12.3412871312461,40.4136550762709));
#51192=CARTESIAN_POINT('Ctrl Pts',(19.5888067819264,12.3455186797276,40.4274257406651));
#51193=CARTESIAN_POINT('Ctrl Pts',(19.6666611299686,12.3497453406537,40.4411804995616));
#51194=CARTESIAN_POINT('Ctrl Pts',(19.7452926343172,12.3539720015798,40.4510397838242));
#51195=CARTESIAN_POINT('Ctrl Pts',(19.8242786340817,12.3581986625059,40.4569286035983));
#51196=CARTESIAN_POINT('Ctrl Pts',(19.9032147754217,12.3624226554319,40.4628137061659));
#51197=CARTESIAN_POINT('Ctrl Pts',(19.9825045017686,12.3666466483579,40.4647332841742));
#51198=CARTESIAN_POINT('Ctrl Pts',(20.0617186101721,12.3708706412839,40.4626640163295));
#51199=CARTESIAN_POINT('Ctrl Pts',(20.1409073801535,12.3750932830704,40.460595410387));
#51200=CARTESIAN_POINT('Ctrl Pts',(20.2200201119486,12.3793159248569,40.4545405045538));
#51201=CARTESIAN_POINT('Ctrl Pts',(20.2986276679923,12.3835385666433,40.4445280882961));
#51202=CARTESIAN_POINT('Ctrl Pts',(20.3772345541679,12.3877611724458,40.434515757361));
#51203=CARTESIAN_POINT('Ctrl Pts',(20.4553358083166,12.3919837782483,40.4205460437042));
#51204=CARTESIAN_POINT('Ctrl Pts',(20.5325089679762,12.3962063840508,40.4026994245722));
#51205=CARTESIAN_POINT('Ctrl Pts',(20.6097588664379,12.4004331886928,40.3848350592681));
#51206=CARTESIAN_POINT('Ctrl Pts',(20.68607836919,12.4046599933347,40.3630861938033));
#51207=CARTESIAN_POINT('Ctrl Pts',(20.7610573430146,12.4088867979767,40.3375840010028));
#51208=CARTESIAN_POINT('Ctrl Pts',(20.8360726503362,12.4131156508542,40.3120694502865));
#51209=CARTESIAN_POINT('Ctrl Pts',(20.9097456984525,12.4173445037316,40.2827981222891));
#51210=CARTESIAN_POINT('Ctrl Pts',(20.9816860085487,12.4215733566091,40.2499495392961));
#51211=CARTESIAN_POINT('Ctrl Pts',(21.0537556111472,12.4258098096619,40.2170419202012));
#51212=CARTESIAN_POINT('Ctrl Pts',(21.1240858363615,12.4300462627146,40.1805444165595));
#51213=CARTESIAN_POINT('Ctrl Pts',(21.1923107142304,12.4342827157674,40.1406826312858));
#51214=CARTESIAN_POINT('Ctrl Pts',(21.2543184256263,12.4381331112015,40.104453353137));
#51215=CARTESIAN_POINT('Ctrl Pts',(21.3145871456284,12.4419835066356,40.0654457249484));
#51216=CARTESIAN_POINT('Ctrl Pts',(21.3728651577554,12.4458339020698,40.0238585445716));
#51217=CARTESIAN_POINT('Ctrl Pts',(21.4370043813992,12.4500715444472,39.9780888045694));
#51218=CARTESIAN_POINT('Ctrl Pts',(21.4989726316662,12.4543091868247,39.9290221511788));
#51219=CARTESIAN_POINT('Ctrl Pts',(21.5584113756626,12.4585468292022,39.8768917876746));
#51220=CARTESIAN_POINT('Ctrl Pts',(21.6177646444126,12.4627783776837,39.8248363896789));
#51221=CARTESIAN_POINT('Ctrl Pts',(21.6745952811693,12.4670099261651,39.7697263374953));
#51222=CARTESIAN_POINT('Ctrl Pts',(21.7285749384423,12.4712414746466,39.7118371887661));
#51223=CARTESIAN_POINT('Ctrl Pts',(21.7824922477204,12.4754681355727,39.6540149036023));
#51224=CARTESIAN_POINT('Ctrl Pts',(21.8335648033793,12.4796947964988,39.5934202419499));
#51225=CARTESIAN_POINT('Ctrl Pts',(21.8814996295203,12.4839214574249,39.5303669406887));
#51226=CARTESIAN_POINT('Ctrl Pts',(21.9294041977053,12.4881454503509,39.467353440636));
#51227=CARTESIAN_POINT('Ctrl Pts',(21.974174684751,12.4923694432769,39.4018847536659));
#51228=CARTESIAN_POINT('Ctrl Pts',(22.0155578967642,12.496593436203,39.3343082296134));
#51229=CARTESIAN_POINT('Ctrl Pts',(22.0569278714223,12.5008160779894,39.2667533214386));
#51230=CARTESIAN_POINT('Ctrl Pts',(22.09491247802,12.5050387197759,39.1970923145672));
#51231=CARTESIAN_POINT('Ctrl Pts',(22.1293022722832,12.5092613615623,39.1257008697226));
#51232=CARTESIAN_POINT('Ctrl Pts',(22.1636917734877,12.5134839673648,39.0543100332526));
#51233=CARTESIAN_POINT('Ctrl Pts',(22.1944863211164,12.5177065731673,38.9811892110775));
#51234=CARTESIAN_POINT('Ctrl Pts',(22.2215234635945,12.5219291789698,38.9067365998882));
#51235=CARTESIAN_POINT('Ctrl Pts',(22.2485874910406,12.5261559836118,38.8322099551331));
#51236=CARTESIAN_POINT('Ctrl Pts',(22.2718864897644,12.5303827882538,38.7563493177261));
#51237=CARTESIAN_POINT('Ctrl Pts',(22.2913072463144,12.5346095928957,38.6795701371597));
#51238=CARTESIAN_POINT('Ctrl Pts',(22.3107374138227,12.5388384457732,38.6027537507478));
#51239=CARTESIAN_POINT('Ctrl Pts',(22.3262855032581,12.5430672986506,38.5250183947225));
#51240=CARTESIAN_POINT('Ctrl Pts',(22.3378895585545,12.5472961515281,38.446789349464));
#51241=CARTESIAN_POINT('Ctrl Pts',(22.3495144688812,12.5515326045809,38.3684197094681));
#51242=CARTESIAN_POINT('Ctrl Pts',(22.357181136506,12.5557690576337,38.2895550750729));
#51243=CARTESIAN_POINT('Ctrl Pts',(22.3608796019484,12.5600055106864,38.2106252502993));
#51244=CARTESIAN_POINT('Ctrl Pts',(22.3642410352691,12.5638559061206,38.1388881076613));
#51245=CARTESIAN_POINT('Ctrl Pts',(22.3643252059902,12.5677063015547,38.0670973938957));
#51246=CARTESIAN_POINT('Ctrl Pts',(22.3611618609618,12.5715566969889,37.995572478534));
#51247=CARTESIAN_POINT('Ctrl Pts',(22.3576803679109,12.5757943393664,37.9168540669924));
#51248=CARTESIAN_POINT('Ctrl Pts',(22.3502514631331,12.5800319817439,37.8381621875518));
#51249=CARTESIAN_POINT('Ctrl Pts',(22.3388756111042,12.5842696241213,37.7599245426642));
#51250=CARTESIAN_POINT('Ctrl Pts',(22.3275161179968,12.5885011726028,37.6817994065802));
#51251=CARTESIAN_POINT('Ctrl Pts',(22.3122210162743,12.5927327210843,37.604127667903));
#51252=CARTESIAN_POINT('Ctrl Pts',(22.2930427311057,12.5969642695657,37.5273347625153));
#51253=CARTESIAN_POINT('Ctrl Pts',(22.273886597386,12.6011909304918,37.4506305550539));
#51254=CARTESIAN_POINT('Ctrl Pts',(22.2508563064176,12.6054175914179,37.374803616172));
#51255=CARTESIAN_POINT('Ctrl Pts',(22.2240555647086,12.609644252344,37.3002704919858));
#51256=CARTESIAN_POINT('Ctrl Pts',(22.197271740463,12.61386824527,37.2257844154303));
#51257=CARTESIAN_POINT('Ctrl Pts',(22.1667223477699,12.618092238196,37.1525909724864));
#51258=CARTESIAN_POINT('Ctrl Pts',(22.1325609447152,12.6223162311221,37.0810916341616));
#51259=CARTESIAN_POINT('Ctrl Pts',(22.098410468957,12.6265388729085,37.0096151665153));
#51260=CARTESIAN_POINT('Ctrl Pts',(22.0606504791455,12.630761514695,36.939832150056));
#51261=CARTESIAN_POINT('Ctrl Pts',(22.0194820969255,12.6349841564814,36.8721227662762));
#51262=CARTESIAN_POINT('Ctrl Pts',(21.9783140655291,12.6392067622839,36.8044139594937));
#51263=CARTESIAN_POINT('Ctrl Pts',(21.9337379442344,12.6434293680864,36.7387791500589));
#51264=CARTESIAN_POINT('Ctrl Pts',(21.8859993391751,12.6476519738889,36.6755713659396));
#51265=CARTESIAN_POINT('Ctrl Pts',(21.8382132642003,12.6518787785308,36.6123007297917));
#51266=CARTESIAN_POINT('Ctrl Pts',(21.7872587071196,12.6561055831728,36.5514623146082));
#51267=CARTESIAN_POINT('Ctrl Pts',(21.7334225489425,12.6603323878148,36.4933772354042));
#51268=CARTESIAN_POINT('Ctrl Pts',(21.6795603027065,12.6645612406922,36.4352640091885));
#51269=CARTESIAN_POINT('Ctrl Pts',(21.6228140096196,12.6687900935697,36.3799071046296));
#51270=CARTESIAN_POINT('Ctrl Pts',(21.5635066987201,12.6730189464471,36.3275899898846));
#51271=CARTESIAN_POINT('Ctrl Pts',(21.5040927995864,12.6772553994999,36.2751788498197));
#51272=CARTESIAN_POINT('Ctrl Pts',(21.442109053553,12.6814918525527,36.2258187082233));
#51273=CARTESIAN_POINT('Ctrl Pts',(21.3779105879832,12.6857283056055,36.1797518773805));
#51274=CARTESIAN_POINT('Ctrl Pts',(21.3195623717677,12.6895787010396,36.1378830043082));
#51275=CARTESIAN_POINT('Ctrl Pts',(21.2593852859931,12.6934290964738,36.0987341599395));
#51276=CARTESIAN_POINT('Ctrl Pts',(21.1976634316755,12.697279491908,36.0624542347895));
#51277=CARTESIAN_POINT('Ctrl Pts',(21.1297340072963,12.7015171342855,36.0225255181428));
#51278=CARTESIAN_POINT('Ctrl Pts',(21.0596781233794,12.705754776663,35.9859225996151));
#51279=CARTESIAN_POINT('Ctrl Pts',(20.9878548184795,12.7099924190405,35.952877903214));
#51280=CARTESIAN_POINT('Ctrl Pts',(20.9161347983107,12.7142239675219,35.9198807263831));
#51281=CARTESIAN_POINT('Ctrl Pts',(20.8426528269265,12.7184555160034,35.8904318043761));
#51282=CARTESIAN_POINT('Ctrl Pts',(20.767794325582,12.7226870644849,35.8647187392849));
#51283=CARTESIAN_POINT('Ctrl Pts',(20.6930222878737,12.726913725411,35.839035373494));
#51284=CARTESIAN_POINT('Ctrl Pts',(20.6168773209006,12.7311403863371,35.8170794411071));
#51285=CARTESIAN_POINT('Ctrl Pts',(20.5397653028354,12.7353670472632,35.7989906869474));
#51286=CARTESIAN_POINT('Ctrl Pts',(20.462701960279,12.7395910401892,35.7809133509729));
#51287=CARTESIAN_POINT('Ctrl Pts',(20.3846732334631,12.7438150331153,35.766698454722));
#51288=CARTESIAN_POINT('Ctrl Pts',(20.3060994905254,12.7480390260413,35.7564357182275));
#51289=CARTESIAN_POINT('Ctrl Pts',(20.2275508811745,12.7522616678277,35.746176264501));
#51290=CARTESIAN_POINT('Ctrl Pts',(20.1484580663881,12.7564843096142,35.7398665207724));
#51291=CARTESIAN_POINT('Ctrl Pts',(20.0692494457552,12.7607069514007,35.7375447189073));
#51292=CARTESIAN_POINT('Ctrl Pts',(19.9900415001122,12.7649295572032,35.7352229368279));
#51293=CARTESIAN_POINT('Ctrl Pts',(19.910718219198,12.7691521630057,35.7368890413476));
#51294=CARTESIAN_POINT('Ctrl Pts',(19.8317094388776,12.7733747688082,35.7425291671079));
#51295=CARTESIAN_POINT('Ctrl Pts',(19.7526220944659,12.7776015734501,35.7481749012493));
#51296=CARTESIAN_POINT('Ctrl Pts',(19.6738503439991,12.7818283780921,35.7578025166216));
#51297=CARTESIAN_POINT('Ctrl Pts',(19.5958197199819,12.7860551827341,35.7713461523566));
#51298=CARTESIAN_POINT('Ctrl Pts',(19.5177512836915,12.7902840356116,35.7848963511001));
#51299=CARTESIAN_POINT('Ctrl Pts',(19.4404251471274,12.794512888489,35.8023662470807));
#51300=CARTESIAN_POINT('Ctrl Pts',(19.3642549387221,12.7987417413665,35.8236391634979));
#51301=CARTESIAN_POINT('Ctrl Pts',(19.2879478357604,12.8029781944193,35.8449503120076));
#51302=CARTESIAN_POINT('Ctrl Pts',(19.2128012575486,12.8072146474721,35.8700779886578));
#51303=CARTESIAN_POINT('Ctrl Pts',(19.1392117804505,12.8114511005249,35.8988561878003));
#51304=CARTESIAN_POINT('Ctrl Pts',(19.0723283326503,12.8153014959589,35.9250118999488));
#51305=CARTESIAN_POINT('Ctrl Pts',(19.0067311100855,12.819151891393,35.9541823997606));
#51306=CARTESIAN_POINT('Ctrl Pts',(18.9426996584608,12.8230022868271,35.9862104104994));
#51307=CARTESIAN_POINT('Ctrl Pts',(18.8722283529694,12.8272399292046,36.0214595837071));
#51308=CARTESIAN_POINT('Ctrl Pts',(18.8033894442427,12.831477571582,36.060302924982));
#51309=CARTESIAN_POINT('Ctrl Pts',(18.7365733426896,12.8357152139595,36.1025657651633));
#51310=CARTESIAN_POINT('Ctrl Pts',(18.6698533253128,12.839946762441,36.1447678297219));
#51311=CARTESIAN_POINT('Ctrl Pts',(18.6051507312514,12.8441783109224,36.1903793792192));
#51312=CARTESIAN_POINT('Ctrl Pts',(18.5428327323031,12.8484098594038,36.2391792147408));
#51313=CARTESIAN_POINT('Ctrl Pts',(18.4805867123643,12.8526365203299,36.2879226851049));
#51314=CARTESIAN_POINT('Ctrl Pts',(18.4207201813142,12.856863181256,36.33984683577));
#51315=CARTESIAN_POINT('Ctrl Pts',(18.3635713004658,12.8610898421821,36.3946872567647));
#51316=CARTESIAN_POINT('Ctrl Pts',(18.3064584937719,12.8653138351081,36.4494930607767));
#51317=CARTESIAN_POINT('Ctrl Pts',(18.252060269619,12.8695378280341,36.5072111575306));
#51318=CARTESIAN_POINT('Ctrl Pts',(18.2006807125478,12.8737618209602,36.5675377516224));
#51319=CARTESIAN_POINT('Ctrl Pts',(18.1493175903886,12.8779844627466,36.6278450488903));
#51320=CARTESIAN_POINT('Ctrl Pts',(18.1009715215737,12.8822071045331,36.690758829947));
#51321=CARTESIAN_POINT('Ctrl Pts',(18.0559077706933,12.8864297463195,36.7559405352257));
#51322=CARTESIAN_POINT('Ctrl Pts',(18.0108444038316,12.890652352122,36.8211216850471));
#51323=CARTESIAN_POINT('Ctrl Pts',(17.9690635646959,12.8948749579245,36.8885703342577));
#51324=CARTESIAN_POINT('Ctrl Pts',(17.9307875970201,12.8990975637269,36.9579183600749));
#51325=CARTESIAN_POINT('Ctrl Pts',(17.8924735688071,12.9033243683689,37.0273353436029));
#51326=CARTESIAN_POINT('Ctrl Pts',(17.857671600695,12.9075511730109,37.0986550650328));
#51327=CARTESIAN_POINT('Ctrl Pts',(17.8265580765977,12.9117779776529,37.171484708528));
#51328=CARTESIAN_POINT('Ctrl Pts',(17.7954294754318,12.9160068305303,37.2443496439924));
#51329=CARTESIAN_POINT('Ctrl Pts',(17.7679930413479,12.9202356834078,37.3187255187517));
#51330=CARTESIAN_POINT('Ctrl Pts',(17.7443760506119,12.9244645362852,37.3942018419924));
#51331=CARTESIAN_POINT('Ctrl Pts',(17.7207166149682,12.928700989338,37.4698138127258));
#51332=CARTESIAN_POINT('Ctrl Pts',(17.7008904559355,12.9329374423907,37.5465297287325));
#51333=CARTESIAN_POINT('Ctrl Pts',(17.6849741873614,12.9371738954435,37.6239265521821));
#51334=CARTESIAN_POINT('Ctrl Pts',(17.6705083294649,12.9410242908777,37.6942703921629));
#51335=CARTESIAN_POINT('Ctrl Pts',(17.6592716173198,12.9448746863119,37.7651763155258));
#51336=CARTESIAN_POINT('Ctrl Pts',(17.6512842832292,12.9487250817461,37.8363242091241));
#51337=CARTESIAN_POINT('Ctrl Pts',(17.6415185618787,12.9534327712546,37.9233132464774));
#51338=CARTESIAN_POINT('Ctrl Pts',(17.6365843354261,12.9581404607632,38.0108546571211));
#51339=CARTESIAN_POINT('Ctrl Pts',(17.6365304462657,12.9628481502717,38.0985475981509));
#51340=CARTESIAN_POINT('',(17.6365301790272,13.7565981502284,38.0990800810601));
#51341=CARTESIAN_POINT('Ctrl Pts',(17.6365304462654,12.9628481502994,38.0985475986668));
#51342=CARTESIAN_POINT('Ctrl Pts',(17.6364826128399,12.9670268198915,38.1763861701059));
#51343=CARTESIAN_POINT('Ctrl Pts',(17.640284307832,12.9712054894835,38.2543759824577));
#51344=CARTESIAN_POINT('Ctrl Pts',(17.6479539514616,12.9753841590756,38.3320987428979));
#51345=CARTESIAN_POINT('Ctrl Pts',(17.6556128976047,12.9795570003315,38.4097130969743));
#51346=CARTESIAN_POINT('Ctrl Pts',(17.6671290306768,12.9837298415874,38.4870606623887));
#51347=CARTESIAN_POINT('Ctrl Pts',(17.6824687502264,12.9879026828433,38.5637233520351));
#51348=CARTESIAN_POINT('Ctrl Pts',(17.6977966391079,12.99207230582,38.6403269160354));
#51349=CARTESIAN_POINT('Ctrl Pts',(17.7169421724458,12.9962419287968,38.7162461806144));
#51350=CARTESIAN_POINT('Ctrl Pts',(17.7398201132759,13.0004115517735,38.7910696929744));
#51351=CARTESIAN_POINT('Ctrl Pts',(17.7626879857003,13.0045793397313,38.8658602760824));
#51352=CARTESIAN_POINT('Ctrl Pts',(17.7892848659156,13.008747127689,38.9395556029792));
#51353=CARTESIAN_POINT('Ctrl Pts',(17.8194751502271,13.0129149156468,39.0117575447579));
#51354=CARTESIAN_POINT('Ctrl Pts',(17.8496621445242,13.017082249416,39.0839516182627));
#51355=CARTESIAN_POINT('Ctrl Pts',(17.8834415781697,13.0212495831852,39.1546521852162));
#51356=CARTESIAN_POINT('Ctrl Pts',(17.9206296373,13.0254169169544,39.2234809013174));
#51357=CARTESIAN_POINT('Ctrl Pts',(17.9578512201433,13.0295880074267,39.2923716640587));
#51358=CARTESIAN_POINT('Ctrl Pts',(17.9984873370944,13.0337590978991,39.3593867795776));
#51359=CARTESIAN_POINT('Ctrl Pts',(18.0423084863937,13.0379301883715,39.4241730923312));
#51360=CARTESIAN_POINT('Ctrl Pts',(18.0861484987403,13.042103074312,39.4889872926984));
#51361=CARTESIAN_POINT('Ctrl Pts',(18.133175982708,13.0462759602526,39.5515703941878));
#51362=CARTESIAN_POINT('Ctrl Pts',(18.183120018302,13.0504488461931,39.6116009966275));
#51363=CARTESIAN_POINT('Ctrl Pts',(18.2331526724192,13.0546291363208,39.6717381147556));
#51364=CARTESIAN_POINT('Ctrl Pts',(18.2861118880157,13.0588094264485,39.7293133313685));
#51365=CARTESIAN_POINT('Ctrl Pts',(18.3416889378209,13.0629897165762,39.7840412292917));
#51366=CARTESIAN_POINT('Ctrl Pts',(18.3924677685148,13.0668091032726,39.8340442192421));
#51367=CARTESIAN_POINT('Ctrl Pts',(18.4454312783559,13.0706284899689,39.8816705988585));
#51368=CARTESIAN_POINT('Ctrl Pts',(18.5003215091152,13.0744478766652,39.9267333863697));
#51369=CARTESIAN_POINT('Ctrl Pts',(18.5612226920721,13.0786855190427,39.9767309365493));
#51370=CARTESIAN_POINT('Ctrl Pts',(18.6247412175117,13.0829231614202,40.0237734433076));
#51371=CARTESIAN_POINT('Ctrl Pts',(18.6905585163841,13.0871608037977,40.0675755238074));
#51372=CARTESIAN_POINT('Ctrl Pts',(18.756281167398,13.0913923522792,40.1113146151965));
#51373=CARTESIAN_POINT('Ctrl Pts',(18.8242956399514,13.0956239007607,40.1518222768073));
#51374=CARTESIAN_POINT('Ctrl Pts',(18.8942503390128,13.0998554492421,40.1888533045972));
#51375=CARTESIAN_POINT('Ctrl Pts',(18.9641242384648,13.1040821101682,40.2258415605273));
#51376=CARTESIAN_POINT('Ctrl Pts',(19.0359334987553,13.1083087710944,40.2593609444544));
#51377=CARTESIAN_POINT('Ctrl Pts',(19.1092988811206,13.1125354320205,40.2892103502695));
#51378=CARTESIAN_POINT('Ctrl Pts',(19.1826179529704,13.1167594249465,40.3190409142095));
#51379=CARTESIAN_POINT('Ctrl Pts',(19.2574907641177,13.1209834178725,40.3452059220412));
#51380=CARTESIAN_POINT('Ctrl Pts',(19.3335159898157,13.1252074107985,40.3675514338309));
#51381=CARTESIAN_POINT('Ctrl Pts',(19.409516897128,13.129430052585,40.3898897979039));
#51382=CARTESIAN_POINT('Ctrl Pts',(19.4866690375485,13.1336526943715,40.4084109599972));
#51383=CARTESIAN_POINT('Ctrl Pts',(19.5645551530859,13.1378753361579,40.4230105953689));
#51384=CARTESIAN_POINT('Ctrl Pts',(19.6424406049032,13.1420979419604,40.4376101063272));
#51385=CARTESIAN_POINT('Ctrl Pts',(19.7210595583898,13.1463205477629,40.4482880720475));
#51386=CARTESIAN_POINT('Ctrl Pts',(19.7999852427785,13.1505431535654,40.4549914092823));
#51387=CARTESIAN_POINT('Ctrl Pts',(19.8789894086302,13.1547699582074,40.4617014121257));
#51388=CARTESIAN_POINT('Ctrl Pts',(19.9583004464542,13.1589967628494,40.4644288520671));
#51389=CARTESIAN_POINT('Ctrl Pts',(20.0374877584534,13.1632235674913,40.4631726785968));
#51390=CARTESIAN_POINT('Ctrl Pts',(20.1167134432364,13.1674524203688,40.4619158964067));
#51391=CARTESIAN_POINT('Ctrl Pts',(20.1958148144115,13.1716812732463,40.4566716862937));
#51392=CARTESIAN_POINT('Ctrl Pts',(20.2743651388343,13.1759101261237,40.4474910460942));
#51393=CARTESIAN_POINT('Ctrl Pts',(20.3530566354036,13.1801465791765,40.4382939062724));
#51394=CARTESIAN_POINT('Ctrl Pts',(20.4311946430298,13.1843830322293,40.4251462785399));
#51395=CARTESIAN_POINT('Ctrl Pts',(20.5083616097451,13.1886194852821,40.408150539856));
#51396=CARTESIAN_POINT('Ctrl Pts',(20.5784965392721,13.1924698807161,40.3927035813244));
#51397=CARTESIAN_POINT('Ctrl Pts',(20.6478292455125,13.1963202761502,40.3740786111803));
#51398=CARTESIAN_POINT('Ctrl Pts',(20.7160591422646,13.2001706715843,40.3523875656022));
#51399=CARTESIAN_POINT('Ctrl Pts',(20.7911511443299,13.2044083139617,40.3285149801684));
#51400=CARTESIAN_POINT('Ctrl Pts',(20.8651889687577,13.2086459563392,40.3008382558305));
#51401=CARTESIAN_POINT('Ctrl Pts',(20.9377598086829,13.2128835987167,40.2694692858206));
#51402=CARTESIAN_POINT('Ctrl Pts',(21.0102262888923,13.2171151471982,40.2381454256207));
#51403=CARTESIAN_POINT('Ctrl Pts',(21.0812295472923,13.2213466956796,40.2031400485707));
#51404=CARTESIAN_POINT('Ctrl Pts',(21.1503725044909,13.225578244161,40.1646146230741));
#51405=CARTESIAN_POINT('Ctrl Pts',(21.2194355996647,13.2298049050871,40.1261336955077));
#51406=CARTESIAN_POINT('Ctrl Pts',(21.2866422562177,13.2340315660132,40.0841410261804));
#51407=CARTESIAN_POINT('Ctrl Pts',(21.35161733962,13.2382582269393,40.0388452769983));
#51408=CARTESIAN_POINT('Ctrl Pts',(21.4165514087248,13.2424822198654,39.9935781199046));
#51409=CARTESIAN_POINT('Ctrl Pts',(21.479256317124,13.2467062127914,39.9450122888448));
#51410=CARTESIAN_POINT('Ctrl Pts',(21.5393844742776,13.2509302057174,39.8934006471654));
#51411=CARTESIAN_POINT('Ctrl Pts',(21.5994933980818,13.2551528475038,39.8418055146355));
#51412=CARTESIAN_POINT('Ctrl Pts',(21.6570268519539,13.2593754892903,39.7871668112994));
#51413=CARTESIAN_POINT('Ctrl Pts',(21.711670192899,13.2635981310767,39.7297777736983));
#51414=CARTESIAN_POINT('Ctrl Pts',(21.7663130681914,13.2678207368792,39.6723892251479));
#51415=CARTESIAN_POINT('Ctrl Pts',(21.8180655573098,13.2720433426817,39.612250729413));
#51416=CARTESIAN_POINT('Ctrl Pts',(21.8666508239462,13.2762659484842,39.5496913955601));
#51417=CARTESIAN_POINT('Ctrl Pts',(21.9152844023945,13.2804927531261,39.4870698544791));
#51418=CARTESIAN_POINT('Ctrl Pts',(21.9607441792256,13.2847195577681,39.422023037956));
#51419=CARTESIAN_POINT('Ctrl Pts',(22.0027948835204,13.2889463624101,39.3549115886965));
#51420=CARTESIAN_POINT('Ctrl Pts',(22.0448659648496,13.2931752152875,39.2877676184046));
#51421=CARTESIAN_POINT('Ctrl Pts',(22.0835244538215,13.297404068165,39.2185574320744));
#51422=CARTESIAN_POINT('Ctrl Pts',(22.1185808448557,13.3016329210424,39.1476667622439));
#51423=CARTESIAN_POINT('Ctrl Pts',(22.1537002399067,13.3058693740952,39.0766486863448));
#51424=CARTESIAN_POINT('Ctrl Pts',(22.1852044149956,13.310105827148,39.0039445234467));
#51425=CARTESIAN_POINT('Ctrl Pts',(22.2129519624632,13.3143422802008,38.9299602717783));
#51426=CARTESIAN_POINT('Ctrl Pts',(22.2381709437073,13.318192675635,38.8627180242476));
#51427=CARTESIAN_POINT('Ctrl Pts',(22.2602873153771,13.3220430710692,38.7944188311924));
#51428=CARTESIAN_POINT('Ctrl Pts',(22.279231357355,13.3258934665034,38.7253757754739));
#51429=CARTESIAN_POINT('Ctrl Pts',(22.3000806639933,13.3301311088809,38.6493888323705));
#51430=CARTESIAN_POINT('Ctrl Pts',(22.3171649754614,13.3343687512583,38.5722154767498));
#51431=CARTESIAN_POINT('Ctrl Pts',(22.3303534499209,13.3386063936358,38.4942629063728));
#51432=CARTESIAN_POINT('Ctrl Pts',(22.3435229588367,13.3428379421173,38.4164224348513));
#51433=CARTESIAN_POINT('Ctrl Pts',(22.3528076789724,13.3470694905987,38.3378054322512));
#51434=CARTESIAN_POINT('Ctrl Pts',(22.3581269165168,13.3513010390802,38.2588328885931));
#51435=CARTESIAN_POINT('Ctrl Pts',(22.363440010195,13.3555277000063,38.1799515604037));
#51436=CARTESIAN_POINT('Ctrl Pts',(22.3647966920309,13.3597543609324,38.1007159725868));
#51437=CARTESIAN_POINT('Ctrl Pts',(22.3621678026812,13.3639810218585,38.0215543954304));
#51438=CARTESIAN_POINT('Ctrl Pts',(22.3595405727684,13.3682050147845,37.9424427875283));
#51439=CARTESIAN_POINT('Ctrl Pts',(22.3529327808065,13.3724290077105,37.8634055648463));
#51440=CARTESIAN_POINT('Ctrl Pts',(22.3423673397802,13.3766530006365,37.784871952326));
#51441=CARTESIAN_POINT('Ctrl Pts',(22.331805278349,13.380875642423,37.7063634605558));
#51442=CARTESIAN_POINT('Ctrl Pts',(22.3172881442246,13.3850982842095,37.6283587233051));
#51443=CARTESIAN_POINT('Ctrl Pts',(22.2988906526755,13.3893209259959,37.5512813034522));
#51444=CARTESIAN_POINT('Ctrl Pts',(22.2804933179039,13.3935435317984,37.4742045404281));
#51445=CARTESIAN_POINT('Ctrl Pts',(22.2582158016787,13.3977661376009,37.3980555347218));
#51446=CARTESIAN_POINT('Ctrl Pts',(22.2321834910903,13.4019887434034,37.3232456610973));
#51447=CARTESIAN_POINT('Ctrl Pts',(22.2061252947101,13.4062155480453,37.2483613986554));
#51448=CARTESIAN_POINT('Ctrl Pts',(22.1763050003823,13.4104423526873,37.1748193719255));
#51449=CARTESIAN_POINT('Ctrl Pts',(22.1428970732627,13.4146691573293,37.1030132526948));
#51450=CARTESIAN_POINT('Ctrl Pts',(22.1094729572469,13.4188980102067,37.0311723374768));
#51451=CARTESIAN_POINT('Ctrl Pts',(22.0724579642951,13.4231268630842,36.9610694205743));
#51452=CARTESIAN_POINT('Ctrl Pts',(22.0320725183102,13.4273557159616,36.8930734400021));
#51453=CARTESIAN_POINT('Ctrl Pts',(21.9916144908288,13.4315921690144,36.8249552557522));
#51454=CARTESIAN_POINT('Ctrl Pts',(21.9477741669369,13.4358286220672,36.7589519652903));
#51455=CARTESIAN_POINT('Ctrl Pts',(21.9008151521759,13.44006507512,36.6954031901793));
#51456=CARTESIAN_POINT('Ctrl Pts',(21.8581353977266,13.4439154705541,36.6376454597181));
#51457=CARTESIAN_POINT('Ctrl Pts',(21.8128801453055,13.4477658659883,36.5819150748636));
#51458=CARTESIAN_POINT('Ctrl Pts',(21.7652740788398,13.4516162614224,36.528440943688));
#51459=CARTESIAN_POINT('Ctrl Pts',(21.7128801135627,13.4558539037999,36.469588743117));
#51460=CARTESIAN_POINT('Ctrl Pts',(21.6574414846348,13.4600915461774,36.4132490684755));
#51461=CARTESIAN_POINT('Ctrl Pts',(21.5992285551981,13.4643291885549,36.3597533309502));
#51462=CARTESIAN_POINT('Ctrl Pts',(21.5410993382385,13.4685607370364,36.3063345223949));
#51463=CARTESIAN_POINT('Ctrl Pts',(21.4802040859639,13.4727922855178,36.255751843776));
#51464=CARTESIAN_POINT('Ctrl Pts',(21.4168520287486,13.4770238339993,36.2083021463429));
#51465=CARTESIAN_POINT('Ctrl Pts',(21.3535731449087,13.4812504949254,36.1609072546206));
#51466=CARTESIAN_POINT('Ctrl Pts',(21.2878434686099,13.4854771558515,36.1166384324546));
#51467=CARTESIAN_POINT('Ctrl Pts',(21.2200063894486,13.4897038167776,36.0757532634077));
#51468=CARTESIAN_POINT('Ctrl Pts',(21.1522121311656,13.4939278097036,36.0348939023535));
#51469=CARTESIAN_POINT('Ctrl Pts',(21.0823135108773,13.4981518026296,35.9974141963021));
#51470=CARTESIAN_POINT('Ctrl Pts',(21.0106830638267,13.5023757955557,35.9635285666797));
#51471=CARTESIAN_POINT('Ctrl Pts',(20.9390755293927,13.5065984373421,35.9296537761413));
#51472=CARTESIAN_POINT('Ctrl Pts',(20.8657376917039,13.5108210791286,35.8993709793767));
#51473=CARTESIAN_POINT('Ctrl Pts',(20.7910655341056,13.5150437209151,35.8728480604929));
#51474=CARTESIAN_POINT('Ctrl Pts',(20.7163940128394,13.5192663267175,35.8463253676289));
#51475=CARTESIAN_POINT('Ctrl Pts',(20.6403886364857,13.52348893252,35.8235626444933));
#51476=CARTESIAN_POINT('Ctrl Pts',(20.5634627466488,13.5277115383225,35.8046786338208));
#51477=CARTESIAN_POINT('Ctrl Pts',(20.4864603638877,13.5319383429645,35.7857758454233));
#51478=CARTESIAN_POINT('Ctrl Pts',(20.4085360955777,13.5361651476065,35.7707595856452));
#51479=CARTESIAN_POINT('Ctrl Pts',(20.3301151478045,13.5403919522485,35.7596977908633));
#51480=CARTESIAN_POINT('Ctrl Pts',(20.2516561986142,13.5446208051259,35.7486306357295));
#51481=CARTESIAN_POINT('Ctrl Pts',(20.1727005579758,13.5488496580034,35.7415218051048));
#51482=CARTESIAN_POINT('Ctrl Pts',(20.093677700594,13.5530785108808,35.7383872185916));
#51483=CARTESIAN_POINT('Ctrl Pts',(20.0145128218205,13.5573149639336,35.7352469985396));
#51484=CARTESIAN_POINT('Ctrl Pts',(19.9352809547857,13.5615514169864,35.7360952891515));
#51485=CARTESIAN_POINT('Ctrl Pts',(19.8564104868735,13.5657878700392,35.7408958283662));
#51486=CARTESIAN_POINT('Ctrl Pts',(19.7847272920522,13.5696382654733,35.7452589061681));
#51487=CARTESIAN_POINT('Ctrl Pts',(19.7133428366945,13.5734886609074,35.752886041988));
#51488=CARTESIAN_POINT('Ctrl Pts',(19.6425714478075,13.5773390563415,35.7637133585586));
#51489=CARTESIAN_POINT('Ctrl Pts',(19.5646823473772,13.581576698719,35.7756296139977));
#51490=CARTESIAN_POINT('Ctrl Pts',(19.4872436049088,13.5858143410965,35.7914675962248));
#51491=CARTESIAN_POINT('Ctrl Pts',(19.4106803987692,13.590051983474,35.8111809052472));
#51492=CARTESIAN_POINT('Ctrl Pts',(19.3342272935246,13.5942835319554,35.8308658657576));
#51493=CARTESIAN_POINT('Ctrl Pts',(19.2586476744575,13.5985150804369,35.8544149699349));
#51494=CARTESIAN_POINT('Ctrl Pts',(19.1843588855393,13.6027466289184,35.8817304011232));
#51495=CARTESIAN_POINT('Ctrl Pts',(19.1101559022238,13.6069732898445,35.9090142822341));
#51496=CARTESIAN_POINT('Ctrl Pts',(19.0372412239228,13.6111999507706,35.9400556844346));
#51497=CARTESIAN_POINT('Ctrl Pts',(18.9660178482963,13.6154266116967,35.9747067612073));
#51498=CARTESIAN_POINT('Ctrl Pts',(18.8948394310842,13.6196506046227,36.0093359651404));
#51499=CARTESIAN_POINT('Ctrl Pts',(18.825350617903,13.6238745975487,36.0475701164525));
#51500=CARTESIAN_POINT('Ctrl Pts',(18.7579340641067,13.6280985904747,36.0892134246038));
#51501=CARTESIAN_POINT('Ctrl Pts',(18.690539075018,13.6323212322612,36.1308434122023));
#51502=CARTESIAN_POINT('Ctrl Pts',(18.6252154275414,13.6365438740477,36.1758801449555));
#51503=CARTESIAN_POINT('Ctrl Pts',(18.5623195020174,13.6407665158341,36.2240828305545));
#51504=CARTESIAN_POINT('Ctrl Pts',(18.4994241124719,13.6449891216366,36.2722851053859));
#51505=CARTESIAN_POINT('Ctrl Pts',(18.4389567749458,13.6492117274391,36.3236529931348));
#51506=CARTESIAN_POINT('Ctrl Pts',(18.3812420953924,13.6534343332416,36.3779043908161));
#51507=CARTESIAN_POINT('Ctrl Pts',(18.3234700259979,13.6576611378836,36.4322097345491));
#51508=CARTESIAN_POINT('Ctrl Pts',(18.2684564244321,13.6618879425256,36.4894039938075));
#51509=CARTESIAN_POINT('Ctrl Pts',(18.2164897350997,13.6661147471676,36.5491674571717));
#51510=CARTESIAN_POINT('Ctrl Pts',(18.1644978636203,13.6703436000451,36.6089598808629));
#51511=CARTESIAN_POINT('Ctrl Pts',(18.1155561354708,13.6745724529225,36.6713236195836));
#51512=CARTESIAN_POINT('Ctrl Pts',(18.0699116834311,13.6788013058,36.7359070665294));
#51513=CARTESIAN_POINT('Ctrl Pts',(18.0241851983087,13.6830377588528,36.8006065840822));
#51514=CARTESIAN_POINT('Ctrl Pts',(17.9817680814153,13.6872742119055,36.867533383985));
#51515=CARTESIAN_POINT('Ctrl Pts',(17.9428631001573,13.6915106649583,36.9363083672185));
#51516=CARTESIAN_POINT('Ctrl Pts',(17.9075034348117,13.6953610603924,36.9988160542204));
#51517=CARTESIAN_POINT('Ctrl Pts',(17.8750444964466,13.6992114558265,37.0628498811227));
#51518=CARTESIAN_POINT('Ctrl Pts',(17.8456037998514,13.7030618512606,37.1281113985208));
#51519=CARTESIAN_POINT('Ctrl Pts',(17.8102375024772,13.7076872251708,37.2065082606305));
#51520=CARTESIAN_POINT('Ctrl Pts',(17.7791119595227,13.712312599081,37.2869312211764));
#51521=CARTESIAN_POINT('Ctrl Pts',(17.7524417551234,13.7169379729913,37.3689238228562));
#51522=CARTESIAN_POINT('Ctrl Pts',(17.7258416135051,13.7215511960175,37.4507010294978));
#51523=CARTESIAN_POINT('Ctrl Pts',(17.7036736021471,13.7261644190438,37.5340393592405));
#51524=CARTESIAN_POINT('Ctrl Pts',(17.6861045739136,13.73077764207,37.6184624645612));
#51525=CARTESIAN_POINT('Ctrl Pts',(17.6686127640987,13.7353705893142,37.7025145181311));
#51526=CARTESIAN_POINT('Ctrl Pts',(17.6556797311303,13.7399635365585,37.7876415314826));
#51527=CARTESIAN_POINT('Ctrl Pts',(17.6474222125353,13.7445564838027,37.8733544731799));
#51528=CARTESIAN_POINT('Ctrl Pts',(17.6402057652928,13.7485703726113,37.9482611070111));
#51529=CARTESIAN_POINT('Ctrl Pts',(17.636559551907,13.7525842614199,38.0236148285961));
#51530=CARTESIAN_POINT('Ctrl Pts',(17.6365301790272,13.7565981502284,38.0990800810601));
#51531=CARTESIAN_POINT('',(17.6365309503988,14.5503481503104,38.1021195464647));
#51532=CARTESIAN_POINT('Ctrl Pts',(17.6365301790269,13.7565981502717,38.0990800818733));
#51533=CARTESIAN_POINT('Ctrl Pts',(17.6364986455271,13.7609072978428,38.1800965038199));
#51534=CARTESIAN_POINT('Ctrl Pts',(17.6406371502407,13.765216445414,38.2610898530213));
#51535=CARTESIAN_POINT('Ctrl Pts',(17.6489123164394,13.7695255929851,38.34161362774));
#51536=CARTESIAN_POINT('Ctrl Pts',(17.6571923099408,13.7738372542894,38.4221843758518));
#51537=CARTESIAN_POINT('Ctrl Pts',(17.6696137192139,13.7781489155937,38.5022845658516));
#51538=CARTESIAN_POINT('Ctrl Pts',(17.6860915665036,13.782460576898,38.5814750276955));
#51539=CARTESIAN_POINT('Ctrl Pts',(17.7025966209716,13.7867793573445,38.6607962438168));
#51540=CARTESIAN_POINT('Ctrl Pts',(17.7231713963529,13.791098137791,38.7392042997413));
#51541=CARTESIAN_POINT('Ctrl Pts',(17.7476802625299,13.7954169182375,38.8162724628956));
#51542=CARTESIAN_POINT('Ctrl Pts',(17.7722111442425,13.7997395781072,38.893409853932));
#51543=CARTESIAN_POINT('Ctrl Pts',(17.8006830009683,13.8040622379769,38.9692045418666));
#51544=CARTESIAN_POINT('Ctrl Pts',(17.8329119001906,13.8083848978467,39.0432494943356));
#51545=CARTESIAN_POINT('Ctrl Pts',(17.8652070717965,13.812716446415,39.117446705666));
#51546=CARTESIAN_POINT('Ctrl Pts',(17.9012745212117,13.8170479949834,39.1898865993884));
#51547=CARTESIAN_POINT('Ctrl Pts',(17.9408842013788,13.8213795435518,39.2601864370733));
#51548=CARTESIAN_POINT('Ctrl Pts',(17.9634560939373,13.8238479110944,39.3002473609788));
#51549=CARTESIAN_POINT('Ctrl Pts',(17.9871774796518,13.826316278637,39.339613849284));
#51550=CARTESIAN_POINT('Ctrl Pts',(18.0119997541912,13.8287846461796,39.3782196460562));
#51551=CARTESIAN_POINT('Ctrl Pts',(18.0546141220591,13.8330222885571,39.4444972799964));
#51552=CARTESIAN_POINT('Ctrl Pts',(18.1006265355379,13.8372599309346,39.508765921821));
#51553=CARTESIAN_POINT('Ctrl Pts',(18.1498214031218,13.8414975733121,39.5706561802657));
#51554=CARTESIAN_POINT('Ctrl Pts',(18.1989455265555,13.8457291217936,39.63245743809));
#51555=CARTESIAN_POINT('Ctrl Pts',(18.2512427263197,13.849960670275,39.6918867408173));
#51556=CARTESIAN_POINT('Ctrl Pts',(18.3064536463111,13.8541922187565,39.7486027989807));
#51557=CARTESIAN_POINT('Ctrl Pts',(18.3616007961654,13.8584188796826,39.8052533485308));
#51558=CARTESIAN_POINT('Ctrl Pts',(18.4196546529653,13.8626455406087,39.8591965471098));
#51559=CARTESIAN_POINT('Ctrl Pts',(18.4803160154472,13.8668722015348,39.9101245890804));
#51560=CARTESIAN_POINT('Ctrl Pts',(18.5409390865866,13.8710961944608,39.9610204836839));
#51561=CARTESIAN_POINT('Ctrl Pts',(18.6041660383181,13.8753201873868,40.0089046988142));
#51562=CARTESIAN_POINT('Ctrl Pts',(18.6696621718654,13.8795441803128,40.0535075387452));
#51563=CARTESIAN_POINT('Ctrl Pts',(18.735137354995,13.8837668220993,40.0980961114502));
#51564=CARTESIAN_POINT('Ctrl Pts',(18.8028798913659,13.8879894638858,40.1394051296273));
#51565=CARTESIAN_POINT('Ctrl Pts',(18.8725246886765,13.8922121056722,40.1772072268447));
#51566=CARTESIAN_POINT('Ctrl Pts',(18.9421688924969,13.8964347114747,40.215009001925));
#51567=CARTESIAN_POINT('Ctrl Pts',(19.0137149123486,13.9006573172772,40.2493036930975));
#51568=CARTESIAN_POINT('Ctrl Pts',(19.0867728737301,13.9048799230797,40.2799097817903));
#51569=CARTESIAN_POINT('Ctrl Pts',(19.1599034818773,13.9091067277217,40.3105463043099));
#51570=CARTESIAN_POINT('Ctrl Pts',(19.234548601295,13.9133335323637,40.3374867162676));
#51571=CARTESIAN_POINT('Ctrl Pts',(19.3102987436765,13.9175603370057,40.3605978452449));
#51572=CARTESIAN_POINT('Ctrl Pts',(19.3860855932496,13.9217891898831,40.3837201734703));
#51573=CARTESIAN_POINT('Ctrl Pts',(19.4629780772484,13.9260180427606,40.4030094079282));
#51574=CARTESIAN_POINT('Ctrl Pts',(19.5405544091374,13.930246895638,40.4183830981822));
#51575=CARTESIAN_POINT('Ctrl Pts',(19.6182701626948,13.9344833486908,40.4337844183266));
#51576=CARTESIAN_POINT('Ctrl Pts',(19.6966717549177,13.9387198017436,40.445256065448));
#51577=CARTESIAN_POINT('Ctrl Pts',(19.7753303663308,13.9429562547963,40.4527673060902));
#51578=CARTESIAN_POINT('Ctrl Pts',(19.8468210106192,13.9468066502305,40.4595940657198));
#51579=CARTESIAN_POINT('Ctrl Pts',(19.9185236541111,13.9506570456646,40.4631499880943));
#51580=CARTESIAN_POINT('Ctrl Pts',(19.9901178623789,13.9545074410988,40.4634493403194));
#51581=CARTESIAN_POINT('Ctrl Pts',(20.0689125358425,13.9587450834763,40.4637787993832));
#51582=CARTESIAN_POINT('Ctrl Pts',(20.1478716078969,13.9629827258538,40.4601641823324));
#51583=CARTESIAN_POINT('Ctrl Pts',(20.2265678540668,13.9672203682312,40.4525852691037));
#51584=CARTESIAN_POINT('Ctrl Pts',(20.3051509319465,13.9714519167127,40.4450172546495));
#51585=CARTESIAN_POINT('Ctrl Pts',(20.3834714717638,13.9756834651942,40.4334963098714));
#51586=CARTESIAN_POINT('Ctrl Pts',(20.4611020001047,13.9799150136756,40.4180542242147));
#51587=CARTESIAN_POINT('Ctrl Pts',(20.5386428630417,13.9841416746017,40.4026299745933));
#51588=CARTESIAN_POINT('Ctrl Pts',(20.615494840868,13.9883683355278,40.3832936754001));
#51589=CARTESIAN_POINT('Ctrl Pts',(20.6912368595323,13.9925949964539,40.3601287673325));
#51590=CARTESIAN_POINT('Ctrl Pts',(20.7669310674742,13.99681898938,40.3369784816767));
#51591=CARTESIAN_POINT('Ctrl Pts',(20.841516259845,14.001042982306,40.3100045208452));
#51592=CARTESIAN_POINT('Ctrl Pts',(20.9145840092054,14.005266975232,40.2793408478267));
#51593=CARTESIAN_POINT('Ctrl Pts',(20.9876283861956,14.0094896170185,40.2486869832766));
#51594=CARTESIAN_POINT('Ctrl Pts',(21.0591558521197,14.0137122588049,40.2143459315276));
#51595=CARTESIAN_POINT('Ctrl Pts',(21.1287769439355,14.0179349005914,40.1765001930507));
#51596=CARTESIAN_POINT('Ctrl Pts',(21.198397442463,14.0221575063939,40.138654777083));
#51597=CARTESIAN_POINT('Ctrl Pts',(21.2661111880111,14.0263801121964,40.0973049589083));
#51598=CARTESIAN_POINT('Ctrl Pts',(21.3315536879893,14.0306027179988,40.0526789846009));
#51599=CARTESIAN_POINT('Ctrl Pts',(21.3970612621344,14.0348295226408,40.0080086354898));
#51600=CARTESIAN_POINT('Ctrl Pts',(21.4602926912241,14.0390563272828,39.9600558876579));
#51601=CARTESIAN_POINT('Ctrl Pts',(21.5209133621982,14.0432831319248,39.9090917570944));
#51602=CARTESIAN_POINT('Ctrl Pts',(21.5815634088872,14.0475119848022,39.8581029302063));
#51603=CARTESIAN_POINT('Ctrl Pts',(21.6395998335552,14.0517408376797,39.8041001333042));
#51604=CARTESIAN_POINT('Ctrl Pts',(21.6947238778059,14.0559696905572,39.7473923087396));
#51605=CARTESIAN_POINT('Ctrl Pts',(21.749946992044,14.0602061436099,39.6905825677875));
#51606=CARTESIAN_POINT('Ctrl Pts',(21.8022469573061,14.0644425966627,39.6310584383577));
#51607=CARTESIAN_POINT('Ctrl Pts',(21.8513645706152,14.0686790497155,39.5691629138971));
#51608=CARTESIAN_POINT('Ctrl Pts',(21.8960062157988,14.0725294451496,39.5129077773939));
#51609=CARTESIAN_POINT('Ctrl Pts',(21.9380194603227,14.0763798405837,39.454694368697));
#51610=CARTESIAN_POINT('Ctrl Pts',(21.9772418485556,14.0802302360178,39.3947992559546));
#51611=CARTESIAN_POINT('Ctrl Pts',(22.0204089614837,14.0844678783952,39.3288802945633));
#51612=CARTESIAN_POINT('Ctrl Pts',(22.0603570047894,14.0887055207727,39.2606765237577));
#51613=CARTESIAN_POINT('Ctrl Pts',(22.0968364630553,14.0929431631502,39.1905353218038));
#51614=CARTESIAN_POINT('Ctrl Pts',(22.1332634624287,14.0971747116316,39.1204949856508));
#51615=CARTESIAN_POINT('Ctrl Pts',(22.1662315678807,14.1014062601131,39.0485231637431));
#51616=CARTESIAN_POINT('Ctrl Pts',(22.1955347575789,14.1056378085945,38.9749957537971));
#51617=CARTESIAN_POINT('Ctrl Pts',(22.2248041012839,14.1098644695206,38.9015532700399));
#51618=CARTESIAN_POINT('Ctrl Pts',(22.2504167687586,14.1140911304467,38.8265592020938));
#51619=CARTESIAN_POINT('Ctrl Pts',(22.2722135501325,14.1183177913728,38.750412195069));
#51620=CARTESIAN_POINT('Ctrl Pts',(22.2939965726987,14.1225417842988,38.674313254408));
#51621=CARTESIAN_POINT('Ctrl Pts',(22.3119683615138,14.1267657772248,38.5970632687079));
#51622=CARTESIAN_POINT('Ctrl Pts',(22.3260189722204,14.1309897701509,38.5190777753241));
#51623=CARTESIAN_POINT('Ctrl Pts',(22.3400650885218,14.1352124119373,38.441117227362));
#51624=CARTESIAN_POINT('Ctrl Pts',(22.3501924344012,14.1394350537238,38.3624220999262));
#51625=CARTESIAN_POINT('Ctrl Pts',(22.3563421050171,14.1436576955102,38.2834184424301));
#51626=CARTESIAN_POINT('Ctrl Pts',(22.3624917232275,14.1478803013127,38.2044154581773));
#51627=CARTESIAN_POINT('Ctrl Pts',(22.3646636986166,14.1521029071152,38.1251044165617));
#51628=CARTESIAN_POINT('Ctrl Pts',(22.3628510931506,14.1563255129177,38.0459153210517));
#51629=CARTESIAN_POINT('Ctrl Pts',(22.3610366852811,14.1605523175597,37.9666474821502));
#51630=CARTESIAN_POINT('Ctrl Pts',(22.3552297928876,14.1647791222016,37.8875023013112));
#51631=CARTESIAN_POINT('Ctrl Pts',(22.3454756207214,14.1690059268436,37.8089079982177));
#51632=CARTESIAN_POINT('Ctrl Pts',(22.3357167218543,14.173234779721,37.7302756097021));
#51633=CARTESIAN_POINT('Ctrl Pts',(22.3220068139017,14.1774636325985,37.6521950930199));
#51634=CARTESIAN_POINT('Ctrl Pts',(22.3044424337787,14.1816924854759,37.5750852352049));
#51635=CARTESIAN_POINT('Ctrl Pts',(22.2868464866157,14.1859289385287,37.4978367940776));
#51636=CARTESIAN_POINT('Ctrl Pts',(22.2653823530887,14.1901653915815,37.4215629497883));
#51637=CARTESIAN_POINT('Ctrl Pts',(22.2401966658929,14.1944018446342,37.3466678428328));
#51638=CARTESIAN_POINT('Ctrl Pts',(22.2173060888518,14.1982522400685,37.2785977440324));
#51639=CARTESIAN_POINT('Ctrl Pts',(22.191342048871,14.2021026355027,37.2116665682194));
#51640=CARTESIAN_POINT('Ctrl Pts',(22.1624481196334,14.2059530309369,37.1461611400274));
#51641=CARTESIAN_POINT('Ctrl Pts',(22.1306482328213,14.2101906733143,37.0740676152958));
#51642=CARTESIAN_POINT('Ctrl Pts',(22.0951794394757,14.2144283156918,37.0034307607884));
#51643=CARTESIAN_POINT('Ctrl Pts',(22.0561973238576,14.2186659580693,36.9346489772344));
#51644=CARTESIAN_POINT('Ctrl Pts',(22.0172712660515,14.2228975065508,36.8659661045843));
#51645=CARTESIAN_POINT('Ctrl Pts',(21.9748421485907,14.2271290550322,36.7991334096114));
#51646=CARTESIAN_POINT('Ctrl Pts',(21.9291131548827,14.2313606035137,36.7345283318361));
#51647=CARTESIAN_POINT('Ctrl Pts',(21.8834369794253,14.2355872644398,36.6699978747097));
#51648=CARTESIAN_POINT('Ctrl Pts',(21.8344687714853,14.2398139253659,36.6076903023494));
#51649=CARTESIAN_POINT('Ctrl Pts',(21.7824562779356,14.244040586292,36.5479561674528));
#51650=CARTESIAN_POINT('Ctrl Pts',(21.7304766162926,14.248264579218,36.4882597386035));
#51651=CARTESIAN_POINT('Ctrl Pts',(21.6754567903276,14.252488572144,36.4311338755057));
#51652=CARTESIAN_POINT('Ctrl Pts',(21.6176855342393,14.25671256507,36.3768969986641));
#51653=CARTESIAN_POINT('Ctrl Pts',(21.5599327575922,14.2609352068565,36.3226774707126));
#51654=CARTESIAN_POINT('Ctrl Pts',(21.4994306400565,14.265157848643,36.2713454145448));
#51655=CARTESIAN_POINT('Ctrl Pts',(21.4365045166777,14.2693804904294,36.2231821573566));
#51656=CARTESIAN_POINT('Ctrl Pts',(21.3735789295349,14.2736030962319,36.1750193106));
#51657=CARTESIAN_POINT('Ctrl Pts',(21.3082297507391,14.2778257020344,36.1300254929143));
#51658=CARTESIAN_POINT('Ctrl Pts',(21.2408139196441,14.2820483078368,36.0884405905573));
#51659=CARTESIAN_POINT('Ctrl Pts',(21.1733310521579,14.2862751124788,36.0468143373523));
#51660=CARTESIAN_POINT('Ctrl Pts',(21.1037778273624,14.2905019171208,36.0086040171511));
#51661=CARTESIAN_POINT('Ctrl Pts',(21.0325380714226,14.2947287217628,35.9740048043415));
#51662=CARTESIAN_POINT('Ctrl Pts',(20.9612637939451,14.2989575746402,35.9393888253596));
#51663=CARTESIAN_POINT('Ctrl Pts',(20.8883017892339,14.3031864275177,35.9083876232862));
#51664=CARTESIAN_POINT('Ctrl Pts',(20.8140559126307,14.3074152803951,35.8811481770945));
#51665=CARTESIAN_POINT('Ctrl Pts',(20.7396765999173,14.3116517334479,35.8538597756489));
#51666=CARTESIAN_POINT('Ctrl Pts',(20.6640092536251,14.3158881865007,35.8303467780549));
#51667=CARTESIAN_POINT('Ctrl Pts',(20.5874727115031,14.3201246395535,35.8107061669285));
#51668=CARTESIAN_POINT('Ctrl Pts',(20.5179107575141,14.3239750349876,35.7928553567193));
#51669=CARTESIAN_POINT('Ctrl Pts',(20.4476312140241,14.3278254304218,35.7782027312014));
#51670=CARTESIAN_POINT('Ctrl Pts',(20.3769528411782,14.331675825856,35.7667839799051));
#51671=CARTESIAN_POINT('Ctrl Pts',(20.2991661117201,14.3359134682335,35.7542168072032));
#51672=CARTESIAN_POINT('Ctrl Pts',(20.2206042195142,14.340151110611,35.7455202786349));
#51673=CARTESIAN_POINT('Ctrl Pts',(20.1416860600604,14.3443887529885,35.7407807432787));
#51674=CARTESIAN_POINT('Ctrl Pts',(20.0628813880167,14.3486203014699,35.7360480235604));
#51675=CARTESIAN_POINT('Ctrl Pts',(19.9837219302221,14.3528518499514,35.7352610244925));
#51676=CARTESIAN_POINT('Ctrl Pts',(19.9046349084043,14.3570833984329,35.7384547558421));
#51677=CARTESIAN_POINT('Ctrl Pts',(19.8256392342808,14.361310059359,35.7416447983437));
#51678=CARTESIAN_POINT('Ctrl Pts',(19.7467162958905,14.3655367202851,35.748806415352));
#51679=CARTESIAN_POINT('Ctrl Pts',(19.668295017955,14.3697633812112,35.7599225983343));
#51680=CARTESIAN_POINT('Ctrl Pts',(19.589923241974,14.3739873741372,35.7710317644354));
#51681=CARTESIAN_POINT('Ctrl Pts',(19.5120529608245,14.3782113670632,35.7860904761207));
#51682=CARTESIAN_POINT('Ctrl Pts',(19.4351084554308,14.3824353599893,35.8050298512237));
#51683=CARTESIAN_POINT('Ctrl Pts',(19.3581885624752,14.3866580017757,35.8239631681398));
#51684=CARTESIAN_POINT('Ctrl Pts',(19.2821943120779,14.3908806435622,35.8467745715013));
#51685=CARTESIAN_POINT('Ctrl Pts',(19.2075387919301,14.3951032853487,35.8733442846717));
#51686=CARTESIAN_POINT('Ctrl Pts',(19.1328839079724,14.3993258911512,35.8999137714236));
#51687=CARTESIAN_POINT('Ctrl Pts',(19.0595681727386,14.4035484969537,35.9302413457806));
#51688=CARTESIAN_POINT('Ctrl Pts',(18.9879871138078,14.4077711027561,35.9641581615015));
#51689=CARTESIAN_POINT('Ctrl Pts',(18.9163348767012,14.4119979073981,35.9981087031424));
#51690=CARTESIAN_POINT('Ctrl Pts',(18.8464211860292,14.4162247120401,36.0356554141299));
#51691=CARTESIAN_POINT('Ctrl Pts',(18.7786186974788,14.4204515166821,36.0765825554889));
#51692=CARTESIAN_POINT('Ctrl Pts',(18.7107833530305,14.4246803695596,36.1175295294235));
#51693=CARTESIAN_POINT('Ctrl Pts',(18.6450616378687,14.4289092224371,36.1618599345387));
#51694=CARTESIAN_POINT('Ctrl Pts',(18.5817966807019,14.4331380753145,36.2093149955554));
#51695=CARTESIAN_POINT('Ctrl Pts',(18.5184180225433,14.4373745283673,36.2568553437159));
#51696=CARTESIAN_POINT('Ctrl Pts',(18.4575053058653,14.4416109814201,36.3075312679571));
#51697=CARTESIAN_POINT('Ctrl Pts',(18.3993678745093,14.4458474344729,36.3610442099504));
#51698=CARTESIAN_POINT('Ctrl Pts',(18.3465283652661,14.4496978299069,36.4096806482508));
#51699=CARTESIAN_POINT('Ctrl Pts',(18.2959811000384,14.453548225341,36.4606599346863));
#51700=CARTESIAN_POINT('Ctrl Pts',(18.2479295300893,14.4573986207751,36.513734098782));
#51701=CARTESIAN_POINT('Ctrl Pts',(18.1956152135631,14.4615905921446,36.5715165733777));
#51702=CARTESIAN_POINT('Ctrl Pts',(18.1460536011349,14.4657825635142,36.6320102148364));
#51703=CARTESIAN_POINT('Ctrl Pts',(18.0995425725386,14.4699745348837,36.694919216804));
#51704=CARTESIAN_POINT('Ctrl Pts',(18.0530930388454,14.4741609638071,36.7577450431658));
#51705=CARTESIAN_POINT('Ctrl Pts',(18.009686371673,14.4783473927304,36.8229795146034));
#51706=CARTESIAN_POINT('Ctrl Pts',(17.969582416137,14.4825338216538,36.8902914086276));
#51707=CARTESIAN_POINT('Ctrl Pts',(17.9295183415414,14.4867160874286,36.9575363650744));
#51708=CARTESIAN_POINT('Ctrl Pts',(17.8927507061616,14.4908983532035,37.0268542355731));
#51709=CARTESIAN_POINT('Ctrl Pts',(17.859496993302,14.4950806189784,37.0978835800083));
#51710=CARTESIAN_POINT('Ctrl Pts',(17.8262654562584,14.4992600957366,37.1688655572916));
#51711=CARTESIAN_POINT('Ctrl Pts',(17.7965433924196,14.5034395724949,37.2415563094894));
#51712=CARTESIAN_POINT('Ctrl Pts',(17.7705023263606,14.5076190492532,37.31556991125));
#51713=CARTESIAN_POINT('Ctrl Pts',(17.7444633363955,14.5117981928075,37.3895776123614));
#51714=CARTESIAN_POINT('Ctrl Pts',(17.7221049331247,14.5159773363619,37.4649075058114));
#51715=CARTESIAN_POINT('Ctrl Pts',(17.7035499709274,14.5201564799162,37.5411550260828));
#51716=CARTESIAN_POINT('Ctrl Pts',(17.6849958812562,14.524335426951,37.6173989609012));
#51717=CARTESIAN_POINT('Ctrl Pts',(17.6702449825026,14.5285143739858,37.6945599686642));
#51718=CARTESIAN_POINT('Ctrl Pts',(17.6593693564179,14.5326933210207,37.7722216736504));
#51719=CARTESIAN_POINT('Ctrl Pts',(17.6484862171153,14.536875155001,37.8499370297378));
#51720=CARTESIAN_POINT('Ctrl Pts',(17.6414837496195,14.5410569889813,37.928153296773));
#51721=CARTESIAN_POINT('Ctrl Pts',(17.6383822176429,14.5452388229617,38.0064484582978));
#51722=CARTESIAN_POINT('Ctrl Pts',(17.637119076311,14.546941932065,38.0383352340443));
#51723=CARTESIAN_POINT('Ctrl Pts',(17.6365023565896,14.5486450411684,38.0702350809376));
#51724=CARTESIAN_POINT('Ctrl Pts',(17.6365309503982,14.5503481502717,38.1021195457395));
#51725=CARTESIAN_POINT('',(17.6365301165987,15.3440981503131,38.0992576019166));
#51726=CARTESIAN_POINT('Ctrl Pts',(17.6365309503988,14.5503481503104,38.1021195464647));
#51727=CARTESIAN_POINT('Ctrl Pts',(17.6366226564826,14.5558103612077,38.2043793903881));
#51728=CARTESIAN_POINT('Ctrl Pts',(17.6433550821026,14.561272572105,38.3063458974693));
#51729=CARTESIAN_POINT('Ctrl Pts',(17.6565905908059,14.5667347830023,38.407282901901));
#51730=CARTESIAN_POINT('Ctrl Pts',(17.6698260995093,14.5721969938996,38.5082199063327));
#51731=CARTESIAN_POINT('Ctrl Pts',(17.6895645153101,14.5776592047969,38.6081277364946));
#51732=CARTESIAN_POINT('Ctrl Pts',(17.7156187406071,14.5831214156942,38.7062942376721));
#51733=CARTESIAN_POINT('Ctrl Pts',(17.7358318907963,14.5873590580717,38.7824528725667));
#51734=CARTESIAN_POINT('Ctrl Pts',(17.7598957095871,14.5915967004492,38.8577425341505));
#51735=CARTESIAN_POINT('Ctrl Pts',(17.787718398304,14.5958343428268,38.9317454873321));
#51736=CARTESIAN_POINT('Ctrl Pts',(17.8155010769026,14.6000658913082,39.0056420213629));
#51737=CARTESIAN_POINT('Ctrl Pts',(17.8470317271923,14.6042974397897,39.0782550864287));
#51738=CARTESIAN_POINT('Ctrl Pts',(17.8821682727408,14.6085289882712,39.1491802590186));
#51739=CARTESIAN_POINT('Ctrl Pts',(17.9172642346088,14.6127556491973,39.2200235110755));
#51740=CARTESIAN_POINT('Ctrl Pts',(17.9559576079721,14.6169823101235,39.2891823270005));
#51741=CARTESIAN_POINT('Ctrl Pts',(17.9980581168457,14.6212089710496,39.356271920156));
#51742=CARTESIAN_POINT('Ctrl Pts',(18.0401320505661,14.6254329639756,39.4233191642698));
#51743=CARTESIAN_POINT('Ctrl Pts',(18.0856086023958,14.6296569569017,39.4882993821646));
#51744=CARTESIAN_POINT('Ctrl Pts',(18.134252014581,14.6338809498277,39.5508531613519));
#51745=CARTESIAN_POINT('Ctrl Pts',(18.182879867072,14.6381035916142,39.6133869312999));
#51746=CARTESIAN_POINT('Ctrl Pts',(18.2346722807604,14.6423262334007,39.6734954340356));
#51747=CARTESIAN_POINT('Ctrl Pts',(18.2893515785705,14.6465488751871,39.7308502135882));
#51748=CARTESIAN_POINT('Ctrl Pts',(18.3440304104214,14.6507714809896,39.7882045043821));
#51749=CARTESIAN_POINT('Ctrl Pts',(18.4015957529806,14.6549940867921,39.842804780346));
#51750=CARTESIAN_POINT('Ctrl Pts',(18.4617322702618,14.6592166925946,39.894358613139));
#51751=CARTESIAN_POINT('Ctrl Pts',(18.5219285855909,14.6634434972366,39.9459637096018));
#51752=CARTESIAN_POINT('Ctrl Pts',(18.5847008259455,14.6676703018786,39.9945160060486));
#51753=CARTESIAN_POINT('Ctrl Pts',(18.6497001484648,14.6718971065206,40.0397630659037));
#51754=CARTESIAN_POINT('Ctrl Pts',(18.7147309685168,14.6761259593981,40.0850320516911));
#51755=CARTESIAN_POINT('Ctrl Pts',(18.7819906224036,14.6803548122755,40.1269923617539));
#51756=CARTESIAN_POINT('Ctrl Pts',(18.8511029935441,14.684583665153,40.1654360579443));
#51757=CARTESIAN_POINT('Ctrl Pts',(18.9203395747608,14.6888201182058,40.2039488458814));
#51758=CARTESIAN_POINT('Ctrl Pts',(18.9914351047638,14.6930565712586,40.2389321842645));
#51759=CARTESIAN_POINT('Ctrl Pts',(19.0639908989435,14.6972930243114,40.2702251965267));
#51760=CARTESIAN_POINT('Ctrl Pts',(19.1299348608219,14.7011434197453,40.2986665530167));
#51761=CARTESIAN_POINT('Ctrl Pts',(19.1970845759434,14.7049938151792,40.3240600448236));
#51762=CARTESIAN_POINT('Ctrl Pts',(19.2651306994886,14.7088442106131,40.3463208924964));
#51763=CARTESIAN_POINT('Ctrl Pts',(19.3400204456741,14.7130818529906,40.3708205868983));
#51764=CARTESIAN_POINT('Ctrl Pts',(19.4162772940511,14.7173194953681,40.3916170671704));
#51765=CARTESIAN_POINT('Ctrl Pts',(19.4935008509108,14.7215571377456,40.4085599521936));
#51766=CARTESIAN_POINT('Ctrl Pts',(19.5706133572652,14.725788686227,40.4254784726832));
#51767=CARTESIAN_POINT('Ctrl Pts',(19.6486893572643,14.7300202347085,40.4385543034406));
#51768=CARTESIAN_POINT('Ctrl Pts',(19.7273122558831,14.73425178319,40.4476864856936));
#51769=CARTESIAN_POINT('Ctrl Pts',(19.8058443428827,14.7384784441161,40.4568081200239));
#51770=CARTESIAN_POINT('Ctrl Pts',(19.8849216099028,14.7427051050422,40.4619951040148));
#51771=CARTESIAN_POINT('Ctrl Pts',(19.9641176979259,14.7469317659683,40.4631976009843));
#51772=CARTESIAN_POINT('Ctrl Pts',(20.0432637949103,14.7511557588943,40.4643993389002));
#51773=CARTESIAN_POINT('Ctrl Pts',(20.1225280965307,14.7553797518203,40.4616215749565));
#51774=CARTESIAN_POINT('Ctrl Pts',(20.2014807719779,14.7596037447464,40.4548664377037));
#51775=CARTESIAN_POINT('Ctrl Pts',(20.2804081926282,14.7638263865328,40.4481134612341));
#51776=CARTESIAN_POINT('Ctrl Pts',(20.3590237183212,14.7680490283193,40.437385677831));
#51777=CARTESIAN_POINT('Ctrl Pts',(20.4369006684905,14.7722716701057,40.422737231538));
#51778=CARTESIAN_POINT('Ctrl Pts',(20.5147769550178,14.7764942759082,40.4080889100742));
#51779=CARTESIAN_POINT('Ctrl Pts',(20.591914218106,14.7807168817107,40.3895200802112));
#51780=CARTESIAN_POINT('Ctrl Pts',(20.6678955005168,14.7849394875132,40.3671360879509));
#51781=CARTESIAN_POINT('Ctrl Pts',(20.7439523365607,14.7891662921552,40.3447298376834));
#51782=CARTESIAN_POINT('Ctrl Pts',(20.8188504451349,14.7933930967972,40.3185009798862));
#51783=CARTESIAN_POINT('Ctrl Pts',(20.892188177814,14.7976199014392,40.2886047373313));
#51784=CARTESIAN_POINT('Ctrl Pts',(20.9655614486734,14.8018487543166,40.2586940075811));
#51785=CARTESIAN_POINT('Ctrl Pts',(21.037372412157,14.8060776071941,40.2251125516116));
#51786=CARTESIAN_POINT('Ctrl Pts',(21.1072419020736,14.8103064600716,40.1880626933099));
#51787=CARTESIAN_POINT('Ctrl Pts',(21.1772369627748,14.8145429131244,40.1509462482937));
#51788=CARTESIAN_POINT('Ctrl Pts',(21.2452831745163,14.8187793661771,40.1103491865972));
#51789=CARTESIAN_POINT('Ctrl Pts',(21.3110285649619,14.8230158192299,40.0665183809855));
#51790=CARTESIAN_POINT('Ctrl Pts',(21.3707827385673,14.826866214664,40.0266817696272));
#51791=CARTESIAN_POINT('Ctrl Pts',(21.4286364916091,14.8307166100982,39.9841746299141));
#51792=CARTESIAN_POINT('Ctrl Pts',(21.4843503179773,14.8345670055323,39.9392103127214));
#51793=CARTESIAN_POINT('Ctrl Pts',(21.5456674672597,14.8388046479098,39.889723786137));
#51794=CARTESIAN_POINT('Ctrl Pts',(21.6046222725346,14.8430422902873,39.837074650806));
#51795=CARTESIAN_POINT('Ctrl Pts',(21.6608706354333,14.8472799326648,39.7815169262471));
#51796=CARTESIAN_POINT('Ctrl Pts',(21.7170381109788,14.8515114811462,39.7260390958763));
#51797=CARTESIAN_POINT('Ctrl Pts',(21.7705065424822,14.8557430296277,39.667661309361));
#51798=CARTESIAN_POINT('Ctrl Pts',(21.8209644714277,14.8599745781092,39.6066780793183));
#51799=CARTESIAN_POINT('Ctrl Pts',(21.8713641200717,14.8642012390353,39.5457652865903));
#51800=CARTESIAN_POINT('Ctrl Pts',(21.9187598789322,14.8684278999614,39.4822533900328));
#51801=CARTESIAN_POINT('Ctrl Pts',(21.9628778592699,14.8726545608875,39.4164729205297));
#51802=CARTESIAN_POINT('Ctrl Pts',(22.0069679909635,14.8768785538135,39.3507339737089));
#51803=CARTESIAN_POINT('Ctrl Pts',(22.0477841905145,14.8811025467395,39.2827296845934));
#51804=CARTESIAN_POINT('Ctrl Pts',(22.0850942713132,14.8853265396655,39.212821782963));
#51805=CARTESIAN_POINT('Ctrl Pts',(22.1223924176397,14.889549181452,39.1429362429542));
#51806=CARTESIAN_POINT('Ctrl Pts',(22.1561864517544,14.8937718232384,39.0711487128743));
#51807=CARTESIAN_POINT('Ctrl Pts',(22.1862895359481,14.8979944650249,38.9978465937474));
#51808=CARTESIAN_POINT('Ctrl Pts',(22.2163923636132,14.9022170708274,38.9245450992773));
#51809=CARTESIAN_POINT('Ctrl Pts',(22.2428041271381,14.9064396766298,38.8497294755966));
#51810=CARTESIAN_POINT('Ctrl Pts',(22.26538623323,14.9106622824323,38.7738068381903));
#51811=CARTESIAN_POINT('Ctrl Pts',(22.287990794328,14.9148890870743,38.6978087054656));
#51812=CARTESIAN_POINT('Ctrl Pts',(22.306757957336,14.9191158917163,38.6207018105602));
#51813=CARTESIAN_POINT('Ctrl Pts',(22.3215993020975,14.9233426963583,38.5429075765895));
#51814=CARTESIAN_POINT('Ctrl Pts',(22.3364478387147,14.9275715492357,38.4650756448961));
#51815=CARTESIAN_POINT('Ctrl Pts',(22.3473667026679,14.9318004021132,38.3865561755179));
#51816=CARTESIAN_POINT('Ctrl Pts',(22.3543192232785,14.9360292549906,38.3077773707634));
#51817=CARTESIAN_POINT('Ctrl Pts',(22.3612842390922,14.9402657080434,38.2288569832333));
#51818=CARTESIAN_POINT('Ctrl Pts',(22.3642686506542,14.9445021610962,38.1496767986011));
#51819=CARTESIAN_POINT('Ctrl Pts',(22.363287960477,14.9487386141489,38.0706664566691));
#51820=CARTESIAN_POINT('Ctrl Pts',(22.3623966382002,14.9525890095831,37.9988561342048));
#51821=CARTESIAN_POINT('Ctrl Pts',(22.3582306298081,14.9564394050172,37.9271863494851));
#51822=CARTESIAN_POINT('Ctrl Pts',(22.3508385367489,14.9602898004514,37.855974150885));
#51823=CARTESIAN_POINT('Ctrl Pts',(22.3427029965578,14.9645274428289,37.777599907059));
#51824=CARTESIAN_POINT('Ctrl Pts',(22.3306285386171,14.9687650852063,37.6994858367418));
#51825=CARTESIAN_POINT('Ctrl Pts',(22.3146409466993,14.9730027275838,37.6220588647513));
#51826=CARTESIAN_POINT('Ctrl Pts',(22.2986763455661,14.9772342760653,37.5447432357851));
#51827=CARTESIAN_POINT('Ctrl Pts',(22.278809879646,14.9814658245467,37.468113198217));
#51828=CARTESIAN_POINT('Ctrl Pts',(22.255119068091,14.9856973730282,37.3925903381828));
#51829=CARTESIAN_POINT('Ctrl Pts',(22.2314556200775,14.9899240339543,37.3171547091374));
#51830=CARTESIAN_POINT('Ctrl Pts',(22.2039767441644,14.9941506948804,37.2428241613066));
#51831=CARTESIAN_POINT('Ctrl Pts',(22.1728106246247,14.9983773558065,37.1700083707806));
#51832=CARTESIAN_POINT('Ctrl Pts',(22.1416641781108,15.0026013487325,37.0972385438506));
#51833=CARTESIAN_POINT('Ctrl Pts',(22.10683529178,15.0068253416585,37.0259820061797));
#51834=CARTESIAN_POINT('Ctrl Pts',(22.0685010215988,15.0110493345845,36.9566304339608));
#51835=CARTESIAN_POINT('Ctrl Pts',(22.0301790134999,15.015271976371,36.887301045409));
#51836=CARTESIAN_POINT('Ctrl Pts',(21.9883540747974,15.0194946181574,36.8198758222411));
#51837=CARTESIAN_POINT('Ctrl Pts',(21.9432494812504,15.0237172599439,36.7547223726977));
#51838=CARTESIAN_POINT('Ctrl Pts',(21.89814527207,15.0279398657464,36.6895694783708));
#51839=CARTESIAN_POINT('Ctrl Pts',(21.8497617316133,15.0321624715489,36.6266887037883));
#51840=CARTESIAN_POINT('Ctrl Pts',(21.7983649346115,15.0363850773513,36.5664179177952));
#51841=CARTESIAN_POINT('Ctrl Pts',(21.7469170300919,15.0406118819933,36.5060872002412));
#51842=CARTESIAN_POINT('Ctrl Pts',(21.6924501887901,15.0448386866353,36.4483720129164));
#51843=CARTESIAN_POINT('Ctrl Pts',(21.635269798666,15.0490654912773,36.3935759241997));
#51844=CARTESIAN_POINT('Ctrl Pts',(21.5780616999267,15.0532943441547,36.3387532822585));
#51845=CARTESIAN_POINT('Ctrl Pts',(21.518137787653,15.0575231970322,36.2868528641554));
#51846=CARTESIAN_POINT('Ctrl Pts',(21.4558373057294,15.0617520499096,36.2381385174652));
#51847=CARTESIAN_POINT('Ctrl Pts',(21.3934248561873,15.0659885029624,36.1893366204188));
#51848=CARTESIAN_POINT('Ctrl Pts',(21.3286276869489,15.0702249560152,36.1437325064659));
#51849=CARTESIAN_POINT('Ctrl Pts',(21.2618146474872,15.074461409068,36.1015470392609));
#51850=CARTESIAN_POINT('Ctrl Pts',(21.201090117112,15.0783118045021,36.0632058306388));
#51851=CARTESIAN_POINT('Ctrl Pts',(21.1387009512912,15.0821621999363,36.0276881497473));
#51852=CARTESIAN_POINT('Ctrl Pts',(21.0749395671253,15.0860125953705,35.9951258071019));
#51853=CARTESIAN_POINT('Ctrl Pts',(21.0047654906677,15.0902502377479,35.9592885624698));
#51854=CARTESIAN_POINT('Ctrl Pts',(20.9326655724501,15.0944878801254,35.9268971699541));
#51855=CARTESIAN_POINT('Ctrl Pts',(20.8590119808882,15.0987255225029,35.8981623907312));
#51856=CARTESIAN_POINT('Ctrl Pts',(20.7854643060815,15.1029570709844,35.8694689332485));
#51857=CARTESIAN_POINT('Ctrl Pts',(20.7103678280376,15.1071886194658,35.8444218154254));
#51858=CARTESIAN_POINT('Ctrl Pts',(20.63411839813,15.1114201679473,35.8231854932707));
#51859=CARTESIAN_POINT('Ctrl Pts',(20.5579570384195,15.1156468288734,35.8019736996545));
#51860=CARTESIAN_POINT('Ctrl Pts',(20.4806458225512,15.1198734897995,35.7845640798067));
#51861=CARTESIAN_POINT('Ctrl Pts',(20.4025981897729,15.1241001507256,35.7710721053473));
#51862=CARTESIAN_POINT('Ctrl Pts',(20.3245998230925,15.1283241436516,35.7575886474425));
#51863=CARTESIAN_POINT('Ctrl Pts',(20.2458664228906,15.1325481365776,35.7480180060565));
#51864=CARTESIAN_POINT('Ctrl Pts',(20.1668229314838,15.1367721295036,35.742424857946));
#51865=CARTESIAN_POINT('Ctrl Pts',(20.0878047239234,15.1409947712901,35.7368334989302));
#51866=CARTESIAN_POINT('Ctrl Pts',(20.0084770893962,15.1452174130766,35.7352171397353));
#51867=CARTESIAN_POINT('Ctrl Pts',(19.9292699394693,15.149440054863,35.7375885837904));
#51868=CARTESIAN_POINT('Ctrl Pts',(19.8500634645198,15.1536626606655,35.7399600076369));
#51869=CARTESIAN_POINT('Ctrl Pts',(19.7709779406491,15.157885266468,35.7463191517079));
#51870=CARTESIAN_POINT('Ctrl Pts',(19.69244162901,15.1621078722705,35.7566267285526));
#51871=CARTESIAN_POINT('Ctrl Pts',(19.6138272230891,15.1663346769124,35.7669445549595));
#51872=CARTESIAN_POINT('Ctrl Pts',(19.5357635861472,15.1705614815544,35.7812185956183));
#51873=CARTESIAN_POINT('Ctrl Pts',(19.4586716053749,15.1747882861964,35.7993579135223));
#51874=CARTESIAN_POINT('Ctrl Pts',(19.3815422671796,15.1790171390739,35.8175060214219));
#51875=CARTESIAN_POINT('Ctrl Pts',(19.305385974045,15.1832459919513,35.839523007534));
#51876=CARTESIAN_POINT('Ctrl Pts',(19.2306087216496,15.1874748448287,35.8652679127693));
#51877=CARTESIAN_POINT('Ctrl Pts',(19.1556970781451,15.1917112978815,35.891059087241));
#51878=CARTESIAN_POINT('Ctrl Pts',(19.0821698635692,15.1959477509343,35.9205913927295));
#51879=CARTESIAN_POINT('Ctrl Pts',(19.0104131311567,15.2001842039871,35.9536756373016));
#51880=CARTESIAN_POINT('Ctrl Pts',(18.9451954144938,15.2040345994212,35.9837449954783));
#51881=CARTESIAN_POINT('Ctrl Pts',(18.8814401435087,15.2078849948554,36.0167477088419));
#51882=CARTESIAN_POINT('Ctrl Pts',(18.8194170627884,15.2117353902896,36.0525102273113));
#51883=CARTESIAN_POINT('Ctrl Pts',(18.751156116676,15.2159730326671,36.0918694999842));
#51884=CARTESIAN_POINT('Ctrl Pts',(18.6847374801201,15.2202106750446,36.1347199986297));
#51885=CARTESIAN_POINT('Ctrl Pts',(18.6205405383324,15.2244483174221,36.1808642480231));
#51886=CARTESIAN_POINT('Ctrl Pts',(18.5564359142663,15.2286798659035,36.2269421401751));
#51887=CARTESIAN_POINT('Ctrl Pts',(18.4945470177231,15.232911414385,36.2763041053966));
#51888=CARTESIAN_POINT('Ctrl Pts',(18.4352272814854,15.2371429628664,36.3287075960496));
#51889=CARTESIAN_POINT('Ctrl Pts',(18.3759760611813,15.2413696237925,36.3810505592237));
#51890=CARTESIAN_POINT('Ctrl Pts',(18.3192884536529,15.2455962847187,36.4364277577356));
#51891=CARTESIAN_POINT('Ctrl Pts',(18.2654863739721,15.2498229456448,36.494555226106));
#51892=CARTESIAN_POINT('Ctrl Pts',(18.2117182558406,15.2540469385708,36.5526460026069));
#51893=CARTESIAN_POINT('Ctrl Pts',(18.1608323678019,15.2582709314968,36.6134832599616));
#51894=CARTESIAN_POINT('Ctrl Pts',(18.1131142762925,15.2624949244228,36.6767457336903));
#51895=CARTESIAN_POINT('Ctrl Pts',(18.0654114484926,15.2667175662093,36.7399879714877));
#51896=CARTESIAN_POINT('Ctrl Pts',(18.0208746871121,15.2709402079958,36.8056535111753));
#51897=CARTESIAN_POINT('Ctrl Pts',(17.9797487486737,15.2751628497822,36.8733886832356));
#51898=CARTESIAN_POINT('Ctrl Pts',(17.9386231606971,15.2793854555847,36.9411232780789));
#51899=CARTESIAN_POINT('Ctrl Pts',(17.9009085799361,15.2836080613872,37.0109270687873));
#51900=CARTESIAN_POINT('Ctrl Pts',(17.8668051671834,15.2878306671897,37.0824194154051));
#51901=CARTESIAN_POINT('Ctrl Pts',(17.8326678429639,15.2920574718317,37.1539828519856));
#51902=CARTESIAN_POINT('Ctrl Pts',(17.8021490617755,15.2962842764737,37.2272377743056));
#51903=CARTESIAN_POINT('Ctrl Pts',(17.775401643363,15.3005110811156,37.3017816134991));
#51904=CARTESIAN_POINT('Ctrl Pts',(17.7486412636203,15.3047399339931,37.3763615753309));
#51905=CARTESIAN_POINT('Ctrl Pts',(17.7256560234111,15.3089687868706,37.4522312490748));
#51906=CARTESIAN_POINT('Ctrl Pts',(17.7065486745972,15.313197639748,37.5289733290746));
#51907=CARTESIAN_POINT('Ctrl Pts',(17.6874069856903,15.3174340928008,37.6058533314093));
#51908=CARTESIAN_POINT('Ctrl Pts',(17.672157204191,15.3216705458536,37.6836084117256));
#51909=CARTESIAN_POINT('Ctrl Pts',(17.6608507656111,15.3259069989063,37.7618117385863));
#51910=CARTESIAN_POINT('Ctrl Pts',(17.6505746551618,15.3297573943404,37.8328885872905));
#51911=CARTESIAN_POINT('Ctrl Pts',(17.6435553024465,15.3336077897745,37.9043353671689));
#51912=CARTESIAN_POINT('Ctrl Pts',(17.6397939534902,15.3374581852086,37.9758313287551));
#51913=CARTESIAN_POINT('Ctrl Pts',(17.6376318183635,15.3396715068963,38.0169293315632));
#51914=CARTESIAN_POINT('Ctrl Pts',(17.6365430497082,15.341884828584,38.0580842963015));
#51915=CARTESIAN_POINT('Ctrl Pts',(17.6365301165989,15.3440981502717,38.0992576011458));
#51916=CARTESIAN_POINT('',(17.636530500807,16.137848150243,38.0984614018017));
#51917=CARTESIAN_POINT('Ctrl Pts',(17.6365301165987,15.3440981503131,38.0992576019166));
#51918=CARTESIAN_POINT('Ctrl Pts',(17.6365055556943,15.3483014116799,38.1774487489868));
#51919=CARTESIAN_POINT('Ctrl Pts',(17.6403654742914,15.3525046730467,38.2557956400634));
#51920=CARTESIAN_POINT('Ctrl Pts',(17.6481300745053,15.3567079344135,38.3338766650466));
#51921=CARTESIAN_POINT('Ctrl Pts',(17.6558838071005,15.3609053127418,38.4118484049693));
#51922=CARTESIAN_POINT('Ctrl Pts',(17.6675313256336,15.3651026910701,38.4895545467128));
#51923=CARTESIAN_POINT('Ctrl Pts',(17.6830408144045,15.3693000693984,38.566573223819));
#51924=CARTESIAN_POINT('Ctrl Pts',(17.6985335795304,15.3734929217578,38.6435088528609));
#51925=CARTESIAN_POINT('Ctrl Pts',(17.7178799495353,15.3776857741171,38.7197580242518));
#51926=CARTESIAN_POINT('Ctrl Pts',(17.7409964574754,15.3818786264764,38.7949053430225));
#51927=CARTESIAN_POINT('Ctrl Pts',(17.7640997835948,15.3860690879284,38.8700098102308));
#51928=CARTESIAN_POINT('Ctrl Pts',(17.7909688421192,15.3902595493804,38.9440132164779));
#51929=CARTESIAN_POINT('Ctrl Pts',(17.8214696921664,15.3944500108324,39.0165130325044));
#51930=CARTESIAN_POINT('Ctrl Pts',(17.8519630306406,15.3986394402817,39.0889949936954));
#51931=CARTESIAN_POINT('Ctrl Pts',(17.8860861997453,15.4028288697311,39.1599736603698));
#51932=CARTESIAN_POINT('Ctrl Pts',(17.9236568444375,15.4070182991805,39.2290657825161));
#51933=CARTESIAN_POINT('Ctrl Pts',(17.9612304077784,15.4112080540827,39.2981632720344));
#51934=CARTESIAN_POINT('Ctrl Pts',(18.0022517483518,15.4153978089849,39.3653735081291));
#51935=CARTESIAN_POINT('Ctrl Pts',(18.0464929897183,15.4195875638871,39.4303386041457));
#51936=CARTESIAN_POINT('Ctrl Pts',(18.0907799873747,15.423781652023,39.4953708899986));
#51937=CARTESIAN_POINT('Ctrl Pts',(18.1382932624232,15.4279757401589,39.558153007021));
#51938=CARTESIAN_POINT('Ctrl Pts',(18.1887625663253,15.4321698282949,39.6183574677116));
#51939=CARTESIAN_POINT('Ctrl Pts',(18.2392613895006,15.4363663695345,39.6785971417255));
#51940=CARTESIAN_POINT('Ctrl Pts',(18.2927193568771,15.440562910774,39.7362558104875));
#51941=CARTESIAN_POINT('Ctrl Pts',(18.3488288009787,15.4447594520136,39.7910423153849));
#51942=CARTESIAN_POINT('Ctrl Pts',(18.405030866315,15.4489629205867,39.845919257709));
#51943=CARTESIAN_POINT('Ctrl Pts',(18.4638927850808,15.4531663891597,39.8979142602253));
#51944=CARTESIAN_POINT('Ctrl Pts',(18.5250737735749,15.4573698577328,39.9467763988917));
#51945=CARTESIAN_POINT('Ctrl Pts',(18.5532671735569,15.4593068985311,39.9692930311545));
#51946=CARTESIAN_POINT('Ctrl Pts',(18.5819526347241,15.4612439393293,39.991144991887));
#51947=CARTESIAN_POINT('Ctrl Pts',(18.6110949153144,15.4631809801276,40.0123109335656));
#51948=CARTESIAN_POINT('Ctrl Pts',(18.6748491549338,15.4674186225051,40.0586154262208));
#51949=CARTESIAN_POINT('Ctrl Pts',(18.7410412070984,15.4716562648826,40.1018151107839));
#51950=CARTESIAN_POINT('Ctrl Pts',(18.8093361667405,15.4758939072601,40.1416439643258));
#51951=CARTESIAN_POINT('Ctrl Pts',(18.8775329155506,15.4801254557416,40.1814155424132));
#51952=CARTESIAN_POINT('Ctrl Pts',(18.9478261647317,15.484357004223,40.2178256817351));
#51953=CARTESIAN_POINT('Ctrl Pts',(19.0198504197545,15.4885885527045,40.250650422836));
#51954=CARTESIAN_POINT('Ctrl Pts',(19.0917914847737,15.4928152136306,40.2834372504544));
#51955=CARTESIAN_POINT('Ctrl Pts',(19.1654591580007,15.4970418745567,40.3126467161055));
#51956=CARTESIAN_POINT('Ctrl Pts',(19.2404629602685,15.5012685354828,40.3381005174424));
#51957=CARTESIAN_POINT('Ctrl Pts',(19.315419417799,15.5054925284089,40.3635382515468));
#51958=CARTESIAN_POINT('Ctrl Pts',(19.3917098875559,15.5097165213349,40.3852248766461));
#51959=CARTESIAN_POINT('Ctrl Pts',(19.4689246353764,15.5139405142609,40.4030304813419));
#51960=CARTESIAN_POINT('Ctrl Pts',(19.5461146843157,15.5181631560474,40.4208303905128));
#51961=CARTESIAN_POINT('Ctrl Pts',(19.6242279677574,15.5223857978338,40.4347516392608));
#51962=CARTESIAN_POINT('Ctrl Pts',(19.7028417834731,15.5266084396203,40.4447147876129));
#51963=CARTESIAN_POINT('Ctrl Pts',(19.7814549292675,15.5308310454228,40.4546778510623));
#51964=CARTESIAN_POINT('Ctrl Pts',(19.8605681336227,15.5350536512253,40.4606828236603));
#51965=CARTESIAN_POINT('Ctrl Pts',(19.9397522317301,15.5392762570278,40.4627019802164));
#51966=CARTESIAN_POINT('Ctrl Pts',(20.0190150682599,15.5435030616698,40.4647231445645));
#51967=CARTESIAN_POINT('Ctrl Pts',(20.0983484696451,15.5477298663118,40.462750564019));
#51968=CARTESIAN_POINT('Ctrl Pts',(20.1773225311129,15.5519566709537,40.4568086814291));
#51969=CARTESIAN_POINT('Ctrl Pts',(20.256334862027,15.5561855238312,40.4508639195071));
#51970=CARTESIAN_POINT('Ctrl Pts',(20.3349870404514,15.5604143767087,40.4409460825169));
#51971=CARTESIAN_POINT('Ctrl Pts',(20.4128561007656,15.5646432295861,40.4271313415793));
#51972=CARTESIAN_POINT('Ctrl Pts',(20.4908651088454,15.5688796826389,40.4132917725249));
#51973=CARTESIAN_POINT('Ctrl Pts',(20.5680877286801,15.5731161356917,40.3955414109331));
#51974=CARTESIAN_POINT('Ctrl Pts',(20.6441132013823,15.5773525887445,40.3740071734067));
#51975=CARTESIAN_POINT('Ctrl Pts',(20.7132106584581,15.5812029841786,40.3544352983462));
#51976=CARTESIAN_POINT('Ctrl Pts',(20.7813191600196,15.5850533796127,40.3317384773659));
#51977=CARTESIAN_POINT('Ctrl Pts',(20.8481452737109,15.5889037750468,40.3060462451141));
#51978=CARTESIAN_POINT('Ctrl Pts',(20.9216923096317,15.5931414174243,40.277770060492));
#51979=CARTESIAN_POINT('Ctrl Pts',(20.993961810663,15.5973790598018,40.2457588165799));
#51980=CARTESIAN_POINT('Ctrl Pts',(21.0645483180642,15.6016167021793,40.2101486486517));
#51981=CARTESIAN_POINT('Ctrl Pts',(21.1350333192977,15.6058482506607,40.1745896895425));
#51982=CARTESIAN_POINT('Ctrl Pts',(21.2038397181442,15.6100797991422,40.1354422936695));
#51983=CARTESIAN_POINT('Ctrl Pts',(21.270580690617,15.6143113476237,40.092891153458));
#51984=CARTESIAN_POINT('Ctrl Pts',(21.3372445754236,15.6185380085498,40.0503891609886));
#51985=CARTESIAN_POINT('Ctrl Pts',(21.4018473814208,15.6227646694759,40.0044914876315));
#51986=CARTESIAN_POINT('Ctrl Pts',(21.4640269848645,15.626991330402,39.9554286374012));
#51987=CARTESIAN_POINT('Ctrl Pts',(21.5261673386048,15.631215323328,39.906396757171));
#51988=CARTESIAN_POINT('Ctrl Pts',(21.5858871588354,15.635439316254,39.8542039554113));
#51989=CARTESIAN_POINT('Ctrl Pts',(21.6428544342319,15.63966330918,39.7991232294405));
#51990=CARTESIAN_POINT('Ctrl Pts',(21.6998034873587,15.6438859509665,39.7440601222842));
#51991=CARTESIAN_POINT('Ctrl Pts',(21.7540014073151,15.648108592753,39.6861112509478));
#51992=CARTESIAN_POINT('Ctrl Pts',(21.8051514626409,15.6523312345394,39.6255879646305));
#51993=CARTESIAN_POINT('Ctrl Pts',(21.8563010820825,15.6565538403419,39.565065194073));
#51994=CARTESIAN_POINT('Ctrl Pts',(21.904402587041,15.6607764461444,39.5019684111127));
#51995=CARTESIAN_POINT('Ctrl Pts',(21.949199110099,15.6649990519469,39.4366425363908));
#51996=CARTESIAN_POINT('Ctrl Pts',(21.9940401775497,15.6692258565889,39.3712517034709));
#51997=CARTESIAN_POINT('Ctrl Pts',(22.0355694328128,15.6734526612309,39.3036277387348));
#51998=CARTESIAN_POINT('Ctrl Pts',(22.0735733677598,15.6776794658729,39.2341445804734));
#51999=CARTESIAN_POINT('Ctrl Pts',(22.1115957187478,15.6819083187503,39.164627751891));
#52000=CARTESIAN_POINT('Ctrl Pts',(22.1460891420403,15.6861371716278,39.0932503576331));
#52001=CARTESIAN_POINT('Ctrl Pts',(22.1768872999061,15.6903660245052,39.020408672497));
#52002=CARTESIAN_POINT('Ctrl Pts',(22.2077408088106,15.694602477558,38.9474360748902));
#52003=CARTESIAN_POINT('Ctrl Pts',(22.2348856215499,15.6988389306108,38.8729943695623));
#52004=CARTESIAN_POINT('Ctrl Pts',(22.2582046136914,15.7030753836636,38.7974972140468));
#52005=CARTESIAN_POINT('Ctrl Pts',(22.2793986030383,15.7069257790977,38.728879929903));
#52006=CARTESIAN_POINT('Ctrl Pts',(22.2974328529144,15.7107761745318,38.6593912293901));
#52007=CARTESIAN_POINT('Ctrl Pts',(22.3122563000806,15.7146265699659,38.5893477737126));
#52008=CARTESIAN_POINT('Ctrl Pts',(22.3285705901236,15.7188642123434,38.5122598171312));
#52009=CARTESIAN_POINT('Ctrl Pts',(22.3410562523573,15.7231018547209,38.43421041768));
#52010=CARTESIAN_POINT('Ctrl Pts',(22.3496067806518,15.7273394970983,38.3556138048215));
#52011=CARTESIAN_POINT('Ctrl Pts',(22.358145012951,15.7315710455798,38.2771302169765));
#52012=CARTESIAN_POINT('Ctrl Pts',(22.3627592990368,15.7358025940613,38.1981014406366));
#52013=CARTESIAN_POINT('Ctrl Pts',(22.3633940093584,15.7400341425427,38.1189525045558));
#52014=CARTESIAN_POINT('Ctrl Pts',(22.364027986572,15.7442608034688,38.0398949876819));
#52015=CARTESIAN_POINT('Ctrl Pts',(22.3606915187227,15.7484874643949,37.9607180532591));
#52016=CARTESIAN_POINT('Ctrl Pts',(22.3533808513365,15.7527141253211,37.8818509466842));
#52017=CARTESIAN_POINT('Ctrl Pts',(22.3460747986714,15.7569381182471,37.8030336234847));
#52018=CARTESIAN_POINT('Ctrl Pts',(22.3347995689948,15.7611621111731,37.7245262054935));
#52019=CARTESIAN_POINT('Ctrl Pts',(22.3196034453482,15.7653861040991,37.6467558083896));
#52020=CARTESIAN_POINT('Ctrl Pts',(22.3044121825251,15.7696087458856,37.5690102879042));
#52021=CARTESIAN_POINT('Ctrl Pts',(22.2853026061308,15.773831387672,37.4920017798888));
#52022=CARTESIAN_POINT('Ctrl Pts',(22.2623743754399,15.7780540294585,37.4161486811793));
#52023=CARTESIAN_POINT('Ctrl Pts',(22.239446340136,15.782276635261,37.3402962288652));
#52024=CARTESIAN_POINT('Ctrl Pts',(22.2126998522416,15.7864992410634,37.2655996145877));
#52025=CARTESIAN_POINT('Ctrl Pts',(22.1822844324412,15.7907218468659,37.192462068658));
#52026=CARTESIAN_POINT('Ctrl Pts',(22.1518387684096,15.7949486515079,37.1192517968258));
#52027=CARTESIAN_POINT('Ctrl Pts',(22.1177170654331,15.7991754561499,37.0476041239026));
#52028=CARTESIAN_POINT('Ctrl Pts',(22.0801167881635,15.8034022607919,36.9779017028351));
#52029=CARTESIAN_POINT('Ctrl Pts',(22.0424982904583,15.8076311136693,36.9081655051956));
#52030=CARTESIAN_POINT('Ctrl Pts',(22.0013981037828,15.8118599665468,36.8403768386156));
#52031=CARTESIAN_POINT('Ctrl Pts',(21.9570581066831,15.8160888194242,36.7748909448781));
#52032=CARTESIAN_POINT('Ctrl Pts',(21.912638420892,15.820325272477,36.7092873586391));
#52033=CARTESIAN_POINT('Ctrl Pts',(21.8649675731551,15.8245617255298,36.6459951898754));
#52034=CARTESIAN_POINT('Ctrl Pts',(21.8143288123796,15.8287981785825,36.5853378589701));
#52035=CARTESIAN_POINT('Ctrl Pts',(21.7683046381822,15.8326485740167,36.5302080824672));
#52036=CARTESIAN_POINT('Ctrl Pts',(21.7198295025753,15.8364989694508,36.4772545661008));
#52037=CARTESIAN_POINT('Ctrl Pts',(21.6691412468445,15.840349364885,36.4266925151119));
#52038=CARTESIAN_POINT('Ctrl Pts',(21.6133551063818,15.8445870072624,36.3710452722176));
#52039=CARTESIAN_POINT('Ctrl Pts',(21.5546783845076,15.8488246496399,36.3180863935836));
#52040=CARTESIAN_POINT('Ctrl Pts',(21.4934005898209,15.8530622920174,36.2681307035647));
#52041=CARTESIAN_POINT('Ctrl Pts',(21.4322109150079,15.8572938404988,36.2182468517885));
#52042=CARTESIAN_POINT('Ctrl Pts',(21.3684279558925,15.8615253889803,36.1713579058385));
#52043=CARTESIAN_POINT('Ctrl Pts',(21.3023779741795,15.8657569374617,36.1277418897943));
#52044=CARTESIAN_POINT('Ctrl Pts',(21.2364042820192,15.8699835983878,36.084176251453));
#52045=CARTESIAN_POINT('Ctrl Pts',(21.1681691600272,15.8742102593139,36.0438762875696));
#52046=CARTESIAN_POINT('Ctrl Pts',(21.0980306445605,15.87843692024,36.0070788011714));
#52047=CARTESIAN_POINT('Ctrl Pts',(21.0279364027105,15.882660913166,35.9703045424933));
#52048=CARTESIAN_POINT('Ctrl Pts',(20.9559415662199,15.886884906092,35.9370285901768));
#52049=CARTESIAN_POINT('Ctrl Pts',(20.8824307107632,15.891108899018,35.907442935383));
#52050=CARTESIAN_POINT('Ctrl Pts',(20.8089433694144,15.8953315408045,35.8778667442293));
#52051=CARTESIAN_POINT('Ctrl Pts',(20.7339414066413,15.8995541825909,35.8519786814036));
#52052=CARTESIAN_POINT('Ctrl Pts',(20.6578300500723,15.9037768243773,35.8299228942342));
#52053=CARTESIAN_POINT('Ctrl Pts',(20.5817193420994,15.9079994301798,35.8078672950171));
#52054=CARTESIAN_POINT('Ctrl Pts',(20.5044997097749,15.9122220359823,35.789644035625));
#52055=CARTESIAN_POINT('Ctrl Pts',(20.4265907993584,15.9164446417848,35.7753471805874));
#52056=CARTESIAN_POINT('Ctrl Pts',(20.34860441853,15.9206714464267,35.7610361091626));
#52057=CARTESIAN_POINT('Ctrl Pts',(20.269927852669,15.9248982510687,35.7506593257667));
#52058=CARTESIAN_POINT('Ctrl Pts',(20.1909895839562,15.9291250557107,35.7442594752986));
#52059=CARTESIAN_POINT('Ctrl Pts',(20.1120130631414,15.9333539085881,35.7378565235752));
#52060=CARTESIAN_POINT('Ctrl Pts',(20.0327750559952,15.9375827614656,35.7354343582328));
#52061=CARTESIAN_POINT('Ctrl Pts',(19.9537052264222,15.941811614343,35.7369834459235));
#52062=CARTESIAN_POINT('Ctrl Pts',(19.8744932910383,15.9460480673958,35.7385353176643));
#52063=CARTESIAN_POINT('Ctrl Pts',(19.7954506058933,15.9502845204486,35.7440726704425));
#52064=CARTESIAN_POINT('Ctrl Pts',(19.7170026603079,15.9545209735013,35.7535339451364));
#52065=CARTESIAN_POINT('Ctrl Pts',(19.6457034843836,15.9583713689355,35.7621330369779));
#52066=CARTESIAN_POINT('Ctrl Pts',(19.574895757171,15.9622217643697,35.7739727766214));
#52067=CARTESIAN_POINT('Ctrl Pts',(19.5048894728339,15.9660721598039,35.7889707905807));
#52068=CARTESIAN_POINT('Ctrl Pts',(19.4278424260391,15.9703098021814,35.8054772041732));
#52069=CARTESIAN_POINT('Ctrl Pts',(19.35147711472,15.9745474445589,35.8258718050086));
#52070=CARTESIAN_POINT('Ctrl Pts',(19.2762152246405,15.9787850869364,35.8500831037886));
#52071=CARTESIAN_POINT('Ctrl Pts',(19.2010615641123,15.9830166354179,35.8742595857708));
#52072=CARTESIAN_POINT('Ctrl Pts',(19.1270086162236,15.9872481838993,35.9022417235528));
#52073=CARTESIAN_POINT('Ctrl Pts',(19.0544672022013,15.9914797323808,35.9339071651504));
#52074=CARTESIAN_POINT('Ctrl Pts',(18.9820095755155,15.9957063933069,35.9655360322884));
#52075=CARTESIAN_POINT('Ctrl Pts',(18.9110604406773,15.999933054233,36.0008395622537));
#52076=CARTESIAN_POINT('Ctrl Pts',(18.8420133359816,16.0041597151591,36.0396463102527));
#52077=CARTESIAN_POINT('Ctrl Pts',(18.7730098159699,16.0083837080851,36.078428562223));
#52078=CARTESIAN_POINT('Ctrl Pts',(18.7059063505851,16.0126077010112,36.120709413885));
#52079=CARTESIAN_POINT('Ctrl Pts',(18.6410733331933,16.0168316939372,36.1662707647807));
#52080=CARTESIAN_POINT('Ctrl Pts',(18.5762610541068,16.0210543357236,36.2118175418492));
#52081=CARTESIAN_POINT('Ctrl Pts',(18.5137181640778,16.0252769775101,36.2606424650291));
#52082=CARTESIAN_POINT('Ctrl Pts',(18.453786163424,16.0294996192965,36.3124840665099));
#52083=CARTESIAN_POINT('Ctrl Pts',(18.3938546734911,16.033722225099,36.3643252262135));
#52084=CARTESIAN_POINT('Ctrl Pts',(18.3365343822978,16.0379448309015,36.4191827053458));
#52085=CARTESIAN_POINT('Ctrl Pts',(18.2821326258983,16.042167436704,36.4767556789267));
#52086=CARTESIAN_POINT('Ctrl Pts',(18.2276767739346,16.046394241346,36.5343859014403));
#52087=CARTESIAN_POINT('Ctrl Pts',(18.1761455764438,16.050621045988,36.5947366705696));
#52088=CARTESIAN_POINT('Ctrl Pts',(18.1278080449245,16.05484785063,36.657471759635));
#52089=CARTESIAN_POINT('Ctrl Pts',(18.0794470898843,16.0590767035074,36.7202372490254));
#52090=CARTESIAN_POINT('Ctrl Pts',(18.0342831512126,16.0633055563849,36.7853889742914));
#52091=CARTESIAN_POINT('Ctrl Pts',(17.9925421130222,16.0675344092623,36.8525613149695));
#52092=CARTESIAN_POINT('Ctrl Pts',(17.9507260570391,16.0717708623151,36.9198543790639));
#52093=CARTESIAN_POINT('Ctrl Pts',(17.9123454208389,16.0760073153679,36.9891749035545));
#52094=CARTESIAN_POINT('Ctrl Pts',(17.8775801734251,16.0802437684207,37.0601324504237));
#52095=CARTESIAN_POINT('Ctrl Pts',(17.8459829980898,16.0840941638548,37.1246238093691));
#52096=CARTESIAN_POINT('Ctrl Pts',(17.8173718101545,16.0879445592889,37.1904669076602));
#52097=CARTESIAN_POINT('Ctrl Pts',(17.7918462500092,16.0917949547231,37.2573568624254));
#52098=CARTESIAN_POINT('Ctrl Pts',(17.759851353345,16.0966212152764,37.3411997704125));
#52099=CARTESIAN_POINT('Ctrl Pts',(17.7326042815355,16.1014474758297,37.4269487816098));
#52100=CARTESIAN_POINT('Ctrl Pts',(17.7103056779464,16.1062737363831,37.5140901498903));
#52101=CARTESIAN_POINT('Ctrl Pts',(17.6880976991037,16.1110803823163,37.6008773630611));
#52102=CARTESIAN_POINT('Ctrl Pts',(17.6707981761703,16.1158870282495,37.6890454480439));
#52103=CARTESIAN_POINT('Ctrl Pts',(17.6585584633483,16.1206936741827,37.7780652685057));
#52104=CARTESIAN_POINT('Ctrl Pts',(17.6464027197852,16.1254673446285,37.8664743778784));
#52105=CARTESIAN_POINT('Ctrl Pts',(17.6392377111805,16.1302410150742,37.9557233688363));
#52106=CARTESIAN_POINT('Ctrl Pts',(17.6371636382762,16.13501468552,38.0452755208704));
#52107=CARTESIAN_POINT('Ctrl Pts',(17.6367532753299,16.135959173761,38.0629937432554));
#52108=CARTESIAN_POINT('Ctrl Pts',(17.6365420478448,16.136903662002,38.0807237808861));
#52109=CARTESIAN_POINT('Ctrl Pts',(17.636530500807,16.137848150243,38.0984614018017));
#52110=CARTESIAN_POINT('',(17.6365307541938,16.9315981503216,38.1018881282061));
#52111=CARTESIAN_POINT('Ctrl Pts',(17.6365305008067,16.1378481502717,38.0984614023413));
#52112=CARTESIAN_POINT('Ctrl Pts',(17.6364785885184,16.1420943096752,38.1782048682515));
#52113=CARTESIAN_POINT('Ctrl Pts',(17.6404668253251,16.1463404690787,38.2579711622715));
#52114=CARTESIAN_POINT('Ctrl Pts',(17.648475589581,16.1505866284822,38.3373254897886));
#52115=CARTESIAN_POINT('Ctrl Pts',(17.6564848530562,16.1548330525664,38.4166847637895));
#52116=CARTESIAN_POINT('Ctrl Pts',(17.6685150947909,16.1590794766506,38.495631561438));
#52117=CARTESIAN_POINT('Ctrl Pts',(17.6844948615814,16.1633259007348,38.5737366302674));
#52118=CARTESIAN_POINT('Ctrl Pts',(17.7004803878264,16.1675738553223,38.6518698498574));
#52119=CARTESIAN_POINT('Ctrl Pts',(17.7204181734841,16.1718218099098,38.7291602865282));
#52120=CARTESIAN_POINT('Ctrl Pts',(17.7441860494605,16.1760697644973,38.8051906561003));
#52121=CARTESIAN_POINT('Ctrl Pts',(17.767985373847,16.1803233397561,38.8813216250804));
#52122=CARTESIAN_POINT('Ctrl Pts',(17.7956247620737,16.184576915015,38.956188759763));
#52123=CARTESIAN_POINT('Ctrl Pts',(17.8269329028224,16.1888304902738,39.0293921842065));
#52124=CARTESIAN_POINT('Ctrl Pts',(17.8582656665114,16.1930874108456,39.1026531810099));
#52125=CARTESIAN_POINT('Ctrl Pts',(17.8932727228514,16.1973443314174,39.1742474499582));
#52126=CARTESIAN_POINT('Ctrl Pts',(17.9317366813445,16.2016012519892,39.243799495368));
#52127=CARTESIAN_POINT('Ctrl Pts',(17.9702674063473,16.205865561809,39.3134722706117));
#52128=CARTESIAN_POINT('Ctrl Pts',(18.0122667634631,16.2101298716289,39.3810953587803));
#52129=CARTESIAN_POINT('Ctrl Pts',(18.0574742721319,16.2143941814487,39.4463224864312));
#52130=CARTESIAN_POINT('Ctrl Pts',(18.0685123018993,16.2154353708465,39.4622485791945));
#52131=CARTESIAN_POINT('Ctrl Pts',(18.0797414043603,16.2164765602444,39.4780319944199));
#52132=CARTESIAN_POINT('Ctrl Pts',(18.0911574403174,16.2175177496422,39.4936680104115));
#52133=CARTESIAN_POINT('Ctrl Pts',(18.1376207234194,16.2217553920197,39.5573066184481));
#52134=CARTESIAN_POINT('Ctrl Pts',(18.1873571594556,16.2259930343972,39.6187385925859));
#52135=CARTESIAN_POINT('Ctrl Pts',(18.2401296669689,16.2302306767746,39.6776079525082));
#52136=CARTESIAN_POINT('Ctrl Pts',(18.2928262855455,16.2344622252561,39.7363926559807));
#52137=CARTESIAN_POINT('Ctrl Pts',(18.3485499948283,16.2386937737375,39.792621717413));
#52138=CARTESIAN_POINT('Ctrl Pts',(18.4070216891549,16.242925322219,39.8459697998755));
#52139=CARTESIAN_POINT('Ctrl Pts',(18.46542584706,16.247151983145,39.8992562638295));
#52140=CARTESIAN_POINT('Ctrl Pts',(18.5265713379303,16.2513786440711,39.9496680472584));
#52141=CARTESIAN_POINT('Ctrl Pts',(18.590141263079,16.2556053049972,39.9969155971807));
#52142=CARTESIAN_POINT('Ctrl Pts',(18.6536710609099,16.2598292979232,40.0441333229772));
#52143=CARTESIAN_POINT('Ctrl Pts',(18.7196218801348,16.2640532908492,40.0881905009103));
#52144=CARTESIAN_POINT('Ctrl Pts',(18.7876436429308,16.2682772837752,40.1288377225332));
#52145=CARTESIAN_POINT('Ctrl Pts',(18.8556436474293,16.2724999255617,40.1694719422241));
#52146=CARTESIAN_POINT('Ctrl Pts',(18.9257128779157,16.2767225673481,40.206698131335));
#52147=CARTESIAN_POINT('Ctrl Pts',(18.9974734222548,16.2809452091346,40.2403109357788));
#52148=CARTESIAN_POINT('Ctrl Pts',(19.069233355074,16.285167814937,40.2739234537854));
#52149=CARTESIAN_POINT('Ctrl Pts',(19.1426841479714,16.2893904207395,40.3039224508015));
#52150=CARTESIAN_POINT('Ctrl Pts',(19.2174258642835,16.293613026542,40.3301498073016));
#52151=CARTESIAN_POINT('Ctrl Pts',(19.2922419016392,16.297839831184,40.3564032435415));
#52152=CARTESIAN_POINT('Ctrl Pts',(19.3683509831628,16.3020666358259,40.3788773922223));
#52153=CARTESIAN_POINT('Ctrl Pts',(19.4453364548924,16.3062934404679,40.3974635563222));
#52154=CARTESIAN_POINT('Ctrl Pts',(19.5223592324327,16.3105222933453,40.4160587269516));
#52155=CARTESIAN_POINT('Ctrl Pts',(19.6002587849685,16.3147511462228,40.4307620726978));
#52156=CARTESIAN_POINT('Ctrl Pts',(19.6786091846356,16.3189799991002,40.4415162576201));
#52157=CARTESIAN_POINT('Ctrl Pts',(19.7571003971406,16.323216452153,40.4522897701695));
#52158=CARTESIAN_POINT('Ctrl Pts',(19.83604360763,16.3274529052057,40.4590999000014));
#52159=CARTESIAN_POINT('Ctrl Pts',(19.9150089292952,16.3316893582585,40.4619413538021));
#52160=CARTESIAN_POINT('Ctrl Pts',(19.9867783340819,16.3355397536927,40.4645238728587));
#52161=CARTESIAN_POINT('Ctrl Pts',(20.0585657317189,16.339390149127,40.4638287408858));
#52162=CARTESIAN_POINT('Ctrl Pts',(20.1300520943976,16.3432405445612,40.4598891697796));
#52163=CARTESIAN_POINT('Ctrl Pts',(20.208728075884,16.3474781869387,40.4555533830392));
#52164=CARTESIAN_POINT('Ctrl Pts',(20.2873346771541,16.3517158293162,40.4472707051577));
#52165=CARTESIAN_POINT('Ctrl Pts',(20.3654442259973,16.3559534716937,40.4350462433505));
#52166=CARTESIAN_POINT('Ctrl Pts',(20.443441450244,16.3601850201752,40.4228393607991));
#52167=CARTESIAN_POINT('Ctrl Pts',(20.5209425822431,16.3644165686567,40.4067020232024));
#52168=CARTESIAN_POINT('Ctrl Pts',(20.5975227802602,16.3686481171381,40.3866912708038));
#52169=CARTESIAN_POINT('Ctrl Pts',(20.6740145260339,16.3728747780642,40.3667036313768));
#52170=CARTESIAN_POINT('Ctrl Pts',(20.7495870004239,16.3771014389903,40.3428515858283));
#52171=CARTESIAN_POINT('Ctrl Pts',(20.8238248076045,16.3813280999164,40.3152433562197));
#52172=CARTESIAN_POINT('Ctrl Pts',(20.8980157535678,16.3855520928424,40.2876525537859));
#52173=CARTESIAN_POINT('Ctrl Pts',(20.9708732663339,16.3897760857684,40.2563104364766));
#52174=CARTESIAN_POINT('Ctrl Pts',(21.0419975654431,16.3940000786945,40.2213749113513));
#52175=CARTESIAN_POINT('Ctrl Pts',(21.1130991138386,16.3982227204809,40.1864505611429));
#52176=CARTESIAN_POINT('Ctrl Pts',(21.1824681290684,16.4024453622674,40.1479352921867));
#52177=CARTESIAN_POINT('Ctrl Pts',(21.249726635242,16.4066680040538,40.1060343411982));
#52178=CARTESIAN_POINT('Ctrl Pts',(21.3169845682606,16.4108906098563,40.064133747276));
#52179=CARTESIAN_POINT('Ctrl Pts',(21.3821316308602,16.4151132156588,40.0188477777724));
#52180=CARTESIAN_POINT('Ctrl Pts',(21.4448174819599,16.4193358214613,39.9704258565159));
#52181=CARTESIAN_POINT('Ctrl Pts',(21.5075656660929,16.4235626261033,39.9219557858735));
#52182=CARTESIAN_POINT('Ctrl Pts',(21.5678473782707,16.4277894307452,39.8703438218898));
#52183=CARTESIAN_POINT('Ctrl Pts',(21.6253446365292,16.4320162353872,39.8158803144176));
#52184=CARTESIAN_POINT('Ctrl Pts',(21.6828697569516,16.4362450882647,39.761390414884));
#52185=CARTESIAN_POINT('Ctrl Pts',(21.7376074114044,16.4404739411421,39.7040465586615));
#52186=CARTESIAN_POINT('Ctrl Pts',(21.7892776549551,16.4447027940196,39.6441748328406));
#52187=CARTESIAN_POINT('Ctrl Pts',(21.8410407612566,16.4489392470723,39.5841955044081));
#52188=CARTESIAN_POINT('Ctrl Pts',(21.8897251528208,16.4531757001251,39.5216795994815));
#52189=CARTESIAN_POINT('Ctrl Pts',(21.9350923865942,16.4574121531779,39.4569848548327));
#52190=CARTESIAN_POINT('Ctrl Pts',(21.976325415169,16.461262548612,39.3981855842386));
#52191=CARTESIAN_POINT('Ctrl Pts',(22.0148187226789,16.4651129440462,39.3375870781129));
#52192=CARTESIAN_POINT('Ctrl Pts',(22.0504265113351,16.4689633394803,39.2754750369591));
#52193=CARTESIAN_POINT('Ctrl Pts',(22.0896154925085,16.4732009818578,39.2071161833692));
#52194=CARTESIAN_POINT('Ctrl Pts',(22.1254557885139,16.4774386242354,39.13666709751));
#52195=CARTESIAN_POINT('Ctrl Pts',(22.1577188864489,16.4816762666129,39.064489319776));
#52196=CARTESIAN_POINT('Ctrl Pts',(22.1899355887829,16.4859078150943,38.9924153365189));
#52197=CARTESIAN_POINT('Ctrl Pts',(22.2185851191369,16.4901393635758,38.9186180226358));
#52198=CARTESIAN_POINT('Ctrl Pts',(22.2434840702714,16.4943709120572,38.8434848131188));
#52199=CARTESIAN_POINT('Ctrl Pts',(22.2683542624298,16.4985975729833,38.7684383845336));
#52200=CARTESIAN_POINT('Ctrl Pts',(22.28948233747,16.5028242339094,38.6920595693594));
#52201=CARTESIAN_POINT('Ctrl Pts',(22.3067329646642,16.5070508948356,38.614755738804));
#52202=CARTESIAN_POINT('Ctrl Pts',(22.3239727027249,16.5112748877616,38.5375007048354));
#52203=CARTESIAN_POINT('Ctrl Pts',(22.3373397492575,16.5154988806876,38.4593222707827));
#52204=CARTESIAN_POINT('Ctrl Pts',(22.3467489526675,16.5197228736136,38.3806417539391));
#52205=CARTESIAN_POINT('Ctrl Pts',(22.3561551463312,16.5239455154001,38.3019864048362));
#52206=CARTESIAN_POINT('Ctrl Pts',(22.3616059552865,16.5281681571865,38.2228297569886));
#52207=CARTESIAN_POINT('Ctrl Pts',(22.3630678002548,16.532390798973,38.1436005997561));
#52208=CARTESIAN_POINT('Ctrl Pts',(22.3645296327657,16.5366134047755,38.0643721176886));
#52209=CARTESIAN_POINT('Ctrl Pts',(22.3620025616588,16.540836010578,37.9850715961843));
#52210=CARTESIAN_POINT('Ctrl Pts',(22.3555051174012,16.5450586163805,37.9061286952722));
#52211=CARTESIAN_POINT('Ctrl Pts',(22.3490012122692,16.5492854210225,37.8271072957774));
#52212=CARTESIAN_POINT('Ctrl Pts',(22.3385190863278,16.5535122256644,37.7484446954828));
#52213=CARTESIAN_POINT('Ctrl Pts',(22.3241292157766,16.5577390303064,37.6705656868929));
#52214=CARTESIAN_POINT('Ctrl Pts',(22.3097323721462,16.5619678831839,37.5926489395));
#52215=CARTESIAN_POINT('Ctrl Pts',(22.2914241199844,16.5661967360613,37.5155169969323));
#52216=CARTESIAN_POINT('Ctrl Pts',(22.2693256192087,16.5704255889388,37.4395821967096));
#52217=CARTESIAN_POINT('Ctrl Pts',(22.2471874025845,16.5746620419916,37.3635109250106));
#52218=CARTESIAN_POINT('Ctrl Pts',(22.2212454803348,16.5788984950444,37.2886415386048));
#52219=CARTESIAN_POINT('Ctrl Pts',(22.1916701532164,16.5831349480972,37.2153687884771));
#52220=CARTESIAN_POINT('Ctrl Pts',(22.1647899534174,16.5869853435312,37.1487732050921));
#52221=CARTESIAN_POINT('Ctrl Pts',(22.1349091057282,16.5908357389653,37.0834964970803));
#52222=CARTESIAN_POINT('Ctrl Pts',(22.1021879121243,16.5946861343994,37.0198164864161));
#52223=CARTESIAN_POINT('Ctrl Pts',(22.066175840369,16.5989237767769,36.9497319674593));
#52224=CARTESIAN_POINT('Ctrl Pts',(22.0265875321937,16.6031614191544,36.8813187642604));
#52225=CARTESIAN_POINT('Ctrl Pts',(21.983601884425,16.6073990615319,36.8149653681688));
#52226=CARTESIAN_POINT('Ctrl Pts',(21.9406780517048,16.6116306100133,36.748707390865));
#52227=CARTESIAN_POINT('Ctrl Pts',(21.8943668343264,16.6158621584948,36.6845037284246));
#52228=CARTESIAN_POINT('Ctrl Pts',(21.8448934038699,16.6200937069762,36.6227191298683));
#52229=CARTESIAN_POINT('Ctrl Pts',(21.7954771165918,16.6243203679023,36.5610058942294));
#52230=CARTESIAN_POINT('Ctrl Pts',(21.7429061660821,16.6285470288284,36.50170653399));
#52231=CARTESIAN_POINT('Ctrl Pts',(21.6874486175196,16.6327736897545,36.4451563203338));
#52232=CARTESIAN_POINT('Ctrl Pts',(21.6320260754899,16.6369976826806,36.3886418029347));
#52233=CARTESIAN_POINT('Ctrl Pts',(21.5737208794609,16.6412216756066,36.3348733214615));
#52234=CARTESIAN_POINT('Ctrl Pts',(21.5128401078154,16.6454456685326,36.2841516447993));
#52235=CARTESIAN_POINT('Ctrl Pts',(21.4519788102601,16.649668310319,36.2334461926113));
#52236=CARTESIAN_POINT('Ctrl Pts',(21.3885439330015,16.6538909521055,36.1857859097344));
#52237=CARTESIAN_POINT('Ctrl Pts',(21.3228768951412,16.658113593892,36.141432370021));
#52238=CARTESIAN_POINT('Ctrl Pts',(21.2572104168741,16.6623361996944,36.0970792082741));
#52239=CARTESIAN_POINT('Ctrl Pts',(21.1893122050906,16.6665588054969,36.0560329948581));
#52240=CARTESIAN_POINT('Ctrl Pts',(21.1195527744545,16.6707814112994,36.0185120643849));
#52241=CARTESIAN_POINT('Ctrl Pts',(21.049723977018,16.6750082159414,35.980953824162));
#52242=CARTESIAN_POINT('Ctrl Pts',(20.9780306776654,16.6792350205834,35.9469280915867));
#52243=CARTESIAN_POINT('Ctrl Pts',(20.9048675837599,16.6834618252254,35.9166069761125));
#52244=CARTESIAN_POINT('Ctrl Pts',(20.8316690363011,16.6876906781028,35.8862711675571));
#52245=CARTESIAN_POINT('Ctrl Pts',(20.756999717534,16.6919195309803,35.8596437099928));
#52246=CARTESIAN_POINT('Ctrl Pts',(20.6812714756874,16.6961483838577,35.8368474162543));
#52247=CARTESIAN_POINT('Ctrl Pts',(20.6054071335952,16.7003848369105,35.8140101525805));
#52248=CARTESIAN_POINT('Ctrl Pts',(20.5284805219995,16.7046212899633,35.7950179231385));
#52249=CARTESIAN_POINT('Ctrl Pts',(20.4509154854594,16.7088577430161,35.7799427451304));
#52250=CARTESIAN_POINT('Ctrl Pts',(20.380418761237,16.7127081384502,35.7662413312712));
#52251=CARTESIAN_POINT('Ctrl Pts',(20.3093950395558,16.7165585338844,35.7557749743961));
#52252=CARTESIAN_POINT('Ctrl Pts',(20.2381646343263,16.7204089293185,35.7485604307454));
#52253=CARTESIAN_POINT('Ctrl Pts',(20.1597703527705,16.724646571696,35.7406202966913));
#52254=CARTESIAN_POINT('Ctrl Pts',(20.0808314112834,16.7288842140735,35.7365899080065));
#52255=CARTESIAN_POINT('Ctrl Pts',(20.0017710825654,16.7331218564509,35.7365306635866));
#52256=CARTESIAN_POINT('Ctrl Pts',(19.9228244457023,16.7373534049324,35.7364715043625));
#52257=CARTESIAN_POINT('Ctrl Pts',(19.8437572331678,16.7415849534138,35.7403721489073));
#52258=CARTESIAN_POINT('Ctrl Pts',(19.7649979899845,16.7458165018953,35.7482422539325));
#52259=CARTESIAN_POINT('Ctrl Pts',(19.6863297159023,16.7500431628214,35.756103268769));
#52260=CARTESIAN_POINT('Ctrl Pts',(19.6079691683695,16.7542698237475,35.7679245864878));
#52261=CARTESIAN_POINT('Ctrl Pts',(19.5303435129165,16.7584964846736,35.7836638359166));
#52262=CARTESIAN_POINT('Ctrl Pts',(19.4527668571963,16.7627204775996,35.7993931502408));
#52263=CARTESIAN_POINT('Ctrl Pts',(19.3759246310148,16.7669444705256,35.8190353944952));
#52264=CARTESIAN_POINT('Ctrl Pts',(19.3002362933157,16.7711684634516,35.8424966897682));
#52265=CARTESIAN_POINT('Ctrl Pts',(19.2245721662411,16.7753911052381,35.865950480416));
#52266=CARTESIAN_POINT('Ctrl Pts',(19.1500616421277,16.7796137470245,35.8932207575148));
#52267=CARTESIAN_POINT('Ctrl Pts',(19.0771099933496,16.783836388811,35.9241634995881));
#52268=CARTESIAN_POINT('Ctrl Pts',(19.0041589662422,16.7880589946134,35.9551059779772));
#52269=CARTESIAN_POINT('Ctrl Pts',(18.9327672190563,16.7922816004159,35.9897206747529));
#52270=CARTESIAN_POINT('Ctrl Pts',(18.8633195899172,16.7965042062183,36.0278156244595));
#52271=CARTESIAN_POINT('Ctrl Pts',(18.7938029040242,16.8007310108603,36.0659484547044));
#52272=CARTESIAN_POINT('Ctrl Pts',(18.7262346096606,16.8049578155023,36.1075682245992));
#52273=CARTESIAN_POINT('Ctrl Pts',(18.6609739371107,16.8091846201442,36.1524375122212));
#52274=CARTESIAN_POINT('Ctrl Pts',(18.5956816403823,16.8134134730217,36.1973285427139));
#52275=CARTESIAN_POINT('Ctrl Pts',(18.5326995660242,16.8176423258991,36.2454719427909));
#52276=CARTESIAN_POINT('Ctrl Pts',(18.4723549213669,16.8218711787766,36.2965890777119));
#52277=CARTESIAN_POINT('Ctrl Pts',(18.4119018241592,16.8261076318293,36.3477980813261));
#52278=CARTESIAN_POINT('Ctrl Pts',(18.3540959705091,16.8303440848821,36.4019911771457));
#52279=CARTESIAN_POINT('Ctrl Pts',(18.2992284869659,16.8345805379349,36.4588520172295));
#52280=CARTESIAN_POINT('Ctrl Pts',(18.2493609431761,16.8384309333691,36.5105312678474));
#52281=CARTESIAN_POINT('Ctrl Pts',(18.2019203203939,16.8422813288033,36.5644135560128));
#52282=CARTESIAN_POINT('Ctrl Pts',(18.1570950331286,16.8461317242375,36.6202393017853));
#52283=CARTESIAN_POINT('Ctrl Pts',(18.1079067904915,16.8503568881221,36.6814987045908));
#52284=CARTESIAN_POINT('Ctrl Pts',(18.0616790360622,16.8545820520066,36.7453345810201));
#52285=CARTESIAN_POINT('Ctrl Pts',(18.0186939304945,16.8588072158912,36.8114284265744));
#52286=CARTESIAN_POINT('Ctrl Pts',(17.975768405893,16.8630265233437,36.8774306605082));
#52287=CARTESIAN_POINT('Ctrl Pts',(17.936076864836,16.8672458307963,36.9456842612171));
#52288=CARTESIAN_POINT('Ctrl Pts',(17.8998612449744,16.8714651382489,37.0158378117001));
#52289=CARTESIAN_POINT('Ctrl Pts',(17.8636843923002,16.8756799291231,37.0859162659717));
#52290=CARTESIAN_POINT('Ctrl Pts',(17.8309762887945,16.8798947199974,37.1578902158748));
#52291=CARTESIAN_POINT('Ctrl Pts',(17.8019347238809,16.8841095108716,37.2313807031736));
#52292=CARTESIAN_POINT('Ctrl Pts',(17.7729126268906,16.8883214763738,37.3048219263509));
#52293=CARTESIAN_POINT('Ctrl Pts',(17.7475523634037,16.892533441876,37.379777232228));
#52294=CARTESIAN_POINT('Ctrl Pts',(17.7260044227758,16.8967454073782,37.4558458603218));
#52295=CARTESIAN_POINT('Ctrl Pts',(17.7044654610623,16.9009556177764,37.531882791015));
#52296=CARTESIAN_POINT('Ctrl Pts',(17.6867357926461,16.9051658281745,37.6090316686098));
#52297=CARTESIAN_POINT('Ctrl Pts',(17.6729161652158,16.9093760385726,37.6868762088842));
#52298=CARTESIAN_POINT('Ctrl Pts',(17.6590929138932,16.9135873530055,37.7647411621709));
#52299=CARTESIAN_POINT('Ctrl Pts',(17.6491818400631,16.9177986674384,37.8433016790901));
#52300=CARTESIAN_POINT('Ctrl Pts',(17.6432324255559,16.9220099818713,37.9221319563585));
#52301=CARTESIAN_POINT('Ctrl Pts',(17.6387172882919,16.9252060380047,37.9819579311661));
#52302=CARTESIAN_POINT('Ctrl Pts',(17.6364828620914,16.9284020941382,38.0419390384473));
#52303=CARTESIAN_POINT('Ctrl Pts',(17.636530754193,16.9315981502717,38.1018881272695));
#52304=CARTESIAN_POINT('',(17.6365300019755,17.7253481502437,38.1000966336477));
#52305=CARTESIAN_POINT('Ctrl Pts',(17.6365307541938,16.9315981503216,38.1018881282061));
#52306=CARTESIAN_POINT('Ctrl Pts',(17.6366053049449,16.9365732560039,38.1952072189802));
#52307=CARTESIAN_POINT('Ctrl Pts',(17.6422106724848,16.9415483616861,38.2882936701097));
#52308=CARTESIAN_POINT('Ctrl Pts',(17.6532411624811,16.9465234673684,38.3805590836651));
#52309=CARTESIAN_POINT('Ctrl Pts',(17.6643975571371,16.9515553601007,38.4738776367906));
#52310=CARTESIAN_POINT('Ctrl Pts',(17.6811035375494,16.956587252833,38.5663562147621));
#52311=CARTESIAN_POINT('Ctrl Pts',(17.7032004638078,16.9616191455653,38.6574067917125));
#52312=CARTESIAN_POINT('Ctrl Pts',(17.7181829172308,16.9650309367624,38.7191421214297));
#52313=CARTESIAN_POINT('Ctrl Pts',(17.7356427284869,16.9684427279595,38.7802213906737));
#52314=CARTESIAN_POINT('Ctrl Pts',(17.7555180592357,16.9718545191566,38.8404669192362));
#52315=CARTESIAN_POINT('Ctrl Pts',(17.7802043717861,16.9760921615341,38.9152953568933));
#52316=CARTESIAN_POINT('Ctrl Pts',(17.8086831558674,16.9803298039116,38.9890283845905));
#52317=CARTESIAN_POINT('Ctrl Pts',(17.8408380437667,16.9845674462891,39.0612544344007));
#52318=CARTESIAN_POINT('Ctrl Pts',(17.8729466916755,16.9887989947706,39.1333766203169));
#52319=CARTESIAN_POINT('Ctrl Pts',(17.908720756057,16.9930305432521,39.2039957072802));
#52320=CARTESIAN_POINT('Ctrl Pts',(17.947994467672,16.9972620917336,39.2727163920553));
#52321=CARTESIAN_POINT('Ctrl Pts',(17.9872228170654,17.0014887526597,39.3413577025416));
#52322=CARTESIAN_POINT('Ctrl Pts',(18.0299425494248,17.0057154135858,39.4081045633627));
#52323=CARTESIAN_POINT('Ctrl Pts',(18.0759409430028,17.0099420745119,39.4725841271438));
#52324=CARTESIAN_POINT('Ctrl Pts',(18.1219103009614,17.014166067438,39.5370229894149));
#52325=CARTESIAN_POINT('Ctrl Pts',(18.171153940697,17.018390060364,39.5991970147754));
#52326=CARTESIAN_POINT('Ctrl Pts',(18.22341524062,17.02261405329,39.6587613780303));
#52327=CARTESIAN_POINT('Ctrl Pts',(18.2756598235857,17.0268366950765,39.718306688278));
#52328=CARTESIAN_POINT('Ctrl Pts',(18.3309198409661,17.031059336863,39.7752436419715));
#52329=CARTESIAN_POINT('Ctrl Pts',(18.3888986580057,17.0352819786495,39.8292607977758));
#52330=CARTESIAN_POINT('Ctrl Pts',(18.4468769809688,17.039504584452,39.8832774932636));
#52331=CARTESIAN_POINT('Ctrl Pts',(18.5075737135671,17.0437271902545,39.934374121833));
#52332=CARTESIAN_POINT('Ctrl Pts',(18.5706567610301,17.047949796057,39.9822774360096));
#52333=CARTESIAN_POINT('Ctrl Pts',(18.633802536487,17.052176600699,40.0302283838838));
#52334=CARTESIAN_POINT('Ctrl Pts',(18.6993389924538,17.056403405341,40.07497939045));
#52335=CARTESIAN_POINT('Ctrl Pts',(18.7669029535764,17.060630209983,40.1162991134753));
#52336=CARTESIAN_POINT('Ctrl Pts',(18.8344996550106,17.0648590628604,40.1576388593144));
#52337=CARTESIAN_POINT('Ctrl Pts',(18.904125406601,17.0690879157379,40.195543784812));
#52338=CARTESIAN_POINT('Ctrl Pts',(18.9753924414283,17.0733167686154,40.229828582731));
#52339=CARTESIAN_POINT('Ctrl Pts',(19.0467875587346,17.0775532216682,40.264174997945));
#52340=CARTESIAN_POINT('Ctrl Pts',(19.1198294200048,17.0817896747209,40.2948881035024));
#52341=CARTESIAN_POINT('Ctrl Pts',(19.1941105159324,17.0860261277737,40.3218309072405));
#52342=CARTESIAN_POINT('Ctrl Pts',(19.2616225570264,17.0898765232077,40.3463184790842));
#52343=CARTESIAN_POINT('Ctrl Pts',(19.3301578021318,17.0937269186418,40.3676921508715));
#52344=CARTESIAN_POINT('Ctrl Pts',(19.3994024300127,17.0975773140758,40.3858856051486));
#52345=CARTESIAN_POINT('Ctrl Pts',(19.4756112180581,17.1018149564533,40.4059088350113));
#52346=CARTESIAN_POINT('Ctrl Pts',(19.5529654791961,17.1060525988307,40.4221544128668));
#52347=CARTESIAN_POINT('Ctrl Pts',(19.6310566193519,17.1102902412082,40.4344959247718));
#52348=CARTESIAN_POINT('Ctrl Pts',(19.7090354613836,17.1145217896897,40.4468196890983));
#52349=CARTESIAN_POINT('Ctrl Pts',(19.7877486188433,17.1187533381711,40.4552504641836));
#52350=CARTESIAN_POINT('Ctrl Pts',(19.8667742505727,17.1229848866526,40.4597121308731));
#52351=CARTESIAN_POINT('Ctrl Pts',(19.9457086055152,17.1272115475786,40.4641686442143));
#52352=CARTESIAN_POINT('Ctrl Pts',(20.0249542518364,17.1314382085047,40.4646651332847));
#52353=CARTESIAN_POINT('Ctrl Pts',(20.1040826279532,17.1356648694308,40.4611770893896));
#52354=CARTESIAN_POINT('Ctrl Pts',(20.1831610557731,17.1398888623568,40.4576912472565));
#52355=CARTESIAN_POINT('Ctrl Pts',(20.2621218932258,17.1441128552828,40.4502258850654));
#52356=CARTESIAN_POINT('Ctrl Pts',(20.3405361893824,17.1483368482088,40.4388085737445));
#52357=CARTESIAN_POINT('Ctrl Pts',(20.4189254029551,17.1525594899953,40.4273949145086));
#52358=CARTESIAN_POINT('Ctrl Pts',(20.4967679588492,17.1567821317817,40.4120318839297));
#52359=CARTESIAN_POINT('Ctrl Pts',(20.5736411301864,17.1610047735682,40.392798790705));
#52360=CARTESIAN_POINT('Ctrl Pts',(20.6505136464356,17.1652273793707,40.3735658613786));
#52361=CARTESIAN_POINT('Ctrl Pts',(20.726416340144,17.1694499851731,40.3504630501428));
#52362=CARTESIAN_POINT('Ctrl Pts',(20.8009392218789,17.1736725909756,40.3236202022279));
#52363=CARTESIAN_POINT('Ctrl Pts',(20.8755362070547,17.1778993956176,40.296750662546));
#52364=CARTESIAN_POINT('Ctrl Pts',(20.9487501975282,17.1821262002595,40.2661338167213));
#52365=CARTESIAN_POINT('Ctrl Pts',(21.0201894385494,17.1863530049015,40.2319483929899));
#52366=CARTESIAN_POINT('Ctrl Pts',(21.0916632977751,17.1905818577789,40.1977464036011));
#52367=CARTESIAN_POINT('Ctrl Pts',(21.1613602816399,17.1948107106564,40.1599726150488));
#52368=CARTESIAN_POINT('Ctrl Pts',(21.2289138665968,17.1990395635338,40.1188514431196));
#52369=CARTESIAN_POINT('Ctrl Pts',(21.2965888601495,17.2032760165866,40.0776563674333));
#52370=CARTESIAN_POINT('Ctrl Pts',(21.3621123692442,17.2075124696394,40.0331021520699));
#52371=CARTESIAN_POINT('Ctrl Pts',(21.4251476538011,17.2117489226921,39.985456073677));
#52372=CARTESIAN_POINT('Ctrl Pts',(21.4824386868489,17.2155993181263,39.9421518660256));
#52373=CARTESIAN_POINT('Ctrl Pts',(21.5376745363659,17.2194497135605,39.8962943192532));
#52374=CARTESIAN_POINT('Ctrl Pts',(21.5906287467406,17.2233001089947,39.8481105888766));
#52375=CARTESIAN_POINT('Ctrl Pts',(21.6489087363638,17.2275377513722,39.795080862128));
#52376=CARTESIAN_POINT('Ctrl Pts',(21.7046432978637,17.2317753937497,39.739033924919));
#52377=CARTESIAN_POINT('Ctrl Pts',(21.757503974408,17.2360130361272,39.6802437219746));
#52378=CARTESIAN_POINT('Ctrl Pts',(21.8102886352249,17.2402445846087,39.6215380616492));
#52379=CARTESIAN_POINT('Ctrl Pts',(21.8602073075257,17.2444761330901,39.5600973155472));
#52380=CARTESIAN_POINT('Ctrl Pts',(21.9069665142878,17.2487076815716,39.4962339181832));
#52381=CARTESIAN_POINT('Ctrl Pts',(21.9536717128749,17.2529343424977,39.4324442848067));
#52382=CARTESIAN_POINT('Ctrl Pts',(21.9972244224118,17.2571610034238,39.3662379372689));
#52383=CARTESIAN_POINT('Ctrl Pts',(22.0373708020521,17.2613876643499,39.2979610410383));
#52384=CARTESIAN_POINT('Ctrl Pts',(22.0774918400465,17.2656116572759,39.2297272433123));
#52385=CARTESIAN_POINT('Ctrl Pts',(22.114210579034,17.2698356502019,39.1594258941711));
#52386=CARTESIAN_POINT('Ctrl Pts',(22.1473166541412,17.2740596431279,39.0874318344817));
#52387=CARTESIAN_POINT('Ctrl Pts',(22.1804121395224,17.2782822849144,39.0154608037186));
#52388=CARTESIAN_POINT('Ctrl Pts',(22.2098970600938,17.2825049267009,38.9417985632177));
#52389=CARTESIAN_POINT('Ctrl Pts',(22.2356078400915,17.2867275684873,38.8668428953975));
#52390=CARTESIAN_POINT('Ctrl Pts',(22.2613184009903,17.2909501742898,38.7918878663251));
#52391=CARTESIAN_POINT('Ctrl Pts',(22.283254734519,17.2951727800923,38.715639875725));
#52392=CARTESIAN_POINT('Ctrl Pts',(22.3013025918172,17.2993953858948,38.6385135298163));
#52393=CARTESIAN_POINT('Ctrl Pts',(22.3193683953931,17.3036221905368,38.5613104916558));
#52394=CARTESIAN_POINT('Ctrl Pts',(22.3335378921486,17.3078489951787,38.4832278110472));
#52395=CARTESIAN_POINT('Ctrl Pts',(22.3437477653784,17.3120757998207,38.4046914064819));
#52396=CARTESIAN_POINT('Ctrl Pts',(22.3539625861338,17.3163046526982,38.326116944551));
#52397=CARTESIAN_POINT('Ctrl Pts',(22.3602139239478,17.3205335055756,38.2470887885748));
#52398=CARTESIAN_POINT('Ctrl Pts',(22.3624905221608,17.3247623584531,38.1680365607634));
#52399=CARTESIAN_POINT('Ctrl Pts',(22.3647712119197,17.3289988115059,38.0888422587751));
#52400=CARTESIAN_POINT('Ctrl Pts',(22.363062898846,17.3332352645586,38.0096242682856));
#52401=CARTESIAN_POINT('Ctrl Pts',(22.3574064930663,17.3374717176114,37.9308105578091));
#52402=CARTESIAN_POINT('Ctrl Pts',(22.3522655417288,17.3413221130456,37.8591789482557));
#52403=CARTESIAN_POINT('Ctrl Pts',(22.3438639675438,17.3451725084797,37.7878814923479));
#52404=CARTESIAN_POINT('Ctrl Pts',(22.3322690560765,17.3490229039139,37.717231805177));
#52405=CARTESIAN_POINT('Ctrl Pts',(22.3195080061954,17.3532605462914,37.6394766464063));
#52406=CARTESIAN_POINT('Ctrl Pts',(22.3028303492847,17.3574981886689,37.5622143899281));
#52407=CARTESIAN_POINT('Ctrl Pts',(22.2822870979711,17.3617358310464,37.4858696853805));
#52408=CARTESIAN_POINT('Ctrl Pts',(22.2617733886591,17.3659673795279,37.4096347675142));
#52409=CARTESIAN_POINT('Ctrl Pts',(22.237405245159,17.3701989280093,37.3343152301535));
#52410=CARTESIAN_POINT('Ctrl Pts',(22.2092850086877,17.3744304764908,37.2603273308677));
#52411=CARTESIAN_POINT('Ctrl Pts',(22.1811972518661,17.3786571374169,37.1864248896487));
#52412=CARTESIAN_POINT('Ctrl Pts',(22.1493661800651,17.382883798343,37.1138514659295));
#52413=CARTESIAN_POINT('Ctrl Pts',(22.1139440056845,17.3871104592691,37.0430084287326));
#52414=CARTESIAN_POINT('Ctrl Pts',(22.0785441908843,17.3913344521951,36.9722101098683));
#52415=CARTESIAN_POINT('Ctrl Pts',(22.0395579819799,17.3955584451212,36.9031404276685));
#52416=CARTESIAN_POINT('Ctrl Pts',(21.9971853117504,17.3997824380472,36.836179889609));
#52417=CARTESIAN_POINT('Ctrl Pts',(21.9548261953766,17.4040050798337,36.7692407703904));
#52418=CARTESIAN_POINT('Ctrl Pts',(21.9090830192574,17.4082277216201,36.7044098514143));
#52419=CARTESIAN_POINT('Ctrl Pts',(21.8602004300706,17.4124503634066,36.6420408781914));
#52420=CARTESIAN_POINT('Ctrl Pts',(21.8113182574454,17.4166729692091,36.5796724364565));
#52421=CARTESIAN_POINT('Ctrl Pts',(21.7592970152437,17.4208955750116,36.5197662668323));
#52422=CARTESIAN_POINT('Ctrl Pts',(21.7044223134702,17.4251181808141,36.4626438938811));
#52423=CARTESIAN_POINT('Ctrl Pts',(21.649493045849,17.4293449854561,36.4054647200616));
#52424=CARTESIAN_POINT('Ctrl Pts',(21.5917049764482,17.4335717900981,36.3510752111073));
#52425=CARTESIAN_POINT('Ctrl Pts',(21.5313809289529,17.43779859474,36.2997603239182));
#52426=CARTESIAN_POINT('Ctrl Pts',(21.4710276494813,17.4420274476175,36.2484205704339));
#52427=CARTESIAN_POINT('Ctrl Pts',(21.4081363161896,17.446256300495,36.2001586925353));
#52428=CARTESIAN_POINT('Ctrl Pts',(21.3430611978254,17.4504851533724,36.155217991703));
#52429=CARTESIAN_POINT('Ctrl Pts',(21.2778691252131,17.4547216064252,36.1101965225831));
#52430=CARTESIAN_POINT('Ctrl Pts',(21.2104858251109,17.458958059478,36.0685084041545));
#52431=CARTESIAN_POINT('Ctrl Pts',(21.1412925752695,17.4631945125308,36.0303522767063));
#52432=CARTESIAN_POINT('Ctrl Pts',(21.0784047372744,17.4670449079649,35.9956732239522));
#52433=CARTESIAN_POINT('Ctrl Pts',(21.0140223370739,17.4708953033989,35.963911293723));
#52434=CARTESIAN_POINT('Ctrl Pts',(20.9484450821268,17.474745698833,35.9351807541761));
#52435=CARTESIAN_POINT('Ctrl Pts',(20.8762725067844,17.4789833412105,35.9035606896927));
#52436=CARTESIAN_POINT('Ctrl Pts',(20.8023814628332,17.483220983588,35.8754944441318));
#52437=CARTESIAN_POINT('Ctrl Pts',(20.7271559430759,17.4874586259655,35.8511703765404));
#52438=CARTESIAN_POINT('Ctrl Pts',(20.6520386005681,17.4916901744469,35.8268812879128));
#52439=CARTESIAN_POINT('Ctrl Pts',(20.5755910356176,17.4959217229284,35.8063238333286));
#52440=CARTESIAN_POINT('Ctrl Pts',(20.4982181411682,17.5001532714098,35.7896387458428));
#52441=CARTESIAN_POINT('Ctrl Pts',(20.4209346145485,17.5043799323359,35.7729729300938));
#52442=CARTESIAN_POINT('Ctrl Pts',(20.3427283382872,17.508606593262,35.7601706913982));
#52443=CARTESIAN_POINT('Ctrl Pts',(20.2640188624652,17.5128332541881,35.7513228231273));
#52444=CARTESIAN_POINT('Ctrl Pts',(20.1853590705172,17.5170572471141,35.7424805399067));
#52445=CARTESIAN_POINT('Ctrl Pts',(20.1061971741,17.5212812400401,35.7375877248133));
#52446=CARTESIAN_POINT('Ctrl Pts',(20.0269611991178,17.5255052329662,35.7366837844584));
#52447=CARTESIAN_POINT('Ctrl Pts',(19.947750569552,17.5297278747526,35.7357801332491));
#52448=CARTESIAN_POINT('Ctrl Pts',(19.868466376881,17.5339505165391,35.7388628283737));
#52449=CARTESIAN_POINT('Ctrl Pts',(19.7895385366271,17.5381731583255,35.7459191999137));
#52450=CARTESIAN_POINT('Ctrl Pts',(19.7106113689705,17.542395764128,35.7529755113217));
#52451=CARTESIAN_POINT('Ctrl Pts',(19.6320410144762,17.5466183699305,35.7640053886495));
#52452=CARTESIAN_POINT('Ctrl Pts',(19.5542526573517,17.550840975733,35.7789442601648));
#52453=CARTESIAN_POINT('Ctrl Pts',(19.4763869496902,17.555067780375,35.7938979864704));
#52454=CARTESIAN_POINT('Ctrl Pts',(19.3993052540812,17.559294585017,35.8127683826339));
#52455=CARTESIAN_POINT('Ctrl Pts',(19.323422336034,17.5635213896589,35.8354397544949));
#52456=CARTESIAN_POINT('Ctrl Pts',(19.2475026464544,17.5677502425364,35.8581221125053));
#52457=CARTESIAN_POINT('Ctrl Pts',(19.1727833340701,17.5719790954138,35.884608958642));
#52458=CARTESIAN_POINT('Ctrl Pts',(19.0996613376738,17.5762079482913,35.914735545976));
#52459=CARTESIAN_POINT('Ctrl Pts',(19.0264079250261,17.5804444013441,35.9449162773894));
#52460=CARTESIAN_POINT('Ctrl Pts',(18.9547579892537,17.5846808543968,35.9787496197392));
#52461=CARTESIAN_POINT('Ctrl Pts',(18.8850857062837,17.5889173074496,36.0160238584458));
#52462=CARTESIAN_POINT('Ctrl Pts',(18.8217624882773,17.5927677028838,36.0499013868261));
#52463=CARTESIAN_POINT('Ctrl Pts',(18.7600728064957,17.5966180983179,36.0866205484366));
#52464=CARTESIAN_POINT('Ctrl Pts',(18.7002756582113,17.600468493752,36.1259921286221));
#52465=CARTESIAN_POINT('Ctrl Pts',(18.6345424421239,17.604701118256,36.1692721287941));
#52466=CARTESIAN_POINT('Ctrl Pts',(18.5708485327689,17.6089337427599,36.2159212483599));
#52467=CARTESIAN_POINT('Ctrl Pts',(18.5095604553716,17.6131663672639,36.265720739716));
#52468=CARTESIAN_POINT('Ctrl Pts',(18.4483605673713,17.6173929013075,36.3154485729732));
#52469=CARTESIAN_POINT('Ctrl Pts',(18.3895599986511,17.6216194353511,36.3683174822045));
#52470=CARTESIAN_POINT('Ctrl Pts',(18.3334967480836,17.6258459693948,36.4240652303112));
#52471=CARTESIAN_POINT('Ctrl Pts',(18.2774981086243,17.6300676324927,36.479748730916));
#52472=CARTESIAN_POINT('Ctrl Pts',(18.2242308501914,17.6342892955907,36.5383041478187));
#52473=CARTESIAN_POINT('Ctrl Pts',(18.1739990900591,17.6385109586886,36.5994297358021));
#52474=CARTESIAN_POINT('Ctrl Pts',(18.1237988641362,17.6427299715348,36.6605169507107));
#52475=CARTESIAN_POINT('Ctrl Pts',(18.0766306519891,17.6469489843811,36.7241707721064));
#52476=CARTESIAN_POINT('Ctrl Pts',(18.0327600941566,17.6511679972273,36.7900543546554));
#52477=CARTESIAN_POINT('Ctrl Pts',(17.9889033281849,17.6553856837161,36.8559172249717));
#52478=CARTESIAN_POINT('Ctrl Pts',(17.9483424182565,17.659603370205,36.9240080735154));
#52479=CARTESIAN_POINT('Ctrl Pts',(17.9113003524991,17.6638210566939,36.9939601167094));
#52480=CARTESIAN_POINT('Ctrl Pts',(17.8742583231946,17.6680387390321,37.0639120910639));
#52481=CARTESIAN_POINT('Ctrl Pts',(17.8407353497272,17.6722564213704,37.135724840284));
#52482=CARTESIAN_POINT('Ctrl Pts',(17.8109083021627,17.6764741037086,37.2090073067864));
#52483=CARTESIAN_POINT('Ctrl Pts',(17.7810515334304,17.6806959887574,37.2823627956183));
#52484=CARTESIAN_POINT('Ctrl Pts',(17.7548982238135,17.6849178738061,37.3571904904136));
#52485=CARTESIAN_POINT('Ctrl Pts',(17.7325766757284,17.6891397588548,37.4330802826057));
#52486=CARTESIAN_POINT('Ctrl Pts',(17.7102440755141,17.6933637342971,37.5090076503188));
#52487=CARTESIAN_POINT('Ctrl Pts',(17.6917471255497,17.6975877097393,37.5859977053169));
#52488=CARTESIAN_POINT('Ctrl Pts',(17.6771632698953,17.7018116851816,37.6636286373093));
#52489=CARTESIAN_POINT('Ctrl Pts',(17.6625534885534,17.7060431695755,37.7413975736359));
#52490=CARTESIAN_POINT('Ctrl Pts',(17.6518707623599,17.7102746539695,37.8198091963865));
#52491=CARTESIAN_POINT('Ctrl Pts',(17.6451407419896,17.7145061383634,37.8984353308179));
#52492=CARTESIAN_POINT('Ctrl Pts',(17.6393928015494,17.7181201423235,37.9655879266325));
#52493=CARTESIAN_POINT('Ctrl Pts',(17.6365272544186,17.7217341462836,38.0328967675363));
#52494=CARTESIAN_POINT('Ctrl Pts',(17.6365300019755,17.7253481502437,38.1000966336477));
#52495=CARTESIAN_POINT('',(17.6365308155374,18.5190981502267,38.0980365857439));
#52496=CARTESIAN_POINT('Ctrl Pts',(17.6365300019755,17.7253481502717,38.100096634168));
#52497=CARTESIAN_POINT('Ctrl Pts',(17.6365302156428,17.7256291964049,38.1053224896805));
#52498=CARTESIAN_POINT('Ctrl Pts',(17.6365477615718,17.725910242538,38.1105483033315));
#52499=CARTESIAN_POINT('Ctrl Pts',(17.6365826391035,17.7261912886711,38.1157740011787));
#52500=CARTESIAN_POINT('Ctrl Pts',(17.6371085260988,17.7304289310486,38.1945676084847));
#52501=CARTESIAN_POINT('Ctrl Pts',(17.6415800413973,17.7346665734261,38.2734827912252));
#52502=CARTESIAN_POINT('Ctrl Pts',(17.6500127662927,17.7389042158035,38.3520921306049));
#52503=CARTESIAN_POINT('Ctrl Pts',(17.6584333645989,17.743135764285,38.4305884266698));
#52504=CARTESIAN_POINT('Ctrl Pts',(17.670803810442,17.7473673127664,38.508779290557));
#52505=CARTESIAN_POINT('Ctrl Pts',(17.6870876759688,17.7515988612478,38.5862376191171));
#52506=CARTESIAN_POINT('Ctrl Pts',(17.7033527331813,17.7558255221739,38.6636064811689));
#52507=CARTESIAN_POINT('Ctrl Pts',(17.7235221315334,17.7600521831,38.7402440328805));
#52508=CARTESIAN_POINT('Ctrl Pts',(17.7475078644291,17.7642788440261,38.8157301307695));
#52509=CARTESIAN_POINT('Ctrl Pts',(17.7714784567827,17.7685028369521,38.8911685794812));
#52510=CARTESIAN_POINT('Ctrl Pts',(17.7992604605148,17.7727268298781,38.9654565714615));
#52511=CARTESIAN_POINT('Ctrl Pts',(17.8307154869953,17.7769508228041,39.0381871575214));
#52512=CARTESIAN_POINT('Ctrl Pts',(17.8621604518751,17.7811734645905,39.1108944790603));
#52513=CARTESIAN_POINT('Ctrl Pts',(17.8972759204384,17.7853961063769,39.1820449540007));
#52514=CARTESIAN_POINT('Ctrl Pts',(17.9358751752938,17.7896187481634,39.2512511233139));
#52515=CARTESIAN_POINT('Ctrl Pts',(17.9744741012189,17.7938413539658,39.3204567028747));
#52516=CARTESIAN_POINT('Ctrl Pts',(18.0165565248192,17.7980639597683,39.3877176010481));
#52517=CARTESIAN_POINT('Ctrl Pts',(18.061890256853,17.8022865655707,39.4526718243605));
#52518=CARTESIAN_POINT('Ctrl Pts',(18.1072690674647,17.8065133702127,39.5176906363111));
#52519=CARTESIAN_POINT('Ctrl Pts',(18.1559053755455,17.8107401748546,39.5803978064397));
#52520=CARTESIAN_POINT('Ctrl Pts',(18.207524548805,17.8149669794966,39.6404616833156));
#52521=CARTESIAN_POINT('Ctrl Pts',(18.2591687358114,17.819195832374,39.7005546660937));
#52522=CARTESIAN_POINT('Ctrl Pts',(18.3137983440383,17.8234246852514,39.7580014637972));
#52523=CARTESIAN_POINT('Ctrl Pts',(18.3711012062747,17.8276535381289,39.8125066892425));
#52524=CARTESIAN_POINT('Ctrl Pts',(18.4285070543117,17.8318899911816,39.8671098725221));
#52525=CARTESIAN_POINT('Ctrl Pts',(18.4885953997276,17.8361264442344,39.9187606140064));
#52526=CARTESIAN_POINT('Ctrl Pts',(18.5510204556017,17.8403628972871,39.9672034492297));
#52527=CARTESIAN_POINT('Ctrl Pts',(18.6077568686182,17.8442132927215,40.0112318072093));
#52528=CARTESIAN_POINT('Ctrl Pts',(18.6664229068114,17.8480636881558,40.0526106620861));
#52529=CARTESIAN_POINT('Ctrl Pts',(18.7267402548508,17.8519140835901,40.0911805699842));
#52530=CARTESIAN_POINT('Ctrl Pts',(18.7931239171296,17.8561517259677,40.1336295804805));
#52531=CARTESIAN_POINT('Ctrl Pts',(18.8617573107764,17.8603893683452,40.1728349091079));
#52532=CARTESIAN_POINT('Ctrl Pts',(18.9322903694693,17.8646270107228,40.2085508259874));
#52533=CARTESIAN_POINT('Ctrl Pts',(19.0027219988558,17.8688585592043,40.2442153819768));
#52534=CARTESIAN_POINT('Ctrl Pts',(19.0750474534436,17.8730901076858,40.2764002813037));
#52535=CARTESIAN_POINT('Ctrl Pts',(19.1488886212691,17.8773216561673,40.3049035946941));
#52536=CARTESIAN_POINT('Ctrl Pts',(19.2226445005066,17.8815483170935,40.3333739859703));
#52537=CARTESIAN_POINT('Ctrl Pts',(19.2979121788094,17.8857749780197,40.3581710738102));
#52538=CARTESIAN_POINT('Ctrl Pts',(19.3742913063108,17.8900016389458,40.3791399850693));
#52539=CARTESIAN_POINT('Ctrl Pts',(19.4506222209268,17.8942256318719,40.4000956600982));
#52540=CARTESIAN_POINT('Ctrl Pts',(19.5280627413151,17.898449624798,40.4172278311821));
#52541=CARTESIAN_POINT('Ctrl Pts',(19.6061961611427,17.902673617724,40.4304310711543));
#52542=CARTESIAN_POINT('Ctrl Pts',(19.6843045882309,17.9068962595106,40.4436300877719));
#52543=CARTESIAN_POINT('Ctrl Pts',(19.7631050127389,17.9111189012971,40.4529025908986));
#52544=CARTESIAN_POINT('Ctrl Pts',(19.8421707709355,17.9153415430836,40.4581943039862));
#52545=CARTESIAN_POINT('Ctrl Pts',(19.9212358553596,17.9195641488861,40.4634859719796));
#52546=CARTESIAN_POINT('Ctrl Pts',(20.0005658011548,17.9237867546887,40.4647968875055));
#52547=CARTESIAN_POINT('Ctrl Pts',(20.0797305548749,17.9280093604912,40.4621247806836));
#52548=CARTESIAN_POINT('Ctrl Pts',(20.1589740277818,17.9322361651333,40.4594500167944));
#52549=CARTESIAN_POINT('Ctrl Pts',(20.2380515109032,17.9364629697753,40.4527843350827));
#52550=CARTESIAN_POINT('Ctrl Pts',(20.3165353004896,17.9406897744173,40.4421775860178));
#52551=CARTESIAN_POINT('Ctrl Pts',(20.3950571219453,17.9449186272949,40.4315656971081));
#52552=CARTESIAN_POINT('Ctrl Pts',(20.4729842153547,17.9491474801724,40.4170090225433));
#52553=CARTESIAN_POINT('Ctrl Pts',(20.5498988662793,17.9533763330499,40.3986086395393));
#52554=CARTESIAN_POINT('Ctrl Pts',(20.6269517496866,17.9576127861027,40.3801751870149));
#52555=CARTESIAN_POINT('Ctrl Pts',(20.7029881040009,17.9618492391555,40.357884355413));
#52556=CARTESIAN_POINT('Ctrl Pts',(20.7776054042554,17.9660856922084,40.3318871557883));
#52557=CARTESIAN_POINT('Ctrl Pts',(20.84542301219,17.969936087642,40.3082590174674));
#52558=CARTESIAN_POINT('Ctrl Pts',(20.9120684013927,17.9737864830757,40.2815699604525));
#52559=CARTESIAN_POINT('Ctrl Pts',(20.9772563226411,17.9776368785093,40.2519666634867));
#52560=CARTESIAN_POINT('Ctrl Pts',(21.0490004077203,17.9818745208867,40.2193860654945));
#52561=CARTESIAN_POINT('Ctrl Pts',(21.1192480819326,17.9861121632642,40.1831525894848));
#52562=CARTESIAN_POINT('Ctrl Pts',(21.1876026569099,17.9903498056416,40.1434261352445));
#52563=CARTESIAN_POINT('Ctrl Pts',(21.2558589353261,17.994581354123,40.1037568092045));
#52564=CARTESIAN_POINT('Ctrl Pts',(21.3222271188972,17.9988129026045,40.0606047138301));
#52565=CARTESIAN_POINT('Ctrl Pts',(21.3863319959239,18.0030444510859,40.0141771177134));
#52566=CARTESIAN_POINT('Ctrl Pts',(21.4503628300475,18.0072711120119,39.9678031467523));
#52567=CARTESIAN_POINT('Ctrl Pts',(21.5121351749246,18.011497772938,39.9181614669805));
#52568=CARTESIAN_POINT('Ctrl Pts',(21.5713011878368,18.0157244338641,39.8655036159698));
#52569=CARTESIAN_POINT('Ctrl Pts',(21.630429853318,18.01994842679,39.8128790042356));
#52570=CARTESIAN_POINT('Ctrl Pts',(21.6869551031147,18.024172419716,39.7572423111346));
#52571=CARTESIAN_POINT('Ctrl Pts',(21.740561669731,18.028396412642,39.6988857103506));
#52572=CARTESIAN_POINT('Ctrl Pts',(21.794151089076,18.0326190544284,39.6405477762436));
#52573=CARTESIAN_POINT('Ctrl Pts',(21.8448233623029,18.0368416962148,39.5794920071253));
#52574=CARTESIAN_POINT('Ctrl Pts',(21.8923007103463,18.0410643380012,39.5160467727172));
#52575=CARTESIAN_POINT('Ctrl Pts',(21.9397776538033,18.0452869438037,39.4526020789686));
#52576=CARTESIAN_POINT('Ctrl Pts',(21.9840594464951,18.0495095496061,39.3867683365935));
#52577=CARTESIAN_POINT('Ctrl Pts',(22.0249100909219,18.0537321554085,39.3189050679124));
#52578=CARTESIAN_POINT('Ctrl Pts',(22.0658013560714,18.0579589600505,39.2509743179208));
#52579=CARTESIAN_POINT('Ctrl Pts',(22.1032544154758,18.0621857646924,39.1810104130094));
#52580=CARTESIAN_POINT('Ctrl Pts',(22.1370782727308,18.0664125693344,39.1093992753722));
#52581=CARTESIAN_POINT('Ctrl Pts',(22.1709185204344,18.0706414222118,39.0377534362324));
#52582=CARTESIAN_POINT('Ctrl Pts',(22.2011258837041,18.0748702750892,38.9644592081811));
#52583=CARTESIAN_POINT('Ctrl Pts',(22.2275577761299,18.0790991279666,38.8899220182418));
#52584=CARTESIAN_POINT('Ctrl Pts',(22.2540371724587,18.0833355810193,38.8152508686382));
#52585=CARTESIAN_POINT('Ctrl Pts',(22.2767274056021,18.0875720340721,38.7393327438554));
#52586=CARTESIAN_POINT('Ctrl Pts',(22.2955360451978,18.0918084871248,38.6625875097242));
#52587=CARTESIAN_POINT('Ctrl Pts',(22.3126306994114,18.0956588825593,38.5928358813121));
#52588=CARTESIAN_POINT('Ctrl Pts',(22.3265195678366,18.0995092779938,38.522401422398));
#52589=CARTESIAN_POINT('Ctrl Pts',(22.3371704232296,18.1033596734283,38.4516032617607));
#52590=CARTESIAN_POINT('Ctrl Pts',(22.348892470208,18.1075973158057,38.3736846970679));
#52591=CARTESIAN_POINT('Ctrl Pts',(22.3567356866119,18.1118349581831,38.295033031655));
#52592=CARTESIAN_POINT('Ctrl Pts',(22.3606182756164,18.1160726005605,38.216068073672));
#52593=CARTESIAN_POINT('Ctrl Pts',(22.3644952813055,18.1203041490418,38.1372166703975));
#52594=CARTESIAN_POINT('Ctrl Pts',(22.3644229475746,18.1245356975232,38.0580533335972));
#52595=CARTESIAN_POINT('Ctrl Pts',(22.360370904268,18.1287672460045,37.9790056398634));
#52596=CARTESIAN_POINT('Ctrl Pts',(22.3563235411834,18.1329939069305,37.9000492483988));
#52597=CARTESIAN_POINT('Ctrl Pts',(22.3483056271484,18.1372205678565,37.8212087003508));
#52598=CARTESIAN_POINT('Ctrl Pts',(22.3363388257283,18.1414472287825,37.7429127105393));
#52599=CARTESIAN_POINT('Ctrl Pts',(22.3243795781262,18.1456712217084,37.6646661435963));
#52600=CARTESIAN_POINT('Ctrl Pts',(22.3084764614353,18.1498952146343,37.5869639147795));
#52601=CARTESIAN_POINT('Ctrl Pts',(22.2887029593892,18.1541192075602,37.5102295322897));
#52602=CARTESIAN_POINT('Ctrl Pts',(22.2689357823444,18.1583418493466,37.4335196950256));
#52603=CARTESIAN_POINT('Ctrl Pts',(22.2453007953191,18.1625644911329,37.3577775429256));
#52604=CARTESIAN_POINT('Ctrl Pts',(22.2179222520145,18.1667871329193,37.283414839151));
#52605=CARTESIAN_POINT('Ctrl Pts',(22.190543942021,18.1710097387217,37.2090527690711));
#52606=CARTESIAN_POINT('Ctrl Pts',(22.1594223024813,18.175232344524,37.1360705633542));
#52607=CARTESIAN_POINT('Ctrl Pts',(22.1247304631931,18.1794549503264,37.0648618934272));
#52608=CARTESIAN_POINT('Ctrl Pts',(22.0900041273234,18.1836817549683,36.9935824156175));
#52609=CARTESIAN_POINT('Ctrl Pts',(22.0517007061414,18.1879085596101,36.9240804187054));
#52610=CARTESIAN_POINT('Ctrl Pts',(22.010039971138,18.192135364252,36.8567261945462));
#52611=CARTESIAN_POINT('Ctrl Pts',(21.9683590480724,18.1963642171294,36.7893393317102));
#52612=CARTESIAN_POINT('Ctrl Pts',(21.9233178369004,18.2005930700067,36.7241027012231));
#52613=CARTESIAN_POINT('Ctrl Pts',(21.8751788223621,18.204821922884,36.6613566025368));
#52614=CARTESIAN_POINT('Ctrl Pts',(21.8269532914656,18.2090583759367,36.598497735361));
#52615=CARTESIAN_POINT('Ctrl Pts',(21.7756191373549,18.2132948289894,36.5381387014706));
#52616=CARTESIAN_POINT('Ctrl Pts',(21.7214782587364,18.217531282042,36.4805855855903));
#52617=CARTESIAN_POINT('Ctrl Pts',(21.6722711061265,18.2213816774772,36.4282771445646));
#52618=CARTESIAN_POINT('Ctrl Pts',(21.620746126031,18.2252320729123,36.3782862444275));
#52619=CARTESIAN_POINT('Ctrl Pts',(21.5671534828053,18.2290824683475,36.3308136327025));
#52620=CARTESIAN_POINT('Ctrl Pts',(21.5081708510469,18.2333201107254,36.2785665441573));
#52621=CARTESIAN_POINT('Ctrl Pts',(21.446461859556,18.2375577531032,36.2291742280913));
#52622=CARTESIAN_POINT('Ctrl Pts',(21.3823341468647,18.2417953954811,36.1829338177017));
#52623=CARTESIAN_POINT('Ctrl Pts',(21.3182986523408,18.2460269439629,36.1367599028368));
#52624=CARTESIAN_POINT('Ctrl Pts',(21.251851721123,18.2502584924448,36.0937291643045));
#52625=CARTESIAN_POINT('Ctrl Pts',(21.1833355018012,18.2544900409266,36.0540998237752));
#52626=CARTESIAN_POINT('Ctrl Pts',(21.1148984206048,18.2587167018531,36.0145162562285));
#52627=CARTESIAN_POINT('Ctrl Pts',(21.0443972047368,18.2629433627796,35.9783265128687));
#52628=CARTESIAN_POINT('Ctrl Pts',(20.9722032814123,18.2671700237061,35.9457457855418));
#52629=CARTESIAN_POINT('Ctrl Pts',(20.9000549291419,18.2713940166325,35.9131856241852));
#52630=CARTESIAN_POINT('Ctrl Pts',(20.8262164164086,18.2756180095589,35.8842301493618));
#52631=CARTESIAN_POINT('Ctrl Pts',(20.7510830103226,18.2798420024853,35.8590482485103));
#52632=CARTESIAN_POINT('Ctrl Pts',(20.6759736373538,18.2840646442721,35.8338744026587));
#52633=CARTESIAN_POINT('Ctrl Pts',(20.599570637706,18.2882872860589,35.8124718826541));
#52634=CARTESIAN_POINT('Ctrl Pts',(20.5222870618533,18.2925099278458,35.7949605934126));
#52635=CARTESIAN_POINT('Ctrl Pts',(20.445004144586,18.2967325336486,35.7774494533967));
#52636=CARTESIAN_POINT('Ctrl Pts',(20.3668411235336,18.3009551394515,35.763829580409));
#52637=CARTESIAN_POINT('Ctrl Pts',(20.2882224775962,18.3051777452544,35.7541700308189));
#52638=CARTESIAN_POINT('Ctrl Pts',(20.2095256555063,18.3094045498967,35.7445008760465));
#52639=CARTESIAN_POINT('Ctrl Pts',(20.1303727698975,18.3136313545391,35.7387999682103));
#52640=CARTESIAN_POINT('Ctrl Pts',(20.0511940760366,18.3178581591814,35.7370845111433));
#52641=CARTESIAN_POINT('Ctrl Pts',(19.9719770135682,18.3220870120592,35.7353682227959));
#52642=CARTESIAN_POINT('Ctrl Pts',(19.8927345871141,18.3263158649371,35.7376412190946));
#52643=CARTESIAN_POINT('Ctrl Pts',(19.813895142625,18.3305447178149,35.7438685471813));
#52644=CARTESIAN_POINT('Ctrl Pts',(19.7349140063775,18.334781170868,35.7501070671413));
#52645=CARTESIAN_POINT('Ctrl Pts',(19.6563377651814,18.3390176239211,35.7603140584373));
#52646=CARTESIAN_POINT('Ctrl Pts',(19.578587517784,18.3432540769743,35.7744028808212));
#52647=CARTESIAN_POINT('Ctrl Pts',(19.5079224605854,18.347104472405,35.7872078232227));
#52648=CARTESIAN_POINT('Ctrl Pts',(19.4379398374659,18.3509548678358,35.8032186358183));
#52649=CARTESIAN_POINT('Ctrl Pts',(19.3689442223624,18.3548052632666,35.8223347378488));
#52650=CARTESIAN_POINT('Ctrl Pts',(19.2930094910718,18.3590429056437,35.8433734092026));
#52651=CARTESIAN_POINT('Ctrl Pts',(19.2179854814123,18.3632805480208,35.8682530894602));
#52652=CARTESIAN_POINT('Ctrl Pts',(19.1442889073757,18.3675181903979,35.896877450785));
#52653=CARTESIAN_POINT('Ctrl Pts',(19.0706983119047,18.371749738879,35.9254606491549));
#52654=CARTESIAN_POINT('Ctrl Pts',(18.9984317945087,18.37598128736,35.9577776661635));
#52655=CARTESIAN_POINT('Ctrl Pts',(18.9278922126119,18.3802128358411,35.9936820436787));
#52656=CARTESIAN_POINT('Ctrl Pts',(18.85743410588,18.3844394967668,36.0295449506463));
#52657=CARTESIAN_POINT('Ctrl Pts',(18.7886993864146,18.3886661576926,36.068986772376));
#52658=CARTESIAN_POINT('Ctrl Pts',(18.7220707527108,18.3928928186183,36.1118130671834));
#52659=CARTESIAN_POINT('Ctrl Pts',(18.6554841770769,18.3971168115439,36.1546123286989));
#52660=CARTESIAN_POINT('Ctrl Pts',(18.5910014417465,18.4013408044696,36.2007915700013));
#52661=CARTESIAN_POINT('Ctrl Pts',(18.5289793788504,18.4055647973952,36.250111145757));
#52662=CARTESIAN_POINT('Ctrl Pts',(18.4669771551121,18.4097874391813,36.2994149455323));
#52663=CARTESIAN_POINT('Ctrl Pts',(18.4074344074242,18.4140100809674,36.3518567934551));
#52664=CARTESIAN_POINT('Ctrl Pts',(18.3506765581838,18.4182327227535,36.4071554633767));
#52665=CARTESIAN_POINT('Ctrl Pts',(18.2939191926152,18.4224553285556,36.4624536620611));
#52666=CARTESIAN_POINT('Ctrl Pts',(18.2399470130703,18.4266779343577,36.5206083061871));
#52667=CARTESIAN_POINT('Ctrl Pts',(18.1890490076465,18.4309005401598,36.5813009039991));
#52668=CARTESIAN_POINT('Ctrl Pts',(18.1381003906889,18.4351273448015,36.6420538528099));
#52669=CARTESIAN_POINT('Ctrl Pts',(18.0902323558881,18.4393541494431,36.7053494363262));
#52670=CARTESIAN_POINT('Ctrl Pts',(18.045693538211,18.4435809540847,36.7708360920076));
#52671=CARTESIAN_POINT('Ctrl Pts',(18.0011331378032,18.4478098069618,36.836354481375));
#52672=CARTESIAN_POINT('Ctrl Pts',(17.9599054124639,18.4520386598389,36.9040656571423));
#52673=CARTESIAN_POINT('Ctrl Pts',(17.922214205294,18.456267512716,36.9735912676928));
#52674=CARTESIAN_POINT('Ctrl Pts',(17.8844552587651,18.4605039657685,37.0432418310013));
#52675=CARTESIAN_POINT('Ctrl Pts',(17.8502457329749,18.4647404188209,37.1147129209253));
#52676=CARTESIAN_POINT('Ctrl Pts',(17.8197421672373,18.4689768718733,37.1876041300088));
#52677=CARTESIAN_POINT('Ctrl Pts',(17.792018316911,18.4728272673107,37.2538529413159));
#52678=CARTESIAN_POINT('Ctrl Pts',(17.7673552403086,18.4766776627481,37.3212743498509));
#52679=CARTESIAN_POINT('Ctrl Pts',(17.7458343539072,18.4805280581856,37.3895581087274));
#52680=CARTESIAN_POINT('Ctrl Pts',(17.7172495838534,18.4856422837868,37.4802549094767));
#52681=CARTESIAN_POINT('Ctrl Pts',(17.6941206659814,18.490756509388,37.5727480809934));
#52682=CARTESIAN_POINT('Ctrl Pts',(17.6766370864719,18.4958707349892,37.6664389167118));
#52683=CARTESIAN_POINT('Ctrl Pts',(17.659368835943,18.5009219734323,37.7589758495841));
#52684=CARTESIAN_POINT('Ctrl Pts',(17.6476077702664,18.5059732118755,37.8526810990171));
#52685=CARTESIAN_POINT('Ctrl Pts',(17.6414902309452,18.5110244503186,37.9469571622939));
#52686=CARTESIAN_POINT('Ctrl Pts',(17.638230886581,18.5137156836213,37.9971862069121));
#52687=CARTESIAN_POINT('Ctrl Pts',(17.6365727340863,18.516406916924,38.0475769344872));
#52688=CARTESIAN_POINT('Ctrl Pts',(17.6365308155374,18.5190981502267,38.0980365857439));
#52689=CARTESIAN_POINT('',(17.6365304226752,19.3128481502999,38.1014134921557));
#52690=CARTESIAN_POINT('Ctrl Pts',(17.6365308155367,18.5190981502717,38.0980365865869));
#52691=CARTESIAN_POINT('Ctrl Pts',(17.6364653475663,18.523301293328,38.1768439990069));
#52692=CARTESIAN_POINT('Ctrl Pts',(17.6403457991141,18.5275044363842,38.2557159250519));
#52693=CARTESIAN_POINT('Ctrl Pts',(17.6481648313519,18.5317075794405,38.3342259174604));
#52694=CARTESIAN_POINT('Ctrl Pts',(17.6559813183685,18.5359093543058,38.4127103535983));
#52695=CARTESIAN_POINT('Ctrl Pts',(17.6677337940143,18.5401111291712,38.4908326190067));
#52696=CARTESIAN_POINT('Ctrl Pts',(17.6833629476021,18.5443129040365,38.5681700634994));
#52697=CARTESIAN_POINT('Ctrl Pts',(17.6989919989068,18.5485146514038,38.6455070018668));
#52698=CARTESIAN_POINT('Ctrl Pts',(17.7184975824096,18.5527163987711,38.7220586655415));
#52699=CARTESIAN_POINT('Ctrl Pts',(17.7417693239072,18.5569181461385,38.7974128292865));
#52700=CARTESIAN_POINT('Ctrl Pts',(17.7650647959264,18.5611241780866,38.8728438327307));
#52701=CARTESIAN_POINT('Ctrl Pts',(17.7921339562944,18.5653302100348,38.9470744436813));
#52702=CARTESIAN_POINT('Ctrl Pts',(17.8228167847401,18.5695362419829,39.0197084799492));
#52703=CARTESIAN_POINT('Ctrl Pts',(17.8535149226381,18.5737443725657,39.0923787575735));
#52704=CARTESIAN_POINT('Ctrl Pts',(17.8878301126272,18.5779525031484,39.1634504473205));
#52705=CARTESIAN_POINT('Ctrl Pts',(17.9255556060353,18.5821606337312,39.2325506157556));
#52706=CARTESIAN_POINT('Ctrl Pts',(17.9633505311331,18.5863765091461,39.3017779592391));
#52707=CARTESIAN_POINT('Ctrl Pts',(18.0045680504769,18.5905923845611,39.3690261279718));
#52708=CARTESIAN_POINT('Ctrl Pts',(18.0489573443338,18.5948082599761,39.4339501477458));
#52709=CARTESIAN_POINT('Ctrl Pts',(18.0891173410826,18.5986224576856,39.4926883748382));
#52710=CARTESIAN_POINT('Ctrl Pts',(18.131872794144,18.6024366553952,39.5495244326457));
#52711=CARTESIAN_POINT('Ctrl Pts',(18.177010871039,18.6062508531047,39.6042277342843));
#52712=CARTESIAN_POINT('Ctrl Pts',(18.2271600877748,18.6104884954849,39.6650040880581));
#52713=CARTESIAN_POINT('Ctrl Pts',(18.2804460833656,18.6147261378651,39.7233839064688));
#52714=CARTESIAN_POINT('Ctrl Pts',(18.3366111180252,18.6189637802453,39.7790258688366));
#52715=CARTESIAN_POINT('Ctrl Pts',(18.392695385161,18.6231953287294,39.8345878158792));
#52716=CARTESIAN_POINT('Ctrl Pts',(18.4516501391006,18.6274268772136,39.8874193984905));
#52717=CARTESIAN_POINT('Ctrl Pts',(18.5131775036553,18.6316584256977,39.9372123734787));
#52718=CARTESIAN_POINT('Ctrl Pts',(18.5746338024049,18.6358850866265,39.9869478362059));
#52719=CARTESIAN_POINT('Ctrl Pts',(18.6386564442277,18.6401117475553,40.033651372513));
#52720=CARTESIAN_POINT('Ctrl Pts',(18.7049119446151,18.6443384084841,40.0770526977547));
#52721=CARTESIAN_POINT('Ctrl Pts',(18.7711256224658,18.6485624014127,40.1204266267274));
#52722=CARTESIAN_POINT('Ctrl Pts',(18.8395689701737,18.6527863943414,40.1605022258573));
#52723=CARTESIAN_POINT('Ctrl Pts',(18.9098777588544,18.6570103872701,40.1970512488396));
#52724=CARTESIAN_POINT('Ctrl Pts',(18.9801640576806,18.6612330290593,40.2335885807912));
#52725=CARTESIAN_POINT('Ctrl Pts',(19.0523141969129,18.6654556708484,40.2666013606293));
#52726=CARTESIAN_POINT('Ctrl Pts',(19.1259387702036,18.6696783126375,40.2959069669425));
#52727=CARTESIAN_POINT('Ctrl Pts',(19.1995627160894,18.6739009184426,40.3252123235229));
#52728=CARTESIAN_POINT('Ctrl Pts',(19.2746606349845,18.6781235242478,40.3508103973575));
#52729=CARTESIAN_POINT('Ctrl Pts',(19.3508239309417,18.6823461300529,40.3725670226117));
#52730=CARTESIAN_POINT('Ctrl Pts',(19.4270629615204,18.6865729346975,40.394345282037));
#52731=CARTESIAN_POINT('Ctrl Pts',(19.5043690334875,18.6907997393421,40.4122743337015));
#52732=CARTESIAN_POINT('Ctrl Pts',(19.582319788744,18.6950265439867,40.426270337262));
#52733=CARTESIAN_POINT('Ctrl Pts',(19.6603083175704,18.6992553968668,40.4402731230406));
#52734=CARTESIAN_POINT('Ctrl Pts',(19.7389416864538,18.7034842497468,40.4503390043688));
#52735=CARTESIAN_POINT('Ctrl Pts',(19.8177913202494,18.7077131026269,40.4564359609214));
#52736=CARTESIAN_POINT('Ctrl Pts',(19.8967826641148,18.7119495556822,40.4625438750409));
#52737=CARTESIAN_POINT('Ctrl Pts',(19.9759905797868,18.7161860087375,40.464668599304));
#52738=CARTESIAN_POINT('Ctrl Pts',(20.0549856210584,18.7204224617929,40.4628302991067));
#52739=CARTESIAN_POINT('Ctrl Pts',(20.1267820366863,18.7242728572032,40.4611595187276));
#52740=CARTESIAN_POINT('Ctrl Pts',(20.1984023756985,18.7281232526135,40.4562157707697));
#52741=CARTESIAN_POINT('Ctrl Pts',(20.2695301359815,18.7319736480237,40.4480510954189));
#52742=CARTESIAN_POINT('Ctrl Pts',(20.347811449674,18.7362112903979,40.4390652717435));
#52743=CARTESIAN_POINT('Ctrl Pts',(20.4257898477129,18.740448932772,40.4261435866177));
#52744=CARTESIAN_POINT('Ctrl Pts',(20.503038710321,18.7446865751462,40.4093164566206));
#52745=CARTESIAN_POINT('Ctrl Pts',(20.5801764860331,18.7489181236243,40.3925135246967));
#52746=CARTESIAN_POINT('Ctrl Pts',(20.6565863554827,18.7531496721024,40.3718164000696));
#52747=CARTESIAN_POINT('Ctrl Pts',(20.7318475988545,18.7573812205805,40.3473071736972));
#52748=CARTESIAN_POINT('Ctrl Pts',(20.8070219134126,18.7616078815033,40.3228262561578));
#52749=CARTESIAN_POINT('Ctrl Pts',(20.8810497948919,18.7658345424261,40.2945421313271));
#52750=CARTESIAN_POINT('Ctrl Pts',(20.9535229827976,18.7700612033489,40.2625874230136));
#52751=CARTESIAN_POINT('Ctrl Pts',(21.025950423369,18.7742851962716,40.2306528855077));
#52752=CARTESIAN_POINT('Ctrl Pts',(21.0968246904719,18.7785091891943,40.1950525521099));
#52753=CARTESIAN_POINT('Ctrl Pts',(21.1657560529569,18.7827331821171,40.1559677200516));
#52754=CARTESIAN_POINT('Ctrl Pts',(21.2346653661889,18.7869558239003,40.1168953901595));
#52755=CARTESIAN_POINT('Ctrl Pts',(21.3016326014543,18.7911784656835,40.0743410060243));
#52756=CARTESIAN_POINT('Ctrl Pts',(21.3662925958599,18.7954011074667,40.028531820686));
#52757=CARTESIAN_POINT('Ctrl Pts',(21.4309520392545,18.7996237132659,39.9827230257183));
#52758=CARTESIAN_POINT('Ctrl Pts',(21.493303899202,18.8038463190652,39.9336597568539));
#52759=CARTESIAN_POINT('Ctrl Pts',(21.5530132150415,18.8080689248644,39.881611740758));
#52760=CARTESIAN_POINT('Ctrl Pts',(21.6127819041329,18.8122957295033,39.8295119695894));
#52761=CARTESIAN_POINT('Ctrl Pts',(21.6699024461431,18.8165225341421,39.7744218314421));
#52762=CARTESIAN_POINT('Ctrl Pts',(21.7240746056064,18.8207493387809,39.7166499915576));
#52763=CARTESIAN_POINT('Ctrl Pts',(21.7782730159494,18.8249781916552,39.6588501564514));
#52764=CARTESIAN_POINT('Ctrl Pts',(21.8295198941157,18.8292070445296,39.5983663889541));
#52765=CARTESIAN_POINT('Ctrl Pts',(21.8775550906141,18.8334358974039,39.5355407770625));
#52766=CARTESIAN_POINT('Ctrl Pts',(21.9256766168881,18.8376723504536,39.4726022537773));
#52767=CARTESIAN_POINT('Ctrl Pts',(21.9705746620337,18.8419088035034,39.4073138636635));
#52768=CARTESIAN_POINT('Ctrl Pts',(22.0120323793199,18.8461452565531,39.3400468319658));
#52769=CARTESIAN_POINT('Ctrl Pts',(22.0497121564072,18.8499956520164,39.2789096800526));
#52770=CARTESIAN_POINT('Ctrl Pts',(22.0845505022411,18.8538460474796,39.2161386405155));
#52771=CARTESIAN_POINT('Ctrl Pts',(22.1164187882959,18.8576964429429,39.1520275440539));
#52772=CARTESIAN_POINT('Ctrl Pts',(22.1514921724919,18.8619340853174,39.0814685841664));
#52773=CARTESIAN_POINT('Ctrl Pts',(22.1830990023349,18.866171727692,39.0090213011705));
#52774=CARTESIAN_POINT('Ctrl Pts',(22.211032569004,18.8704093700665,38.9350601293942));
#52775=CARTESIAN_POINT('Ctrl Pts',(22.2389259661075,18.8746409185449,38.8612053166863));
#52776=CARTESIAN_POINT('Ctrl Pts',(22.2631564259306,18.8788724670234,38.7858413734966));
#52777=CARTESIAN_POINT('Ctrl Pts',(22.2835637991729,18.8831040155018,38.7093659130664));
#52778=CARTESIAN_POINT('Ctrl Pts',(22.3039476013352,18.8873306764248,38.6329787839059));
#52779=CARTESIAN_POINT('Ctrl Pts',(22.3205169719132,18.8915573373479,38.5554831394366));
#52780=CARTESIAN_POINT('Ctrl Pts',(22.3331609340279,18.8957839982709,38.4772936480062));
#52781=CARTESIAN_POINT('Ctrl Pts',(22.3457969148797,18.9000079911938,38.3991535122201));
#52782=CARTESIAN_POINT('Ctrl Pts',(22.3545123308703,18.9042319841167,38.3203208603617));
#52783=CARTESIAN_POINT('Ctrl Pts',(22.3592471218585,18.9084559770396,38.2412213117851));
#52784=CARTESIAN_POINT('Ctrl Pts',(22.3639803983169,18.912678618823,38.1621470649863));
#52785=CARTESIAN_POINT('Ctrl Pts',(22.3647355502911,18.9169012606063,38.0828065586014));
#52786=CARTESIAN_POINT('Ctrl Pts',(22.3615044418532,18.9211239023896,38.0036298178498));
#52787=CARTESIAN_POINT('Ctrl Pts',(22.3582733609497,18.925346508189,37.924453751817));
#52788=CARTESIAN_POINT('Ctrl Pts',(22.3510561077185,18.9295691139883,37.8454419169673));
#52789=CARTESIAN_POINT('Ctrl Pts',(22.3398966161269,18.9337917197877,37.7670221227501));
#52790=CARTESIAN_POINT('Ctrl Pts',(22.3287260278533,18.9380185244265,37.6885243501131));
#52791=CARTESIAN_POINT('Ctrl Pts',(22.3136054370985,18.9422453290653,37.610620259233));
#52792=CARTESIAN_POINT('Ctrl Pts',(22.2946303442971,18.9464721337041,37.5337297253689));
#52793=CARTESIAN_POINT('Ctrl Pts',(22.2756460564984,18.9507009865784,37.4568019316996));
#52794=CARTESIAN_POINT('Ctrl Pts',(22.2528036809747,18.9549298394526,37.3808891229445));
#52795=CARTESIAN_POINT('Ctrl Pts',(22.2262485756469,18.9591586923269,37.306395740731));
#52796=CARTESIAN_POINT('Ctrl Pts',(22.1996457449755,18.9633951453765,37.2317684775848));
#52797=CARTESIAN_POINT('Ctrl Pts',(22.1693170318744,18.9676315984261,37.1585661722692));
#52798=CARTESIAN_POINT('Ctrl Pts',(22.1354558077887,18.9718680514757,37.0871728015691));
#52799=CARTESIAN_POINT('Ctrl Pts',(22.1046802740975,18.9757184469378,37.0222853338347));
#52800=CARTESIAN_POINT('Ctrl Pts',(22.070987433048,18.9795688423999,36.9588920675937));
#52801=CARTESIAN_POINT('Ctrl Pts',(22.0345537526132,18.9834192378619,36.8972608476367));
#52802=CARTESIAN_POINT('Ctrl Pts',(21.9944558171186,18.9876568802583,36.8294311732038));
#52803=CARTESIAN_POINT('Ctrl Pts',(21.9508868598386,18.9918945226547,36.763481597527));
#52804=CARTESIAN_POINT('Ctrl Pts',(21.9040484626433,18.996132165051,36.6997893398471));
#52805=CARTESIAN_POINT('Ctrl Pts',(21.8572774209003,19.0003637135514,36.6361886741322));
#52806=CARTESIAN_POINT('Ctrl Pts',(21.8072465515749,19.0045952620518,36.5748392544678));
#52807=CARTESIAN_POINT('Ctrl Pts',(21.7542022245776,19.0088268105522,36.5160918599278));
#52808=CARTESIAN_POINT('Ctrl Pts',(21.7012191652426,19.0130534714972,36.4574123202506));
#52809=CARTESIAN_POINT('Ctrl Pts',(21.6452298776808,19.0172801324422,36.4013291793598));
#52810=CARTESIAN_POINT('Ctrl Pts',(21.5865218050746,19.0215067933872,36.3481612508787));
#52811=CARTESIAN_POINT('Ctrl Pts',(21.5278507908333,19.0257307863321,36.295026883651));
#52812=CARTESIAN_POINT('Ctrl Pts',(21.4664647445317,19.029954779277,36.2448043901422));
#52813=CARTESIAN_POINT('Ctrl Pts',(21.4026880115855,19.0341787722219,36.1977758325964));
#52814=CARTESIAN_POINT('Ctrl Pts',(21.3389316790685,19.0384014140273,36.1507623181975));
#52815=CARTESIAN_POINT('Ctrl Pts',(21.2727865554974,19.0426240558326,36.1069409889715));
#52816=CARTESIAN_POINT('Ctrl Pts',(21.2046089464197,19.0468466976379,36.066552747892));
#52817=CARTESIAN_POINT('Ctrl Pts',(21.13643191833,19.0510693034592,36.0261648509883));
#52818=CARTESIAN_POINT('Ctrl Pts',(21.0662228432157,19.0552919092805,35.9892102217553));
#52819=CARTESIAN_POINT('Ctrl Pts',(20.9943645113807,19.0595145151017,35.9558848772963));
#52820=CARTESIAN_POINT('Ctrl Pts',(20.9224347256623,19.0637413197623,35.9225263950618));
#52821=CARTESIAN_POINT('Ctrl Pts',(20.8488528336226,19.0679681244228,35.8928046039927));
#52822=CARTESIAN_POINT('Ctrl Pts',(20.7740230392906,19.0721949290833,35.8668679448928));
#52823=CARTESIAN_POINT('Ctrl Pts',(20.6991569837533,19.0764237819792,35.840918717343));
#52824=CARTESIAN_POINT('Ctrl Pts',(20.623042271929,19.0806526348751,35.8187584069275));
#52825=CARTESIAN_POINT('Ctrl Pts',(20.5460973002749,19.084881487771,35.8004852295468));
#52826=CARTESIAN_POINT('Ctrl Pts',(20.4690140416526,19.0891179408419,35.7821792112638));
#52827=CARTESIAN_POINT('Ctrl Pts',(20.3910980037781,19.0933543939127,35.7677743702033));
#52828=CARTESIAN_POINT('Ctrl Pts',(20.3127765512825,19.0975908469836,35.7573175055361));
#52829=CARTESIAN_POINT('Ctrl Pts',(20.2415923448588,19.1014412422494,35.7478135498598));
#52830=CARTESIAN_POINT('Ctrl Pts',(20.1700735816283,19.1052916375152,35.741570175401));
#52831=CARTESIAN_POINT('Ctrl Pts',(20.0985410056413,19.109142032781,35.7385851463355));
#52832=CARTESIAN_POINT('Ctrl Pts',(20.019814160111,19.1133796751298,35.7352999029496));
#52833=CARTESIAN_POINT('Ctrl Pts',(19.9407750679908,19.1176173174786,35.7359497917051));
#52834=CARTESIAN_POINT('Ctrl Pts',(19.8618498944411,19.1218549598274,35.7405710459448));
#52835=CARTESIAN_POINT('Ctrl Pts',(19.7830382183881,19.1260865082802,35.7451856546395));
#52836=CARTESIAN_POINT('Ctrl Pts',(19.7043405996813,19.130318056733,35.7537602601678));
#52837=CARTESIAN_POINT('Ctrl Pts',(19.6261854034043,19.1345496051858,35.7662791323143));
#52838=CARTESIAN_POINT('Ctrl Pts',(19.5481204785333,19.1387762660835,35.7787835448183));
#52839=CARTESIAN_POINT('Ctrl Pts',(19.4705971915837,19.1430029269812,35.7952230967783));
#52840=CARTESIAN_POINT('Ctrl Pts',(19.3940394505008,19.1472295878789,35.815530203012));
#52841=CARTESIAN_POINT('Ctrl Pts',(19.3175300350472,19.1514535807767,35.835824490768));
#52842=CARTESIAN_POINT('Ctrl Pts',(19.2419854076235,19.1556775736744,35.8599813671734));
#52843=CARTESIAN_POINT('Ctrl Pts',(19.1678187338312,19.1599015665722,35.8878822858768));
#52844=CARTESIAN_POINT('Ctrl Pts',(19.0936757839217,19.1641242083306,35.9157742798422));
#52845=CARTESIAN_POINT('Ctrl Pts',(19.0209103508,19.168346850089,35.9474077729394));
#52846=CARTESIAN_POINT('Ctrl Pts',(18.949918469925,19.1725694918474,35.982615004045));
#52847=CARTESIAN_POINT('Ctrl Pts',(18.8789271940157,19.176792097622,36.017821935128));
#52848=CARTESIAN_POINT('Ctrl Pts',(18.8097098596318,19.1810147033967,36.0566023341128));
#52849=CARTESIAN_POINT('Ctrl Pts',(18.7426392655245,19.1852373091714,36.0987417896985));
#52850=CARTESIAN_POINT('Ctrl Pts',(18.6755019783107,19.1894641137861,36.1409231475699));
#52851=CARTESIAN_POINT('Ctrl Pts',(18.6105160932173,19.1936909184008,36.1864699840429));
#52852=CARTESIAN_POINT('Ctrl Pts',(18.548026155031,19.1979177230155,36.2351240270662));
#52853=CARTESIAN_POINT('Ctrl Pts',(18.4855059353114,19.2021465758659,36.2838016469895));
#52854=CARTESIAN_POINT('Ctrl Pts',(18.4254844273257,19.2063754287164,36.3355891663651));
#52855=CARTESIAN_POINT('Ctrl Pts',(18.3682717692599,19.2106042815668,36.3901890683746));
#52856=CARTESIAN_POINT('Ctrl Pts',(18.3109562874994,19.2148407345933,36.4448870983832));
#52857=CARTESIAN_POINT('Ctrl Pts',(18.2564600654632,19.2190771876198,36.5024072692392));
#52858=CARTESIAN_POINT('Ctrl Pts',(18.2050549912046,19.2233136406463,36.5624165530611));
#52859=CARTESIAN_POINT('Ctrl Pts',(18.1583343324713,19.2271640363309,36.6169573413142));
#52860=CARTESIAN_POINT('Ctrl Pts',(18.1141667590309,19.2310144320155,36.6735536290899));
#52861=CARTESIAN_POINT('Ctrl Pts',(18.0727249877601,19.2348648277001,36.7319351374677));
#52862=CARTESIAN_POINT('Ctrl Pts',(18.0266912746906,19.2391418652087,36.7967855896276));
#52863=CARTESIAN_POINT('Ctrl Pts',(17.9838497684247,19.2434189027173,36.8640810570083));
#52864=CARTESIAN_POINT('Ctrl Pts',(17.9444667914954,19.2476959402259,36.9334779600732));
#52865=CARTESIAN_POINT('Ctrl Pts',(17.9051427866996,19.2519665732916,37.0027709481031));
#52866=CARTESIAN_POINT('Ctrl Pts',(17.8692672489419,19.2562372063573,37.0741587279191));
#52867=CARTESIAN_POINT('Ctrl Pts',(17.8370642044437,19.260507839423,37.1472675164553));
#52868=CARTESIAN_POINT('Ctrl Pts',(17.8041745185864,19.2648695319937,37.2219351488433));
#52869=CARTESIAN_POINT('Ctrl Pts',(17.7751160414248,19.2692312245644,37.2983976442449));
#52870=CARTESIAN_POINT('Ctrl Pts',(17.7500787937588,19.2735929171352,37.376228622695));
#52871=CARTESIAN_POINT('Ctrl Pts',(17.7256186167874,19.2778540792884,37.4522657147962));
#52872=CARTESIAN_POINT('Ctrl Pts',(17.7049964412684,19.2821152414415,37.5296084235428));
#52873=CARTESIAN_POINT('Ctrl Pts',(17.688340841097,19.2863764035947,37.6078390771711));
#52874=CARTESIAN_POINT('Ctrl Pts',(17.6710958262146,19.2907883613742,37.688838186912));
#52875=CARTESIAN_POINT('Ctrl Pts',(17.6581035610096,19.2952003191537,37.7707887872257));
#52876=CARTESIAN_POINT('Ctrl Pts',(17.6494498003634,19.2996122769332,37.8532122371583));
#52877=CARTESIAN_POINT('Ctrl Pts',(17.6407960397172,19.3040242347127,37.9356356870909));
#52878=CARTESIAN_POINT('Ctrl Pts',(17.6364808544133,19.3084361924922,38.0185314454336));
#52879=CARTESIAN_POINT('Ctrl Pts',(17.6365304226749,19.3128481502717,38.1014134916261));
#52880=CARTESIAN_POINT('',(17.6365301782972,20.106598150223,38.1009180413976));
#52881=CARTESIAN_POINT('Ctrl Pts',(17.6365304226752,19.3128481502999,38.1014134921557));
#52882=CARTESIAN_POINT('Ctrl Pts',(17.6365835982443,19.3175811845135,38.1903272079986));
#52883=CARTESIAN_POINT('Ctrl Pts',(17.6416582714512,19.3223142187271,38.2790563289598));
#52884=CARTESIAN_POINT('Ctrl Pts',(17.6516677115378,19.3270472529406,38.3670690994213));
#52885=CARTESIAN_POINT('Ctrl Pts',(17.6617198026594,19.3318004549964,38.4554568994273));
#52886=CARTESIAN_POINT('Ctrl Pts',(17.6767486737287,19.3365536570522,38.5431219950087));
#52887=CARTESIAN_POINT('Ctrl Pts',(17.6966167680631,19.3413068591079,38.6295433199767));
#52888=CARTESIAN_POINT('Ctrl Pts',(17.7165895218556,19.3460850996774,38.7164198878526));
#52889=CARTESIAN_POINT('Ctrl Pts',(17.7414524899748,19.3508633402468,38.8020393177264));
#52890=CARTESIAN_POINT('Ctrl Pts',(17.7710177346128,19.3556415808162,38.8858934415614));
#52891=CARTESIAN_POINT('Ctrl Pts',(17.7812189048112,19.3572902614172,38.9148264065869));
#52892=CARTESIAN_POINT('Ctrl Pts',(17.791979480223,19.3589389420181,38.943549408275));
#52893=CARTESIAN_POINT('Ctrl Pts',(17.803290462004,19.3605876226191,38.9720422275196));
#52894=CARTESIAN_POINT('Ctrl Pts',(17.8323633443828,19.3648252651262,39.0452779906548));
#52895=CARTESIAN_POINT('Ctrl Pts',(17.8651571983814,19.3690629076334,39.1171957494667));
#52896=CARTESIAN_POINT('Ctrl Pts',(17.9015314954163,19.3733005501405,39.1873915468544));
#52897=CARTESIAN_POINT('Ctrl Pts',(17.9378534847901,19.377532098752,39.2574863999413));
#52898=CARTESIAN_POINT('Ctrl Pts',(17.9777454782337,19.3817636473636,39.325863796429));
#52899=CARTESIAN_POINT('Ctrl Pts',(18.0210185951564,19.3859951959751,39.3921389399687));
#52900=CARTESIAN_POINT('Ctrl Pts',(18.0642417304364,19.3902218570314,39.4583375338909));
#52901=CARTESIAN_POINT('Ctrl Pts',(18.110837973413,19.3944485180877,39.5224383097033));
#52902=CARTESIAN_POINT('Ctrl Pts',(18.1605729027309,19.3986751791439,39.584081667137));
#52903=CARTESIAN_POINT('Ctrl Pts',(18.2102764378123,19.4028991722001,39.6456861133635));
#52904=CARTESIAN_POINT('Ctrl Pts',(18.2631144331148,19.4071231652563,39.7048358562903));
#52905=CARTESIAN_POINT('Ctrl Pts',(18.3188103033576,19.4113471583124,39.7612018675656));
#52906=CARTESIAN_POINT('Ctrl Pts',(18.3744883580162,19.4155698002288,39.8175498488969));
#52907=CARTESIAN_POINT('Ctrl Pts',(18.4330221430347,19.4197924421453,39.8711155336049));
#52908=CARTESIAN_POINT('Ctrl Pts',(18.49409710648,19.4240150840617,39.9216055874387));
#52909=CARTESIAN_POINT('Ctrl Pts',(18.5551715494589,19.4282376899937,39.9720952110084));
#52910=CARTESIAN_POINT('Ctrl Pts',(18.6187867655975,19.4324602959258,40.0195089582365));
#52911=CARTESIAN_POINT('Ctrl Pts',(18.6845950662279,19.4366829018579,40.0635937209891));
#52912=CARTESIAN_POINT('Ctrl Pts',(18.7504688047415,19.4409097066279,40.1077223203631));
#52913=CARTESIAN_POINT('Ctrl Pts',(18.8185395934184,19.445136511398,40.1485150615237));
#52914=CARTESIAN_POINT('Ctrl Pts',(18.8884311983215,19.4493633161681,40.1857625080615));
#52915=CARTESIAN_POINT('Ctrl Pts',(18.9583566714606,19.453592169173,40.2230280040533));
#52916=CARTESIAN_POINT('Ctrl Pts',(19.0301042937365,19.4578210221779,40.2567445833614));
#52917=CARTESIAN_POINT('Ctrl Pts',(19.1032760080623,19.4620498751829,40.2867502196601));
#52918=CARTESIAN_POINT('Ctrl Pts',(19.1765792279461,19.4662863283606,40.3168097826431));
#52919=CARTESIAN_POINT('Ctrl Pts',(19.2513112106449,19.4705227815383,40.3431449203859));
#52920=CARTESIAN_POINT('Ctrl Pts',(19.3270570515768,19.4747592347161,40.3656430056537));
#52921=CARTESIAN_POINT('Ctrl Pts',(19.395900336271,19.4786096289901,40.3860908886016));
#52922=CARTESIAN_POINT('Ctrl Pts',(19.4655806860639,19.4824600232642,40.4033697608079));
#52923=CARTESIAN_POINT('Ctrl Pts',(19.5357809044098,19.4863104175383,40.4174319994747));
#52924=CARTESIAN_POINT('Ctrl Pts',(19.6130414087937,19.490548059681,40.4329085275791));
#52925=CARTESIAN_POINT('Ctrl Pts',(19.6912217391311,19.4947857018238,40.4445462172815));
#52926=CARTESIAN_POINT('Ctrl Pts',(19.7699065342695,19.4990233439665,40.4522430652312));
#52927=CARTESIAN_POINT('Ctrl Pts',(19.8484781775839,19.5032548922135,40.4599288448113));
#52928=CARTESIAN_POINT('Ctrl Pts',(19.9275523823503,19.5074864404605,40.463684991685));
#52929=CARTESIAN_POINT('Ctrl Pts',(20.0067035410302,19.5117179887075,40.4634604933101));
#52930=CARTESIAN_POINT('Ctrl Pts',(20.0857632779596,19.5159446494006,40.463236254237));
#52931=CARTESIAN_POINT('Ctrl Pts',(20.1648993257691,19.5201713100938,40.4590405081321));
#52932=CARTESIAN_POINT('Ctrl Pts',(20.2436824236344,19.5243979707869,40.4508741602459));
#52933=CARTESIAN_POINT('Ctrl Pts',(20.3224157911697,19.5286219634811,40.4427129672112));
#52934=CARTESIAN_POINT('Ctrl Pts',(20.4007961859249,19.5328459561752,40.4305861954623));
#52935=CARTESIAN_POINT('Ctrl Pts',(20.4783970415405,19.5370699488693,40.4145467615811));
#52936=CARTESIAN_POINT('Ctrl Pts',(20.5559730747929,19.5412925904252,40.3985124582702));
#52937=CARTESIAN_POINT('Ctrl Pts',(20.6327696053325,19.5455152319811,40.3785680729797));
#52938=CARTESIAN_POINT('Ctrl Pts',(20.7083693428251,19.549737873537,40.3548178008534));
#52939=CARTESIAN_POINT('Ctrl Pts',(20.783968436111,19.5539604791105,40.33106773111));
#52940=CARTESIAN_POINT('Ctrl Pts',(20.858370309833,19.5581830846841,40.3035119808758));
#52941=CARTESIAN_POINT('Ctrl Pts',(20.9311733805399,19.5624056902577,40.2723044391323));
#52942=CARTESIAN_POINT('Ctrl Pts',(21.0040488446322,19.5666324946749,40.2410658654615));
#52943=CARTESIAN_POINT('Ctrl Pts',(21.0753218982057,19.5708592990922,40.2061684319789));
#52944=CARTESIAN_POINT('Ctrl Pts',(21.1446120543996,19.5750861035094,40.1678137454382));
#52945=CARTESIAN_POINT('Ctrl Pts',(21.2139357874224,19.579314956164,40.12944047287));
#52946=CARTESIAN_POINT('Ctrl Pts',(21.2812743101845,19.5835438088187,40.087606857488));
#52947=CARTESIAN_POINT('Ctrl Pts',(21.346275027494,19.5877726614733,40.0425586197709));
#52948=CARTESIAN_POINT('Ctrl Pts',(21.4113925654325,19.5920091143091,39.9974294204323));
#52949=CARTESIAN_POINT('Ctrl Pts',(21.4741635305669,19.5962455671449,39.949074341736));
#52950=CARTESIAN_POINT('Ctrl Pts',(21.5342675963127,19.6004820199807,39.8977801266575));
#52951=CARTESIAN_POINT('Ctrl Pts',(21.5888945573553,19.6043324174729,39.8511602008002));
#52952=CARTESIAN_POINT('Ctrl Pts',(21.6413187786523,19.6081828149651,39.8021130789163));
#52953=CARTESIAN_POINT('Ctrl Pts',(21.691327649107,19.6120332124573,39.750878924775));
#52954=CARTESIAN_POINT('Ctrl Pts',(21.7463660469705,19.6162708548432,39.6944920131293));
#52955=CARTESIAN_POINT('Ctrl Pts',(21.7986848613811,19.6205084972291,39.6352438729319));
#52956=CARTESIAN_POINT('Ctrl Pts',(21.8479724291805,19.624746139615,39.5734274131726));
#52957=CARTESIAN_POINT('Ctrl Pts',(21.8971891194963,19.6289776881025,39.5116998479422));
#52958=CARTESIAN_POINT('Ctrl Pts',(21.9433829300499,19.63320923659,39.447411661293));
#52959=CARTESIAN_POINT('Ctrl Pts',(21.9862793947481,19.6374407850776,39.3808921136844));
#52960=CARTESIAN_POINT('Ctrl Pts',(22.0291263128098,19.6416674460062,39.3144493980451));
#52961=CARTESIAN_POINT('Ctrl Pts',(22.068683200752,19.6458941069349,39.2457808351275));
#52962=CARTESIAN_POINT('Ctrl Pts',(22.104717156022,19.6501207678636,39.1752470107128));
#52963=CARTESIAN_POINT('Ctrl Pts',(22.1407283655185,19.65434476079,39.1047577094813));
#52964=CARTESIAN_POINT('Ctrl Pts',(22.1732208436059,19.6585687537165,39.0324059001456));
#52965=CARTESIAN_POINT('Ctrl Pts',(22.202006785044,19.662792746643,38.9585782198032));
#52966=CARTESIAN_POINT('Ctrl Pts',(22.2307835186341,19.6670153884278,38.8847741549488));
#52967=CARTESIAN_POINT('Ctrl Pts',(22.255855899816,19.6712380302126,38.8094955930018));
#52968=CARTESIAN_POINT('Ctrl Pts',(22.2770841885425,19.6754606719974,38.7331493024475));
#52969=CARTESIAN_POINT('Ctrl Pts',(22.298312296358,19.6796832777962,38.656803662529));
#52970=CARTESIAN_POINT('Ctrl Pts',(22.3156962526527,19.6839058835949,38.5793907641174));
#52971=CARTESIAN_POINT('Ctrl Pts',(22.329146553743,19.6881284893937,38.5013312498262));
#52972=CARTESIAN_POINT('Ctrl Pts',(22.3426102294212,19.6923552940287,38.4231941154261));
#52973=CARTESIAN_POINT('Ctrl Pts',(22.3521323568461,19.6965820986637,38.3444095438386));
#52974=CARTESIAN_POINT('Ctrl Pts',(22.35767494485,19.7008089032988,38.2654064549122));
#52975=CARTESIAN_POINT('Ctrl Pts',(22.3632202186926,19.7050377561675,38.1863650825061));
#52976=CARTESIAN_POINT('Ctrl Pts',(22.3647821022416,19.7092666090362,38.1071054510986));
#52977=CARTESIAN_POINT('Ctrl Pts',(22.3623747923296,19.713495461905,38.0280570957931));
#52978=CARTESIAN_POINT('Ctrl Pts',(22.3599631559557,19.7177319149462,37.9488666733233));
#52979=CARTESIAN_POINT('Ctrl Pts',(22.3535681106041,19.7219683679874,37.8698887540043));
#52980=CARTESIAN_POINT('Ctrl Pts',(22.3432558305,19.7262048210286,37.7915481338562));
#52981=CARTESIAN_POINT('Ctrl Pts',(22.3338832832305,19.7300552164779,37.720346502592));
#52982=CARTESIAN_POINT('Ctrl Pts',(22.321275613787,19.7339056119271,37.6496714687195));
#52983=CARTESIAN_POINT('Ctrl Pts',(22.3055185558231,19.7377560073764,37.5798321139715));
#52984=CARTESIAN_POINT('Ctrl Pts',(22.2881767552031,19.741993650618,37.5029687700501));
#52985=CARTESIAN_POINT('Ctrl Pts',(22.2669543952425,19.7462312938597,37.4268293289515));
#52986=CARTESIAN_POINT('Ctrl Pts',(22.2419275386174,19.7504689371013,37.3518346756972));
#52987=CARTESIAN_POINT('Ctrl Pts',(22.2169366715643,19.7547004864507,37.2769478676078));
#52988=CARTESIAN_POINT('Ctrl Pts',(22.1881523199338,19.7589320358002,37.2032030190581));
#52989=CARTESIAN_POINT('Ctrl Pts',(22.1557012881523,19.7631635851496,37.1310095990369));
#52990=CARTESIAN_POINT('Ctrl Pts',(22.1232877381884,19.7673902469453,37.0588995643644));
#52991=CARTESIAN_POINT('Ctrl Pts',(22.0872161155294,19.771616908741,36.9883378225812));
#52992=CARTESIAN_POINT('Ctrl Pts',(22.0476621269062,19.7758435705367,36.9197160278416));
#52993=CARTESIAN_POINT('Ctrl Pts',(22.0081331059825,19.7800675643329,36.8511375492987));
#52994=CARTESIAN_POINT('Ctrl Pts',(21.9651263157194,19.7842915581291,36.7844969922669));
#52995=CARTESIAN_POINT('Ctrl Pts',(21.9188638645174,19.7885155519253,36.7201623608739));
#52996=CARTESIAN_POINT('Ctrl Pts',(21.8726162114092,19.7927381945814,36.655848308371));
#52997=CARTESIAN_POINT('Ctrl Pts',(21.8231152388519,19.7969608372374,36.5938390970891));
#52998=CARTESIAN_POINT('Ctrl Pts',(21.7706261064023,19.8011834798935,36.5344733690459));
#52999=CARTESIAN_POINT('Ctrl Pts',(21.7181374212705,19.8054060865637,36.4751081469234));
#53000=CARTESIAN_POINT('Ctrl Pts',(21.662660938458,19.809628693234,36.4183867134876));
#53001=CARTESIAN_POINT('Ctrl Pts',(21.604500801512,19.8138512999042,36.3646131212761));
#53002=CARTESIAN_POINT('Ctrl Pts',(21.5462828319092,19.8180781054051,36.3107860582532));
#53003=CARTESIAN_POINT('Ctrl Pts',(21.4853762227442,19.8223049109059,36.2599130106039));
#53004=CARTESIAN_POINT('Ctrl Pts',(21.4221201011581,19.8265317164068,36.2122593242762));
#53005=CARTESIAN_POINT('Ctrl Pts',(21.3588333268225,19.8307605701396,36.1645825458514));
#53006=CARTESIAN_POINT('Ctrl Pts',(21.2931951606116,19.8349894238724,36.1201284997407));
#53007=CARTESIAN_POINT('Ctrl Pts',(21.225573653567,19.8392182776052,36.0791190879761));
#53008=CARTESIAN_POINT('Ctrl Pts',(21.1578306161347,19.8434547314975,36.0380359734811));
#53009=CARTESIAN_POINT('Ctrl Pts',(21.0880975292011,19.8476911853897,36.0004100861761));
#53010=CARTESIAN_POINT('Ctrl Pts',(21.0167667614865,19.8519276392819,35.9664171462921));
#53011=CARTESIAN_POINT('Ctrl Pts',(20.9519363359535,19.8557780269531,35.935521968399));
#53012=CARTESIAN_POINT('Ctrl Pts',(20.8857866695396,19.8596284146243,35.9076272632682));
#53013=CARTESIAN_POINT('Ctrl Pts',(20.8186237068181,19.8634788022955,35.8828293553415));
#53014=CARTESIAN_POINT('Ctrl Pts',(20.7447058271781,19.867716442818,35.8555373971078));
#53015=CARTESIAN_POINT('Ctrl Pts',(20.6692828805866,19.8719540833406,35.8318947553759));
#53016=CARTESIAN_POINT('Ctrl Pts',(20.5927493369304,19.8761917238632,35.8120667263951));
#53017=CARTESIAN_POINT('Ctrl Pts',(20.5163258515487,19.8804232704905,35.7922672109072));
#53018=CARTESIAN_POINT('Ctrl Pts',(20.438795390803,19.8846548171177,35.7762715309429));
#53019=CARTESIAN_POINT('Ctrl Pts',(20.3605704686141,19.888886363745,35.7641962030035));
#53020=CARTESIAN_POINT('Ctrl Pts',(20.2824358982314,19.8931130228266,35.7521348223798));
#53021=CARTESIAN_POINT('Ctrl Pts',(20.2036089213631,19.8973396819081,35.7439848664458));
#53022=CARTESIAN_POINT('Ctrl Pts',(20.1245137269355,19.9015663409897,35.7398121319046));
#53023=CARTESIAN_POINT('Ctrl Pts',(20.0454684597556,19.9057903320779,35.735642031318));
#53024=CARTESIAN_POINT('Ctrl Pts',(19.9661557779702,19.9100143231661,35.7354441936097));
#53025=CARTESIAN_POINT('Ctrl Pts',(19.8870052893639,19.9142383142543,35.739232617078));
#53026=CARTESIAN_POINT('Ctrl Pts',(19.8078801186683,19.9184609542121,35.7430198287413));
#53027=CARTESIAN_POINT('Ctrl Pts',(19.7289175060268,19.92268359417,35.7507907471139));
#53028=CARTESIAN_POINT('Ctrl Pts',(19.6505458625885,19.9269062341278,35.7625072734347));
#53029=CARTESIAN_POINT('Ctrl Pts',(19.5721748867913,19.9311288381133,35.7742236999433));
#53030=CARTESIAN_POINT('Ctrl Pts',(19.4943953335967,19.9353514420988,35.7898855968436));
#53031=CARTESIAN_POINT('Ctrl Pts',(19.4176278185341,19.9395740460843,35.8094033346845));
#53032=CARTESIAN_POINT('Ctrl Pts',(19.3407839674375,19.9438008489402,35.8289404805614));
#53033=CARTESIAN_POINT('Ctrl Pts',(19.2649546200374,19.9480276517961,35.852341010371));
#53034=CARTESIAN_POINT('Ctrl Pts',(19.1905469649741,19.9522544546519,35.8794648786864));
#53035=CARTESIAN_POINT('Ctrl Pts',(19.1161032530027,19.9564833057573,35.9066018908486));
#53036=CARTESIAN_POINT('Ctrl Pts',(19.0430830381416,19.9607121568626,35.9374656531096));
#53037=CARTESIAN_POINT('Ctrl Pts',(18.9718728096299,19.964941007968,35.9718682086577));
#53038=CARTESIAN_POINT('Ctrl Pts',(18.9005345999336,19.9691774592929,36.0063325935231));
#53039=CARTESIAN_POINT('Ctrl Pts',(18.831013288595,19.9734139106179,36.0443482541861));
#53040=CARTESIAN_POINT('Ctrl Pts',(18.763669861402,19.9776503619428,36.0856816961329));
#53041=CARTESIAN_POINT('Ctrl Pts',(18.702462991796,19.9815007737,36.1232486970571));
#53042=CARTESIAN_POINT('Ctrl Pts',(18.6430550338593,19.9853511854573,36.1635556649019));
#53043=CARTESIAN_POINT('Ctrl Pts',(18.5856933321888,19.9892015972146,36.2063983813155));
#53044=CARTESIAN_POINT('Ctrl Pts',(18.5231591640587,19.9933992114621,36.2531043463293));
#53045=CARTESIAN_POINT('Ctrl Pts',(18.4628128069114,19.9975968257097,36.303007336959));
#53046=CARTESIAN_POINT('Ctrl Pts',(18.4050040176627,20.0017944399573,36.3558732106788));
#53047=CARTESIAN_POINT('Ctrl Pts',(18.344864939825,20.0061612612184,36.4108701226693));
#53048=CARTESIAN_POINT('Ctrl Pts',(18.287472821428,20.0105280824795,36.4690736301524));
#53049=CARTESIAN_POINT('Ctrl Pts',(18.2331876128407,20.0148949037405,36.5301705731258));
#53050=CARTESIAN_POINT('Ctrl Pts',(18.1811422599262,20.0190815460978,36.5887466022467));
#53051=CARTESIAN_POINT('Ctrl Pts',(18.1319528489829,20.0232681884551,36.649981609482));
#53052=CARTESIAN_POINT('Ctrl Pts',(18.0859008250745,20.0274548308124,36.7135603909836));
#53053=CARTESIAN_POINT('Ctrl Pts',(18.0398760992656,20.0316389914682,36.77710148511));
#53054=CARTESIAN_POINT('Ctrl Pts',(17.9969853508088,20.0358231521239,36.8429832103659));
#53055=CARTESIAN_POINT('Ctrl Pts',(17.9574694509647,20.0400073127797,36.9108577052523));
#53056=CARTESIAN_POINT('Ctrl Pts',(17.9179640881504,20.0441903577168,36.9787141012071));
#53057=CARTESIAN_POINT('Ctrl Pts',(17.881832027718,20.0483734026539,37.0485617982512));
#53058=CARTESIAN_POINT('Ctrl Pts',(17.8492696610642,20.0525564475911,37.1200257911143));
#53059=CARTESIAN_POINT('Ctrl Pts',(17.8167053584166,20.0567397412309,37.1914940328654));
#53060=CARTESIAN_POINT('Ctrl Pts',(17.787711366745,20.0609230348707,37.2645783245426));
#53061=CARTESIAN_POINT('Ctrl Pts',(17.7624364599671,20.0651063285106,37.338882502359));
#53062=CARTESIAN_POINT('Ctrl Pts',(17.7371370902075,20.069293671061,37.4132585974235));
#53063=CARTESIAN_POINT('Ctrl Pts',(17.7155641412164,20.0734810136113,37.4888564804706));
#53064=CARTESIAN_POINT('Ctrl Pts',(17.6978166147843,20.0776683561617,37.5652644562621));
#53065=CARTESIAN_POINT('Ctrl Pts',(17.6800588871303,20.0818581055832,37.6417163511154));
#53066=CARTESIAN_POINT('Ctrl Pts',(17.6661310406482,20.0860478550048,37.7189787943313));
#53067=CARTESIAN_POINT('Ctrl Pts',(17.656080564927,20.0902376044263,37.7966320340127));
#53068=CARTESIAN_POINT('Ctrl Pts',(17.6460147322593,20.0944337557099,37.8744039264516));
#53069=CARTESIAN_POINT('Ctrl Pts',(17.639838124863,20.0986299069934,37.9525673304946));
#53070=CARTESIAN_POINT('Ctrl Pts',(17.6375461898729,20.1028260582769,38.0307003902189));
#53071=CARTESIAN_POINT('Ctrl Pts',(17.6368594185172,20.104083422259,38.0541127241566));
#53072=CARTESIAN_POINT('Ctrl Pts',(17.6365210907241,20.105340786241,38.0775223592207));
#53073=CARTESIAN_POINT('Ctrl Pts',(17.6365301782972,20.106598150223,38.1009180413976));
#53074=CARTESIAN_POINT('',(17.6365309629368,20.9003481398077,38.0978665184563));
#53075=CARTESIAN_POINT('Ctrl Pts',(17.6365301782975,20.1065981502717,38.1009180423036));
#53076=CARTESIAN_POINT('Ctrl Pts',(17.6365502375663,20.1093735642257,38.152559972328));
#53077=CARTESIAN_POINT('Ctrl Pts',(17.6382627322631,20.1121489781797,38.2041669172878));
#53078=CARTESIAN_POINT('Ctrl Pts',(17.6416616041977,20.1149243921337,38.2556613368326));
#53079=CARTESIAN_POINT('Ctrl Pts',(17.6468511805558,20.1191620400701,38.3342857238022));
#53080=CARTESIAN_POINT('Ctrl Pts',(17.6559866728642,20.1233996880065,38.4127978873952));
#53081=CARTESIAN_POINT('Ctrl Pts',(17.6690583310005,20.1276373359429,38.4907702350764));
#53082=CARTESIAN_POINT('Ctrl Pts',(17.6821111916988,20.131868890014,38.5686304561741));
#53083=CARTESIAN_POINT('Ctrl Pts',(17.6990889004778,20.136100444085,38.6459519444627));
#53084=CARTESIAN_POINT('Ctrl Pts',(17.7199298079772,20.1403319981561,38.7223105015577));
#53085=CARTESIAN_POINT('Ctrl Pts',(17.7407466437816,20.1445586646915,38.7985808628823));
#53086=CARTESIAN_POINT('Ctrl Pts',(17.7654176882308,20.1487853312269,38.8738900533054));
#53087=CARTESIAN_POINT('Ctrl Pts',(17.793830215714,20.1530119977623,38.9478238754621));
#53088=CARTESIAN_POINT('Ctrl Pts',(17.8222248084113,20.157235996307,39.0217110285122));
#53089=CARTESIAN_POINT('Ctrl Pts',(17.8543560286524,20.1614599948517,39.0942241000917));
#53090=CARTESIAN_POINT('Ctrl Pts',(17.8900616382825,20.1656839933964,39.1649650466813));
#53091=CARTESIAN_POINT('Ctrl Pts',(17.925755826695,20.169906640803,39.2356833652371));
#53092=CARTESIAN_POINT('Ctrl Pts',(17.9650219229629,20.1741292882097,39.3046302662762));
#53093=CARTESIAN_POINT('Ctrl Pts',(18.0076505987758,20.1783519356164,39.3714300233758));
#53094=CARTESIAN_POINT('Ctrl Pts',(18.050278911258,20.1825745470328,39.4382292111312));
#53095=CARTESIAN_POINT('Ctrl Pts',(18.0962694929201,20.1867971584492,39.5028808969397));
#53096=CARTESIAN_POINT('Ctrl Pts',(18.1453691309369,20.1910197698656,39.5650374672404));
#53097=CARTESIAN_POINT('Ctrl Pts',(18.1945175916058,20.1952465800724,39.6272558434675));
#53098=CARTESIAN_POINT('Ctrl Pts',(18.2467809926973,20.1994733902792,39.6869737795948));
#53099=CARTESIAN_POINT('Ctrl Pts',(18.3018655490479,20.203700200486,39.7438764635427));
#53100=CARTESIAN_POINT('Ctrl Pts',(18.3569767981394,20.2079290589103,39.8008067212554));
#53101=CARTESIAN_POINT('Ctrl Pts',(18.414911582831,20.2121579173346,39.8549186887404));
#53102=CARTESIAN_POINT('Ctrl Pts',(18.475340795717,20.2163867757588,39.9059359766324));
#53103=CARTESIAN_POINT('Ctrl Pts',(18.5358786116362,20.2206232342631,39.9570449525001));
#53104=CARTESIAN_POINT('Ctrl Pts',(18.5989194393215,20.2248596927673,40.0050478512135));
#53105=CARTESIAN_POINT('Ctrl Pts',(18.6641029740525,20.2290961512716,40.0497101263943));
#53106=CARTESIAN_POINT('Ctrl Pts',(18.7233456442571,20.2329464965319,40.0903018563465));
#53107=CARTESIAN_POINT('Ctrl Pts',(18.7843576564607,20.2367968417922,40.1281345668769));
#53108=CARTESIAN_POINT('Ctrl Pts',(18.8468517562158,20.2406471870526,40.1630655754865));
#53109=CARTESIAN_POINT('Ctrl Pts',(18.915631758473,20.2448848151924,40.2015100824148));
#53110=CARTESIAN_POINT('Ctrl Pts',(18.9864655113814,20.2491224433323,40.2365834365342));
#53111=CARTESIAN_POINT('Ctrl Pts',(19.0589890180882,20.2533600714721,40.2680610629826));
#53112=CARTESIAN_POINT('Ctrl Pts',(19.1314082327038,20.2575916057106,40.2994934231769));
#53113=CARTESIAN_POINT('Ctrl Pts',(19.205511949012,20.261823139949,40.3273401393661));
#53114=CARTESIAN_POINT('Ctrl Pts',(19.2809107665492,20.2660546741875,40.3514220206872));
#53115=CARTESIAN_POINT('Ctrl Pts',(19.3562224971132,20.2702813209287,40.3754760870077));
#53116=CARTESIAN_POINT('Ctrl Pts',(19.4328259119544,20.27450796767,40.3957738180204));
#53117=CARTESIAN_POINT('Ctrl Pts',(19.5103121972968,20.2787346144113,40.412184312892));
#53118=CARTESIAN_POINT('Ctrl Pts',(19.5877495714838,20.2829585931943,40.4285844490755));
#53119=CARTESIAN_POINT('Ctrl Pts',(19.6660682526112,20.2871825719772,40.4411021225969));
#53120=CARTESIAN_POINT('Ctrl Pts',(19.7448460262413,20.2914065507602,40.449656760162));
#53121=CARTESIAN_POINT('Ctrl Pts',(19.823598602073,20.2956291784646,40.4582086614473));
#53122=CARTESIAN_POINT('Ctrl Pts',(19.9028095131013,20.299851806169,40.4627999934345));
#53123=CARTESIAN_POINT('Ctrl Pts',(19.9820496330305,20.3040744338734,40.4634018332111));
#53124=CARTESIAN_POINT('Ctrl Pts',(20.0612890792022,20.3082970256739,40.4640036678705));
#53125=CARTESIAN_POINT('Ctrl Pts',(20.1405572650074,20.3125196174744,40.460616075635));
#53126=CARTESIAN_POINT('Ctrl Pts',(20.2194247591814,20.3167422092749,40.4532622497202));
#53127=CARTESIAN_POINT('Ctrl Pts',(20.2983706813693,20.3209690001372,40.4459011109578));
#53128=CARTESIAN_POINT('Ctrl Pts',(20.3769146481654,20.3251957909996,40.4345659037171));
#53129=CARTESIAN_POINT('Ctrl Pts',(20.4546326594229,20.329422581862,40.4193317110509));
#53130=CARTESIAN_POINT('Ctrl Pts',(20.5323883334244,20.3336514210596,40.4040901357781));
#53131=CARTESIAN_POINT('Ctrl Pts',(20.6093167990298,20.3378802602573,40.3849459243705));
#53132=CARTESIAN_POINT('Ctrl Pts',(20.6850070606099,20.3421090994549,40.3620247053944));
#53133=CARTESIAN_POINT('Ctrl Pts',(20.7608333604773,20.3463455391553,40.3390622900568));
#53134=CARTESIAN_POINT('Ctrl Pts',(20.8354165674048,20.3505819788557,40.3123094618713));
#53135=CARTESIAN_POINT('Ctrl Pts',(20.9083638047661,20.354818418556,40.281940796422));
#53136=CARTESIAN_POINT('Ctrl Pts',(20.9746659120371,20.3586689396946,40.2543385651775));
#53137=CARTESIAN_POINT('Ctrl Pts',(21.0396165636773,20.3625194608332,40.2237499834598));
#53138=CARTESIAN_POINT('Ctrl Pts',(21.1029396668827,20.3663699819718,40.1903383774204));
#53139=CARTESIAN_POINT('Ctrl Pts',(21.1726292584982,20.3706076335093,40.1535675771558));
#53140=CARTESIAN_POINT('Ctrl Pts',(21.2406088047282,20.3748452850467,40.1132388818508));
#53141=CARTESIAN_POINT('Ctrl Pts',(21.3064917779805,20.3790829365842,40.0695353957138));
#53142=CARTESIAN_POINT('Ctrl Pts',(21.3722800075188,20.3833144941215,40.0258947578422));
#53143=CARTESIAN_POINT('Ctrl Pts',(21.4359772641782,20.3875460516589,39.978889224043));
#53144=CARTESIAN_POINT('Ctrl Pts',(21.4972212636356,20.3917776091963,39.9287479128129));
#53145=CARTESIAN_POINT('Ctrl Pts',(21.5583945218872,20.3960042789816,39.8786645183885));
#53146=CARTESIAN_POINT('Ctrl Pts',(21.6171197933096,20.4002309487669,39.8254528399105));
#53147=CARTESIAN_POINT('Ctrl Pts',(21.6730647353122,20.4044576185522,39.7693845669452));
#53148=CARTESIAN_POINT('Ctrl Pts',(21.7289743615636,20.408681620214,39.7133516875848));
#53149=CARTESIAN_POINT('Ctrl Pts',(21.7821068118514,20.4129056218758,39.65446612396));
#53150=CARTESIAN_POINT('Ctrl Pts',(21.8321646673188,20.4171296235375,39.5930382020326));
#53151=CARTESIAN_POINT('Ctrl Pts',(21.8822065090906,20.4213522739253,39.5316299311276));
#53152=CARTESIAN_POINT('Ctrl Pts',(21.9291754133107,20.4255749243131,39.467681280123));
#53153=CARTESIAN_POINT('Ctrl Pts',(21.9728135265791,20.4297975747009,39.4015364882502));
#53154=CARTESIAN_POINT('Ctrl Pts',(22.0164512664753,20.4340201889593,39.335392262319));
#53155=CARTESIAN_POINT('Ctrl Pts',(22.0567580151298,20.4382428032177,39.2670523249554));
#53156=CARTESIAN_POINT('Ctrl Pts',(22.093519471624,20.4424654174761,39.1968895399407));
#53157=CARTESIAN_POINT('Ctrl Pts',(22.1303174801156,20.4466922302892,39.1266569919137));
#53158=CARTESIAN_POINT('Ctrl Pts',(22.163562936996,20.4509190431022,39.0545983920297));
#53159=CARTESIAN_POINT('Ctrl Pts',(22.1930880263597,20.4551458559153,38.9811102936283));
#53160=CARTESIAN_POINT('Ctrl Pts',(22.2226274220386,20.459374716821,38.9075865867352));
#53161=CARTESIAN_POINT('Ctrl Pts',(22.2484427061719,20.4636035777266,38.8326324452511));
#53162=CARTESIAN_POINT('Ctrl Pts',(22.2704155425845,20.4678324386323,38.7566610273883));
#53163=CARTESIAN_POINT('Ctrl Pts',(22.2924278671954,20.4720688993805,38.6805530784764));
#53164=CARTESIAN_POINT('Ctrl Pts',(22.3105838387478,20.4763053601287,38.6034246576765));
#53165=CARTESIAN_POINT('Ctrl Pts',(22.3248160438984,20.4805418208769,38.5257003675506));
#53166=CARTESIAN_POINT('Ctrl Pts',(22.3377510215795,20.4843921395483,38.4550604387819));
#53167=CARTESIAN_POINT('Ctrl Pts',(22.3474455405035,20.4882424582196,38.3839286802298));
#53168=CARTESIAN_POINT('Ctrl Pts',(22.3538863219802,20.4920927768909,38.3126255490165));
#53169=CARTESIAN_POINT('Ctrl Pts',(22.3609750725108,20.4963304534248,38.2341490301268));
#53170=CARTESIAN_POINT('Ctrl Pts',(22.3641483276393,20.5005681299588,38.1551703345829));
#53171=CARTESIAN_POINT('Ctrl Pts',(22.3633492908255,20.5048058064928,38.0761133833532));
#53172=CARTESIAN_POINT('Ctrl Pts',(22.3625514030035,20.5090373893705,37.9971701137321));
#53173=CARTESIAN_POINT('Ctrl Pts',(22.3577925715276,20.5132689722482,37.9181492767671));
#53174=CARTESIAN_POINT('Ctrl Pts',(22.3490677962963,20.5175005551259,37.839479503103));
#53175=CARTESIAN_POINT('Ctrl Pts',(22.3403530979342,20.5217272506448,37.7609005908076));
#53176=CARTESIAN_POINT('Ctrl Pts',(22.3276816099419,20.5259539461637,37.6826723995959));
#53177=CARTESIAN_POINT('Ctrl Pts',(22.3111003420476,20.5301806416826,37.6052216153798));
#53178=CARTESIAN_POINT('Ctrl Pts',(22.2945295402749,20.5344046693049,37.5278197182165));
#53179=CARTESIAN_POINT('Ctrl Pts',(22.2740539549072,20.5386286969271,37.4511947112408));
#53180=CARTESIAN_POINT('Ctrl Pts',(22.2497720166536,20.5428527245494,37.3757650146655));
#53181=CARTESIAN_POINT('Ctrl Pts',(22.2254978451484,20.5470754010867,37.300359444808));
#53182=CARTESIAN_POINT('Ctrl Pts',(22.1974198819901,20.5512980776241,37.2261488720142));
#53183=CARTESIAN_POINT('Ctrl Pts',(22.1656865434081,20.5555207541615,37.153536986142));
#53184=CARTESIAN_POINT('Ctrl Pts',(22.1339534752,20.5597433947209,37.0809257189366));
#53185=CARTESIAN_POINT('Ctrl Pts',(22.0985652825216,20.5639660352802,37.0099135405335));
#53186=CARTESIAN_POINT('Ctrl Pts',(22.059718100853,20.5681886758396,36.9408831871126));
#53187=CARTESIAN_POINT('Ctrl Pts',(22.0208322931237,20.572415515004,36.8717841962637));
#53188=CARTESIAN_POINT('Ctrl Pts',(21.9784808568169,20.5766423541684,36.8046713760373));
#53189=CARTESIAN_POINT('Ctrl Pts',(21.9329051031451,20.5808691933328,36.7399013627182));
#53190=CARTESIAN_POINT('Ctrl Pts',(21.8873072652332,20.5850980806592,36.6750999643664));
#53191=CARTESIAN_POINT('Ctrl Pts',(21.8384822865885,20.5893269679857,36.6126440042219));
#53192=CARTESIAN_POINT('Ctrl Pts',(21.7867123412089,20.5935558553122,36.552857650159));
#53193=CARTESIAN_POINT('Ctrl Pts',(21.7348493611133,20.597792342286,36.4929638552549));
#53194=CARTESIAN_POINT('Ctrl Pts',(21.6800311647458,20.6020288292599,36.4357495915753));
#53195=CARTESIAN_POINT('Ctrl Pts',(21.6225772454314,20.6062653162338,36.381502538987));
#53196=CARTESIAN_POINT('Ctrl Pts',(21.5703635869588,20.6101154014259,36.3322032551298));
#53197=CARTESIAN_POINT('Ctrl Pts',(21.5159737244961,20.6139654866179,36.2853542747074));
#53198=CARTESIAN_POINT('Ctrl Pts',(21.45966920065,20.61781557181,36.2411411388775));
#53199=CARTESIAN_POINT('Ctrl Pts',(21.3976985092085,20.6220531077158,36.19247864409));
#53200=CARTESIAN_POINT('Ctrl Pts',(21.3331753313424,20.6262906436217,36.1468271399636));
#53201=CARTESIAN_POINT('Ctrl Pts',(21.2664243354685,20.6305281795275,36.1044650232499));
#53202=CARTESIAN_POINT('Ctrl Pts',(21.1997693343686,20.6347596214224,36.0621638276021));
#53203=CARTESIAN_POINT('Ctrl Pts',(21.1308932703097,20.6389910633172,36.0231428742147));
#53204=CARTESIAN_POINT('Ctrl Pts',(21.0601529588401,20.6432225052121,35.9876396744962));
#53205=CARTESIAN_POINT('Ctrl Pts',(20.9894943510225,20.6474490598758,35.9521774802668));
#53206=CARTESIAN_POINT('Ctrl Pts',(20.9169761915445,20.6516756145395,35.9202251748641));
#53207=CARTESIAN_POINT('Ctrl Pts',(20.8429819769238,20.6559021692032,35.89197558268));
#53208=CARTESIAN_POINT('Ctrl Pts',(20.7690344666336,20.6601260561123,35.8637438213262));
#53209=CARTESIAN_POINT('Ctrl Pts',(20.6936131872793,20.6643499430214,35.8392103010606));
#53210=CARTESIAN_POINT('Ctrl Pts',(20.6171226929917,20.6685738299305,35.8185202120784));
#53211=CARTESIAN_POINT('Ctrl Pts',(20.5406566594799,20.6727963660894,35.7978367395476));
#53212=CARTESIAN_POINT('Ctrl Pts',(20.4631225422344,20.6770189022483,35.7809943799041));
#53213=CARTESIAN_POINT('Ctrl Pts',(20.384939748247,20.6812414384072,35.768088374076));
#53214=CARTESIAN_POINT('Ctrl Pts',(20.306757610646,20.6854639391157,35.7551824766007));
#53215=CARTESIAN_POINT('Ctrl Pts',(20.2279272699033,20.6896864398241,35.7462129421741));
#53216=CARTESIAN_POINT('Ctrl Pts',(20.1488765312761,20.6939089405326,35.7412235758056));
#53217=CARTESIAN_POINT('Ctrl Pts',(20.0697471555963,20.6981356416447,35.736229246181));
#53218=CARTESIAN_POINT('Ctrl Pts',(19.9903974130468,20.7023623427568,35.7352230230069));
#53219=CARTESIAN_POINT('Ctrl Pts',(19.9112578054728,20.7065890438688,35.7381966077147));
#53220=CARTESIAN_POINT('Ctrl Pts',(19.8320798343499,20.7108177939076,35.7411716338911));
#53221=CARTESIAN_POINT('Ctrl Pts',(19.7531126687147,20.7150465439464,35.7481302700112));
#53222=CARTESIAN_POINT('Ctrl Pts',(19.6747818161435,20.7192752939852,35.7590122653484));
#53223=CARTESIAN_POINT('Ctrl Pts',(19.5963101386655,20.7235116465626,35.7699138245731));
#53224=CARTESIAN_POINT('Ctrl Pts',(19.518477521625,20.72774799914,35.7847527485802));
#53225=CARTESIAN_POINT('Ctrl Pts',(19.4416991776763,20.7319843517174,35.8034176190059));
#53226=CARTESIAN_POINT('Ctrl Pts',(19.3718987127443,20.7358356900546,35.820386162043));
#53227=CARTESIAN_POINT('Ctrl Pts',(19.302969678025,20.7396870283918,35.8405161048758));
#53228=CARTESIAN_POINT('Ctrl Pts',(19.2352103821458,20.743538366729,35.8636889122212));
#53229=CARTESIAN_POINT('Ctrl Pts',(19.1606528728991,20.7477761054771,35.8891866210671));
#53230=CARTESIAN_POINT('Ctrl Pts',(19.0872319476852,20.7520138442252,35.9184648282699));
#53231=CARTESIAN_POINT('Ctrl Pts',(19.0153578995573,20.7562515829733,35.9514026959582));
#53232=CARTESIAN_POINT('Ctrl Pts',(18.9435872179411,20.7604832271673,35.9842931936628));
#53233=CARTESIAN_POINT('Ctrl Pts',(18.8733594180529,20.7647148713613,36.0208327059724));
#53234=CARTESIAN_POINT('Ctrl Pts',(18.8050679923315,20.7689465155553,36.0608511731732));
#53235=CARTESIAN_POINT('Ctrl Pts',(18.7368554662643,20.7731732707715,36.1008234055327));
#53236=CARTESIAN_POINT('Ctrl Pts',(18.6705752709255,20.7774000259878,36.1442663694814));
#53237=CARTESIAN_POINT('Ctrl Pts',(18.6065979340457,20.781626781204,36.1909632995947));
#53238=CARTESIAN_POINT('Ctrl Pts',(18.5426609944809,20.7858508675132,36.2376307437887));
#53239=CARTESIAN_POINT('Ctrl Pts',(18.4810244047791,20.7900749538225,36.2875478002407));
#53240=CARTESIAN_POINT('Ctrl Pts',(18.4220301955602,20.7942990401317,36.3404541105228));
#53241=CARTESIAN_POINT('Ctrl Pts',(18.3630548709045,20.7985217742739,36.3933434850314));
#53242=CARTESIAN_POINT('Ctrl Pts',(18.306720595762,20.8027445084161,36.4492199004445));
#53243=CARTESIAN_POINT('Ctrl Pts',(18.2533355846976,20.8069672425583,36.5077833497868));
#53244=CARTESIAN_POINT('Ctrl Pts',(18.1999510430786,20.8111899395675,36.5663462841466));
#53245=CARTESIAN_POINT('Ctrl Pts',(18.1495160287036,20.8154126365768,36.6275958580747));
#53246=CARTESIAN_POINT('Ctrl Pts',(18.1023001799655,20.819635333586,36.6911970208929));
#53247=CARTESIAN_POINT('Ctrl Pts',(18.0550374092106,20.8238622270137,36.7548613890736));
#53248=CARTESIAN_POINT('Ctrl Pts',(18.0110004744393,20.8280891204415,36.8208816369771));
#53249=CARTESIAN_POINT('Ctrl Pts',(17.9704167741943,20.8323160138692,36.8888920896847));
#53250=CARTESIAN_POINT('Ctrl Pts',(17.9298134195799,20.8365449543485,36.9569354793241));
#53251=CARTESIAN_POINT('Ctrl Pts',(17.8926668509941,20.8407738948277,37.0269705792204));
#53252=CARTESIAN_POINT('Ctrl Pts',(17.8591581683313,20.845002835307,37.0986076230182));
#53253=CARTESIAN_POINT('Ctrl Pts',(17.8255892882827,20.8492393729563,37.1703733607072));
#53254=CARTESIAN_POINT('Ctrl Pts',(17.795671529851,20.8534759106056,37.2437463574324));
#53255=CARTESIAN_POINT('Ctrl Pts',(17.7695374667954,20.857712448255,37.3183176291674));
#53256=CARTESIAN_POINT('Ctrl Pts',(17.7457904962732,20.861562019386,37.3860775403581));
#53257=CARTESIAN_POINT('Ctrl Pts',(17.7251670205788,20.865411590517,37.4548263636818));
#53258=CARTESIAN_POINT('Ctrl Pts',(17.7077299169298,20.8692611616481,37.5242497875283));
#53259=CARTESIAN_POINT('Ctrl Pts',(17.6828131325473,20.8747620140699,37.6234525288718));
#53260=CARTESIAN_POINT('Ctrl Pts',(17.6643259671831,20.8802628664916,37.7243300595161));
#53261=CARTESIAN_POINT('Ctrl Pts',(17.6524475134137,20.8857637189134,37.8261610626257));
#53262=CARTESIAN_POINT('Ctrl Pts',(17.6419497240976,20.8906251925449,37.9161559758721));
#53263=CARTESIAN_POINT('Ctrl Pts',(17.6366130815916,20.8954866661763,38.0068955425699));
#53264=CARTESIAN_POINT('Ctrl Pts',(17.6365309629368,20.9003481398077,38.0978665184563));
#53265=CARTESIAN_POINT('',(17.6389973268257,21.6940981586901,38.1008155980709));
#53266=CARTESIAN_POINT('Ctrl Pts',(17.6368549259571,20.9003481502717,38.0978670066765));
#53267=CARTESIAN_POINT('Ctrl Pts',(17.6421592816668,20.9318934190369,38.6880864281803));
#53268=CARTESIAN_POINT('Ctrl Pts',(18.164146447441,21.0053462861083,40.0707873438575));
#53269=CARTESIAN_POINT('Ctrl Pts',(20.4819917868442,21.1207067514864,40.8493537277608));
#53270=CARTESIAN_POINT('Ctrl Pts',(22.5685527330183,21.2464295464053,39.1923202798239));
#53271=CARTESIAN_POINT('Ctrl Pts',(22.3147694606222,21.3721523413244,36.539764552403));
#53272=CARTESIAN_POINT('Ctrl Pts',(19.950593046619,21.4978751362435,35.3092112299817));
#53273=CARTESIAN_POINT('Ctrl Pts',(17.972450588763,21.6051904058926,36.4295872739547));
#53274=CARTESIAN_POINT('Ctrl Pts',(17.6411648689987,21.6705980772353,37.6595592470186));
#53275=CARTESIAN_POINT('Ctrl Pts',(17.6396904081475,21.6940981502717,38.1008152004127));
#53276=CARTESIAN_POINT('',(17.8640015678817,21.7500582353796,39.1118986969983));
#53277=CARTESIAN_POINT('Ctrl Pts',(17.6365301412143,21.6940981886575,38.1008170136285));
#53278=CARTESIAN_POINT('Ctrl Pts',(17.6365600512031,21.6987000667762,38.1873410991501));
#53279=CARTESIAN_POINT('Ctrl Pts',(17.6413455319869,21.7033019448949,38.2737209365862));
#53280=CARTESIAN_POINT('Ctrl Pts',(17.6508139214875,21.7079038230136,38.3594517477744));
#53281=CARTESIAN_POINT('Ctrl Pts',(17.6602963768197,21.7125125374841,38.4453099169623));
#53282=CARTESIAN_POINT('Ctrl Pts',(17.6744755305038,21.7171212519547,38.5305168200371));
#53283=CARTESIAN_POINT('Ctrl Pts',(17.6932279303512,21.7217299664253,38.6145804694974));
#53284=CARTESIAN_POINT('Ctrl Pts',(17.712060860961,21.7263584726714,38.6990051239404));
#53285=CARTESIAN_POINT('Ctrl Pts',(17.7355062649425,21.7309869789176,38.7822763791188));
#53286=CARTESIAN_POINT('Ctrl Pts',(17.7633902310012,21.7356154851638,38.8639156904523));
#53287=CARTESIAN_POINT('Ctrl Pts',(17.7909121752497,21.7401838988031,38.9444950660788));
#53288=CARTESIAN_POINT('Ctrl Pts',(17.8227578968555,21.7447523124424,39.0234843889073));
#53289=CARTESIAN_POINT('Ctrl Pts',(17.8587159851212,21.7493207260817,39.1004465045792));
#53290=CARTESIAN_POINT('Ctrl Pts',(17.860498178638,21.7495471507211,39.1042609838856));
#53291=CARTESIAN_POINT('Ctrl Pts',(17.8622905760233,21.7497735753605,39.1080707250178));
#53292=CARTESIAN_POINT('Ctrl Pts',(17.8640931615355,21.75,39.111875693107));
#53293=CARTESIAN_POINT('',(17.63653,21.75,38.1));
#53294=CARTESIAN_POINT('Origin',(20.,21.75,38.1));
#53295=CARTESIAN_POINT('',(17.9450946017473,21.75,36.932372385933));
#53296=CARTESIAN_POINT('Origin',(20.,21.75,38.1));
#53297=CARTESIAN_POINT('',(17.6365309178096,21.0215268497626,38.0979171101847));
#53298=CARTESIAN_POINT('Ctrl Pts',(17.9450946017473,21.75,36.932372385933));
#53299=CARTESIAN_POINT('Ctrl Pts',(17.9851605709061,21.7456651391115,36.8618603705277));
#53300=CARTESIAN_POINT('Ctrl Pts',(18.028888487075,21.7413302782229,36.7933619642338));
#53301=CARTESIAN_POINT('Ctrl Pts',(18.0760493998635,21.7369954173344,36.7272638530531));
#53302=CARTESIAN_POINT('Ctrl Pts',(18.1231813997955,21.7326632140112,36.6612062645235));
#53303=CARTESIAN_POINT('Ctrl Pts',(18.1737419548967,21.7283310106881,36.5975463986434));
#53304=CARTESIAN_POINT('Ctrl Pts',(18.2274587566072,21.723998807365,36.5366420814888));
#53305=CARTESIAN_POINT('Ctrl Pts',(18.2811699013855,21.7196670602675,36.4757441781859));
#53306=CARTESIAN_POINT('Ctrl Pts',(18.3380363499296,21.71533531317,36.4176015811557));
#53307=CARTESIAN_POINT('Ctrl Pts',(18.3977459308174,21.7110035660725,36.3625385360568));
#53308=CARTESIAN_POINT('Ctrl Pts',(18.4574542812051,21.706671908244,36.3074766257017));
#53309=CARTESIAN_POINT('Ctrl Pts',(18.5200053258509,21.7023402504155,36.2554944382585));
#53310=CARTESIAN_POINT('Ctrl Pts',(18.5850514603843,21.698008592587,36.2068779566179));
#53311=CARTESIAN_POINT('Ctrl Pts',(18.6501122764574,21.6936759570615,36.1582505017685));
#53312=CARTESIAN_POINT('Ctrl Pts',(18.7176689517958,21.6893433215361,36.1129905258459));
#53313=CARTESIAN_POINT('Ctrl Pts',(18.7873432679355,21.6850106860106,36.0713418003324));
#53314=CARTESIAN_POINT('Ctrl Pts',(18.8570504778676,21.6806760050139,36.0296734121281));
#53315=CARTESIAN_POINT('Ctrl Pts',(18.9288769414282,21.6763413240172,35.9916198898748));
#53316=CARTESIAN_POINT('Ctrl Pts',(19.0024190898503,21.6720066430205,35.9573794622927));
#53317=CARTESIAN_POINT('Ctrl Pts',(19.0760706189195,21.6676655149696,35.9230881082663));
#53318=CARTESIAN_POINT('Ctrl Pts',(19.1514425308926,21.6633243869187,35.8926213592826));
#53319=CARTESIAN_POINT('Ctrl Pts',(19.2281105539884,21.6589832588679,35.8661295641788));
#53320=CARTESIAN_POINT('Ctrl Pts',(19.3048387862111,21.6546387216313,35.8396169644711));
#53321=CARTESIAN_POINT('Ctrl Pts',(19.3828647373174,21.6502941843947,35.8170856609605));
#53322=CARTESIAN_POINT('Ctrl Pts',(19.461750524746,21.6459496471581,35.7986356343923));
#53323=CARTESIAN_POINT('Ctrl Pts',(19.5407886017683,21.6415967227604,35.780149989912));
#53324=CARTESIAN_POINT('Ctrl Pts',(19.6206894004145,21.6372437983627,35.7657614431077));
#53325=CARTESIAN_POINT('Ctrl Pts',(19.7010063587428,21.6328908739649,35.7555185555463));
#53326=CARTESIAN_POINT('Ctrl Pts',(19.7539840523267,21.6300196510036,35.748762266838));
#53327=CARTESIAN_POINT('Ctrl Pts',(19.8071426961314,21.6271484280423,35.7438086087321));
#53328=CARTESIAN_POINT('Ctrl Pts',(19.860354082761,21.6242772050809,35.7406591050256));
#53329=CARTESIAN_POINT('Ctrl Pts',(19.9381292905192,21.6200805476269,35.7360557048773));
#53330=CARTESIAN_POINT('Ctrl Pts',(20.0163084813515,21.6158838901729,35.7352919334201));
#53331=CARTESIAN_POINT('Ctrl Pts',(20.0944748898714,21.6116872327189,35.7384189753295));
#53332=CARTESIAN_POINT('Ctrl Pts',(20.1725163937938,21.6074972812377,35.7415410204389));
#53333=CARTESIAN_POINT('Ctrl Pts',(20.250544682398,21.6033073297565,35.7485415218038));
#53334=CARTESIAN_POINT('Ctrl Pts',(20.3281387129406,21.5991173782753,35.7594198526926));
#53335=CARTESIAN_POINT('Ctrl Pts',(20.4057359322867,21.5949272546039,35.7702986306371));
#53336=CARTESIAN_POINT('Ctrl Pts',(20.4828983768163,21.5907371309325,35.7850555670828));
#53337=CARTESIAN_POINT('Ctrl Pts',(20.5592058395492,21.5865470072611,35.803637818219));
#53338=CARTESIAN_POINT('Ctrl Pts',(20.6353510052443,21.5823657954921,35.8221805470829));
#53339=CARTESIAN_POINT('Ctrl Pts',(20.7106443491242,21.5781845837231,35.8445322558333));
#53340=CARTESIAN_POINT('Ctrl Pts',(20.7846763779237,21.5740033719541,35.8705889964324));
#53341=CARTESIAN_POINT('Ctrl Pts',(20.8586776733355,21.5698238959582,35.8966349199307));
#53342=CARTESIAN_POINT('Ctrl Pts',(20.9314182411447,21.5656444199623,35.926382664346));
#53343=CARTESIAN_POINT('Ctrl Pts',(21.0025041375631,21.5614649439663,35.9596785533316));
#53344=CARTESIAN_POINT('Ctrl Pts',(21.0735837645821,21.557285836578,35.9929715057962));
#53345=CARTESIAN_POINT('Ctrl Pts',(21.1430085765028,21.5531067291897,36.0298117771111));
#53346=CARTESIAN_POINT('Ctrl Pts',(21.2104064971494,21.5489276218014,36.06999838607));
#53347=CARTESIAN_POINT('Ctrl Pts',(21.2781053581212,21.5447298541648,36.1103644333714));
#53348=CARTESIAN_POINT('Ctrl Pts',(21.3437587583622,21.5405320865282,36.1541065357132));
#53349=CARTESIAN_POINT('Ctrl Pts',(21.4070181129212,21.5363343188915,36.2009764427971));
#53350=CARTESIAN_POINT('Ctrl Pts',(21.4700838811366,21.5321493972679,36.2477029185418));
#53351=CARTESIAN_POINT('Ctrl Pts',(21.5307698904924,21.5279644756442,36.2975377427675));
#53352=CARTESIAN_POINT('Ctrl Pts',(21.5887647458843,21.5237795540205,36.3501951471278));
#53353=CARTESIAN_POINT('Ctrl Pts',(21.6470266323214,21.5195753633774,36.4030950068167));
#53354=CARTESIAN_POINT('Ctrl Pts',(21.7025721844741,21.5153711727343,36.4588431509752));
#53355=CARTESIAN_POINT('Ctrl Pts',(21.7551252698619,21.5111669820912,36.5171147457911));
#53356=CARTESIAN_POINT('Ctrl Pts',(21.8076783552497,21.5069627914481,36.575386340607));
#53357=CARTESIAN_POINT('Ctrl Pts',(21.8572387223883,21.5027586008049,36.6361809685824));
#53358=CARTESIAN_POINT('Ctrl Pts',(21.9035741464061,21.4985544101618,36.6991445791823));
#53359=CARTESIAN_POINT('Ctrl Pts',(21.9503378161638,21.4943113631411,36.7626901181573));
#53360=CARTESIAN_POINT('Ctrl Pts',(21.9940026520819,21.4900683161204,36.8286974682417));
#53361=CARTESIAN_POINT('Ctrl Pts',(22.0343003622833,21.4858252690997,36.8968323155462));
#53362=CARTESIAN_POINT('Ctrl Pts',(22.0745401666081,21.481588319134,36.9648692563433));
#53363=CARTESIAN_POINT('Ctrl Pts',(22.1114222185724,21.4773513691683,37.035027223734));
#53364=CARTESIAN_POINT('Ctrl Pts',(22.1447201399324,21.4731144192026,37.1069411083585));
#53365=CARTESIAN_POINT('Ctrl Pts',(22.1779793978106,21.4688823889205,37.1787714910387));
#53366=CARTESIAN_POINT('Ctrl Pts',(22.2076626007544,21.4646503586385,37.2523533168423));
#53367=CARTESIAN_POINT('Ctrl Pts',(22.2335888985862,21.4604183283564,37.3272962579277));
#53368=CARTESIAN_POINT('Ctrl Pts',(22.2594987142216,21.4561889885146,37.4021915553317));
#53369=CARTESIAN_POINT('Ctrl Pts',(22.281656213478,21.4519596486727,37.4784458097847));
#53370=CARTESIAN_POINT('Ctrl Pts',(22.2999288277623,21.4477303088309,37.5556491681572));
#53371=CARTESIAN_POINT('Ctrl Pts',(22.3181954730667,21.4435023505562,37.6328273070788));
#53372=CARTESIAN_POINT('Ctrl Pts',(22.3325796461432,21.4392743922816,37.7109534797209));
#53373=CARTESIAN_POINT('Ctrl Pts',(22.3429991708417,21.4350464340069,37.7896045645709));
#53374=CARTESIAN_POINT('Ctrl Pts',(22.353418512125,21.4308185501571,37.8682542649241));
#53375=CARTESIAN_POINT('Ctrl Pts',(22.3598732837732,21.4265906663073,37.9474283956148));
#53376=CARTESIAN_POINT('Ctrl Pts',(22.3623329819944,21.4223627824575,38.0266970458871));
#53377=CARTESIAN_POINT('Ctrl Pts',(22.3647950655226,21.4181307985919,38.1060425674101));
#53378=CARTESIAN_POINT('Ctrl Pts',(22.3632543219911,21.4138988147263,38.185482323399));
#53379=CARTESIAN_POINT('Ctrl Pts',(22.3577324085168,21.4096668308607,38.26458532963));
#53380=CARTESIAN_POINT('Ctrl Pts',(22.3522078826181,21.405432844838,38.3437257595965));
#53381=CARTESIAN_POINT('Ctrl Pts',(22.3426984899765,21.4011988588153,38.4225286577333));
#53382=CARTESIAN_POINT('Ctrl Pts',(22.3292776621049,21.3969648727926,38.5005696115769));
#53383=CARTESIAN_POINT('Ctrl Pts',(22.3158331840349,21.3927234256348,38.5787480892799));
#53384=CARTESIAN_POINT('Ctrl Pts',(22.2984636004284,21.388481978477,38.6561614826017));
#53385=CARTESIAN_POINT('Ctrl Pts',(22.2772931704297,21.3842405313192,38.7323972302391));
#53386=CARTESIAN_POINT('Ctrl Pts',(22.2583113111591,21.3804375592937,38.8007518282861));
#53387=CARTESIAN_POINT('Ctrl Pts',(22.2362746075327,21.3766345872682,38.8681596607891));
#53388=CARTESIAN_POINT('Ctrl Pts',(22.2113054209498,21.3728316152427,38.9343373275709));
#53389=CARTESIAN_POINT('Ctrl Pts',(22.1834357300525,21.3685868772538,39.0082024136995));
#53390=CARTESIAN_POINT('Ctrl Pts',(22.1518106828993,21.3643421392649,39.0808028936984));
#53391=CARTESIAN_POINT('Ctrl Pts',(22.1165658357701,21.3600974012759,39.1517316690823));
#53392=CARTESIAN_POINT('Ctrl Pts',(22.0813703688881,21.3558586104318,39.2225610687918));
#53393=CARTESIAN_POINT('Ctrl Pts',(22.0425653810947,21.3516198195878,39.2917230008846));
#53394=CARTESIAN_POINT('Ctrl Pts',(22.0003350258194,21.3473810287437,39.3588289102893));
#53395=CARTESIAN_POINT('Ctrl Pts',(21.9581515078158,21.3431469391008,39.4258603931899));
#53396=CARTESIAN_POINT('Ctrl Pts',(21.9125504199301,21.338912849458,39.4908399919148));
#53397=CARTESIAN_POINT('Ctrl Pts',(21.8637617976855,21.3346787598151,39.5534037300035));
#53398=CARTESIAN_POINT('Ctrl Pts',(21.8150026522956,21.3304472283024,39.6159296686601));
#53399=CARTESIAN_POINT('Ctrl Pts',(21.7630600820158,21.3262156967897,39.6760422768745));
#53400=CARTESIAN_POINT('Ctrl Pts',(21.7082067031625,21.3219841652769,39.733407573195));
#53401=CARTESIAN_POINT('Ctrl Pts',(21.6533695550489,21.3177538858455,39.7907558955165));
#53402=CARTESIAN_POINT('Ctrl Pts',(21.5956236314241,21.313523606414,39.845358183187));
#53403=CARTESIAN_POINT('Ctrl Pts',(21.5352800179998,21.3092933269825,39.8969156093792));
#53404=CARTESIAN_POINT('Ctrl Pts',(21.4749356576554,21.3050629951896,39.948473673738));
#53405=CARTESIAN_POINT('Ctrl Pts',(21.4119938996078,21.3008326633966,39.9969864995924));
#53406=CARTESIAN_POINT('Ctrl Pts',(21.3467995518017,21.2966023316037,40.0421949974621));
#53407=CARTESIAN_POINT('Ctrl Pts',(21.2815391889019,21.2923677162224,40.0874492729693));
#53408=CARTESIAN_POINT('Ctrl Pts',(21.2140220648128,21.2881331008411,40.1293922706003));
#53409=CARTESIAN_POINT('Ctrl Pts',(21.1446221918467,21.2838984854598,40.1678081339506));
#53410=CARTESIAN_POINT('Ctrl Pts',(21.075187789895,21.2796617632018,40.2062431106037));
#53411=CARTESIAN_POINT('Ctrl Pts',(21.0038691928153,21.2754250409438,40.2411472514391));
#53412=CARTESIAN_POINT('Ctrl Pts',(20.9310629697655,21.2711883186858,40.2723517641559));
#53413=CARTESIAN_POINT('Ctrl Pts',(20.8581260144692,21.2669439888883,40.3036123082927));
#53414=CARTESIAN_POINT('Ctrl Pts',(20.7836965347698,21.2626996590908,40.3311597882819));
#53415=CARTESIAN_POINT('Ctrl Pts',(20.7081887250828,21.2584553292933,40.3548745354378));
#53416=CARTESIAN_POINT('Ctrl Pts',(20.6409028730737,21.2546731596368,40.3760070113257));
#53417=CARTESIAN_POINT('Ctrl Pts',(20.5727611740573,21.2508909899802,40.3940966556243));
#53418=CARTESIAN_POINT('Ctrl Pts',(20.5040626209202,21.2471088203236,40.409093180253));
#53419=CARTESIAN_POINT('Ctrl Pts',(20.4271862073671,21.2428764220362,40.4258748878229));
#53420=CARTESIAN_POINT('Ctrl Pts',(20.3493230194014,21.2386440237488,40.4388454898891));
#53421=CARTESIAN_POINT('Ctrl Pts',(20.2708853972536,21.2344116254614,40.4478951302081));
#53422=CARTESIAN_POINT('Ctrl Pts',(20.1925620912636,21.2301853955342,40.4569315814466));
#53423=CARTESIAN_POINT('Ctrl Pts',(20.1136664765453,21.225959165607,40.462058364944));
#53424=CARTESIAN_POINT('Ctrl Pts',(20.0346221513252,21.2217329356798,40.4632163987959));
#53425=CARTESIAN_POINT('Ctrl Pts',(19.9556708721593,21.2175116806072,40.4643730694825));
#53426=CARTESIAN_POINT('Ctrl Pts',(19.8765716979425,21.2132904255345,40.4615702671053));
#53427=CARTESIAN_POINT('Ctrl Pts',(19.7977528874448,21.2090691704619,40.4548007445139));
#53428=CARTESIAN_POINT('Ctrl Pts',(19.7189848419724,21.2048506341834,40.4480355819856));
#53429=CARTESIAN_POINT('Ctrl Pts',(19.6404972689457,21.2006320979049,40.4373088100029));
#53430=CARTESIAN_POINT('Ctrl Pts',(19.5627167333875,21.1964135616264,40.4226652332269));
#53431=CARTESIAN_POINT('Ctrl Pts',(19.4849619080215,21.1921964197761,40.4080264968543));
#53432=CARTESIAN_POINT('Ctrl Pts',(19.4079141177169,21.1879792779259,40.3894736133584));
#53433=CARTESIAN_POINT('Ctrl Pts',(19.3319916212802,21.1837621360757,40.3671028311173));
#53434=CARTESIAN_POINT('Ctrl Pts',(19.2560704177342,21.1795450660396,40.3447324298302));
#53435=CARTESIAN_POINT('Ctrl Pts',(19.1812749205266,21.1753279960034,40.3185443932312));
#53436=CARTESIAN_POINT('Ctrl Pts',(19.1080086049598,21.1711109259673,40.2886849458235));
#53437=CARTESIAN_POINT('Ctrl Pts',(19.0346696529475,21.1668896751152,40.2587958956698));
#53438=CARTESIAN_POINT('Ctrl Pts',(18.9628633472858,21.1626684242631,40.2252283418271));
#53439=CARTESIAN_POINT('Ctrl Pts',(18.8929729394482,21.1584471734111,40.1881766036679));
#53440=CARTESIAN_POINT('Ctrl Pts',(18.8230489316763,21.1542238931854,40.1511070528216));
#53441=CARTESIAN_POINT('Ctrl Pts',(18.7550430607771,21.1500006129597,40.1105502221402));
#53442=CARTESIAN_POINT('Ctrl Pts',(18.6893114773836,21.145777332734,40.0667450362417));
#53443=CARTESIAN_POINT('Ctrl Pts',(18.6234610884587,21.1415464192059,40.0228606753392));
#53444=CARTESIAN_POINT('Ctrl Pts',(18.5598935789063,21.1373155056779,39.975716508835));
#53445=CARTESIAN_POINT('Ctrl Pts',(18.4989335617418,21.1330845921498,39.9255930512671));
#53446=CARTESIAN_POINT('Ctrl Pts',(18.4427483096401,21.1291850699014,39.8793955724827));
#53447=CARTESIAN_POINT('Ctrl Pts',(18.3887778975703,21.125285547653,39.8306678864608));
#53448=CARTESIAN_POINT('Ctrl Pts',(18.337247647282,21.1213860254047,39.7796562310279));
#53449=CARTESIAN_POINT('Ctrl Pts',(18.282035136839,21.117207850223,39.7249993733074));
#53450=CARTESIAN_POINT('Ctrl Pts',(18.2294031944704,21.1130296750413,39.6675008619878));
#53451=CARTESIAN_POINT('Ctrl Pts',(18.1796642322315,21.1088514998596,39.6074376051706));
#53452=CARTESIAN_POINT('Ctrl Pts',(18.1299893454759,21.1046787071503,39.5474517239568));
#53453=CARTESIAN_POINT('Ctrl Pts',(18.0832003544408,21.1005059144411,39.4849080160239));
#53454=CARTESIAN_POINT('Ctrl Pts',(18.0395737127453,21.0963331217318,39.420120908531));
#53455=CARTESIAN_POINT('Ctrl Pts',(17.9959887861599,21.0921643189815,39.3553957494537));
#53456=CARTESIAN_POINT('Ctrl Pts',(17.9555604796703,21.0879955162312,39.288431843644));
#53457=CARTESIAN_POINT('Ctrl Pts',(17.9185246427869,21.0838267134808,39.2195761600777));
#53458=CARTESIAN_POINT('Ctrl Pts',(17.8815119282262,21.0796605134097,39.1507634646947));
#53459=CARTESIAN_POINT('Ctrl Pts',(17.84788770825,21.0754943133386,39.080061759597));
#53460=CARTESIAN_POINT('Ctrl Pts',(17.8178432905259,21.0713281132674,39.0078449956887));
#53461=CARTESIAN_POINT('Ctrl Pts',(17.7877954584808,21.0671614397392,38.9356200248913));
#53462=CARTESIAN_POINT('Ctrl Pts',(17.7613284441657,21.0629947662109,38.8618800900702));
#53463=CARTESIAN_POINT('Ctrl Pts',(17.7385860222733,21.0588280926827,38.7870205690096));
#53464=CARTESIAN_POINT('Ctrl Pts',(17.71584385661,21.0546614660985,38.712161891359));
#53465=CARTESIAN_POINT('Ctrl Pts',(17.6968263319712,21.0504948395144,38.6361841176834));
#53466=CARTESIAN_POINT('Ctrl Pts',(17.6816271136747,21.0463282129303,38.5594971173486));
#53467=CARTESIAN_POINT('Ctrl Pts',(17.6664112266698,21.0421570168819,38.4827260157645));
#53468=CARTESIAN_POINT('Ctrl Pts',(17.655022096355,21.0379858208336,38.4052446104354));
#53469=CARTESIAN_POINT('Ctrl Pts',(17.6475019384674,21.0338146247853,38.3274715617071));
#53470=CARTESIAN_POINT('Ctrl Pts',(17.6401174850886,21.0297186997777,38.2511019613542));
#53471=CARTESIAN_POINT('Ctrl Pts',(17.6364634691103,21.0256227747701,38.1744516028563));
#53472=CARTESIAN_POINT('Ctrl Pts',(17.6365309178096,21.0215268497626,38.0979171101847));
#53473=CARTESIAN_POINT('',(17.6365304175565,20.2277768497005,38.1014049071763));
#53474=CARTESIAN_POINT('Ctrl Pts',(17.6365309178101,21.0215268497283,38.0979171095448));
#53475=CARTESIAN_POINT('Ctrl Pts',(17.6366289743903,21.0155722163544,37.9866516826965));
#53476=CARTESIAN_POINT('Ctrl Pts',(17.6445876386274,21.0096175829806,37.8757208437721));
#53477=CARTESIAN_POINT('Ctrl Pts',(17.6602453328089,21.0036629496068,37.7660261413564));
#53478=CARTESIAN_POINT('Ctrl Pts',(17.667257080226,21.0009963765664,37.7169032285298));
#53479=CARTESIAN_POINT('Ctrl Pts',(17.6758121746669,20.998329803526,37.6680277892764));
#53480=CARTESIAN_POINT('Ctrl Pts',(17.6858932263815,20.9956632304856,37.6194791563385));
#53481=CARTESIAN_POINT('Ctrl Pts',(17.7019167800207,20.9914247861888,37.542312443379));
#53482=CARTESIAN_POINT('Ctrl Pts',(17.7218343216131,20.9871863418919,37.4658039032194));
#53483=CARTESIAN_POINT('Ctrl Pts',(17.7455768104442,20.9829478975951,37.3903757872696));
#53484=CARTESIAN_POINT('Ctrl Pts',(17.7692852625888,20.9787155294346,37.315055803334));
#53485=CARTESIAN_POINT('Ctrl Pts',(17.796807632849,20.9744831612742,37.2408136109299));
#53486=CARTESIAN_POINT('Ctrl Pts',(17.8280239551717,20.9702507931137,37.168060891693));
#53487=CARTESIAN_POINT('Ctrl Pts',(17.8592043978289,20.9660232895863,37.0953917935567));
#53488=CARTESIAN_POINT('Ctrl Pts',(17.8940701712237,20.9617957860589,37.024209194865));
#53489=CARTESIAN_POINT('Ctrl Pts',(17.9324521150821,20.9575682825315,36.9549077834203));
#53490=CARTESIAN_POINT('Ctrl Pts',(17.9708099591438,20.9533434334287,36.8856498859238));
#53491=CARTESIAN_POINT('Ctrl Pts',(18.0126793649726,20.9491185843258,36.8182712399529));
#53492=CARTESIAN_POINT('Ctrl Pts',(18.0578443805922,20.944893735223,36.7531436635993));
#53493=CARTESIAN_POINT('Ctrl Pts',(18.1029950844597,20.9406702248774,36.688036724673));
#53494=CARTESIAN_POINT('Ctrl Pts',(18.151439057479,20.9364467145319,36.6251798236107));
#53495=CARTESIAN_POINT('Ctrl Pts',(18.2029168089793,20.9322232041863,36.5649161438375));
#53496=CARTESIAN_POINT('Ctrl Pts',(18.2543942584224,20.9279997186231,36.5046528176749));
#53497=CARTESIAN_POINT('Ctrl Pts',(18.3089051455131,20.92377623306,36.4469830378799));
#53498=CARTESIAN_POINT('Ctrl Pts',(18.3661504179376,20.9195527474968,36.3922160604765));
#53499=CARTESIAN_POINT('Ctrl Pts',(18.4234527579256,20.9153250515592,36.3373944861111));
#53500=CARTESIAN_POINT('Ctrl Pts',(18.4834945888465,20.9110973556216,36.2854818191307));
#53501=CARTESIAN_POINT('Ctrl Pts',(18.545941224779,20.906869659684,36.2367492066008));
#53502=CARTESIAN_POINT('Ctrl Pts',(18.6084182291228,20.9026399077764,36.1879928949236));
#53503=CARTESIAN_POINT('Ctrl Pts',(18.673301984301,20.8984101558689,36.1424199881516));
#53504=CARTESIAN_POINT('Ctrl Pts',(18.7402281479184,20.8941804039613,36.1002586863289));
#53505=CARTESIAN_POINT('Ctrl Pts',(18.8072746087764,20.8899430492351,36.0580216011654));
#53506=CARTESIAN_POINT('Ctrl Pts',(18.876370403896,20.8857056945089,36.0192086037558));
#53507=CARTESIAN_POINT('Ctrl Pts',(18.9471260920909,20.8814683397827,35.9840021325757));
#53508=CARTESIAN_POINT('Ctrl Pts',(19.0112907143594,20.8776257050439,35.9520752305512));
#53509=CARTESIAN_POINT('Ctrl Pts',(19.0768198616208,20.8737830703051,35.9231137278017));
#53510=CARTESIAN_POINT('Ctrl Pts',(19.1434112199942,20.8699404355663,35.8972185530861));
#53511=CARTESIAN_POINT('Ctrl Pts',(19.2168352001274,20.8657035263996,35.8686663979671));
#53512=CARTESIAN_POINT('Ctrl Pts',(19.2918266078201,20.8614666172328,35.8437355749677));
#53513=CARTESIAN_POINT('Ctrl Pts',(19.3679940539443,20.8572297080661,35.8225982073753));
#53514=CARTESIAN_POINT('Ctrl Pts',(19.4440517504979,20.852998903856,35.8014912965874));
#53515=CARTESIAN_POINT('Ctrl Pts',(19.5212816721688,20.848768099646,35.7841671107602));
#53516=CARTESIAN_POINT('Ctrl Pts',(19.5992735321796,20.844537295436,35.7707493181523));
#53517=CARTESIAN_POINT('Ctrl Pts',(19.6771750513255,20.8403113919234,35.7573470678713));
#53518=CARTESIAN_POINT('Ctrl Pts',(19.7558362950933,20.8360854884108,35.7478422978333));
#53519=CARTESIAN_POINT('Ctrl Pts',(19.8348344164102,20.8318595848983,35.7423081688021));
#53520=CARTESIAN_POINT('Ctrl Pts',(19.9137825196011,20.8276363570414,35.7367775437372));
#53521=CARTESIAN_POINT('Ctrl Pts',(19.9930666103936,20.8234131291846,35.7352126023477));
#53522=CARTESIAN_POINT('Ctrl Pts',(20.0722575189492,20.8191899013277,35.7376348098028));
#53523=CARTESIAN_POINT('Ctrl Pts',(20.1514229684259,20.8149680311961,35.7400562385427));
#53524=CARTESIAN_POINT('Ctrl Pts',(20.2304948267515,20.8107461610644,35.7464622563771));
#53525=CARTESIAN_POINT('Ctrl Pts',(20.3090442131256,20.8065242909328,35.7568222186028));
#53526=CARTESIAN_POINT('Ctrl Pts',(20.387592827256,20.8023024623076,35.7671820789765));
#53527=CARTESIAN_POINT('Ctrl Pts',(20.4656185148977,20.7980806336825,35.7814957437255));
#53528=CARTESIAN_POINT('Ctrl Pts',(20.5426992946748,20.7938588050574,35.7996809098607));
#53529=CARTESIAN_POINT('Ctrl Pts',(20.6198566757411,20.789632780866,35.8178841480389));
#53530=CARTESIAN_POINT('Ctrl Pts',(20.6960668157271,20.7854067566747,35.8399664649233));
#53531=CARTESIAN_POINT('Ctrl Pts',(20.7709202847241,20.7811807324833,35.8657949164186));
#53532=CARTESIAN_POINT('Ctrl Pts',(20.8458099792685,20.7769526630957,35.8916358676658));
#53533=CARTESIAN_POINT('Ctrl Pts',(20.9193412592673,20.772724593708,35.9212263898056));
#53534=CARTESIAN_POINT('Ctrl Pts',(20.9911245636103,20.7684965243204,35.9543852768243));
#53535=CARTESIAN_POINT('Ctrl Pts',(21.0630369701737,20.764260850753,35.9876038000771));
#53536=CARTESIAN_POINT('Ctrl Pts',(21.1331947033183,20.7600251771856,36.0244032930327));
#53537=CARTESIAN_POINT('Ctrl Pts',(21.2012329159404,20.7557895036182,36.0645565783935));
#53538=CARTESIAN_POINT('Ctrl Pts',(21.2631930631457,20.7519322159613,36.1011228457284));
#53539=CARTESIAN_POINT('Ctrl Pts',(21.3233955865241,20.7480749283044,36.1404697551222));
#53540=CARTESIAN_POINT('Ctrl Pts',(21.3815882815538,20.7442176406474,36.1823962189302));
#53541=CARTESIAN_POINT('Ctrl Pts',(21.4455221670195,20.7399797996754,36.2284590749934));
#53542=CARTESIAN_POINT('Ctrl Pts',(21.507269817599,20.7357419587034,36.2778092114351));
#53543=CARTESIAN_POINT('Ctrl Pts',(21.5664737493925,20.7315041177315,36.3302117546542));
#53544=CARTESIAN_POINT('Ctrl Pts',(21.6255925687079,20.7272723691445,36.3825389631754));
#53545=CARTESIAN_POINT('Ctrl Pts',(21.6821745834153,20.7230406205575,36.4379095558165));
#53546=CARTESIAN_POINT('Ctrl Pts',(21.735892690379,20.7188088719706,36.4960464444415));
#53547=CARTESIAN_POINT('Ctrl Pts',(21.7895487710125,20.7145820096287,36.5541162045311));
#53548=CARTESIAN_POINT('Ctrl Pts',(21.8403471989748,20.7103551472868,36.6149455705054));
#53549=CARTESIAN_POINT('Ctrl Pts',(21.8879964182131,20.7061282849448,36.6782194382696));
#53550=CARTESIAN_POINT('Ctrl Pts',(21.9356155691283,20.7019040899009,36.7414533780112));
#53551=CARTESIAN_POINT('Ctrl Pts',(21.9800891745965,20.6976798948569,36.8071283842608));
#53552=CARTESIAN_POINT('Ctrl Pts',(22.021165614587,20.6934556998129,36.8748959230697));
#53553=CARTESIAN_POINT('Ctrl Pts',(22.0622289200178,20.6892328554931,36.9426417926012));
#53554=CARTESIAN_POINT('Ctrl Pts',(22.0998969743171,20.6850100111733,37.0124784654269));
#53555=CARTESIAN_POINT('Ctrl Pts',(22.1339620363046,20.6807871668535,37.0840292974152));
#53556=CARTESIAN_POINT('Ctrl Pts',(22.168026809056,20.6765643583885,37.1555795218871));
#53557=CARTESIAN_POINT('Ctrl Pts',(22.1984884501264,20.6723415499236,37.2288434527625));
#53558=CARTESIAN_POINT('Ctrl Pts',(22.2251863134758,20.6681187414587,37.3034221248239));
#53559=CARTESIAN_POINT('Ctrl Pts',(22.2519107153947,20.6638917353809,37.3780749305809));
#53560=CARTESIAN_POINT('Ctrl Pts',(22.2748637079411,20.659664729303,37.4540446457334));
#53561=CARTESIAN_POINT('Ctrl Pts',(22.2939339613271,20.6554377232252,37.5309152769839));
#53562=CARTESIAN_POINT('Ctrl Pts',(22.3130134538007,20.6512086692627,37.6078231502409));
#53563=CARTESIAN_POINT('Ctrl Pts',(22.3282063697943,20.6469796153002,37.6856323484805));
#53564=CARTESIAN_POINT('Ctrl Pts',(22.3394526809638,20.6427505613377,37.7639172803742));
#53565=CARTESIAN_POINT('Ctrl Pts',(22.3507191953941,20.638513910157,37.8423428460157));
#53566=CARTESIAN_POINT('Ctrl Pts',(22.35802489553,20.6342772589763,37.9212453851012));
#53567=CARTESIAN_POINT('Ctrl Pts',(22.3613617695357,20.6300406077956,38.0001950187851));
#53568=CARTESIAN_POINT('Ctrl Pts',(22.3643929964548,20.6261920204398,38.0719131161635));
#53569=CARTESIAN_POINT('Ctrl Pts',(22.3641498335398,20.6223434330841,38.1436698003567));
#53570=CARTESIAN_POINT('Ctrl Pts',(22.3606634171487,20.6184948457283,38.2151463062182));
#53571=CARTESIAN_POINT('Ctrl Pts',(22.3568244818374,20.6142571195816,38.2938499524566));
#53572=CARTESIAN_POINT('Ctrl Pts',(22.3490381141486,20.6100193934349,38.3725090644142));
#53573=CARTESIAN_POINT('Ctrl Pts',(22.3373067419008,20.6057816672882,38.4506959297812));
#53574=CARTESIAN_POINT('Ctrl Pts',(22.3255922336675,20.6015500329332,38.5287704004171));
#53575=CARTESIAN_POINT('Ctrl Pts',(22.3099440519533,20.5973183985781,38.6063735128841));
#53576=CARTESIAN_POINT('Ctrl Pts',(22.2904165743647,20.593086764223,38.683080060348));
#53577=CARTESIAN_POINT('Ctrl Pts',(22.2709116382999,20.5888600146507,38.7596980616877));
#53578=CARTESIAN_POINT('Ctrl Pts',(22.2475364204582,20.5846332650784,38.8354211027636));
#53579=CARTESIAN_POINT('Ctrl Pts',(22.2203965385268,20.580406515506,38.9098331016933));
#53580=CARTESIAN_POINT('Ctrl Pts',(22.1932737771888,20.5761824322851,38.9841981594616));
#53581=CARTESIAN_POINT('Ctrl Pts',(22.162391225789,20.5719583490641,39.0572533774481));
#53582=CARTESIAN_POINT('Ctrl Pts',(22.1279042839611,20.5677342658431,39.1285979774431));
#53583=CARTESIAN_POINT('Ctrl Pts',(22.0934283608841,20.5635115322379,39.1999197824805));
#53584=CARTESIAN_POINT('Ctrl Pts',(22.0553505381311,20.5592887986327,39.2695316331428));
#53585=CARTESIAN_POINT('Ctrl Pts',(22.013873680876,20.5550660650275,39.3370542584603));
#53586=CARTESIAN_POINT('Ctrl Pts',(21.9723971633108,20.550843366006,39.4045763307767));
#53587=CARTESIAN_POINT('Ctrl Pts',(21.9275219131607,20.5466206669844,39.4700088131039));
#53588=CARTESIAN_POINT('Ctrl Pts',(21.87949515537,20.5423979679628,39.5329997912912));
#53589=CARTESIAN_POINT('Ctrl Pts',(21.8314206244279,20.5381710685402,39.5960534278315));
#53590=CARTESIAN_POINT('Ctrl Pts',(21.7801886088114,20.5339441691177,39.6566603354425));
#53591=CARTESIAN_POINT('Ctrl Pts',(21.7260874621062,20.5297172696951,39.7145007011642));
#53592=CARTESIAN_POINT('Ctrl Pts',(21.6719600866439,20.525488321031,39.7723691084525));
#53593=CARTESIAN_POINT('Ctrl Pts',(21.6149611465521,20.5212593723669,39.8274679757241));
#53594=CARTESIAN_POINT('Ctrl Pts',(21.5554149711715,20.5170304237028,39.8795153015233));
#53595=CARTESIAN_POINT('Ctrl Pts',(21.4957617723445,20.5127938742708,39.9316561729473));
#53596=CARTESIAN_POINT('Ctrl Pts',(21.4335525594428,20.5085573248387,39.9807342531313));
#53597=CARTESIAN_POINT('Ctrl Pts',(21.3691435720366,20.5043207754067,40.0265088424534));
#53598=CARTESIAN_POINT('Ctrl Pts',(21.3106178253108,20.5004712005408,40.0681022928246));
#53599=CARTESIAN_POINT('Ctrl Pts',(21.2502764098076,20.496621625675,40.1069685961243));
#53600=CARTESIAN_POINT('Ctrl Pts',(21.1884039076456,20.4927720508092,40.142960252475));
#53601=CARTESIAN_POINT('Ctrl Pts',(21.1202957754743,20.4885345083695,40.1825792173162));
#53602=CARTESIAN_POINT('Ctrl Pts',(21.0500763465617,20.4842969659297,40.218862981822));
#53603=CARTESIAN_POINT('Ctrl Pts',(20.9781056839902,20.48005942349,40.2515807472289));
#53604=CARTESIAN_POINT('Ctrl Pts',(20.9062385473929,20.4758279765299,40.2842514498686));
#53605=CARTESIAN_POINT('Ctrl Pts',(20.8326256029833,20.4715965295698,40.3133661476995));
#53606=CARTESIAN_POINT('Ctrl Pts',(20.7576530952229,20.4673650826097,40.3387389817036));
#53607=CARTESIAN_POINT('Ctrl Pts',(20.6827672186168,20.4631385251104,40.3640824972553));
#53608=CARTESIAN_POINT('Ctrl Pts',(20.6065253424046,20.4589119676111,40.3856925918189));
#53609=CARTESIAN_POINT('Ctrl Pts',(20.5293339526429,20.4546854101117,40.4034313550613));
#53610=CARTESIAN_POINT('Ctrl Pts',(20.4521913100054,20.4504615217252,40.4211589160997));
#53611=CARTESIAN_POINT('Ctrl Pts',(20.3741007997041,20.4462376333386,40.435019893715));
#53612=CARTESIAN_POINT('Ctrl Pts',(20.2954831726098,20.442013744952,40.444926466993));
#53613=CARTESIAN_POINT('Ctrl Pts',(20.2168907117464,20.4377912086712,40.4548298690852));
#53614=CARTESIAN_POINT('Ctrl Pts',(20.137771933949,20.4335686723905,40.4607813219791));
#53615=CARTESIAN_POINT('Ctrl Pts',(20.0585553895328,20.4293461361097,40.4627445285635));
#53616=CARTESIAN_POINT('Ctrl Pts',(19.9793395355902,20.4251236366338,40.464707718036));
#53617=CARTESIAN_POINT('Ctrl Pts',(19.9000263854131,20.4209011371578,40.4626827201305));
#53618=CARTESIAN_POINT('Ctrl Pts',(19.8210456905612,20.4166786376819,40.4566853409043));
#53619=CARTESIAN_POINT('Ctrl Pts',(19.7419864678658,20.412451939917,40.4506819986861));
#53620=CARTESIAN_POINT('Ctrl Pts',(19.6632608293097,20.4082252421521,40.440698421369));
#53621=CARTESIAN_POINT('Ctrl Pts',(19.5852939882527,20.4039985443872,40.4268023905611));
#53622=CARTESIAN_POINT('Ctrl Pts',(19.5072893735799,20.3997697988587,40.4128996273612));
#53623=CARTESIAN_POINT('Ctrl Pts',(19.4300447461438,20.3955410533302,40.3950807400925));
#53624=CARTESIAN_POINT('Ctrl Pts',(19.3539731854504,20.3913123078018,40.3734642719389));
#53625=CARTESIAN_POINT('Ctrl Pts',(19.2777648958508,20.3870759616438,40.3518089509471));
#53626=CARTESIAN_POINT('Ctrl Pts',(19.2027343308353,20.3828396154858,40.3263425617609));
#53627=CARTESIAN_POINT('Ctrl Pts',(19.1292772947068,20.3786032693277,40.2972328987586));
#53628=CARTESIAN_POINT('Ctrl Pts',(19.062496193662,20.3747519315152,40.2707687851923));
#53629=CARTESIAN_POINT('Ctrl Pts',(18.9970155875755,20.3709005937027,40.2412942454285));
#53630=CARTESIAN_POINT('Ctrl Pts',(18.93311451783,20.3670492558902,40.2089679487453));
#53631=CARTESIAN_POINT('Ctrl Pts',(18.8628033540714,20.3628115796712,40.1733989113433));
#53632=CARTESIAN_POINT('Ctrl Pts',(18.7941409339877,20.3585739034522,40.1342431012601));
#53633=CARTESIAN_POINT('Ctrl Pts',(18.7275168743918,20.3543362272333,40.0916769657609));
#53634=CARTESIAN_POINT('Ctrl Pts',(18.6609886168593,20.3501046445806,40.0491720382342));
#53635=CARTESIAN_POINT('Ctrl Pts',(18.5964932907581,20.345873061928,40.003266774239));
#53636=CARTESIAN_POINT('Ctrl Pts',(18.5343970626178,20.3416414792753,39.9541840444888));
#53637=CARTESIAN_POINT('Ctrl Pts',(18.4723725518753,20.3374147838454,39.9051580023307));
#53638=CARTESIAN_POINT('Ctrl Pts',(18.4127419986812,20.3331880884155,39.8529620764125));
#53639=CARTESIAN_POINT('Ctrl Pts',(18.3558423626936,20.3289613929855,39.7978622160196));
#53640=CARTESIAN_POINT('Ctrl Pts',(18.2989786407279,20.3247373653694,39.7427971336629));
#53641=CARTESIAN_POINT('Ctrl Pts',(18.2448427504704,20.3205133377532,39.6848320802046));
#53642=CARTESIAN_POINT('Ctrl Pts',(18.1937373959541,20.316289310137,39.6242722349126));
#53643=CARTESIAN_POINT('Ctrl Pts',(18.1426483868449,20.3120666335232,39.5637317589279));
#53644=CARTESIAN_POINT('Ctrl Pts',(18.0945882907818,20.3078439569093,39.5005984971424));
#53645=CARTESIAN_POINT('Ctrl Pts',(18.0498208341514,20.3036212802954,39.4352122160878));
#53646=CARTESIAN_POINT('Ctrl Pts',(18.0050537580744,20.2993986395771,39.3698264908604));
#53647=CARTESIAN_POINT('Ctrl Pts',(17.9635795294206,20.2951759988588,39.302188172045));
#53648=CARTESIAN_POINT('Ctrl Pts',(17.9256188197863,20.2909533581405,39.2326663939904));
#53649=CARTESIAN_POINT('Ctrl Pts',(17.8876203643672,20.2867265186891,39.1630754877741));
#53650=CARTESIAN_POINT('Ctrl Pts',(17.8531426316743,20.2824996792377,39.0915977937849));
#53651=CARTESIAN_POINT('Ctrl Pts',(17.8223602217603,20.2782728397863,39.0186269303302));
#53652=CARTESIAN_POINT('Ctrl Pts',(17.7915628953729,20.2740439521023,38.9456207068131));
#53653=CARTESIAN_POINT('Ctrl Pts',(17.7644646194336,20.2698150644182,38.8711203135116));
#53654=CARTESIAN_POINT('Ctrl Pts',(17.7411908066013,20.2655861767341,38.7955368205332));
#53655=CARTESIAN_POINT('Ctrl Pts',(17.7178751682447,20.2613496892878,38.7198174959552));
#53656=CARTESIAN_POINT('Ctrl Pts',(17.6983978413546,20.2571132018415,38.6430116379728));
#53657=CARTESIAN_POINT('Ctrl Pts',(17.6828335197367,20.2528767143951,38.5655426335408));
#53658=CARTESIAN_POINT('Ctrl Pts',(17.6686887939989,20.2490266299204,38.4951394481165));
#53659=CARTESIAN_POINT('Ctrl Pts',(17.6577752103282,20.2451765454458,38.4241889452537));
#53660=CARTESIAN_POINT('Ctrl Pts',(17.6501115451052,20.2413264609711,38.3530112457031));
#53661=CARTESIAN_POINT('Ctrl Pts',(17.6411212934931,20.2368099238901,38.2695126312));
#53662=CARTESIAN_POINT('Ctrl Pts',(17.6365804216128,20.2322933868092,38.1855264951044));
#53663=CARTESIAN_POINT('Ctrl Pts',(17.6365304175568,20.2277768497283,38.1014049076941));
#53664=CARTESIAN_POINT('',(17.6365302000601,19.4340268497732,38.1009724567951));
#53665=CARTESIAN_POINT('Ctrl Pts',(17.6365304175565,20.2277768497005,38.1014049071763));
#53666=CARTESIAN_POINT('Ctrl Pts',(17.636484138951,20.2235968064934,38.0235505989471));
#53667=CARTESIAN_POINT('Ctrl Pts',(17.6402889455708,20.2194167632863,37.9455442675965));
#53668=CARTESIAN_POINT('Ctrl Pts',(17.6479635155589,20.2152367200793,37.8678043567206));
#53669=CARTESIAN_POINT('Ctrl Pts',(17.6556272462681,20.2110625806106,37.7901742428201));
#53670=CARTESIAN_POINT('Ctrl Pts',(17.6671498382723,20.206888441142,37.7128102782396));
#53671=CARTESIAN_POINT('Ctrl Pts',(17.6824979511222,20.2027143016734,37.636130735716));
#53672=CARTESIAN_POINT('Ctrl Pts',(17.6978340511278,20.1985434292701,37.5595112096529));
#53673=CARTESIAN_POINT('Ctrl Pts',(17.7169896401562,20.1943725568669,37.4835755141203));
#53674=CARTESIAN_POINT('Ctrl Pts',(17.7398797370693,20.1902016844636,37.4087353343398));
#53675=CARTESIAN_POINT('Ctrl Pts',(17.7627594901109,20.1860326968478,37.3339289743031));
#53676=CARTESIAN_POINT('Ctrl Pts',(17.7893702621519,20.1818637092321,37.2602176082695));
#53677=CARTESIAN_POINT('Ctrl Pts',(17.8195766931931,20.1776947216163,37.1879996469116));
#53678=CARTESIAN_POINT('Ctrl Pts',(17.8497794653506,20.1735262389871,37.1157904332647));
#53679=CARTESIAN_POINT('Ctrl Pts',(17.8835768446866,20.1693577563579,37.0450747094514));
#53680=CARTESIAN_POINT('Ctrl Pts',(17.9207852401966,20.1651892737287,36.9762311520977));
#53681=CARTESIAN_POINT('Ctrl Pts',(17.9580268962399,20.1610170648986,36.9073260555832));
#53682=CARTESIAN_POINT('Ctrl Pts',(17.998685430597,20.1568448560685,36.8402968943004));
#53683=CARTESIAN_POINT('Ctrl Pts',(18.0425315311718,20.1526726472385,36.7754972123686));
#53684=CARTESIAN_POINT('Ctrl Pts',(18.086395999869,20.1484986905758,36.7106703843857));
#53685=CARTESIAN_POINT('Ctrl Pts',(18.1334504035067,20.1443247339132,36.648075281336));
#53686=CARTESIAN_POINT('Ctrl Pts',(18.1834239701309,20.1401507772506,36.5880337409171));
#53687=CARTESIAN_POINT('Ctrl Pts',(18.2334869365173,20.1359693536257,36.5278847897251));
#53688=CARTESIAN_POINT('Ctrl Pts',(18.2864791712429,20.1317879300009,36.4702988826972));
#53689=CARTESIAN_POINT('Ctrl Pts',(18.3420920191528,20.1276065063761,36.4155619429782));
#53690=CARTESIAN_POINT('Ctrl Pts',(18.3953045286807,20.1236055596014,36.3631875360599));
#53691=CARTESIAN_POINT('Ctrl Pts',(18.4509157702733,20.1196046128267,36.3134214308127));
#53692=CARTESIAN_POINT('Ctrl Pts',(18.5086289464615,20.115603666052,36.2664780280653));
#53693=CARTESIAN_POINT('Ctrl Pts',(18.5697562366471,20.1113660369581,36.2167576142609));
#53694=CARTESIAN_POINT('Ctrl Pts',(18.6334874181541,20.1071284078643,36.1700040667915));
#53695=CARTESIAN_POINT('Ctrl Pts',(18.6995026334712,20.1028907787704,36.1265013198506));
#53696=CARTESIAN_POINT('Ctrl Pts',(18.7654229125818,20.0986592437933,36.0830611340291));
#53697=CARTESIAN_POINT('Ctrl Pts',(18.8336203142797,20.0944277088162,36.0428627205079));
#53698=CARTESIAN_POINT('Ctrl Pts',(18.9037421375054,20.0901961738392,36.0061496854315));
#53699=CARTESIAN_POINT('Ctrl Pts',(18.9737829633769,20.0859695266862,35.9694790573914));
#53700=CARTESIAN_POINT('Ctrl Pts',(19.0457433801388,20.0817428795332,35.9362860235704));
#53701=CARTESIAN_POINT('Ctrl Pts',(19.119243243195,20.0775162323802,35.9067699673216));
#53702=CARTESIAN_POINT('Ctrl Pts',(19.1926967079603,20.0732922533846,35.8772725436867));
#53703=CARTESIAN_POINT('Ctrl Pts',(19.267687256218,20.069068274389,35.8514476645989));
#53704=CARTESIAN_POINT('Ctrl Pts',(19.343812871453,20.0648442953935,35.8294474475958));
#53705=CARTESIAN_POINT('Ctrl Pts',(19.4199141336261,20.0606216676753,35.8074542686001));
#53706=CARTESIAN_POINT('Ctrl Pts',(19.4971492916794,20.0563990399571,35.7892834520501));
#53707=CARTESIAN_POINT('Ctrl Pts',(19.5751006209999,20.0521764122389,35.7750374285539));
#53708=CARTESIAN_POINT('Ctrl Pts',(19.6530512838556,20.0479538206231,35.7607915268578));
#53709=CARTESIAN_POINT('Ctrl Pts',(19.7317176444084,20.0437312290074,35.7504704343655));
#53710=CARTESIAN_POINT('Ctrl Pts',(19.8106726977706,20.0395086373916,35.7441252975741));
#53711=CARTESIAN_POINT('Ctrl Pts',(19.8897062604247,20.035281847024,35.7377738514689));
#53712=CARTESIAN_POINT('Ctrl Pts',(19.9690286209409,20.0310550566564,35.7354062958549));
#53713=CARTESIAN_POINT('Ctrl Pts',(20.0482091834768,20.0268282662887,35.7370217276648));
#53714=CARTESIAN_POINT('Ctrl Pts',(20.1274281143302,20.0225994277564,35.7386379422601));
#53715=CARTESIAN_POINT('Ctrl Pts',(20.206504642121,20.018370589224,35.7442409559412));
#53716=CARTESIAN_POINT('Ctrl Pts',(20.285012271772,20.0141417506917,35.7537778353619));
#53717=CARTESIAN_POINT('Ctrl Pts',(20.3636609982,20.0099053119364,35.7633318548102));
#53718=CARTESIAN_POINT('Ctrl Pts',(20.4417383205281,20.0056688731811,35.7768337866482));
#53719=CARTESIAN_POINT('Ctrl Pts',(20.5188271578966,20.0014324344259,35.7941793605901));
#53720=CARTESIAN_POINT('Ctrl Pts',(20.588893600923,19.9975819133282,35.8099448424658));
#53721=CARTESIAN_POINT('Ctrl Pts',(20.6581433553679,19.9937313922306,35.8288848728598));
#53722=CARTESIAN_POINT('Ctrl Pts',(20.7262763156345,19.9898808711329,35.8508861402214));
#53723=CARTESIAN_POINT('Ctrl Pts',(20.8012592810361,19.9856432233173,35.8750993883015));
#53724=CARTESIAN_POINT('Ctrl Pts',(20.8751708046757,19.9814055755017,35.9031119602584));
#53725=CARTESIAN_POINT('Ctrl Pts',(20.9475985911541,19.9771679276862,35.934810088943));
#53726=CARTESIAN_POINT('Ctrl Pts',(21.0199222248094,19.9729363737056,35.9664626349894));
#53727=CARTESIAN_POINT('Ctrl Pts',(21.0907659326345,19.9687048197251,36.0017900262271));
#53728=CARTESIAN_POINT('Ctrl Pts',(21.1597333717074,19.9644732657445,36.0406289922775));
#53729=CARTESIAN_POINT('Ctrl Pts',(21.2286211526561,19.9602465992537,36.0794230989098));
#53730=CARTESIAN_POINT('Ctrl Pts',(21.2956365650567,19.956019932763,36.1217204913904));
#53731=CARTESIAN_POINT('Ctrl Pts',(21.3604054249507,19.9517932662722,36.1673108059844));
#53732=CARTESIAN_POINT('Ctrl Pts',(21.4251334013478,19.9475692677442,36.2128723429916));
#53733=CARTESIAN_POINT('Ctrl Pts',(21.4876172576274,19.9433452692162,36.2617224072757));
#53734=CARTESIAN_POINT('Ctrl Pts',(21.5475105542658,19.9391212706881,36.3136065591993));
#53735=CARTESIAN_POINT('Ctrl Pts',(21.607384693123,19.9348986232703,36.3654741151883));
#53736=CARTESIAN_POINT('Ctrl Pts',(21.6646695637755,19.9306759758524,36.4203735248843));
#53737=CARTESIAN_POINT('Ctrl Pts',(21.7190518572336,19.9264533284345,36.4780101254811));
#53738=CARTESIAN_POINT('Ctrl Pts',(21.7734336875416,19.922230716979,36.5356462352124));
#53739=CARTESIAN_POINT('Ctrl Pts',(21.8249126691398,19.9180081055235,36.5960191475558));
#53740=CARTESIAN_POINT('Ctrl Pts',(21.8732134622141,19.9137854940681,36.6587984992098));
#53741=CARTESIAN_POINT('Ctrl Pts',(21.9215622840979,19.9095586837788,36.7216402767027));
#53742=CARTESIAN_POINT('Ctrl Pts',(21.9667263182471,19.9053318734896,36.7868929009139));
#53743=CARTESIAN_POINT('Ctrl Pts',(22.0084719329765,19.9011050632003,36.854194663944));
#53744=CARTESIAN_POINT('Ctrl Pts',(22.0502377769302,19.8968762046698,36.921529040279));
#53745=CARTESIAN_POINT('Ctrl Pts',(22.0885816744786,19.8926473461392,36.9909141227472));
#53746=CARTESIAN_POINT('Ctrl Pts',(22.1233158727043,19.8884184876086,37.0619633216394));
#53747=CARTESIAN_POINT('Ctrl Pts',(22.1581124953498,19.8841820289591,37.1331402103948));
#53748=CARTESIAN_POINT('Ctrl Pts',(22.1892862714249,19.8799455703095,37.2059867594037));
#53749=CARTESIAN_POINT('Ctrl Pts',(22.2166976374358,19.8757091116599,37.2800963318252));
#53750=CARTESIAN_POINT('Ctrl Pts',(22.2416107143402,19.8718587665112,37.3474515112919));
#53751=CARTESIAN_POINT('Ctrl Pts',(22.2634164966769,19.8680084213625,37.4158495119528));
#53752=CARTESIAN_POINT('Ctrl Pts',(22.2820466887331,19.8641580762139,37.4849769505601));
#53753=CARTESIAN_POINT('Ctrl Pts',(22.3025508506449,19.859920433354,37.5610577654804));
#53754=CARTESIAN_POINT('Ctrl Pts',(22.3192846692418,19.8556827904941,37.6383078896525));
#53755=CARTESIAN_POINT('Ctrl Pts',(22.3321191526145,19.8514451476342,37.7163195354094));
#53756=CARTESIAN_POINT('Ctrl Pts',(22.3449351795729,19.8472135986458,37.7942189978223));
#53757=CARTESIAN_POINT('Ctrl Pts',(22.3538629315615,19.8429820496574,37.8728773483324));
#53758=CARTESIAN_POINT('Ctrl Pts',(22.3588236267975,19.8387505006691,37.9518732348229));
#53759=CARTESIAN_POINT('Ctrl Pts',(22.363778592335,19.8345238392013,38.0307778795422));
#53760=CARTESIAN_POINT('Ctrl Pts',(22.3647755775293,19.8302971777336,38.1100188200074));
#53761=CARTESIAN_POINT('Ctrl Pts',(22.3617873675864,19.8260705162658,38.1891676578667));
#53762=CARTESIAN_POINT('Ctrl Pts',(22.3588010438797,19.8218465227772,38.2682665349113));
#53763=CARTESIAN_POINT('Ctrl Pts',(22.3518345357827,19.8176225292887,38.3472729575328));
#53764=CARTESIAN_POINT('Ctrl Pts',(22.3409127046275,19.8133985358001,38.4257578091368));
#53765=CARTESIAN_POINT('Ctrl Pts',(22.3299943670141,19.8091758934309,38.5042175559662));
#53766=CARTESIAN_POINT('Ctrl Pts',(22.3151232833054,19.8049532510617,38.5821555991126));
#53767=CARTESIAN_POINT('Ctrl Pts',(22.2963760908792,19.8007306086925,38.6591487191602));
#53768=CARTESIAN_POINT('Ctrl Pts',(22.277629058124,19.7965080022878,38.7361411834523));
#53769=CARTESIAN_POINT('Ctrl Pts',(22.2550060945822,19.7922853958832,38.8121882855207));
#53770=CARTESIAN_POINT('Ctrl Pts',(22.2286344535998,19.7880627894785,38.8868792239778));
#53771=CARTESIAN_POINT('Ctrl Pts',(22.2022365892431,19.7838359842078,38.9616444334458));
#53772=CARTESIAN_POINT('Ctrl Pts',(22.1720827579782,19.7796091789371,39.0350503425325));
#53773=CARTESIAN_POINT('Ctrl Pts',(22.1383492103446,19.7753823736664,39.1067040754455));
#53774=CARTESIAN_POINT('Ctrl Pts',(22.1045993159032,19.7711535201446,39.1783925307605));
#53775=CARTESIAN_POINT('Ctrl Pts',(22.0672664704473,19.7669246666229,39.2483267043674));
#53776=CARTESIAN_POINT('Ctrl Pts',(22.0265727705049,19.7626958131012,39.316138662632));
#53777=CARTESIAN_POINT('Ctrl Pts',(21.9858059348948,19.7584593593851,39.3840724941313));
#53778=CARTESIAN_POINT('Ctrl Pts',(21.9416664376352,19.7542229056691,39.4498760991301));
#53779=CARTESIAN_POINT('Ctrl Pts',(21.8944194233604,19.7499864519531,39.5132110561749));
#53780=CARTESIAN_POINT('Ctrl Pts',(21.8514779789693,19.7461360617336,39.5707743663161));
#53781=CARTESIAN_POINT('Ctrl Pts',(21.8059702735828,19.7422856715142,39.6262986659425));
#53782=CARTESIAN_POINT('Ctrl Pts',(21.758122026966,19.7384352812947,39.6795560702923));
#53783=CARTESIAN_POINT('Ctrl Pts',(21.7054614747271,19.7341976406364,39.7381698027102));
#53784=CARTESIAN_POINT('Ctrl Pts',(21.6497676973461,19.7299599999782,39.7942572176017));
#53785=CARTESIAN_POINT('Ctrl Pts',(21.5913125590873,19.7257223593199,39.8474881344922));
#53786=CARTESIAN_POINT('Ctrl Pts',(21.5329414820595,19.7214908125876,39.9006425028271));
#53787=CARTESIAN_POINT('Ctrl Pts',(21.471817273861,19.7172592658554,39.9509482178125));
#53788=CARTESIAN_POINT('Ctrl Pts',(21.4082505087409,19.7130277191232,39.9981098349493));
#53789=CARTESIAN_POINT('Ctrl Pts',(21.3447571655755,19.7088010599833,40.0452169786814));
#53790=CARTESIAN_POINT('Ctrl Pts',(21.2788272465766,19.7045744008434,40.0891869634653));
#53791=CARTESIAN_POINT('Ctrl Pts',(21.2108053066442,19.7003477417035,40.1297637671173));
#53792=CARTESIAN_POINT('Ctrl Pts',(21.1428263046473,19.6961237505853,40.1703149572074));
#53793=CARTESIAN_POINT('Ctrl Pts',(21.0727583044157,19.6918997594672,40.2074769780759));
#53794=CARTESIAN_POINT('Ctrl Pts',(21.0009748102995,19.6876757683491,40.2410371015108));
#53795=CARTESIAN_POINT('Ctrl Pts',(20.9292142780913,19.6834531283897,40.2745864898252));
#53796=CARTESIAN_POINT('Ctrl Pts',(20.8557397660526,19.6792304884303,40.3045360702867));
#53797=CARTESIAN_POINT('Ctrl Pts',(20.7809480151741,19.6750078484709,40.3307197579471));
#53798=CARTESIAN_POINT('Ctrl Pts',(20.7061569019417,19.6707852445122,40.3569032223753));
#53799=CARTESIAN_POINT('Ctrl Pts',(20.6300490151142,19.6665626405534,40.3793207042952));
#53800=CARTESIAN_POINT('Ctrl Pts',(20.5530382307178,19.6623400365946,40.3978553384111));
#53801=CARTESIAN_POINT('Ctrl Pts',(20.4759508691915,19.6581132338098,40.416408402791));
#53802=CARTESIAN_POINT('Ctrl Pts',(20.3979592735295,19.6538864310249,40.4310707970902));
#53803=CARTESIAN_POINT('Ctrl Pts',(20.3194889535093,19.6496596282401,40.4417765157003));
#53804=CARTESIAN_POINT('Ctrl Pts',(20.2409806083215,19.64543077723,40.4524874220903));
#53805=CARTESIAN_POINT('Ctrl Pts',(20.1619935443124,19.64120192622,40.4592377932839));
#53806=CARTESIAN_POINT('Ctrl Pts',(20.0829573037273,19.63697307521,40.462013659287));
#53807=CARTESIAN_POINT('Ctrl Pts',(20.003779017554,19.6327366240203,40.4647945141347));
#53808=CARTESIAN_POINT('Ctrl Pts',(19.9245518480421,19.6285001728305,40.4635865984202));
#53809=CARTESIAN_POINT('Ctrl Pts',(19.8457040132688,19.6242637216408,40.4584281183404));
#53810=CARTESIAN_POINT('Ctrl Pts',(19.7740410538062,19.6204133098858,40.4537396960152));
#53811=CARTESIAN_POINT('Ctrl Pts',(19.702691649299,19.6165628981307,40.4457885773075));
#53812=CARTESIAN_POINT('Ctrl Pts',(19.6319698377279,19.6127124863756,40.4346400665966));
#53813=CARTESIAN_POINT('Ctrl Pts',(19.5541356153086,19.6084748431607,40.422370363049));
#53814=CARTESIAN_POINT('Ctrl Pts',(19.4767695491811,19.6042371999458,40.4061810158533));
#53815=CARTESIAN_POINT('Ctrl Pts',(19.4002966028418,19.5999995567309,40.3861203547357));
#53816=CARTESIAN_POINT('Ctrl Pts',(19.3239336273925,19.5957680074017,40.3660885415815));
#53817=CARTESIAN_POINT('Ctrl Pts',(19.2484616708388,19.5915364580726,40.3421965881955));
#53818=CARTESIAN_POINT('Ctrl Pts',(19.174297628942,19.5873049087434,40.3145442048713));
#53819=CARTESIAN_POINT('Ctrl Pts',(19.1002192483423,19.583078246958,40.2869237607317));
#53820=CARTESIAN_POINT('Ctrl Pts',(19.0274462173227,19.5788515851727,40.255551681003));
#53821=CARTESIAN_POINT('Ctrl Pts',(18.9563808583605,19.5746249233873,40.220577640197));
#53822=CARTESIAN_POINT('Ctrl Pts',(18.8853603579469,19.5704009295954,40.1856256760362));
#53823=CARTESIAN_POINT('Ctrl Pts',(18.8160458095101,19.5661769358035,40.1470764702211));
#53824=CARTESIAN_POINT('Ctrl Pts',(18.7488189757804,19.5619529420116,40.1051275484449));
#53825=CARTESIAN_POINT('Ctrl Pts',(18.6816136459818,19.5577302993539,40.0631920449227));
#53826=CARTESIAN_POINT('Ctrl Pts',(18.6164951021841,19.5535076566961,40.0178592329244));
#53827=CARTESIAN_POINT('Ctrl Pts',(18.5538186280841,19.5492850140384,39.9693715201702));
#53828=CARTESIAN_POINT('Ctrl Pts',(18.4911426880302,19.5450624073605,39.9208842205643));
#53829=CARTESIAN_POINT('Ctrl Pts',(18.4309091461991,19.5408398006825,39.8692423616193));
#53830=CARTESIAN_POINT('Ctrl Pts',(18.3734413246954,19.5366171940046,39.8147295170642));
#53831=CARTESIAN_POINT('Ctrl Pts',(18.3159163588249,19.5323903884867,39.7601624664873));
#53832=CARTESIAN_POINT('Ctrl Pts',(18.261162947618,19.5281635829688,39.7027190511352));
#53833=CARTESIAN_POINT('Ctrl Pts',(18.2094680812797,19.5239367774509,39.6427202886278));
#53834=CARTESIAN_POINT('Ctrl Pts',(18.1577481645001,19.5197079236959,39.5826924517541));
#53835=CARTESIAN_POINT('Ctrl Pts',(18.1090900332376,19.5154790699409,39.5201071714882));
#53836=CARTESIAN_POINT('Ctrl Pts',(18.0637392217108,19.5112502161859,39.4553171729743));
#53837=CARTESIAN_POINT('Ctrl Pts',(18.0183069049348,19.507013762263,39.3904107327738));
#53838=CARTESIAN_POINT('Ctrl Pts',(17.9761940342619,19.5027773083402,39.3232920551766));
#53839=CARTESIAN_POINT('Ctrl Pts',(17.9376016541955,19.4985408544173,39.2543411558647));
#53840=CARTESIAN_POINT('Ctrl Pts',(17.9025261815392,19.4946904667638,39.1916737230896));
#53841=CARTESIAN_POINT('Ctrl Pts',(17.870358322029,19.4908400791102,39.1274933400953));
#53842=CARTESIAN_POINT('Ctrl Pts',(17.8412142337764,19.4869896914566,39.0620989847467));
#53843=CARTESIAN_POINT('Ctrl Pts',(17.8061044677336,19.4823511449177,38.9833186675543));
#53844=CARTESIAN_POINT('Ctrl Pts',(17.7752695283484,19.4777125983789,38.9025216574394));
#53845=CARTESIAN_POINT('Ctrl Pts',(17.7489228730776,19.47307405184,38.820168181432));
#53846=CARTESIAN_POINT('Ctrl Pts',(17.7226474238737,19.468448041718,38.7380372789183));
#53847=CARTESIAN_POINT('Ctrl Pts',(17.7008361972315,19.4638220315961,38.654358589239));
#53848=CARTESIAN_POINT('Ctrl Pts',(17.6836548021214,19.4591960214741,38.5696119303901));
#53849=CARTESIAN_POINT('Ctrl Pts',(17.6665514361944,19.4545910203441,38.4852501478869));
#53850=CARTESIAN_POINT('Ctrl Pts',(17.6540360738757,19.4499860192141,38.3998303703967));
#53851=CARTESIAN_POINT('Ctrl Pts',(17.6462241266023,19.4453810180841,38.3138447537604));
#53852=CARTESIAN_POINT('Ctrl Pts',(17.6398037036987,19.4415962953138,38.2431755591149));
#53853=CARTESIAN_POINT('Ctrl Pts',(17.6365594758146,19.4378115725435,38.1721245756472));
#53854=CARTESIAN_POINT('Ctrl Pts',(17.6365302000601,19.4340268497732,38.1009724567951));
#53855=CARTESIAN_POINT('',(17.6365309432187,18.6402768496835,38.0978884751228));
#53856=CARTESIAN_POINT('Ctrl Pts',(17.6365302000598,19.4340268497283,38.1009724559519));
#53857=CARTESIAN_POINT('Ctrl Pts',(17.63649691118,19.4297233127912,38.0200667225018));
#53858=CARTESIAN_POINT('Ctrl Pts',(17.6406222859428,19.4254197758541,37.9391804309353));
#53859=CARTESIAN_POINT('Ctrl Pts',(17.6488740476656,19.421116238917,37.8587590475074));
#53860=CARTESIAN_POINT('Ctrl Pts',(17.6571302401675,19.416810391198,37.7782944818598));
#53861=CARTESIAN_POINT('Ctrl Pts',(17.6695171805407,19.412504543479,37.6982957614949));
#53862=CARTESIAN_POINT('Ctrl Pts',(17.6859509702447,19.40819869576,37.6192011555873));
#53863=CARTESIAN_POINT('Ctrl Pts',(17.7024111899348,19.4038859230713,37.5399793441248));
#53864=CARTESIAN_POINT('Ctrl Pts',(17.722931163855,19.3995731503826,37.4616649852144));
#53865=CARTESIAN_POINT('Ctrl Pts',(17.7473763108829,19.3952603776939,37.3846840165853));
#53866=CARTESIAN_POINT('Ctrl Pts',(17.7718426238678,19.3909438707687,37.3076363935866));
#53867=CARTESIAN_POINT('Ctrl Pts',(17.8002407241596,19.3866273638435,37.2319248753286));
#53868=CARTESIAN_POINT('Ctrl Pts',(17.8323876855168,19.3823108569183,37.1579557892536));
#53869=CARTESIAN_POINT('Ctrl Pts',(17.864600726392,19.3779854772199,37.0838346564112));
#53870=CARTESIAN_POINT('Ctrl Pts',(17.9005778246042,19.3736600975215,37.0114635075962));
#53871=CARTESIAN_POINT('Ctrl Pts',(17.9400898782929,19.3693347178231,36.9412244689378));
#53872=CARTESIAN_POINT('Ctrl Pts',(17.9646562138912,19.3666454440612,36.8975538511211));
#53873=CARTESIAN_POINT('Ctrl Pts',(17.9905881561757,19.3639561702994,36.8547068782714));
#53874=CARTESIAN_POINT('Ctrl Pts',(18.0178225475708,19.3612668965376,36.8127692561234));
#53875=CARTESIAN_POINT('Ctrl Pts',(18.0607373325429,19.357029254376,36.7466857512411));
#53876=CARTESIAN_POINT('Ctrl Pts',(18.1070410082588,19.3527916122144,36.6826266423791));
#53877=CARTESIAN_POINT('Ctrl Pts',(18.1565163086918,19.3485539700528,36.6209603383341));
#53878=CARTESIAN_POINT('Ctrl Pts',(18.2059204616512,19.3443224217913,36.5593827129168));
#53879=CARTESIAN_POINT('Ctrl Pts',(18.2584868908242,19.3400908735297,36.5001914215271));
#53880=CARTESIAN_POINT('Ctrl Pts',(18.3139546935983,19.3358593252681,36.4437265727964));
#53881=CARTESIAN_POINT('Ctrl Pts',(18.3693584294601,19.3316326645669,36.3873269425949));
#53882=CARTESIAN_POINT('Ctrl Pts',(18.4276565524602,19.3274060038657,36.3336478296785));
#53883=CARTESIAN_POINT('Ctrl Pts',(18.4885484672282,19.3231793431644,36.2829956783261));
#53884=CARTESIAN_POINT('Ctrl Pts',(18.5494019450779,19.3189553504662,36.2323755002267));
#53885=CARTESIAN_POINT('Ctrl Pts',(18.6128456054235,19.314731357768,36.1847787901325));
#53886=CARTESIAN_POINT('Ctrl Pts',(18.6785435287391,19.3105073650697,36.1404737216708));
#53887=CARTESIAN_POINT('Ctrl Pts',(18.7442204370482,19.3062847235136,36.0961828252142));
#53888=CARTESIAN_POINT('Ctrl Pts',(18.8121497880337,19.3020620819576,36.0551817414331));
#53889=CARTESIAN_POINT('Ctrl Pts',(18.8819654611021,19.2978394404015,36.0176961771318));
#53890=CARTESIAN_POINT('Ctrl Pts',(18.9517805391862,19.2936168348317,35.9802109322907));
#53891=CARTESIAN_POINT('Ctrl Pts',(19.0234814937076,19.2893942292619,35.9462413678524));
#53892=CARTESIAN_POINT('Ctrl Pts',(19.0966776302458,19.2851716236921,35.91596723074));
#53893=CARTESIAN_POINT('Ctrl Pts',(19.1699465509169,19.2809448192847,35.8856629898964));
#53894=CARTESIAN_POINT('Ctrl Pts',(19.2447131892359,19.2767180148774,35.8590616960446));
#53895=CARTESIAN_POINT('Ctrl Pts',(19.3205674566373,19.2724912104701,35.8362946614191));
#53896=CARTESIAN_POINT('Ctrl Pts',(19.3964584816635,19.2682623578287,35.8135165942948));
#53897=CARTESIAN_POINT('Ctrl Pts',(19.4734377299283,19.2640335051874,35.7945765999174));
#53898=CARTESIAN_POINT('Ctrl Pts',(19.5510830450083,19.2598046525461,35.7795552132358));
#53899=CARTESIAN_POINT('Ctrl Pts',(19.6288679057476,19.2555681997291,35.7645068298282));
#53900=CARTESIAN_POINT('Ctrl Pts',(19.7073207599213,19.2513317469122,35.7533911918268));
#53901=CARTESIAN_POINT('Ctrl Pts',(19.7860126529992,19.2470952940952,35.7462370858084));
#53902=CARTESIAN_POINT('Ctrl Pts',(19.8575335882865,19.2432448966029,35.7397349121592));
#53903=CARTESIAN_POINT('Ctrl Pts',(19.9292516733776,19.2393944991107,35.7365045079458));
#53904=CARTESIAN_POINT('Ctrl Pts',(20.0008465413715,19.2355441016184,35.736530151606));
#53905=CARTESIAN_POINT('Ctrl Pts',(20.0796419011123,19.2313064591162,35.7365583743193));
#53906=CARTESIAN_POINT('Ctrl Pts',(20.1585837540419,19.2270688166141,35.7405313790339));
#53907=CARTESIAN_POINT('Ctrl Pts',(20.2372447882762,19.2228311741119,35.7484674462522));
#53908=CARTESIAN_POINT('Ctrl Pts',(20.3157927048903,19.2185996255041,35.7563921010978));
#53909=CARTESIAN_POINT('Ctrl Pts',(20.3940601422223,19.2143680768964,35.7682684540193));
#53910=CARTESIAN_POINT('Ctrl Pts',(20.4716197755453,19.2101365282886,35.7840627754158));
#53911=CARTESIAN_POINT('Ctrl Pts',(20.5490898253874,19.2059098672343,35.7998388539426));
#53912=CARTESIAN_POINT('Ctrl Pts',(20.6258532388433,19.2016832061799,35.8195238148475));
#53913=CARTESIAN_POINT('Ctrl Pts',(20.7014893249499,19.1974565451256,35.8430323068592));
#53914=CARTESIAN_POINT('Ctrl Pts',(20.7770776672229,19.1932325520703,35.8665259595846));
#53915=CARTESIAN_POINT('Ctrl Pts',(20.8515396481232,19.189008559015,35.8938382140542));
#53916=CARTESIAN_POINT('Ctrl Pts',(20.9244674525116,19.1847845659597,35.9248332546339));
#53917=CARTESIAN_POINT('Ctrl Pts',(20.9973719293108,19.180561924043,35.9558183807567));
#53918=CARTESIAN_POINT('Ctrl Pts',(21.068742772998,19.1763392821263,35.9904837704438));
#53919=CARTESIAN_POINT('Ctrl Pts',(21.1381913529671,19.1721166402096,36.0286451571662));
#53920=CARTESIAN_POINT('Ctrl Pts',(21.20763934113,19.1678940342762,36.0668062186963));
#53921=CARTESIAN_POINT('Ctrl Pts',(21.2751646879985,19.1636714283428,36.1084629910251));
#53922=CARTESIAN_POINT('Ctrl Pts',(21.3404039408185,19.1594488224093,36.1533855758424));
#53923=CARTESIAN_POINT('Ctrl Pts',(21.4057080657035,19.1552220176362,36.1983528304057));
#53924=CARTESIAN_POINT('Ctrl Pts',(21.4687211687671,19.150995212863,36.2465921177412));
#53925=CARTESIAN_POINT('Ctrl Pts',(21.529109870627,19.1467684080899,36.2978309056997));
#53926=CARTESIAN_POINT('Ctrl Pts',(21.5895278357976,19.1425395550809,36.3490945230804));
#53927=CARTESIAN_POINT('Ctrl Pts',(21.6473185241433,19.1383107020719,36.40336021534));
#53928=CARTESIAN_POINT('Ctrl Pts',(21.702184582739,19.134081849063,36.4603176871157));
#53929=CARTESIAN_POINT('Ctrl Pts',(21.7571492476496,19.1298453958797,36.5173775239335));
#53930=CARTESIAN_POINT('Ctrl Pts',(21.809178471871,19.1256089426963,36.5771384521025));
#53931=CARTESIAN_POINT('Ctrl Pts',(21.8580146120605,19.121372489513,36.6392563050728));
#53932=CARTESIAN_POINT('Ctrl Pts',(21.9024004193097,19.1175220952418,36.6957134910415));
#53933=CARTESIAN_POINT('Ctrl Pts',(21.9441489652272,19.1136717009706,36.7541169965109));
#53934=CARTESIAN_POINT('Ctrl Pts',(21.9830990514481,19.1098213066993,36.8141895190015));
#53935=CARTESIAN_POINT('Ctrl Pts',(22.0259664888743,19.1055836643344,36.8803037525952));
#53936=CARTESIAN_POINT('Ctrl Pts',(22.0656045182654,19.1013460219694,36.9486881595004));
#53937=CARTESIAN_POINT('Ctrl Pts',(22.1017652036544,19.0971083796045,37.0189942323893));
#53938=CARTESIAN_POINT('Ctrl Pts',(22.1378738885597,19.0928768311355,37.0891992023881));
#53939=CARTESIAN_POINT('Ctrl Pts',(22.1705149474696,19.0886452826664,37.16131993703));
#53940=CARTESIAN_POINT('Ctrl Pts',(22.1994840670144,19.0844137341974,37.2349796072636));
#53941=CARTESIAN_POINT('Ctrl Pts',(22.2284197264279,19.0801870732834,37.3085541985484));
#53942=CARTESIAN_POINT('Ctrl Pts',(22.2536917040894,19.0759604123695,37.3836637590193));
#53943=CARTESIAN_POINT('Ctrl Pts',(22.2751426013675,19.0717337514555,37.4599089249624));
#53944=CARTESIAN_POINT('Ctrl Pts',(22.2965799581715,19.0675097585415,37.5361059625835));
#53945=CARTESIAN_POINT('Ctrl Pts',(22.3142008954915,19.0632857656275,37.6134367327756));
#53946=CARTESIAN_POINT('Ctrl Pts',(22.3278973563818,19.0590617727134,37.6914852033883));
#53947=CARTESIAN_POINT('Ctrl Pts',(22.3415894361502,19.0548391309388,37.7695087084378));
#53948=CARTESIAN_POINT('Ctrl Pts',(22.3513594513638,19.0506164891641,37.848248996637));
#53949=CARTESIAN_POINT('Ctrl Pts',(22.3571504317852,19.0463938473895,37.927279755573));
#53950=CARTESIAN_POINT('Ctrl Pts',(22.362941362858,19.0421712415986,38.0063098410382));
#53951=CARTESIAN_POINT('Ctrl Pts',(22.3647532937258,19.0379486358077,38.0856299246948));
#53952=CARTESIAN_POINT('Ctrl Pts',(22.3625812383724,19.0337260300168,38.1648099760127));
#53953=CARTESIAN_POINT('Ctrl Pts',(22.3604070231885,19.0294992253861,38.2440687617366));
#53954=CARTESIAN_POINT('Ctrl Pts',(22.3542409214272,19.0252724207553,38.3231867672943));
#53955=CARTESIAN_POINT('Ctrl Pts',(22.3441300812228,19.0210456161245,38.4017359826181));
#53956=CARTESIAN_POINT('Ctrl Pts',(22.3340143414819,19.0168167632581,38.4803232615191));
#53957=CARTESIAN_POINT('Ctrl Pts',(22.3199501385357,19.0125879103916,38.55834073918));
#53958=CARTESIAN_POINT('Ctrl Pts',(22.3020359093354,19.0083590575252,38.6353700711007));
#53959=CARTESIAN_POINT('Ctrl Pts',(22.2840894843374,19.0041226044829,38.7125378416199));
#53960=CARTESIAN_POINT('Ctrl Pts',(22.2622793369081,18.9998861514407,38.7887134662149));
#53961=CARTESIAN_POINT('Ctrl Pts',(22.2367539327763,18.9956496983985,38.8634934741764));
#53962=CARTESIAN_POINT('Ctrl Pts',(22.2135545956821,18.9917993028591,38.931458964699));
#53963=CARTESIAN_POINT('Ctrl Pts',(22.1872869971439,18.9879489073197,38.9982715923177));
#53964=CARTESIAN_POINT('Ctrl Pts',(22.1580960113827,18.9840985117803,39.0636451870654));
#53965=CARTESIAN_POINT('Ctrl Pts',(22.1259691931705,18.9798608694289,39.1355936170194));
#53966=CARTESIAN_POINT('Ctrl Pts',(22.0901801186355,18.9756232270776,39.2060687372696));
#53967=CARTESIAN_POINT('Ctrl Pts',(22.050886178917,18.9713855847262,39.274672857449));
#53968=CARTESIAN_POINT('Ctrl Pts',(22.011648745431,18.9671540362714,39.3431783222022));
#53969=CARTESIAN_POINT('Ctrl Pts',(21.9689166870622,18.9629224878167,39.4098177266965));
#53970=CARTESIAN_POINT('Ctrl Pts',(21.9228948984556,18.9586909393619,39.4742145576268));
#53971=CARTESIAN_POINT('Ctrl Pts',(21.8769262662932,18.9544642784631,39.5385370084286));
#53972=CARTESIAN_POINT('Ctrl Pts',(21.8276757260957,18.9502376175643,39.6006216536557));
#53973=CARTESIAN_POINT('Ctrl Pts',(21.7753926134654,18.9460109566655,39.6601190688382));
#53974=CARTESIAN_POINT('Ctrl Pts',(21.72314250357,18.9417869637672,39.7195789273925));
#53975=CARTESIAN_POINT('Ctrl Pts',(21.667863929452,18.9375629708689,39.7764544462935));
#53976=CARTESIAN_POINT('Ctrl Pts',(21.6098470677578,18.9333389779706,39.8304285189894));
#53977=CARTESIAN_POINT('Ctrl Pts',(21.5518487640723,18.9291163362122,39.8843853268543));
#53978=CARTESIAN_POINT('Ctrl Pts',(21.4911142551494,18.9248936944538,39.9354422124553));
#53979=CARTESIAN_POINT('Ctrl Pts',(21.4279701497255,18.9206710526954,39.9833193283118));
#53980=CARTESIAN_POINT('Ctrl Pts',(21.3648265823997,18.9164484469212,40.0311960361717));
#53981=CARTESIAN_POINT('Ctrl Pts',(21.2992738338036,18.9122258411471,40.0758927460787));
#53982=CARTESIAN_POINT('Ctrl Pts',(21.2316699285407,18.908003235373,40.1171711945268));
#53983=CARTESIAN_POINT('Ctrl Pts',(21.163998799875,18.9037764307596,40.1584906890913));
#53984=CARTESIAN_POINT('Ctrl Pts',(21.0942728414268,18.8995496261463,40.1963848877761));
#53985=CARTESIAN_POINT('Ctrl Pts',(21.0228767613701,18.895322821533,40.2306603605336));
#53986=CARTESIAN_POINT('Ctrl Pts',(20.9514460840272,18.8910939686844,40.264952442583));
#53987=CARTESIAN_POINT('Ctrl Pts',(20.8783441056562,18.8868651158357,40.295622123797));
#53988=CARTESIAN_POINT('Ctrl Pts',(20.8039753446254,18.8826362629871,40.3225242599654));
#53989=CARTESIAN_POINT('Ctrl Pts',(20.729472926633,18.8783998099632,40.3494747451681));
#53990=CARTESIAN_POINT('Ctrl Pts',(20.6536996262899,18.8741633569393,40.3726440186046));
#53991=CARTESIAN_POINT('Ctrl Pts',(20.5770747172652,18.8699269039153,40.391936999918));
#53992=CARTESIAN_POINT('Ctrl Pts',(20.5074324440273,18.8660765082306,40.4094718602305));
#53993=CARTESIAN_POINT('Ctrl Pts',(20.4370871063224,18.8622261125459,40.4238053109777));
#53994=CARTESIAN_POINT('Ctrl Pts',(20.3663576230851,18.8583757168611,40.4349031099614));
#53995=CARTESIAN_POINT('Ctrl Pts',(20.2885146476296,18.8541380744656,40.4471170503772));
#53996=CARTESIAN_POINT('Ctrl Pts',(20.20991408771,18.8499004320701,40.4554568677485));
#53997=CARTESIAN_POINT('Ctrl Pts',(20.130975226485,18.8456627896745,40.4598381154111));
#53998=CARTESIAN_POINT('Ctrl Pts',(20.0521498824351,18.8414312411748,40.464213062668));
#53999=CARTESIAN_POINT('Ctrl Pts',(19.9729876673909,18.837199692675,40.4646407193865));
#54000=CARTESIAN_POINT('Ctrl Pts',(19.8939159576045,18.8329681441752,40.4610880154812));
#54001=CARTESIAN_POINT('Ctrl Pts',(19.8149355778206,18.8287414832305,40.4575394150468));
#54002=CARTESIAN_POINT('Ctrl Pts',(19.7360459614858,18.8245148222859,40.4500196111653));
#54003=CARTESIAN_POINT('Ctrl Pts',(19.6576759516972,18.8202881613412,40.4385475592456));
#54004=CARTESIAN_POINT('Ctrl Pts',(19.5793554114975,18.8160641683964,40.4270827488421));
#54005=CARTESIAN_POINT('Ctrl Pts',(19.5015542894333,18.8118401754516,40.4116707099863));
#54006=CARTESIAN_POINT('Ctrl Pts',(19.4246965493785,18.8076161825068,40.3923822501064));
#54007=CARTESIAN_POINT('Ctrl Pts',(19.3478633940053,18.8033935407014,40.3730999600755));
#54008=CARTESIAN_POINT('Ctrl Pts',(19.2719734757476,18.7991708988961,40.3499438253615));
#54009=CARTESIAN_POINT('Ctrl Pts',(19.1974393343323,18.7949482570907,40.3230354965279));
#54010=CARTESIAN_POINT('Ctrl Pts',(19.1229058280705,18.7907256512692,40.2961273969976));
#54011=CARTESIAN_POINT('Ctrl Pts',(19.0497285161126,18.7865030454477,40.2654673274486));
#54012=CARTESIAN_POINT('Ctrl Pts',(18.9783021555091,18.7822804396262,40.2312259278318));
#54013=CARTESIAN_POINT('Ctrl Pts',(18.9068047705569,18.7780536349651,40.1969504795378));
#54014=CARTESIAN_POINT('Ctrl Pts',(18.8370622384995,18.773826830304,40.1590867908324));
#54015=CARTESIAN_POINT('Ctrl Pts',(18.7694462318672,18.769600025643,40.1178522900932));
#54016=CARTESIAN_POINT('Ctrl Pts',(18.7017974597021,18.7653711727464,40.0765978078369));
#54017=CARTESIAN_POINT('Ctrl Pts',(18.6362776537237,18.7611423198498,40.0319695237864));
#54018=CARTESIAN_POINT('Ctrl Pts',(18.5732287644304,18.7569134669532,39.9842277681457));
#54019=CARTESIAN_POINT('Ctrl Pts',(18.510066562469,18.7526770138814,39.9364002101098));
#54020=CARTESIAN_POINT('Ctrl Pts',(18.4493845101543,18.7484405608096,39.8854483021046));
#54021=CARTESIAN_POINT('Ctrl Pts',(18.3914905928753,18.7442041077378,39.8316720036114));
#54022=CARTESIAN_POINT('Ctrl Pts',(18.3388724094092,18.7403537124725,39.7827962102079));
#54023=CARTESIAN_POINT('Ctrl Pts',(18.2885570812017,18.7365033172073,39.7315879983667));
#54024=CARTESIAN_POINT('Ctrl Pts',(18.2407469317621,18.7326529219421,39.6782962595139));
#54025=CARTESIAN_POINT('Ctrl Pts',(18.1886714455363,18.7284590173434,39.6202501491145));
#54026=CARTESIAN_POINT('Ctrl Pts',(18.1393638736236,18.7242651127447,39.5595033357046));
#54027=CARTESIAN_POINT('Ctrl Pts',(18.0931208954266,18.720071208146,39.4963532939201));
#54028=CARTESIAN_POINT('Ctrl Pts',(18.0469392292103,18.7158828641017,39.4332869806126));
#54029=CARTESIAN_POINT('Ctrl Pts',(18.0038143777873,18.7116945200574,39.3678241414009));
#54030=CARTESIAN_POINT('Ctrl Pts',(17.9640048148198,18.7075061760132,39.3002974826363));
#54031=CARTESIAN_POINT('Ctrl Pts',(17.9242350131353,18.7033220152335,39.232838268636));
#54032=CARTESIAN_POINT('Ctrl Pts',(17.8877741716712,18.6991378544537,39.1633197354723));
#54033=CARTESIAN_POINT('Ctrl Pts',(17.8548382602009,18.694953693674,39.0921046068849));
#54034=CARTESIAN_POINT('Ctrl Pts',(17.8219244767009,18.6907723440199,39.0209373241344));
#54035=CARTESIAN_POINT('Ctrl Pts',(17.7925311220298,18.6865909943659,38.9480761426687));
#54036=CARTESIAN_POINT('Ctrl Pts',(17.7668280953728,18.6824096447118,38.8739080599681));
#54037=CARTESIAN_POINT('Ctrl Pts',(17.7411275740086,18.6782287026169,38.7997472064849));
#54038=CARTESIAN_POINT('Ctrl Pts',(17.7191168349262,18.674047760522,38.7242801531567));
#54039=CARTESIAN_POINT('Ctrl Pts',(17.700917020489,18.6698668184272,38.6479123052303));
#54040=CARTESIAN_POINT('Ctrl Pts',(17.6827181465883,18.6656860923965,38.5715484038688));
#54041=CARTESIAN_POINT('Ctrl Pts',(17.6683299089655,18.6615053663659,38.494284268536));
#54042=CARTESIAN_POINT('Ctrl Pts',(17.6578226295373,18.6573246403352,38.4165368954679));
#54043=CARTESIAN_POINT('Ctrl Pts',(17.647308431712,18.6531411615537,38.338738330537));
#54044=CARTESIAN_POINT('Ctrl Pts',(17.6406803453056,18.6489576827721,38.2604563692487));
#54045=CARTESIAN_POINT('Ctrl Pts',(17.6379568524747,18.6447742039905,38.1821133979853));
#54046=CARTESIAN_POINT('Ctrl Pts',(17.6369809093477,18.6432750859031,38.1540397847621));
#54047=CARTESIAN_POINT('Ctrl Pts',(17.6365058655876,18.6417759678157,38.125958345013));
#54048=CARTESIAN_POINT('Ctrl Pts',(17.6365309432179,18.6402768497283,38.0978884759611));
#54049=CARTESIAN_POINT('',(17.6365300981239,17.8465268496895,38.1006810474926));
#54050=CARTESIAN_POINT('Ctrl Pts',(17.6365309432187,18.6402768496835,38.0978884751228));
#54051=CARTESIAN_POINT('Ctrl Pts',(17.6366239153381,18.6347190625734,37.9938230531207));
#54052=CARTESIAN_POINT('Ctrl Pts',(17.6435944777715,18.6291612754634,37.8900613092647));
#54053=CARTESIAN_POINT('Ctrl Pts',(17.6572963530161,18.6236034883533,37.7873819210152));
#54054=CARTESIAN_POINT('Ctrl Pts',(17.6709982282606,18.6180457012432,37.6847025327657));
#54055=CARTESIAN_POINT('Ctrl Pts',(17.6914312182393,18.6124879141331,37.5831051765486));
#54056=CARTESIAN_POINT('Ctrl Pts',(17.7183944712534,18.606930127023,37.4833423542249));
#54057=CARTESIAN_POINT('Ctrl Pts',(17.7389531254918,18.6026924846485,37.4072762590498));
#54058=CARTESIAN_POINT('Ctrl Pts',(17.7633584640601,18.598454842274,37.3320966078432));
#54059=CARTESIAN_POINT('Ctrl Pts',(17.7915167929748,18.5942171998995,37.2582207146837));
#54060=CARTESIAN_POINT('Ctrl Pts',(17.819634629107,18.5899856514211,37.1844510579588));
#54061=CARTESIAN_POINT('Ctrl Pts',(17.8514945721677,18.5857541029427,37.1119818704062));
#54062=CARTESIAN_POINT('Ctrl Pts',(17.8869527113608,18.5815225544643,37.0412169264318));
#54063=CARTESIAN_POINT('Ctrl Pts',(17.9223698954232,18.5772958935414,36.9705337179233));
#54064=CARTESIAN_POINT('Ctrl Pts',(17.9613768076314,18.5730692326184,36.9015512581737));
#54065=CARTESIAN_POINT('Ctrl Pts',(18.003781427272,18.5688425716955,36.8346534661225));
#54066=CARTESIAN_POINT('Ctrl Pts',(18.0461592797947,18.5646185787726,36.7677979020432));
#54067=CARTESIAN_POINT('Ctrl Pts',(18.0919303323664,18.5603945858498,36.7030247886281));
#54068=CARTESIAN_POINT('Ctrl Pts',(18.1408571981563,18.556170592927,36.6406924644706));
#54069=CARTESIAN_POINT('Ctrl Pts',(18.1897684135824,18.5519479511438,36.5783800787158));
#54070=CARTESIAN_POINT('Ctrl Pts',(18.2418331484101,18.5477253093606,36.5185073002988));
#54071=CARTESIAN_POINT('Ctrl Pts',(18.2967722374415,18.5435026675774,36.4614013213267));
#54072=CARTESIAN_POINT('Ctrl Pts',(18.3517108582994,18.5392800617782,36.4042958289937));
#54073=CARTESIAN_POINT('Ctrl Pts',(18.4095234586276,18.535057455979,36.3499574260545));
#54074=CARTESIAN_POINT('Ctrl Pts',(18.4698933782484,18.5308348501798,36.2986771064099));
#54075=CARTESIAN_POINT('Ctrl Pts',(18.5303233280054,18.5266080455411,36.2473457950696));
#54076=CARTESIAN_POINT('Ctrl Pts',(18.5933153184537,18.5223812409024,36.1990789453668));
#54077=CARTESIAN_POINT('Ctrl Pts',(18.6585193644235,18.5181544362638,36.1541274077491));
#54078=CARTESIAN_POINT('Ctrl Pts',(18.7237550071312,18.5139255833897,36.1091540874042));
#54079=CARTESIAN_POINT('Ctrl Pts',(18.7912044414011,18.5096967305156,36.0674995261933));
#54080=CARTESIAN_POINT('Ctrl Pts',(18.8604906106194,18.5054678776415,36.0293699527889));
#54081=CARTESIAN_POINT('Ctrl Pts',(18.9299013022672,18.501231424592,35.9911718521854));
#54082=CARTESIAN_POINT('Ctrl Pts',(19.0011549020658,18.4969949715426,35.9565116032249));
#54083=CARTESIAN_POINT('Ctrl Pts',(19.0738519992355,18.4927585184932,35.9255482710394));
#54084=CARTESIAN_POINT('Ctrl Pts',(19.1399243880608,18.4889081230301,35.8974065514503));
#54085=CARTESIAN_POINT('Ctrl Pts',(19.2071886823368,18.485057727567,35.8723181385503));
#54086=CARTESIAN_POINT('Ctrl Pts',(19.2753351555784,18.481207332104,35.8503664066877));
#54087=CARTESIAN_POINT('Ctrl Pts',(19.3503353434361,18.4769696897239,35.8262069170592));
#54088=CARTESIAN_POINT('Ctrl Pts',(19.4266858091362,18.4727320473439,35.8057568091963));
#54089=CARTESIAN_POINT('Ctrl Pts',(19.5039854804583,18.4684944049639,35.7891646451329));
#54090=CARTESIAN_POINT('Ctrl Pts',(19.5811739918204,18.4642628564798,35.7725963412523));
#54091=CARTESIAN_POINT('Ctrl Pts',(19.659308543504,18.4600313079958,35.7598750611734));
#54092=CARTESIAN_POINT('Ctrl Pts',(19.7379720864863,18.4557997595117,35.7510998715485));
#54093=CARTESIAN_POINT('Ctrl Pts',(19.8165447709051,18.451573098583,35.7423348175098));
#54094=CARTESIAN_POINT('Ctrl Pts',(19.8956447688872,18.4473464376543,35.7375068480514));
#54095=CARTESIAN_POINT('Ctrl Pts',(19.9748454995802,18.4431197767256,35.7366638639397));
#54096=CARTESIAN_POINT('Ctrl Pts',(20.0539962363043,18.4388957837969,35.7358214119457));
#54097=CARTESIAN_POINT('Ctrl Pts',(20.1332471120084,18.4346717908682,35.7389589573902));
#54098=CARTESIAN_POINT('Ctrl Pts',(20.2121683099733,18.4304477979396,35.7460724205824));
#54099=CARTESIAN_POINT('Ctrl Pts',(20.2910642632106,18.4262251561504,35.7531836083727));
#54100=CARTESIAN_POINT('Ctrl Pts',(20.3696302815773,18.4220025143613,35.7642681463416));
#54101=CARTESIAN_POINT('Ctrl Pts',(20.4474399346824,18.4177798725722,35.7792699541413));
#54102=CARTESIAN_POINT('Ctrl Pts',(20.5252489247195,18.413557266767,35.7942716341006));
#54103=CARTESIAN_POINT('Ctrl Pts',(20.6023011022857,18.4093346609618,35.8131904273686));
#54104=CARTESIAN_POINT('Ctrl Pts',(20.6781799926426,18.4051120551566,35.8359190963044));
#54105=CARTESIAN_POINT('Ctrl Pts',(20.7541343348171,18.4008852505119,35.8586703659843));
#54106=CARTESIAN_POINT('Ctrl Pts',(20.8289126092223,18.3966584458673,35.8852389439191));
#54107=CARTESIAN_POINT('Ctrl Pts',(20.9021138761845,18.3924316412226,35.9154677857044));
#54108=CARTESIAN_POINT('Ctrl Pts',(20.9753506151981,18.3882027883424,35.9457112758568));
#54109=CARTESIAN_POINT('Ctrl Pts',(21.0470084001397,18.3839739354622,35.9796183625193));
#54110=CARTESIAN_POINT('Ctrl Pts',(21.1167089871477,18.3797450825821,36.0169850027128));
#54111=CARTESIAN_POINT('Ctrl Pts',(21.1865348413843,18.3755086295266,36.054418798947));
#54112=CARTESIAN_POINT('Ctrl Pts',(21.2543960669251,18.3712721764711,36.0953243294549));
#54113=CARTESIAN_POINT('Ctrl Pts',(21.3199418157071,18.3670357234157,36.1394531262814));
#54114=CARTESIAN_POINT('Ctrl Pts',(21.3795145400991,18.3631853280054,36.1795605733691));
#54115=CARTESIAN_POINT('Ctrl Pts',(21.4371747410107,18.3593349325951,36.2223298945484));
#54116=CARTESIAN_POINT('Ctrl Pts',(21.4926838832828,18.3554845371848,36.2675466539396));
#54117=CARTESIAN_POINT('Ctrl Pts',(21.5537757630851,18.3512468948079,36.3173110119662));
#54118=CARTESIAN_POINT('Ctrl Pts',(21.6124909669647,18.3470092524311,36.3702272225976));
#54119=CARTESIAN_POINT('Ctrl Pts',(21.6684865531871,18.3427716100542,36.4260397069423));
#54120=CARTESIAN_POINT('Ctrl Pts',(21.7244016155589,18.3385400615734,36.4817719307441));
#54121=CARTESIAN_POINT('Ctrl Pts',(21.7776044977201,18.3343085130925,36.5403918288483));
#54122=CARTESIAN_POINT('Ctrl Pts',(21.827785081266,18.3300769646117,36.6016034778466));
#54123=CARTESIAN_POINT('Ctrl Pts',(21.8779077048521,18.3258503036862,36.6627444257));
#54124=CARTESIAN_POINT('Ctrl Pts',(21.9250146713074,18.3216236427608,36.7264708148327));
#54125=CARTESIAN_POINT('Ctrl Pts',(21.9688335951169,18.3173969818353,36.7924508744835));
#54126=CARTESIAN_POINT('Ctrl Pts',(22.0126248590562,18.3131729889099,36.8583892854646));
#54127=CARTESIAN_POINT('Ctrl Pts',(22.0531319413554,18.3089489959845,36.9265781538065));
#54128=CARTESIAN_POINT('Ctrl Pts',(22.0901242998228,18.3047250030591,36.9966546994752));
#54129=CARTESIAN_POINT('Ctrl Pts',(22.1271048254487,18.3005023612733,37.0667088295776));
#54130=CARTESIAN_POINT('Ctrl Pts',(22.1605726411276,18.2962797194875,37.1386490236881));
#54131=CARTESIAN_POINT('Ctrl Pts',(22.1903426696324,18.2920570777017,37.2120870366484));
#54132=CARTESIAN_POINT('Ctrl Pts',(22.2201124444467,18.2878344718998,37.2855244237939));
#54133=CARTESIAN_POINT('Ctrl Pts',(22.2461843199563,18.283611866098,37.360459169439));
#54134=CARTESIAN_POINT('Ctrl Pts',(22.2684215523446,18.2793892602961,37.4364835331671));
#54135=CARTESIAN_POINT('Ctrl Pts',(22.2906808968064,18.2751624556548,37.5125834933672));
#54136=CARTESIAN_POINT('Ctrl Pts',(22.3090978496328,18.2709356510134,37.5897747849498));
#54137=CARTESIAN_POINT('Ctrl Pts',(22.3235859045743,18.266708846372,37.6676355877691));
#54138=CARTESIAN_POINT('Ctrl Pts',(22.3380809801734,18.2624799934952,37.7455341205693));
#54139=CARTESIAN_POINT('Ctrl Pts',(22.3486433026082,18.2582511406184,37.8241023457273));
#54140=CARTESIAN_POINT('Ctrl Pts',(22.3552381453472,18.2540222877416,37.9029118988845));
#54141=CARTESIAN_POINT('Ctrl Pts',(22.3618448404639,18.2497858346894,37.9818630900791));
#54142=CARTESIAN_POINT('Ctrl Pts',(22.3644697930266,18.2455493816372,38.0610560062585));
#54143=CARTESIAN_POINT('Ctrl Pts',(22.3631304556828,18.2413129285851,38.1400610824187));
#54144=CARTESIAN_POINT('Ctrl Pts',(22.3619131688777,18.2374625331453,38.2118666190837));
#54145=CARTESIAN_POINT('Ctrl Pts',(22.3574218676397,18.2336121377055,38.2835167544354));
#54146=CARTESIAN_POINT('Ctrl Pts',(22.349706592117,18.2297617422657,38.3546946639842));
#54147=CARTESIAN_POINT('Ctrl Pts',(22.3412153659513,18.2255240998886,38.4330311700753));
#54148=CARTESIAN_POINT('Ctrl Pts',(22.3287864436435,18.2212864575114,38.5110896251283));
#54149=CARTESIAN_POINT('Ctrl Pts',(22.3124475466707,18.2170488151343,38.5884432257658));
#54150=CARTESIAN_POINT('Ctrl Pts',(22.296132145673,18.2128172666532,38.6656855888899));
#54151=CARTESIAN_POINT('Ctrl Pts',(22.2759180322438,18.208585718172,38.7422246556667));
#54152=CARTESIAN_POINT('Ctrl Pts',(22.2518846384725,18.2043541696909,38.8176391961925));
#54153=CARTESIAN_POINT('Ctrl Pts',(22.2278790039346,18.2001275087652,38.8929666308411));
#54154=CARTESIAN_POINT('Ctrl Pts',(22.200062997182,18.1959008478394,38.9671716760173));
#54155=CARTESIAN_POINT('Ctrl Pts',(22.1685666608388,18.1916741869137,39.0398452417278));
#54156=CARTESIAN_POINT('Ctrl Pts',(22.1370902059647,18.187450193988,39.1124729336189));
#54157=CARTESIAN_POINT('Ctrl Pts',(22.1019382185961,18.1832262010624,39.183570635881));
#54158=CARTESIAN_POINT('Ctrl Pts',(22.0632895308391,18.1790022081367,39.2527474800795));
#54159=CARTESIAN_POINT('Ctrl Pts',(22.0246532057381,18.1747795663506,39.3219021965016));
#54160=CARTESIAN_POINT('Ctrl Pts',(21.9825226298382,18.1705569245645,39.3891368660561));
#54161=CARTESIAN_POINT('Ctrl Pts',(21.9371227453085,18.1663342827784,39.4540848978215));
#54162=CARTESIAN_POINT('Ctrl Pts',(21.8917232476619,18.1621116769763,39.519032376121));
#54163=CARTESIAN_POINT('Ctrl Pts',(21.8430547665216,18.1578890711742,39.5816928719838));
#54164=CARTESIAN_POINT('Ctrl Pts',(21.7913849075893,18.1536664653721,39.6417297278581));
#54165=CARTESIAN_POINT('Ctrl Pts',(21.7396636696142,18.1494396607305,39.7018262826798));
#54166=CARTESIAN_POINT('Ctrl Pts',(21.6849353988243,18.1452128560889,39.7592936301455));
#54167=CARTESIAN_POINT('Ctrl Pts',(21.6275068580425,18.1409860514472,39.8138295912735));
#54168=CARTESIAN_POINT('Ctrl Pts',(21.5700504883961,18.1367571985702,39.8683919795727));
#54169=CARTESIAN_POINT('Ctrl Pts',(21.5098915982557,18.1325283456931,39.9200198460559));
#54170=CARTESIAN_POINT('Ctrl Pts',(21.4473706257125,18.128299492816,39.9684508858208));
#54171=CARTESIAN_POINT('Ctrl Pts',(21.3847372892809,18.1240630397636,40.0169689667773));
#54172=CARTESIAN_POINT('Ctrl Pts',(21.3197337736478,18.1198265867112,40.0622784724595));
#54173=CARTESIAN_POINT('Ctrl Pts',(21.2527299270681,18.1155901336588,40.1041602158331));
#54174=CARTESIAN_POINT('Ctrl Pts',(21.1918319773058,18.1117397382215,40.1422253782695));
#54175=CARTESIAN_POINT('Ctrl Pts',(21.1292822262864,18.1078893427841,40.1774594856631));
#54176=CARTESIAN_POINT('Ctrl Pts',(21.0653736864354,18.1040389473468,40.2097320562458));
#54177=CARTESIAN_POINT('Ctrl Pts',(20.9950376544135,18.0998013049689,40.2452503854585));
#54178=CARTESIAN_POINT('Ctrl Pts',(20.9227914424757,18.0955636625911,40.2773141559457));
#54179=CARTESIAN_POINT('Ctrl Pts',(20.8490081719268,18.0913260202132,40.3057142981133));
#54180=CARTESIAN_POINT('Ctrl Pts',(20.7753310046163,18.0870944717314,40.334073599762));
#54181=CARTESIAN_POINT('Ctrl Pts',(20.7001216021157,18.0828629232496,40.3587795687255));
#54182=CARTESIAN_POINT('Ctrl Pts',(20.6237765582469,18.0786313747678,40.3796695476059));
#54183=CARTESIAN_POINT('Ctrl Pts',(20.5475196950119,18.0744047138413,40.4005353979838));
#54184=CARTESIAN_POINT('Ctrl Pts',(20.4701302469447,18.0701780529149,40.4175938941423));
#54185=CARTESIAN_POINT('Ctrl Pts',(20.3920221732022,18.0659513919884,40.4307314424056));
#54186=CARTESIAN_POINT('Ctrl Pts',(20.3139634037098,18.061727399062,40.4438606978389));
#54187=CARTESIAN_POINT('Ctrl Pts',(20.2351873699961,18.0575034061356,40.4530738404765));
#54188=CARTESIAN_POINT('Ctrl Pts',(20.1561193035916,18.0532794132093,40.4583081231989));
#54189=CARTESIAN_POINT('Ctrl Pts',(20.0770765288943,18.0490567714224,40.4635407316178));
#54190=CARTESIAN_POINT('Ctrl Pts',(19.9977423744188,18.0448341296356,40.4647969765657));
#54191=CARTESIAN_POINT('Ctrl Pts',(19.9185468054221,18.0406114878488,40.4620660062736));
#54192=CARTESIAN_POINT('Ctrl Pts',(19.8393519113042,18.0363888820459,40.4593350592539));
#54193=CARTESIAN_POINT('Ctrl Pts',(19.760296068762,18.0321662762431,40.4526169821363));
#54194=CARTESIAN_POINT('Ctrl Pts',(19.6818073561958,18.0279436704402,40.4419530060035));
#54195=CARTESIAN_POINT('Ctrl Pts',(19.603240596679,18.0237168657979,40.4312784259152));
#54196=CARTESIAN_POINT('Ctrl Pts',(19.5252425591924,18.0194900611555,40.4166501724801));
#54197=CARTESIAN_POINT('Ctrl Pts',(19.4482337137936,18.0152632565132,40.3981610923314));
#54198=CARTESIAN_POINT('Ctrl Pts',(19.3711875512577,18.0110344036353,40.3796630526985));
#54199=CARTESIAN_POINT('Ctrl Pts',(19.2951319860325,18.0068055507575,40.3573005917263));
#54200=CARTESIAN_POINT('Ctrl Pts',(19.2204723697479,18.0025766978797,40.3312165100173));
#54201=CARTESIAN_POINT('Ctrl Pts',(19.145678573772,17.9983402448265,40.3050855494973));
#54202=CARTESIAN_POINT('Ctrl Pts',(19.0722861748444,17.9941037917734,40.2752197809421));
#54203=CARTESIAN_POINT('Ctrl Pts',(19.0006803634098,17.9898673387202,40.2418101467743));
#54204=CARTESIAN_POINT('Ctrl Pts',(18.9355998147263,17.9860169432894,40.2114450509896));
#54205=CARTESIAN_POINT('Ctrl Pts',(18.8719950122391,17.9821665478585,40.1781532688296));
#54206=CARTESIAN_POINT('Ctrl Pts',(18.8101349099469,17.9783161524276,40.1421095730575));
#54207=CARTESIAN_POINT('Ctrl Pts',(18.7420533334829,17.9740785100502,40.1024408441219));
#54208=CARTESIAN_POINT('Ctrl Pts',(18.6758298955651,17.9698408676728,40.0592892881113));
#54209=CARTESIAN_POINT('Ctrl Pts',(18.6118430810831,17.9656032252954,40.0128541003859));
#54210=CARTESIAN_POINT('Ctrl Pts',(18.5479482821514,17.9613716768141,39.9664856882828));
#54211=CARTESIAN_POINT('Ctrl Pts',(18.4862840955409,17.9571401283328,39.9168432949561));
#54212=CARTESIAN_POINT('Ctrl Pts',(18.4272028493791,17.9529085798514,39.8641710699075));
#54213=CARTESIAN_POINT('Ctrl Pts',(18.3681898436882,17.9486819189254,39.8115596827334));
#54214=CARTESIAN_POINT('Ctrl Pts',(18.3117541978809,17.9444552579994,39.7559257286738));
#54215=CARTESIAN_POINT('Ctrl Pts',(18.2582165346876,17.9402285970734,39.6975546315742));
#54216=CARTESIAN_POINT('Ctrl Pts',(18.2047126661356,17.9360046041475,39.63922038013));
#54217=CARTESIAN_POINT('Ctrl Pts',(18.1541034652771,17.9317806112216,39.578152759642));
#54218=CARTESIAN_POINT('Ctrl Pts',(18.1066730372676,17.9275566182957,39.5146743275717));
#54219=CARTESIAN_POINT('Ctrl Pts',(18.0592577809519,17.9233339765093,39.4512162005118));
#54220=CARTESIAN_POINT('Ctrl Pts',(18.0150195587025,17.919111334723,39.3853491684802));
#54221=CARTESIAN_POINT('Ctrl Pts',(17.9742015190833,17.9148886929366,39.3174280083913));
#54222=CARTESIAN_POINT('Ctrl Pts',(17.9333838273021,17.9106660871342,39.2495074271044));
#54223=CARTESIAN_POINT('Ctrl Pts',(17.895986500441,17.9064434813319,39.1795331550997));
#54224=CARTESIAN_POINT('Ctrl Pts',(17.8622079693646,17.9022208755295,39.1078867370154));
#54225=CARTESIAN_POINT('Ctrl Pts',(17.8283958498744,17.8979940708876,39.0361690757642));
#54226=CARTESIAN_POINT('Ctrl Pts',(17.7982099144151,17.8937672662457,38.9627763721112));
#54227=CARTESIAN_POINT('Ctrl Pts',(17.7718011537476,17.8895404616039,38.8881118844807));
#54228=CARTESIAN_POINT('Ctrl Pts',(17.7453795958575,17.8853116087265,38.8134112157477));
#54229=CARTESIAN_POINT('Ctrl Pts',(17.7227389930867,17.8810827558492,38.7374379851508));
#54230=CARTESIAN_POINT('Ctrl Pts',(17.703980201933,17.8768539029718,38.6606099604754));
#54231=CARTESIAN_POINT('Ctrl Pts',(17.6851876971208,17.8726174499192,38.5836438590035));
#54232=CARTESIAN_POINT('Ctrl Pts',(17.6702910319215,17.8683809968665,38.505820355379));
#54233=CARTESIAN_POINT('Ctrl Pts',(17.6593397037708,17.8641445438138,38.4275665101261));
#54234=CARTESIAN_POINT('Ctrl Pts',(17.6493863434018,17.8602941483787,38.3564437466272));
#54235=CARTESIAN_POINT('Ctrl Pts',(17.642691386469,17.8564437529437,38.284965839398));
#54236=CARTESIAN_POINT('Ctrl Pts',(17.6392546229838,17.8525933575086,38.2134535402565));
#54237=CARTESIAN_POINT('Ctrl Pts',(17.6374496869478,17.8505711882485,38.1758963658105));
#54238=CARTESIAN_POINT('Ctrl Pts',(17.6365409370372,17.8485490189884,38.138295778481));
#54239=CARTESIAN_POINT('Ctrl Pts',(17.6365300981241,17.8465268497283,38.1006810482146));
#54240=CARTESIAN_POINT('',(17.6365305274028,17.0527768497571,38.101578924073));
#54241=CARTESIAN_POINT('Ctrl Pts',(17.6365300981239,17.8465268496895,38.1006810474926));
#54242=CARTESIAN_POINT('Ctrl Pts',(17.6365075550966,17.8423210898796,38.0224489608224));
#54243=CARTESIAN_POINT('Ctrl Pts',(17.6403735597462,17.8381153300697,37.9440613389769));
#54244=CARTESIAN_POINT('Ctrl Pts',(17.6481482955731,17.8339095702598,37.8659401758429));
#54245=CARTESIAN_POINT('Ctrl Pts',(17.6559120990009,17.8297097243544,37.7879288623243));
#54246=CARTESIAN_POINT('Ctrl Pts',(17.6675736759225,17.8255098784489,37.7101837339056));
#54247=CARTESIAN_POINT('Ctrl Pts',(17.6831011931123,17.8213100325435,37.6331270413244));
#54248=CARTESIAN_POINT('Ctrl Pts',(17.6986118056779,17.8171147589607,37.556154239453));
#54249=CARTESIAN_POINT('Ctrl Pts',(17.7179799045057,17.8129194853778,37.4798688494731));
#54250=CARTESIAN_POINT('Ctrl Pts',(17.7411220056558,17.808724211795,37.4046866551204));
#54251=CARTESIAN_POINT('Ctrl Pts',(17.7642507353119,17.804531362239,37.3295479010006));
#54252=CARTESIAN_POINT('Ctrl Pts',(17.7911490007325,17.800338512683,37.2555115321422));
#54253=CARTESIAN_POINT('Ctrl Pts',(17.8216828405759,17.7961456631271,37.182980483382));
#54254=CARTESIAN_POINT('Ctrl Pts',(17.8522089048497,17.7919538812977,37.1104679049554));
#54255=CARTESIAN_POINT('Ctrl Pts',(17.8863685204665,17.7877620994684,37.0394603244555));
#54256=CARTESIAN_POINT('Ctrl Pts',(17.9239793027399,17.7835703176391,36.9703414208498));
#54257=CARTESIAN_POINT('Ctrl Pts',(17.9615926609566,17.7793782487167,36.9012177833255));
#54258=CARTESIAN_POINT('Ctrl Pts',(18.0026574252911,17.7751861797943,36.8339834969267));
#54259=CARTESIAN_POINT('Ctrl Pts',(18.0469456729691,17.770994110872,36.7689969058767));
#54260=CARTESIAN_POINT('Ctrl Pts',(18.0912795208766,17.7667977256961,36.7039434030922));
#54261=CARTESIAN_POINT('Ctrl Pts',(18.1388432071584,17.7626013405202,36.6411426088292));
#54262=CARTESIAN_POINT('Ctrl Pts',(18.1893664066169,17.7584049553443,36.5809225064492));
#54263=CARTESIAN_POINT('Ctrl Pts',(18.2399186658585,17.7542061565042,36.5206677668504));
#54264=CARTESIAN_POINT('Ctrl Pts',(18.2934335010051,17.750007357664,36.4629970215123));
#54265=CARTESIAN_POINT('Ctrl Pts',(18.349603130203,17.7458085588238,36.408201958547));
#54266=CARTESIAN_POINT('Ctrl Pts',(18.405866185116,17.7416027762134,36.3533157561526));
#54267=CARTESIAN_POINT('Ctrl Pts',(18.4647924894867,17.737396993603,36.3013150964894));
#54268=CARTESIAN_POINT('Ctrl Pts',(18.5260410722742,17.7331912109926,36.2524514836472));
#54269=CARTESIAN_POINT('Ctrl Pts',(18.556723491604,17.7310843281915,36.2279733032394));
#54270=CARTESIAN_POINT('Ctrl Pts',(18.5879882269045,17.7289774453905,36.2042816852787));
#54271=CARTESIAN_POINT('Ctrl Pts',(18.6197899146442,17.7268705625894,36.1814040130392));
#54272=CARTESIAN_POINT('Ctrl Pts',(18.6837536906915,17.7226329202119,36.1353894016265));
#54273=CARTESIAN_POINT('Ctrl Pts',(18.7501411602903,17.7183952778343,36.0924906324536));
#54274=CARTESIAN_POINT('Ctrl Pts',(18.8186162142466,17.7141576354568,36.0529722054503));
#54275=CARTESIAN_POINT('Ctrl Pts',(18.8869927983881,17.7099260869753,36.013510607496));
#54276=CARTESIAN_POINT('Ctrl Pts',(18.9574506024816,17.7056945384938,35.9774199304681));
#54277=CARTESIAN_POINT('Ctrl Pts',(19.0296231191284,17.7014629900123,35.9449224723992));
#54278=CARTESIAN_POINT('Ctrl Pts',(19.1017122745253,17.6972363290861,35.9124625497919));
#54279=CARTESIAN_POINT('Ctrl Pts',(19.1755117813665,17.6930096681599,35.8835877900102));
#54280=CARTESIAN_POINT('Ctrl Pts',(19.2506303551274,17.6887830072338,35.858474721034));
#54281=CARTESIAN_POINT('Ctrl Pts',(19.3257015117036,17.6845590143077,35.8333775042096));
#54282=CARTESIAN_POINT('Ctrl Pts',(19.4020896390851,17.6803350213816,35.8120374133194));
#54283=CARTESIAN_POINT('Ctrl Pts',(19.4793844176147,17.6761110284556,35.794582498488));
#54284=CARTESIAN_POINT('Ctrl Pts',(19.5566544716635,17.6718883866691,35.7771331670055));
#54285=CARTESIAN_POINT('Ctrl Pts',(19.6348301440226,17.6676657448825,35.7635666468885));
#54286=CARTESIAN_POINT('Ctrl Pts',(19.7134883762113,17.663443103096,35.7539604584888));
#54287=CARTESIAN_POINT('Ctrl Pts',(19.7921459381002,17.6592204972935,35.74435435195));
#54288=CARTESIAN_POINT('Ctrl Pts',(19.8712855861536,17.6549978914909,35.738708565434));
#54289=CARTESIAN_POINT('Ctrl Pts',(19.9504780341298,17.6507752856884,35.7370488757073));
#54290=CARTESIAN_POINT('Ctrl Pts',(20.029749228831,17.6465484810464,35.7353875356321));
#54291=CARTESIAN_POINT('Ctrl Pts',(20.1090728585694,17.6423216764043,35.7377202196232));
#54292=CARTESIAN_POINT('Ctrl Pts',(20.1880191339567,17.6380948717623,35.7440205335856));
#54293=CARTESIAN_POINT('Ctrl Pts',(20.2670036653259,17.6338660188848,35.7503239005698));
#54294=CARTESIAN_POINT('Ctrl Pts',(20.3456100126528,17.6296371660073,35.7605986668219));
#54295=CARTESIAN_POINT('Ctrl Pts',(20.4234155604438,17.6254083131298,35.7747667420076));
#54296=CARTESIAN_POINT('Ctrl Pts',(20.5013609418544,17.6211718600769,35.7889602803292));
#54297=CARTESIAN_POINT('Ctrl Pts',(20.5785021905825,17.6169354070241,35.8070610011872));
#54298=CARTESIAN_POINT('Ctrl Pts',(20.6544291280943,17.6126989539713,35.8289401246991));
#54299=CARTESIAN_POINT('Ctrl Pts',(20.7234370292418,17.6088485585376,35.848825457125));
#54300=CARTESIAN_POINT('Ctrl Pts',(20.7914417997745,17.604998163104,35.8718312140375));
#54301=CARTESIAN_POINT('Ctrl Pts',(20.8581505983656,17.6011477676704,35.8978265301242));
#54302=CARTESIAN_POINT('Ctrl Pts',(20.9315685204291,17.5969101252929,35.9264362807235));
#54303=CARTESIAN_POINT('Ctrl Pts',(21.0036919659445,17.5926724829154,35.9587752529252));
#54304=CARTESIAN_POINT('Ctrl Pts',(21.0741160983171,17.5884348405379,35.9947054723303));
#54305=CARTESIAN_POINT('Ctrl Pts',(21.1444389580236,17.5842032920565,36.0305840226698));
#54306=CARTESIAN_POINT('Ctrl Pts',(21.2130669433908,17.579971743575,36.0700433530018));
#54307=CARTESIAN_POINT('Ctrl Pts',(21.279614072805,17.5757401950936,36.1128970168661));
#54308=CARTESIAN_POINT('Ctrl Pts',(21.346084338447,17.5715135341675,36.1557011835654));
#54309=CARTESIAN_POINT('Ctrl Pts',(21.4104781322585,17.5672868732414,36.2018916401645));
#54310=CARTESIAN_POINT('Ctrl Pts',(21.4724343805696,17.5630602123153,36.2512362412096));
#54311=CARTESIAN_POINT('Ctrl Pts',(21.534351520166,17.5588362193893,36.3005496944049));
#54312=CARTESIAN_POINT('Ctrl Pts',(21.5938338025949,17.5546122264633,36.3530130488623));
#54313=CARTESIAN_POINT('Ctrl Pts',(21.6505504591888,17.5503882335373,36.4083518029532));
#54314=CARTESIAN_POINT('Ctrl Pts',(21.707248973679,17.5461655917509,36.4636728556936));
#54315=CARTESIAN_POINT('Ctrl Pts',(21.7611832837885,17.5419429499644,36.5218671544669));
#54316=CARTESIAN_POINT('Ctrl Pts',(21.8120580744441,17.537720308178,36.5826220063076));
#54317=CARTESIAN_POINT('Ctrl Pts',(21.8629324315612,17.5334977023755,36.6433763404151));
#54318=CARTESIAN_POINT('Ctrl Pts',(21.9107470212018,17.529275096573,36.706690823882));
#54319=CARTESIAN_POINT('Ctrl Pts',(21.955246544318,17.5250524907706,36.772219373604));
#54320=CARTESIAN_POINT('Ctrl Pts',(21.9997903164985,17.5208256861286,36.8378130830583));
#54321=CARTESIAN_POINT('Ctrl Pts',(22.0410121735985,17.5165988814866,36.9056248677755));
#54322=CARTESIAN_POINT('Ctrl Pts',(22.078700307134,17.5123720768447,36.9752798241247));
#54323=CARTESIAN_POINT('Ctrl Pts',(22.1164067036787,17.5081432239672,37.0449685340452));
#54324=CARTESIAN_POINT('Ctrl Pts',(22.1505757630878,17.5039143710898,37.1165017713586));
#54325=CARTESIAN_POINT('Ctrl Pts',(22.1810429481826,17.4996855182123,37.1894825102816));
#54326=CARTESIAN_POINT('Ctrl Pts',(22.2115648894856,17.4954490651596,37.2625944115855));
#54327=CARTESIAN_POINT('Ctrl Pts',(22.2383715040085,17.4912126121068,37.3371585703252));
#54328=CARTESIAN_POINT('Ctrl Pts',(22.2613475462707,17.486976159054,37.4127608015579));
#54329=CARTESIAN_POINT('Ctrl Pts',(22.2822298379241,17.4831257636198,37.4814735861281));
#54330=CARTESIAN_POINT('Ctrl Pts',(22.2999484669787,17.4792753681856,37.5510434348584));
#54331=CARTESIAN_POINT('Ctrl Pts',(22.3144538081643,17.4754249727513,37.621153458012));
#54332=CARTESIAN_POINT('Ctrl Pts',(22.3304179992604,17.4711873303739,37.6983146769765));
#54333=CARTESIAN_POINT('Ctrl Pts',(22.3425492376475,17.4669496879964,37.7764199493418));
#54334=CARTESIAN_POINT('Ctrl Pts',(22.3507428986342,17.4627120456189,37.8550545664423));
#54335=CARTESIAN_POINT('Ctrl Pts',(22.3589247768149,17.4584804971375,37.9335761038776));
#54336=CARTESIAN_POINT('Ctrl Pts',(22.3631802743976,17.454248948656,38.0126250119418));
#54337=CARTESIAN_POINT('Ctrl Pts',(22.3634556917679,17.4500174001746,38.0917760137368));
#54338=CARTESIAN_POINT('Ctrl Pts',(22.3637307910235,17.4457907392485,38.1708355939388));
#54339=CARTESIAN_POINT('Ctrl Pts',(22.3600349440432,17.4415640783224,38.2499965671349));
#54340=CARTESIAN_POINT('Ctrl Pts',(22.3523663448958,17.4373374173963,38.3288296753077));
#54341=CARTESIAN_POINT('Ctrl Pts',(22.3447025864073,17.4331134244703,38.407613021566));
#54342=CARTESIAN_POINT('Ctrl Pts',(22.3330710985764,17.4288894315443,38.4860684482406));
#54343=CARTESIAN_POINT('Ctrl Pts',(22.3175221027841,17.4246654386183,38.5637690632276));
#54344=CARTESIAN_POINT('Ctrl Pts',(22.3019780806894,17.4204427968318,38.6414448239178));
#54345=CARTESIAN_POINT('Ctrl Pts',(22.2825191309671,17.4162201550454,38.718365793051));
#54346=CARTESIAN_POINT('Ctrl Pts',(22.2592468111238,17.4119975132589,38.7941140304928));
#54347=CARTESIAN_POINT('Ctrl Pts',(22.2359746895996,17.4077749074565,38.8698616224328));
#54348=CARTESIAN_POINT('Ctrl Pts',(22.2088894016045,17.403552301654,38.9444360548706));
#54349=CARTESIAN_POINT('Ctrl Pts',(22.1781422966946,17.3993296958515,39.0174347803794));
#54350=CARTESIAN_POINT('Ctrl Pts',(22.1473646177353,17.3951028912096,39.0905060937514));
#54351=CARTESIAN_POINT('Ctrl Pts',(22.112918030922,17.3908760865676,39.1619981374081));
#54352=CARTESIAN_POINT('Ctrl Pts',(22.0750017358759,17.3866492819256,39.2315291587105));
#54353=CARTESIAN_POINT('Ctrl Pts',(22.0370670672575,17.3824204290482,39.3010938735276));
#54354=CARTESIAN_POINT('Ctrl Pts',(21.9956595861073,17.3781915761707,39.3686952726717));
#54355=CARTESIAN_POINT('Ctrl Pts',(21.9510227810537,17.3739627232933,39.433979215996));
#54356=CARTESIAN_POINT('Ctrl Pts',(21.9063057538799,17.3697262702405,39.4993804888727));
#54357=CARTESIAN_POINT('Ctrl Pts',(21.8583480906393,17.3654898171878,39.5624556098572));
#54358=CARTESIAN_POINT('Ctrl Pts',(21.8074345054459,17.361253364135,39.6228824476707));
#54359=CARTESIAN_POINT('Ctrl Pts',(21.7611605509071,17.3574029687007,39.677802735356));
#54360=CARTESIAN_POINT('Ctrl Pts',(21.7124455390639,17.3535525732665,39.7305356595026));
#54361=CARTESIAN_POINT('Ctrl Pts',(21.6615282856477,17.3497021778322,39.7808670967369));
#54362=CARTESIAN_POINT('Ctrl Pts',(21.6054901164498,17.3454645354547,39.836260532291));
#54363=CARTESIAN_POINT('Ctrl Pts',(21.5465735991057,17.3412268930772,39.8889525098605));
#54364=CARTESIAN_POINT('Ctrl Pts',(21.4850696683363,17.3369892506997,39.9386295225214));
#54365=CARTESIAN_POINT('Ctrl Pts',(21.4236541826332,17.3327577022183,39.9882350976885));
#54366=CARTESIAN_POINT('Ctrl Pts',(21.359659034336,17.3285261537368,40.0348340260054));
#54367=CARTESIAN_POINT('Ctrl Pts',(21.2934117438425,17.3242946052554,40.0781497672801));
#54368=CARTESIAN_POINT('Ctrl Pts',(21.2272409707988,17.3200679443292,40.1214154776775));
#54369=CARTESIAN_POINT('Ctrl Pts',(21.158823615332,17.3158412834031,40.1614052817935));
#54370=CARTESIAN_POINT('Ctrl Pts',(21.0885187850471,17.311614622477,40.1978840043004));
#54371=CARTESIAN_POINT('Ctrl Pts',(21.0182583333618,17.307390629551,40.234339700301));
#54372=CARTESIAN_POINT('Ctrl Pts',(20.9461131867294,17.303166636625,40.2672884984783));
#54373=CARTESIAN_POINT('Ctrl Pts',(20.8724687883813,17.2989426436989,40.2965401553808));
#54374=CARTESIAN_POINT('Ctrl Pts',(20.7988479468578,17.2947200019125,40.3257824554801));
#54375=CARTESIAN_POINT('Ctrl Pts',(20.7237292412991,17.290497360126,40.3513297898209));
#54376=CARTESIAN_POINT('Ctrl Pts',(20.6475185494969,17.2862747183395,40.373039852039));
#54377=CARTESIAN_POINT('Ctrl Pts',(20.5713085071374,17.2820521125371,40.394749729251));
#54378=CARTESIAN_POINT('Ctrl Pts',(20.4940069482651,17.2778295067346,40.4126222723031));
#54379=CARTESIAN_POINT('Ctrl Pts',(20.4160339418098,17.2736069009321,40.4265653225651));
#54380=CARTESIAN_POINT('Ctrl Pts',(20.3379834012073,17.2693800962901,40.440522237401));
#54381=CARTESIAN_POINT('Ctrl Pts',(20.2592605418775,17.2651532916481,40.4505417717367));
#54382=CARTESIAN_POINT('Ctrl Pts',(20.1802940351675,17.2609264870061,40.4565832261524));
#54383=CARTESIAN_POINT('Ctrl Pts',(20.1012892626721,17.2566976341287,40.4626276081512));
#54384=CARTESIAN_POINT('Ctrl Pts',(20.022041076807,17.2524687812512,40.4646900577993));
#54385=CARTESIAN_POINT('Ctrl Pts',(19.9429790937746,17.2482399283738,40.4627820587505));
#54386=CARTESIAN_POINT('Ctrl Pts',(19.863775019033,17.244003475321,40.4608706306093));
#54387=CARTESIAN_POINT('Ctrl Pts',(19.7847582843649,17.2397670222682,40.4549745307829));
#54388=CARTESIAN_POINT('Ctrl Pts',(19.7063540952675,17.2355305692154,40.4451572492125));
#54389=CARTESIAN_POINT('Ctrl Pts',(19.6350946884117,17.2316801737813,40.4362345925318));
#54390=CARTESIAN_POINT('Ctrl Pts',(19.564341435708,17.2278297783472,40.424073552306));
#54391=CARTESIAN_POINT('Ctrl Pts',(19.4944039542023,17.2239793829131,40.4087579083511));
#54392=CARTESIAN_POINT('Ctrl Pts',(19.4174326299637,17.2197417405356,40.3919019196681));
#54393=CARTESIAN_POINT('Ctrl Pts',(19.3411606841025,17.2155040981581,40.3711608784529));
#54394=CARTESIAN_POINT('Ctrl Pts',(19.2660094735217,17.2112664557806,40.3466081874551));
#54395=CARTESIAN_POINT('Ctrl Pts',(19.1909663333313,17.2070349072992,40.3220908041906));
#54396=CARTESIAN_POINT('Ctrl Pts',(19.1170411697246,17.2028033588177,40.2937728008795));
#54397=CARTESIAN_POINT('Ctrl Pts',(19.0446442442947,17.1985718103363,40.2617783931154));
#54398=CARTESIAN_POINT('Ctrl Pts',(18.9723309393126,17.1943451494102,40.2298209397757));
#54399=CARTESIAN_POINT('Ctrl Pts',(18.9015427912952,17.1901184884841,40.1941957090735));
#54400=CARTESIAN_POINT('Ctrl Pts',(18.8326725562312,17.1858918275579,40.1550759304523));
#54401=CARTESIAN_POINT('Ctrl Pts',(18.7638457942058,17.1816678346319,40.1159808454544));
#54402=CARTESIAN_POINT('Ctrl Pts',(18.6969349486741,17.1774438417059,40.0733958218646));
#54403=CARTESIAN_POINT('Ctrl Pts',(18.6323094191472,17.1732198487799,40.0275406392464));
#54404=CARTESIAN_POINT('Ctrl Pts',(18.5677045615556,17.1689972069934,39.9817001244441));
#54405=CARTESIAN_POINT('Ctrl Pts',(18.5053839503625,17.1647745652069,39.9325917989046));
#54406=CARTESIAN_POINT('Ctrl Pts',(18.4456878954677,17.1605519234204,39.8804786779415));
#54407=CARTESIAN_POINT('Ctrl Pts',(18.3859923492835,17.156329317618,39.8283660010697));
#54408=CARTESIAN_POINT('Ctrl Pts',(18.3289216671295,17.1521067118155,39.773248889047));
#54409=CARTESIAN_POINT('Ctrl Pts',(18.2747818163375,17.147884106013,39.7154295588667));
#54410=CARTESIAN_POINT('Ctrl Pts',(18.2205881304126,17.143657301371,39.6575527347835));
#54411=CARTESIAN_POINT('Ctrl Pts',(18.1693314183993,17.139430496729,39.596968668207));
#54412=CARTESIAN_POINT('Ctrl Pts',(18.1212791627667,17.135203692087,39.5340148034959));
#54413=CARTESIAN_POINT('Ctrl Pts',(18.0732036218531,17.1309748392096,39.4710304324451));
#54414=CARTESIAN_POINT('Ctrl Pts',(18.0283358963797,17.1267459863321,39.4056743625485));
#54415=CARTESIAN_POINT('Ctrl Pts',(17.9869002084452,17.1225171334547,39.3383132358745));
#54416=CARTESIAN_POINT('Ctrl Pts',(17.9453900514993,17.1182806804019,39.2708310464943));
#54417=CARTESIAN_POINT('Ctrl Pts',(17.9073244823368,17.1140442273491,39.2013370122531));
#54418=CARTESIAN_POINT('Ctrl Pts',(17.8728816957638,17.1098077742963,39.1302223840917));
#54419=CARTESIAN_POINT('Ctrl Pts',(17.841577596201,17.1059573788622,39.0655882582893));
#54420=CARTESIAN_POINT('Ctrl Pts',(17.8132655893203,17.1021069834281,38.9996159615739));
#54421=CARTESIAN_POINT('Ctrl Pts',(17.7880439305086,17.0982565879941,38.9326108259805));
#54422=CARTESIAN_POINT('Ctrl Pts',(17.7563093557472,17.0934119160922,38.8483031481727));
#54423=CARTESIAN_POINT('Ctrl Pts',(17.7293681785243,17.0885672441903,38.7620982479688));
#54424=CARTESIAN_POINT('Ctrl Pts',(17.7074200611923,17.0837225722885,38.6745151565246));
#54425=CARTESIAN_POINT('Ctrl Pts',(17.6855647710021,17.0788983903921,38.5873024881068));
#54426=CARTESIAN_POINT('Ctrl Pts',(17.6686605201809,17.0740742084958,38.4987234425967));
#54427=CARTESIAN_POINT('Ctrl Pts',(17.6568575551637,17.0692500265994,38.4093120173972));
#54428=CARTESIAN_POINT('Ctrl Pts',(17.6451385851259,17.064460175658,38.3205368823854));
#54429=CARTESIAN_POINT('Ctrl Pts',(17.6384486638185,17.0596703247165,38.2309413704542));
#54430=CARTESIAN_POINT('Ctrl Pts',(17.6368868042697,17.054880473775,38.1410665930586));
#54431=CARTESIAN_POINT('Ctrl Pts',(17.6366581565658,17.054179265769,38.1279094167254));
#54432=CARTESIAN_POINT('Ctrl Pts',(17.6365393239043,17.0534780577631,38.1147462846933));
#54433=CARTESIAN_POINT('Ctrl Pts',(17.6365305274028,17.0527768497571,38.101578924073));
#54434=CARTESIAN_POINT('',(17.6365307316195,16.259026849677,38.0981403439098));
#54435=CARTESIAN_POINT('Ctrl Pts',(17.6365305274025,17.0527768497283,38.101578923533));
#54436=CARTESIAN_POINT('Ctrl Pts',(17.6364773100099,17.0485346547335,38.0219185219947));
#54437=CARTESIAN_POINT('Ctrl Pts',(17.6404558360725,17.0442924597387,37.9422319286419));
#54438=CARTESIAN_POINT('Ctrl Pts',(17.6484474808675,17.0400502647438,37.8629531888815));
#54439=CARTESIAN_POINT('Ctrl Pts',(17.6564393552686,17.0358079478675,37.7836721713815));
#54440=CARTESIAN_POINT('Ctrl Pts',(17.6684445303095,17.0315656309911,37.7047994907601));
#54441=CARTESIAN_POINT('Ctrl Pts',(17.6843925358181,17.0273233141148,37.6267637876016));
#54442=CARTESIAN_POINT('Ctrl Pts',(17.7003457880481,17.023079601562,37.5487024115406));
#54443=CARTESIAN_POINT('Ctrl Pts',(17.7202443536963,17.0188358890093,37.4714790125329));
#54444=CARTESIAN_POINT('Ctrl Pts',(17.743967017387,17.0145921764565,37.3955103817214));
#54445=CARTESIAN_POINT('Ctrl Pts',(17.767720457143,17.0103429584185,37.3194431947116));
#54446=CARTESIAN_POINT('Ctrl Pts',(17.7953077558804,17.0060937403806,37.2446344658512));
#54447=CARTESIAN_POINT('Ctrl Pts',(17.8265585157788,17.0018445223426,37.1714836805062));
#54448=CARTESIAN_POINT('Ctrl Pts',(17.8578331082664,16.9975920637476,37.0982771085941));
#54449=CARTESIAN_POINT('Ctrl Pts',(17.892776519481,16.9933396051527,37.0267314113367));
#54450=CARTESIAN_POINT('Ctrl Pts',(17.9311722225806,16.9890871465577,36.9572217764247));
#54451=CARTESIAN_POINT('Ctrl Pts',(17.9696348049536,16.984827280849,36.8875910666658));
#54452=CARTESIAN_POINT('Ctrl Pts',(18.0115614352225,16.9805674151403,36.8200038878202));
#54453=CARTESIAN_POINT('Ctrl Pts',(18.0566924234116,16.9763075494316,36.7548062951107));
#54454=CARTESIAN_POINT('Ctrl Pts',(18.0700193970146,16.975049630646,36.7355537453243));
#54455=CARTESIAN_POINT('Ctrl Pts',(18.083625526166,16.9737917118605,36.7165093401657));
#54456=CARTESIAN_POINT('Ctrl Pts',(18.0975034837418,16.972533793075,36.6976814033446));
#54457=CARTESIAN_POINT('Ctrl Pts',(18.144255167406,16.9682961506975,36.6342543650721));
#54458=CARTESIAN_POINT('Ctrl Pts',(18.1942699535504,16.96405850832,36.5730487960201));
#54459=CARTESIAN_POINT('Ctrl Pts',(18.2473091472338,16.9598208659426,36.5144195966368));
#54460=CARTESIAN_POINT('Ctrl Pts',(18.3002720684751,16.9555893174611,36.4558747083431));
#54461=CARTESIAN_POINT('Ctrl Pts',(18.3562504482264,16.9513577689797,36.3998991768475));
#54462=CARTESIAN_POINT('Ctrl Pts',(18.4149637068756,16.9471262204983,36.3468170687636));
#54463=CARTESIAN_POINT('Ctrl Pts',(18.4736091500898,16.9428995595722,36.2937962719804));
#54464=CARTESIAN_POINT('Ctrl Pts',(18.534982848783,16.9386728986461,36.2436625700329));
#54465=CARTESIAN_POINT('Ctrl Pts',(18.5987665931446,16.93444623772,36.1967040743982));
#54466=CARTESIAN_POINT('Ctrl Pts',(18.6625100752192,16.930222244794,36.1497752204293));
#54467=CARTESIAN_POINT('Ctrl Pts',(18.7286602068436,16.925998251868,36.1060178716758));
#54468=CARTESIAN_POINT('Ctrl Pts',(18.7968657816441,16.921774258942,36.0656798448816));
#54469=CARTESIAN_POINT('Ctrl Pts',(18.8650495393507,16.9175516171556,36.0253547211165));
#54470=CARTESIAN_POINT('Ctrl Pts',(18.9352870314098,16.9133289753691,35.9884469858035));
#54471=CARTESIAN_POINT('Ctrl Pts',(19.0071994174011,16.9091063335827,35.9551602754305));
#54472=CARTESIAN_POINT('Ctrl Pts',(19.0791111905786,16.9048837277802,35.921873848716));
#54473=CARTESIAN_POINT('Ctrl Pts',(19.1526974032996,16.9006611219777,35.8922085812036));
#54474=CARTESIAN_POINT('Ctrl Pts',(19.2275574052582,16.8964385161752,35.8663207753286));
#54475=CARTESIAN_POINT('Ctrl Pts',(19.3024918458803,16.8922117115333,35.8404072273534));
#54476=CARTESIAN_POINT('Ctrl Pts',(19.3787021617585,16.8879849068913,35.818278797607));
#54477=CARTESIAN_POINT('Ctrl Pts',(19.4557712098074,16.8837581022493,35.8000422906441));
#54478=CARTESIAN_POINT('Ctrl Pts',(19.5328776041666,16.8795292493719,35.7817969465895));
#54479=CARTESIAN_POINT('Ctrl Pts',(19.6108430980497,16.8753003964945,35.7674473673279));
#54480=CARTESIAN_POINT('Ctrl Pts',(19.6892415077115,16.871071543617,35.7570489547644));
#54481=CARTESIAN_POINT('Ctrl Pts',(19.7677808164956,16.8668350905643,35.7466318539749));
#54482=CARTESIAN_POINT('Ctrl Pts',(19.8467541273414,16.8625986375115,35.7401801468548));
#54483=CARTESIAN_POINT('Ctrl Pts',(19.9257315338408,16.8583621844587,35.7376971752474));
#54484=CARTESIAN_POINT('Ctrl Pts',(19.9975119222006,16.8545117890245,35.7354404707775));
#54485=CARTESIAN_POINT('Ctrl Pts',(20.0692954247503,16.8506613935902,35.7364614652437));
#54486=CARTESIAN_POINT('Ctrl Pts',(20.1407631677291,16.846810998156,35.7407254989063));
#54487=CARTESIAN_POINT('Ctrl Pts',(20.2194186568709,16.8425733557785,35.7454183804704));
#54488=CARTESIAN_POINT('Ctrl Pts',(20.2979868501066,16.838335713401,35.7540577975682));
#54489=CARTESIAN_POINT('Ctrl Pts',(20.3760401028157,16.8340980710235,35.7666367016741));
#54490=CARTESIAN_POINT('Ctrl Pts',(20.4539811118842,16.829866522542,35.7791975168222));
#54491=CARTESIAN_POINT('Ctrl Pts',(20.5314081920214,16.8256349740606,35.7956864945732));
#54492=CARTESIAN_POINT('Ctrl Pts',(20.607896764797,16.8214034255791,35.816044666757));
#54493=CARTESIAN_POINT('Ctrl Pts',(20.6842969911588,16.817176764653,35.8363793246897));
#54494=CARTESIAN_POINT('Ctrl Pts',(20.7597604136338,16.8129501037269,35.8605741760148));
#54495=CARTESIAN_POINT('Ctrl Pts',(20.8338721319363,16.8087234428008,35.88851911415));
#54496=CARTESIAN_POINT('Ctrl Pts',(20.9079370686125,16.8044994498748,35.9164464125694));
#54497=CARTESIAN_POINT('Ctrl Pts',(20.9806515572187,16.8002754569488,35.9481189342661));
#54498=CARTESIAN_POINT('Ctrl Pts',(21.0516165382129,16.7960514640227,35.9833769590555));
#54499=CARTESIAN_POINT('Ctrl Pts',(21.1225588194548,16.7918288222363,36.0186237057692));
#54500=CARTESIAN_POINT('Ctrl Pts',(21.1917522848677,16.7876061804498,36.057453469622));
#54501=CARTESIAN_POINT('Ctrl Pts',(21.258819894101,16.7833835386634,36.0996593002402));
#54502=CARTESIAN_POINT('Ctrl Pts',(21.325886931806,16.7791609328609,36.141864771194));
#54503=CARTESIAN_POINT('Ctrl Pts',(21.3908277533633,16.7749383270584,36.1874460008249));
#54504=CARTESIAN_POINT('Ctrl Pts',(21.4532931535293,16.7707157212559,36.2361519775462));
#54505=CARTESIAN_POINT('Ctrl Pts',(21.5158206675183,16.766488916614,36.28490638611));
#54506=CARTESIAN_POINT('Ctrl Pts',(21.5758674727437,16.762262111972,36.3367914594122));
#54507=CARTESIAN_POINT('Ctrl Pts',(21.6331169085232,16.75803530733,36.391515407153));
#54508=CARTESIAN_POINT('Ctrl Pts',(21.6903940863761,16.7538064544525,36.44626587316));
#54509=CARTESIAN_POINT('Ctrl Pts',(21.7448708718096,16.7495776015751,36.5038576131085));
#54510=CARTESIAN_POINT('Ctrl Pts',(21.7962688030057,16.7453487486977,36.5639632724936));
#54511=CARTESIAN_POINT('Ctrl Pts',(21.8477591075475,16.7411122956449,36.6241769549203));
#54512=CARTESIAN_POINT('Ctrl Pts',(21.8961592146095,16.7368758425921,36.6869132122772));
#54513=CARTESIAN_POINT('Ctrl Pts',(21.9412323074948,16.7326393895393,36.7518132290968));
#54514=CARTESIAN_POINT('Ctrl Pts',(21.9821979995223,16.7287889941052,36.8107990659103));
#54515=CARTESIAN_POINT('Ctrl Pts',(22.0204158313138,16.724938598671,36.8715716831065));
#54516=CARTESIAN_POINT('Ctrl Pts',(22.0557413034838,16.7210882032368,36.9338447212953));
#54517=CARTESIAN_POINT('Ctrl Pts',(22.0946195746725,16.7168505608593,37.002380763922));
#54518=CARTESIAN_POINT('Ctrl Pts',(22.1301397068541,16.7126129184818,37.0729918163567));
#54519=CARTESIAN_POINT('Ctrl Pts',(22.162074830647,16.7083752761043,37.1453153046253));
#54520=CARTESIAN_POINT('Ctrl Pts',(22.1939640304786,16.7041437276228,37.2175347888796));
#54521=CARTESIAN_POINT('Ctrl Pts',(22.2222782722452,16.6999121791414,37.2914613932861));
#54522=CARTESIAN_POINT('Ctrl Pts',(22.2468359093081,16.6956806306599,37.3667068542911));
#54523=CARTESIAN_POINT('Ctrl Pts',(22.271365181622,16.6914539697338,37.4418654047105));
#54524=CARTESIAN_POINT('Ctrl Pts',(22.2921463271752,16.6872273088077,37.5183393411322));
#54525=CARTESIAN_POINT('Ctrl Pts',(22.3090458658434,16.6830006478815,37.595720682229));
#54526=CARTESIAN_POINT('Ctrl Pts',(22.3259347369962,16.6787766549555,37.673053177812));
#54527=CARTESIAN_POINT('Ctrl Pts',(22.3389467648653,16.6745526620295,37.7512914843803));
#54528=CARTESIAN_POINT('Ctrl Pts',(22.3479987112492,16.6703286691035,37.830013902447));
#54529=CARTESIAN_POINT('Ctrl Pts',(22.3570477621636,16.666106027317,37.90871113937));
#54530=CARTESIAN_POINT('Ctrl Pts',(22.3621391935407,16.6618833855305,37.9878917149128));
#54531=CARTESIAN_POINT('Ctrl Pts',(22.3632413728821,16.657660743744,38.0671266917047));
#54532=CARTESIAN_POINT('Ctrl Pts',(22.3643435428311,16.6534381379415,38.1463609932818));
#54533=CARTESIAN_POINT('Ctrl Pts',(22.3614565232461,16.649215532139,38.225649226439));
#54534=CARTESIAN_POINT('Ctrl Pts',(22.3546007947898,16.6449929263365,38.3045618196903));
#54535=CARTESIAN_POINT('Ctrl Pts',(22.3477382491916,16.6407661216945,38.3835528813872));
#54536=CARTESIAN_POINT('Ctrl Pts',(22.3368991524943,16.6365393170525,38.4621670889591));
#54537=CARTESIAN_POINT('Ctrl Pts',(22.3221559084624,16.6323125124106,38.5399799741959));
#54538=CARTESIAN_POINT('Ctrl Pts',(22.3074055201127,16.6280836595331,38.6178305661934));
#54539=CARTESIAN_POINT('Ctrl Pts',(22.2887473260514,16.6238548066556,38.6948786061157));
#54540=CARTESIAN_POINT('Ctrl Pts',(22.2663043567007,16.6196259537782,38.7707123106814));
#54541=CARTESIAN_POINT('Ctrl Pts',(22.243821052416,16.6153895007254,38.8466823050321));
#54542=CARTESIAN_POINT('Ctrl Pts',(22.2175395374991,16.6111530476726,38.9214331600404));
#54543=CARTESIAN_POINT('Ctrl Pts',(22.1876319028733,16.6069165946198,38.9945709018468));
#54544=CARTESIAN_POINT('Ctrl Pts',(22.1604496779387,16.6030661991858,39.0610437798883));
#54545=CARTESIAN_POINT('Ctrl Pts',(22.1302728228948,16.5992158037517,39.1261841750898));
#54546=CARTESIAN_POINT('Ctrl Pts',(22.0972628992025,16.5953654083177,39.1897149960098));
#54547=CARTESIAN_POINT('Ctrl Pts',(22.0609330588231,16.5911277659402,39.2596353207192));
#54548=CARTESIAN_POINT('Ctrl Pts',(22.0210346055926,16.5868901235628,39.3278681130252));
#54549=CARTESIAN_POINT('Ctrl Pts',(21.9777481980008,16.5826524811853,39.39402569766));
#54550=CARTESIAN_POINT('Ctrl Pts',(21.934524037962,16.5784209327038,39.4600881450917));
#54551=CARTESIAN_POINT('Ctrl Pts',(21.8879218534632,16.5741893842224,39.5240809222287));
#54552=CARTESIAN_POINT('Ctrl Pts',(21.8381684694959,16.569957835741,39.5856403059459));
#54553=CARTESIAN_POINT('Ctrl Pts',(21.7884725520609,16.5657311748149,39.647128586875));
#54554=CARTESIAN_POINT('Ctrl Pts',(21.7356329613737,16.5615045138888,39.7061886970871));
#54555=CARTESIAN_POINT('Ctrl Pts',(21.6799192817715,16.5572778529627,39.7624865857));
#54556=CARTESIAN_POINT('Ctrl Pts',(21.62424077038,16.5530538600367,39.8187489373312));
#54557=CARTESIAN_POINT('Ctrl Pts',(21.5656920999659,16.5488298671107,39.872252195892));
#54558=CARTESIAN_POINT('Ctrl Pts',(21.5045817110499,16.5446058741847,39.9226969895389));
#54559=CARTESIAN_POINT('Ctrl Pts',(21.4434908696723,16.5403832323982,39.973125647279));
#54560=CARTESIAN_POINT('Ctrl Pts',(21.3798402982613,16.5361605906118,40.0204974846483));
#54561=CARTESIAN_POINT('Ctrl Pts',(21.3139725997818,16.5319379488253,40.0645524803178));
#54562=CARTESIAN_POINT('Ctrl Pts',(21.2481054626052,16.5277153430229,40.108607100565));
#54563=CARTESIAN_POINT('Ctrl Pts',(21.1800216263722,16.5234927372204,40.1493446758855));
#54564=CARTESIAN_POINT('Ctrl Pts',(21.1100925930311,16.5192701314179,40.1865485558207));
#54565=CARTESIAN_POINT('Ctrl Pts',(21.0400940242417,16.5150433267759,40.2237894302394));
#54566=CARTESIAN_POINT('Ctrl Pts',(20.9682470081103,16.510816522134,40.2574893697395));
#54567=CARTESIAN_POINT('Ctrl Pts',(20.8949470292018,16.506589717492,40.2874780583638));
#54568=CARTESIAN_POINT('Ctrl Pts',(20.8216115304079,16.5023608646146,40.3174812789811));
#54569=CARTESIAN_POINT('Ctrl Pts',(20.7468221090414,16.4981320117371,40.3437695104374));
#54570=CARTESIAN_POINT('Ctrl Pts',(20.6709911665807,16.4939031588597,40.3662218106952));
#54571=CARTESIAN_POINT('Ctrl Pts',(20.5950239392989,16.4896667058069,40.3887144626568));
#54572=CARTESIAN_POINT('Ctrl Pts',(20.5180119074963,16.4854302527541,40.4073572979661));
#54573=CARTESIAN_POINT('Ctrl Pts',(20.4403792382781,16.4811937997014,40.4220802241511));
#54574=CARTESIAN_POINT('Ctrl Pts',(20.3698210445764,16.4773434042671,40.4354614860358));
#54575=CARTESIAN_POINT('Ctrl Pts',(20.2987505439706,16.4734930088329,40.4456053320298));
#54576=CARTESIAN_POINT('Ctrl Pts',(20.2274881231335,16.4696426133987,40.4524964600894));
#54577=CARTESIAN_POINT('Ctrl Pts',(20.1490586060567,16.4654049710212,40.4600806515816));
#54578=CARTESIAN_POINT('Ctrl Pts',(20.0701021824463,16.4611673286437,40.463752665573));
#54579=CARTESIAN_POINT('Ctrl Pts',(19.9910423993541,16.4569296862662,40.4634530251923));
#54580=CARTESIAN_POINT('Ctrl Pts',(19.9120963073325,16.4526981377847,40.4631538157063));
#54581=CARTESIAN_POINT('Ctrl Pts',(19.8330476159014,16.4484665893033,40.4588942959115));
#54582=CARTESIAN_POINT('Ctrl Pts',(19.7543249095037,16.4442350408218,40.4506667545209));
#54583=CARTESIAN_POINT('Ctrl Pts',(19.6756931300059,16.4400083798957,40.4424487161678));
#54584=CARTESIAN_POINT('Ctrl Pts',(19.5973870511724,16.4357817189696,40.4302718126205));
#54585=CARTESIAN_POINT('Ctrl Pts',(19.5198336417941,16.4315550580435,40.4141803536776));
#54586=CARTESIAN_POINT('Ctrl Pts',(19.4423291865447,16.4273310651175,40.3980990521651));
#54587=CARTESIAN_POINT('Ctrl Pts',(19.3655769155092,16.4231070721915,40.3781081948856));
#54588=CARTESIAN_POINT('Ctrl Pts',(19.2899958571583,16.4188830792655,40.3543035638635));
#54589=CARTESIAN_POINT('Ctrl Pts',(19.2144389751162,16.414660437479,40.3305065472904));
#54590=CARTESIAN_POINT('Ctrl Pts',(19.1400530085988,16.4104377956926,40.3028983202196));
#54591=CARTESIAN_POINT('Ctrl Pts',(19.067242572038,16.4062151539061,40.2716247423258));
#54592=CARTESIAN_POINT('Ctrl Pts',(18.9944327559439,16.4019925481036,40.2403514309352));
#54593=CARTESIAN_POINT('Ctrl Pts',(18.9231988732689,16.3977699423011,40.2054130171434));
#54594=CARTESIAN_POINT('Ctrl Pts',(18.8539248867709,16.3935473364987,40.1670032113514));
#54595=CARTESIAN_POINT('Ctrl Pts',(18.7845820161848,16.3893205318567,40.1285552119375));
#54596=CARTESIAN_POINT('Ctrl Pts',(18.7172033455678,16.3850937272147,40.0866291532722));
#54597=CARTESIAN_POINT('Ctrl Pts',(18.6521470237565,16.3808669225727,40.0414640855117));
#54598=CARTESIAN_POINT('Ctrl Pts',(18.5870591767916,16.3766380696953,39.9962771315507));
#54599=CARTESIAN_POINT('Ctrl Pts',(18.5242962921081,16.3724092168178,39.9478483284716));
#54600=CARTESIAN_POINT('Ctrl Pts',(18.4641843088386,16.3681803639404,39.8964577934598));
#54601=CARTESIAN_POINT('Ctrl Pts',(18.4039642911624,16.3639439108876,39.8449748983949));
#54602=CARTESIAN_POINT('Ctrl Pts',(18.3464050356718,16.3597074578348,39.7905199586914));
#54603=CARTESIAN_POINT('Ctrl Pts',(18.291796229896,16.355471004782,39.7334106405624));
#54604=CARTESIAN_POINT('Ctrl Pts',(18.2421637912015,16.3516206093479,39.6815055550976));
#54605=CARTESIAN_POINT('Ctrl Pts',(18.1949682489154,16.3477702139137,39.627408471479));
#54606=CARTESIAN_POINT('Ctrl Pts',(18.150396837276,16.3439198184796,39.5713798222558));
#54607=CARTESIAN_POINT('Ctrl Pts',(18.1014491845843,16.3396913722288,39.5098500038792));
#54608=CARTESIAN_POINT('Ctrl Pts',(18.055478848153,16.3354629259781,39.4457538867371));
#54609=CARTESIAN_POINT('Ctrl Pts',(18.0127667787908,16.3312344797273,39.379411804472));
#54610=CARTESIAN_POINT('Ctrl Pts',(17.9701141914137,16.3270119221254,39.3131621119884));
#54611=CARTESIAN_POINT('Ctrl Pts',(17.9307111177636,16.3227893645235,39.244673053702));
#54612=CARTESIAN_POINT('Ctrl Pts',(17.8947981223519,16.3185668069216,39.1742976753427));
#54613=CARTESIAN_POINT('Ctrl Pts',(17.8589238529128,16.3143488026199,39.1039981846934));
#54614=CARTESIAN_POINT('Ctrl Pts',(17.8265324023101,16.3101307983182,39.0318168291015));
#54615=CARTESIAN_POINT('Ctrl Pts',(17.7978200563048,16.3059127940165,38.9581339851599));
#54616=CARTESIAN_POINT('Ctrl Pts',(17.7691276003764,16.3016977116784,38.8845021839802));
#54617=CARTESIAN_POINT('Ctrl Pts',(17.7441093602402,16.2974826293404,38.8093713963082));
#54618=CARTESIAN_POINT('Ctrl Pts',(17.7229142175799,16.2932675470023,38.7331435701324));
#54619=CARTESIAN_POINT('Ctrl Pts',(17.7017280833147,16.2890542561656,38.6569481424357));
#54620=CARTESIAN_POINT('Ctrl Pts',(17.684361942341,16.2848409653289,38.5796570559792));
#54621=CARTESIAN_POINT('Ctrl Pts',(17.6709148711716,16.2806276744923,38.501687569599));
#54622=CARTESIAN_POINT('Ctrl Pts',(17.6574647965297,16.2764134425954,38.4237006683329));
#54623=CARTESIAN_POINT('Ctrl Pts',(17.6479356260872,16.2721992106985,38.3450355274437));
#54624=CARTESIAN_POINT('Ctrl Pts',(17.6423751305849,16.2679849788017,38.2661186805136));
#54625=CARTESIAN_POINT('Ctrl Pts',(17.6384351768251,16.2649989357772,38.210201230773));
#54626=CARTESIAN_POINT('Ctrl Pts',(17.6364866553968,16.2620128927528,38.1541576109328));
#54627=CARTESIAN_POINT('Ctrl Pts',(17.6365307316187,16.2590268497283,38.0981403448729));
#54628=CARTESIAN_POINT('',(17.636530005568,15.4652768497734,38.0998377669048));
#54629=CARTESIAN_POINT('Ctrl Pts',(17.6365307316195,16.259026849677,38.0981403439098));
#54630=CARTESIAN_POINT('Ctrl Pts',(17.6366038466735,16.2540735080734,38.0052171501665));
#54631=CARTESIAN_POINT('Ctrl Pts',(17.6421609997246,16.2491201664698,37.9125229754199));
#54632=CARTESIAN_POINT('Ctrl Pts',(17.653098020552,16.2441668248662,37.8206408409181));
#54633=CARTESIAN_POINT('Ctrl Pts',(17.6641551639284,16.239159080146,37.727749554438));
#54634=CARTESIAN_POINT('Ctrl Pts',(17.6807109058829,16.2341513354258,37.6356883472259));
#54635=CARTESIAN_POINT('Ctrl Pts',(17.7026082430101,16.2291435907056,37.5450391402859));
#54636=CARTESIAN_POINT('Ctrl Pts',(17.7185635738396,16.2254947349905,37.4789882740199));
#54637=CARTESIAN_POINT('Ctrl Pts',(17.7373538323789,16.2218458792755,37.4136866406475));
#54638=CARTESIAN_POINT('Ctrl Pts',(17.7589024384412,16.2181970235604,37.3493521728034));
#54639=CARTESIAN_POINT('Ctrl Pts',(17.7839281707136,16.2139593811829,37.2746365664432));
#54640=CARTESIAN_POINT('Ctrl Pts',(17.8127413629706,16.2097217388054,37.2010335741935));
#54641=CARTESIAN_POINT('Ctrl Pts',(17.8452237804385,16.2054840964279,37.1289542315048));
#54642=CARTESIAN_POINT('Ctrl Pts',(17.8776594869154,16.2012525479464,37.0569785417395));
#54643=CARTESIAN_POINT('Ctrl Pts',(17.913753748976,16.1970209994649,36.9865225741272));
#54644=CARTESIAN_POINT('Ctrl Pts',(17.9533390046607,16.1927894509835,36.9179808753422));
#54645=CARTESIAN_POINT('Ctrl Pts',(17.9928785382819,16.1885627900573,36.8495183441121));
#54646=CARTESIAN_POINT('Ctrl Pts',(18.0359008192869,16.1843361291312,36.7829660917124));
#54647=CARTESIAN_POINT('Ctrl Pts',(18.0821914356272,16.1801094682051,36.7186959960536));
#54648=CARTESIAN_POINT('Ctrl Pts',(18.1284528318879,16.1758854752791,36.654466469682));
#54649=CARTESIAN_POINT('Ctrl Pts',(18.1779781952551,16.1716614823531,36.5925166200672));
#54650=CARTESIAN_POINT('Ctrl Pts',(18.2305093414933,16.167437489427,36.5331901039509));
#54651=CARTESIAN_POINT('Ctrl Pts',(18.2830236844577,16.1632148476406,36.4738825647609));
#54652=CARTESIAN_POINT('Ctrl Pts',(18.3385415904698,16.1589922058541,36.4171970434279));
#54653=CARTESIAN_POINT('Ctrl Pts',(18.3967650140825,16.1547695640676,36.3634436315425));
#54654=CARTESIAN_POINT('Ctrl Pts',(18.4549879415343,16.1505469582652,36.3096906777262));
#54655=CARTESIAN_POINT('Ctrl Pts',(18.5159159953454,16.1463243524627,36.2588701006136));
#54656=CARTESIAN_POINT('Ctrl Pts',(18.5792158437952,16.1421017466602,36.2112536373623));
#54657=CARTESIAN_POINT('Ctrl Pts',(18.6425786358197,16.1378749420182,36.1635898256498));
#54658=CARTESIAN_POINT('Ctrl Pts',(18.708317558001,16.1336481373762,36.119136774463));
#54659=CARTESIAN_POINT('Ctrl Pts',(18.7760683885785,16.1294213327342,36.0781241750634));
#54660=CARTESIAN_POINT('Ctrl Pts',(18.8438520500214,16.1251924798568,36.0370917016767));
#54661=CARTESIAN_POINT('Ctrl Pts',(18.9136491487901,16.1209636269793,35.9995032238547));
#54662=CARTESIAN_POINT('Ctrl Pts',(18.9850710807823,16.1167347741018,35.9655422867071));
#54663=CARTESIAN_POINT('Ctrl Pts',(19.0566213736375,16.1124983210491,35.9315203143134));
#54664=CARTESIAN_POINT('Ctrl Pts',(19.1298019005486,16.1082618679963,35.9011390893245));
#54665=CARTESIAN_POINT('Ctrl Pts',(19.2042045345491,16.1040254149435,35.8745337526559));
#54666=CARTESIAN_POINT('Ctrl Pts',(19.2718270382484,16.1001750195095,35.8503528953319));
#54667=CARTESIAN_POINT('Ctrl Pts',(19.3404586002684,16.0963246240755,35.8292905506849));
#54668=CARTESIAN_POINT('Ctrl Pts',(19.4097851015669,16.0924742286415,35.811411610934));
#54669=CARTESIAN_POINT('Ctrl Pts',(19.486083997309,16.088236586264,35.7917345273588));
#54670=CARTESIAN_POINT('Ctrl Pts',(19.5635112061767,16.0839989438865,35.7758402565973));
#54671=CARTESIAN_POINT('Ctrl Pts',(19.641657564465,16.079761301509,35.7638533565303));
#54672=CARTESIAN_POINT('Ctrl Pts',(19.7196915452233,16.0755297530276,35.751883694096));
#54673=CARTESIAN_POINT('Ctrl Pts',(19.7984421621203,16.0712982045461,35.7438103141239));
#54674=CARTESIAN_POINT('Ctrl Pts',(19.8774872328106,16.0670666560647,35.7397074200906));
#54675=CARTESIAN_POINT('Ctrl Pts',(19.9564410042614,16.0628399951386,35.7356092650132));
#54676=CARTESIAN_POINT('Ctrl Pts',(20.0356880878631,16.0586133342125,35.7354725064737));
#54677=CARTESIAN_POINT('Ctrl Pts',(20.1147998151938,16.0543866732864,35.7393197075141));
#54678=CARTESIAN_POINT('Ctrl Pts',(20.1938616047369,16.0501626803604,35.7431644800813));
#54679=CARTESIAN_POINT('Ctrl Pts',(20.272787740605,16.0459386874344,35.7509881979192));
#54680=CARTESIAN_POINT('Ctrl Pts',(20.3511494014435,16.0417146945083,35.7627613432159));
#54681=CARTESIAN_POINT('Ctrl Pts',(20.4294859965346,16.0374920527219,35.7745307226062));
#54682=CARTESIAN_POINT('Ctrl Pts',(20.5072580119162,16.0332694109354,35.790246951167));
#54683=CARTESIAN_POINT('Ctrl Pts',(20.5840430850772,16.029046769149,35.8098288021038));
#54684=CARTESIAN_POINT('Ctrl Pts',(20.6608275039008,16.0248241633465,35.8294104861703));
#54685=CARTESIAN_POINT('Ctrl Pts',(20.7366245433448,16.020601557544,35.8528576098902));
#54686=CARTESIAN_POINT('Ctrl Pts',(20.811024807616,16.0163789517415,35.8800384682767));
#54687=CARTESIAN_POINT('Ctrl Pts',(20.8854990534009,16.0121521470995,35.9072463545382));
#54688=CARTESIAN_POINT('Ctrl Pts',(20.9585733083183,16.0079253424576,35.9381952304075));
#54689=CARTESIAN_POINT('Ctrl Pts',(21.0298566329685,16.0036985378156,35.9727045911696));
#54690=CARTESIAN_POINT('Ctrl Pts',(21.1011745002687,15.9994696849381,36.0072306745633));
#54691=CARTESIAN_POINT('Ctrl Pts',(21.1706992967924,15.9952408320607,36.0453204544234));
#54692=CARTESIAN_POINT('Ctrl Pts',(21.2380655214756,15.9910119791832,36.0867478534884));
#54693=CARTESIAN_POINT('Ctrl Pts',(21.305552818027,15.9867755261305,36.128249706668));
#54694=CARTESIAN_POINT('Ctrl Pts',(21.3708734039049,15.9825390730777,36.1731008985285));
#54695=CARTESIAN_POINT('Ctrl Pts',(21.4336917557667,15.9783026200249,36.221032626588));
#54696=CARTESIAN_POINT('Ctrl Pts',(21.4907856246657,15.9744522245907,36.2645964533493));
#54697=CARTESIAN_POINT('Ctrl Pts',(21.5458127406541,15.9706018291565,36.3107042636834));
#54698=CARTESIAN_POINT('Ctrl Pts',(21.5985476815967,15.9667514337223,36.3591278764476));
#54699=CARTESIAN_POINT('Ctrl Pts',(21.6565863491395,15.9625137913448,36.4124216113454));
#54700=CARTESIAN_POINT('Ctrl Pts',(21.7120659185459,15.9582761489673,36.4687209709738));
#54701=CARTESIAN_POINT('Ctrl Pts',(21.7646591799044,15.9540385065898,36.5277505224427));
#54702=CARTESIAN_POINT('Ctrl Pts',(21.8171768100892,15.9498069581084,36.5866951871001));
#54703=CARTESIAN_POINT('Ctrl Pts',(21.866816065716,15.9455754096269,36.6483618995684));
#54704=CARTESIAN_POINT('Ctrl Pts',(21.9132848910425,15.9413438611455,36.7124368963508));
#54705=CARTESIAN_POINT('Ctrl Pts',(21.9597000435925,15.9371172002194,36.7764378847426));
#54706=CARTESIAN_POINT('Ctrl Pts',(22.0029517692095,15.9328905392933,36.8428412520777));
#54707=CARTESIAN_POINT('Ctrl Pts',(22.0427878010359,15.9286638783672,36.9112996841765));
#54708=CARTESIAN_POINT('Ctrl Pts',(22.0825986871176,15.9244398854412,36.9797149031797));
#54709=CARTESIAN_POINT('Ctrl Pts',(22.1189979238627,15.9202158925152,37.0501822079974));
#54710=CARTESIAN_POINT('Ctrl Pts',(22.1517768501069,15.9159918995891,37.1223258067004));
#54711=CARTESIAN_POINT('Ctrl Pts',(22.1845452912711,15.9117692578027,37.1944463286437));
#54712=CARTESIAN_POINT('Ctrl Pts',(22.2136955277962,15.9075466160162,37.268241653206));
#54713=CARTESIAN_POINT('Ctrl Pts',(22.2390657912856,15.9033239742298,37.3433132595358));
#54714=CARTESIAN_POINT('Ctrl Pts',(22.264435838578,15.8991013684273,37.4183842261298));
#54715=CARTESIAN_POINT('Ctrl Pts',(22.2860258281536,15.8948787626248,37.4947310083105));
#54716=CARTESIAN_POINT('Ctrl Pts',(22.3037233943808,15.8906561568223,37.5719384855126));
#54717=CARTESIAN_POINT('Ctrl Pts',(22.3214385585661,15.8864293521804,37.6492227356412));
#54718=CARTESIAN_POINT('Ctrl Pts',(22.3352534630509,15.8822025475384,37.7273689323715));
#54719=CARTESIAN_POINT('Ctrl Pts',(22.3451067251845,15.8779757428964,37.8059508741821));
#54720=CARTESIAN_POINT('Ctrl Pts',(22.3549647620363,15.873746890019,37.8845708954249));
#54721=CARTESIAN_POINT('Ctrl Pts',(22.3608572972967,15.8695180371415,37.9636266143177));
#54722=CARTESIAN_POINT('Ctrl Pts',(22.3627750246368,15.8652891842641,38.0426883619788));
#54723=CARTESIAN_POINT('Ctrl Pts',(22.3646961985532,15.8610527312113,38.1218922009259));
#54724=CARTESIAN_POINT('Ctrl Pts',(22.3626283032048,15.8568162781586,38.2011016205651));
#54725=CARTESIAN_POINT('Ctrl Pts',(22.3566141910047,15.8525798251058,38.2798888424977));
#54726=CARTESIAN_POINT('Ctrl Pts',(22.3511481301591,15.8487294296716,38.3514963773439));
#54727=CARTESIAN_POINT('Ctrl Pts',(22.3424229969077,15.8448790342374,38.4227549608094));
#54728=CARTESIAN_POINT('Ctrl Pts',(22.3305074997377,15.8410286388033,38.4933512864683));
#54729=CARTESIAN_POINT('Ctrl Pts',(22.3173936217945,15.8367909964258,38.5710477169836));
#54730=CARTESIAN_POINT('Ctrl Pts',(22.3003654146412,15.8325533540483,38.6482334713512));
#54731=CARTESIAN_POINT('Ctrl Pts',(22.2794758180211,15.8283157116708,38.7244841358731));
#54732=CARTESIAN_POINT('Ctrl Pts',(22.2586162614607,15.8240841631893,38.8006251489472));
#54733=CARTESIAN_POINT('Ctrl Pts',(22.2339064656764,15.8198526147078,38.8758332942387));
#54734=CARTESIAN_POINT('Ctrl Pts',(22.2054506603784,15.8156210662264,38.9496927830319));
#54735=CARTESIAN_POINT('Ctrl Pts',(22.1770277223214,15.8113944053003,39.0234669620759));
#54736=CARTESIAN_POINT('Ctrl Pts',(22.1448675407564,15.8071677443741,39.0958951450162));
#54737=CARTESIAN_POINT('Ctrl Pts',(22.1091241484778,15.802941083448,39.1665766579143));
#54738=CARTESIAN_POINT('Ctrl Pts',(22.0734033185423,15.798717090522,39.237213554439));
#54739=CARTESIAN_POINT('Ctrl Pts',(22.0341039783771,15.794493097596,39.3061055521348));
#54740=CARTESIAN_POINT('Ctrl Pts',(21.9914277859658,15.7902691046699,39.3728730550151));
#54741=CARTESIAN_POINT('Ctrl Pts',(21.9487652444987,15.7860464628835,39.4396192008014));
#54742=CARTESIAN_POINT('Ctrl Pts',(21.902728248056,15.781823821097,39.504241806562));
#54743=CARTESIAN_POINT('Ctrl Pts',(21.853563046577,15.7776011793105,39.5663882409732));
#54744=CARTESIAN_POINT('Ctrl Pts',(21.8043982640677,15.773378573508,39.6285341457927));
#54745=CARTESIAN_POINT('Ctrl Pts',(21.7521056214914,15.7691559677055,39.688203554468));
#54746=CARTESIAN_POINT('Ctrl Pts',(21.6969721854293,15.764933361903,39.745076242239));
#54747=CARTESIAN_POINT('Ctrl Pts',(21.6417839262414,15.7607065572611,39.8020054825985));
#54748=CARTESIAN_POINT('Ctrl Pts',(21.583749558053,15.7564797526191,39.8561321096719));
#54749=CARTESIAN_POINT('Ctrl Pts',(21.5231931947481,15.7522529479771,39.9071726349116));
#54750=CARTESIAN_POINT('Ctrl Pts',(21.4626074868906,15.7480240950996,39.9582378934955));
#54751=CARTESIAN_POINT('Ctrl Pts',(21.399497722983,15.7437952422221,40.0062137870362));
#54752=CARTESIAN_POINT('Ctrl Pts',(21.3342192725583,15.7395663893447,40.0508586247173));
#54753=CARTESIAN_POINT('Ctrl Pts',(21.2688235024532,15.7353299362919,40.0955836989552));
#54754=CARTESIAN_POINT('Ctrl Pts',(21.201251658751,15.7310934832391,40.13696551005));
#54755=CARTESIAN_POINT('Ctrl Pts',(21.1318859169762,15.7268570301863,40.1748071505205));
#54756=CARTESIAN_POINT('Ctrl Pts',(21.068841305817,15.7230066347523,40.2092003747266));
#54757=CARTESIAN_POINT('Ctrl Pts',(21.0043153897533,15.7191562393182,40.2406697220902));
#54758=CARTESIAN_POINT('Ctrl Pts',(20.9386083918615,15.7153058438842,40.2691022861145));
#54759=CARTESIAN_POINT('Ctrl Pts',(20.8662930248988,15.7110682015067,40.3003944066965));
#54760=CARTESIAN_POINT('Ctrl Pts',(20.7922753391364,15.7068305591292,40.3281249442038));
#54761=CARTESIAN_POINT('Ctrl Pts',(20.7169401784524,15.7025929167518,40.3521072846161));
#54762=CARTESIAN_POINT('Ctrl Pts',(20.6417133526858,15.6983613682703,40.3760551374816));
#54763=CARTESIAN_POINT('Ctrl Pts',(20.5651732574545,15.6941298197889,40.3962653563772));
#54764=CARTESIAN_POINT('Ctrl Pts',(20.4877254203701,15.6898982713074,40.4125990476572));
#54765=CARTESIAN_POINT('Ctrl Pts',(20.4103670376762,15.6856716103813,40.4289138730726));
#54766=CARTESIAN_POINT('Ctrl Pts',(20.3321034530588,15.6814449494552,40.4413609725379));
#54767=CARTESIAN_POINT('Ctrl Pts',(20.253354624421,15.6772182885291,40.4498514581106));
#54768=CARTESIAN_POINT('Ctrl Pts',(20.1746555044978,15.6729942956031,40.4583365842242));
#54769=CARTESIAN_POINT('Ctrl Pts',(20.0954722133811,15.6687703026771,40.4628700036633));
#54770=CARTESIAN_POINT('Ctrl Pts',(20.0162329514462,15.6645463097511,40.4634142531912));
#54771=CARTESIAN_POINT('Ctrl Pts',(19.9370190359792,15.6603236679647,40.4639583286286));
#54772=CARTESIAN_POINT('Ctrl Pts',(19.8577496536712,15.6561010261782,40.4605157648734));
#54773=CARTESIAN_POINT('Ctrl Pts',(19.7788546581015,15.6518783843917,40.4531011832594));
#54774=CARTESIAN_POINT('Ctrl Pts',(19.6999603348493,15.6476557785893,40.44568666483));
#54775=CARTESIAN_POINT('Ctrl Pts',(19.6214408585744,15.6434331727868,40.4343002411278));
#54776=CARTESIAN_POINT('Ctrl Pts',(19.5437211159885,15.6392105669843,40.419008413289));
#54777=CARTESIAN_POINT('Ctrl Pts',(19.465924091094,15.6349837623423,40.4037013796901));
#54778=CARTESIAN_POINT('Ctrl Pts',(19.3889288493932,15.6307569577003,40.3844812755086));
#54779=CARTESIAN_POINT('Ctrl Pts',(19.3131496269433,15.6265301530584,40.3614656764877));
#54780=CARTESIAN_POINT('Ctrl Pts',(19.2373336832101,15.6223013001809,40.3384389245108));
#54781=CARTESIAN_POINT('Ctrl Pts',(19.162735374289,15.6180724473035,40.3116131725631));
#54782=CARTESIAN_POINT('Ctrl Pts',(19.0897508870357,15.613843594426,40.2811549677287));
#54783=CARTESIAN_POINT('Ctrl Pts',(19.016635230665,15.6096071413733,40.2506420228257));
#54784=CARTESIAN_POINT('Ctrl Pts',(18.9451396152065,15.6053706883205,40.2164837833961));
#54785=CARTESIAN_POINT('Ctrl Pts',(18.8756372516807,15.6011342352677,40.1788936603617));
#54786=CARTESIAN_POINT('Ctrl Pts',(18.812468468774,15.5972838398335,40.1447290334203));
#54787=CARTESIAN_POINT('Ctrl Pts',(18.7509461044902,15.5934334443993,40.1077302177537));
#54788=CARTESIAN_POINT('Ctrl Pts',(18.6913282945177,15.5895830489651,40.068087601752));
#54789=CARTESIAN_POINT('Ctrl Pts',(18.6258430801067,15.5853537092646,40.0245434794524));
#54790=CARTESIAN_POINT('Ctrl Pts',(18.562408207784,15.5811243695641,39.9776440370525));
#54791=CARTESIAN_POINT('Ctrl Pts',(18.5013888786173,15.5768950298636,39.9276091342976));
#54792=CARTESIAN_POINT('Ctrl Pts',(18.4404573839953,15.5726717781049,39.877646254506));
#54793=CARTESIAN_POINT('Ctrl Pts',(18.3819348891868,15.5684485263462,39.8245571725519));
#54794=CARTESIAN_POINT('Ctrl Pts',(18.3261579033514,15.5642252745875,39.7686051289587));
#54795=CARTESIAN_POINT('Ctrl Pts',(18.270445109776,15.5600068832578,39.7127174790947));
#54796=CARTESIAN_POINT('Ctrl Pts',(18.2174718773639,15.555788491928,39.653973746503));
#54797=CARTESIAN_POINT('Ctrl Pts',(18.1675406756892,15.5515701005982,39.5926765442139));
#54798=CARTESIAN_POINT('Ctrl Pts',(18.1176407085403,15.5473543480884,39.5314176864665));
#54799=CARTESIAN_POINT('Ctrl Pts',(18.0707792919992,15.5431385955786,39.4676088933301));
#54800=CARTESIAN_POINT('Ctrl Pts',(18.0272202703293,15.5389228430688,39.4015877147163));
#54801=CARTESIAN_POINT('Ctrl Pts',(17.9836747889534,15.534708401023,39.3355870587437));
#54802=CARTESIAN_POINT('Ctrl Pts',(17.9434299231902,15.5304939589772,39.2673757756398));
#54803=CARTESIAN_POINT('Ctrl Pts',(17.9067067320743,15.5262795169313,39.1973211632686));
#54804=CARTESIAN_POINT('Ctrl Pts',(17.8699833996676,15.5220650586706,39.1272662813651));
#54805=CARTESIAN_POINT('Ctrl Pts',(17.8367819859386,15.5178506004099,39.0553684739288));
#54806=CARTESIAN_POINT('Ctrl Pts',(17.8072773195312,15.5136361421492,38.9820190969915));
#54807=CARTESIAN_POINT('Ctrl Pts',(17.7777432368352,15.5094174820542,38.9085965903869));
#54808=CARTESIAN_POINT('Ctrl Pts',(17.751913438361,15.5051988219591,38.8337200617956));
#54809=CARTESIAN_POINT('Ctrl Pts',(17.7299140914899,15.5009801618641,38.7577996723045));
#54810=CARTESIAN_POINT('Ctrl Pts',(17.7079037028745,15.4967593843713,38.6818411774307));
#54811=CARTESIAN_POINT('Ctrl Pts',(17.6897277029013,15.4925386068786,38.6048382369578));
#54812=CARTESIAN_POINT('Ctrl Pts',(17.6754613444804,15.4883178293859,38.5272124528792));
#54813=CARTESIAN_POINT('Ctrl Pts',(17.6611698301982,15.4840896093987,38.4494497913022));
#54814=CARTESIAN_POINT('Ctrl Pts',(17.6508017904135,15.4798613894116,38.3710625597964));
#54815=CARTESIAN_POINT('Ctrl Pts',(17.644380654783,15.4756331694244,38.2924784178537));
#54816=CARTESIAN_POINT('Ctrl Pts',(17.6391381545257,15.4721810628741,38.2283188348667));
#54817=CARTESIAN_POINT('Ctrl Pts',(17.6365255994157,15.4687289563237,38.1640281765003));
#54818=CARTESIAN_POINT('Ctrl Pts',(17.636530005568,15.4652768497734,38.0998377669048));
#54819=CARTESIAN_POINT('',(17.6365308344677,14.6715268497713,38.1019860710541));
#54820=CARTESIAN_POINT('Ctrl Pts',(17.6365300055681,15.4652768497283,38.0998377660665));
#54821=CARTESIAN_POINT('Ctrl Pts',(17.6365306082695,15.4648046511675,38.0910574406093));
#54822=CARTESIAN_POINT('Ctrl Pts',(17.6365801393059,15.4643324526068,38.0822773116373));
#54823=CARTESIAN_POINT('Ctrl Pts',(17.6366785934394,15.463860254046,38.0734977323131));
#54824=CARTESIAN_POINT('Ctrl Pts',(17.6375621484591,15.4596226116686,37.9947073240134));
#54825=CARTESIAN_POINT('Ctrl Pts',(17.6423918430063,15.4553849692911,37.9158132522039));
#54826=CARTESIAN_POINT('Ctrl Pts',(17.6511813180016,15.4511473269136,37.8372430020054));
#54827=CARTESIAN_POINT('Ctrl Pts',(17.6599581533869,15.4469157784321,37.7587857389101));
#54828=CARTESIAN_POINT('Ctrl Pts',(17.6726834091438,15.4426842299507,37.6806518346703));
#54829=CARTESIAN_POINT('Ctrl Pts',(17.6893187190147,15.4384526814692,37.6032682226753));
#54830=CARTESIAN_POINT('Ctrl Pts',(17.7059348146433,15.4342260205431,37.5259739908891));
#54831=CARTESIAN_POINT('Ctrl Pts',(17.726451891496,15.429999359617,37.4494287851626));
#54832=CARTESIAN_POINT('Ctrl Pts',(17.7507800366961,15.4257726986909,37.3740523451549));
#54833=CARTESIAN_POINT('Ctrl Pts',(17.7750928252128,15.4215487057649,37.2987234851051));
#54834=CARTESIAN_POINT('Ctrl Pts',(17.8032117634887,15.4173247128389,37.224562371345));
#54835=CARTESIAN_POINT('Ctrl Pts',(17.8349966170261,15.4131007199129,37.1519753206737));
#54836=CARTESIAN_POINT('Ctrl Pts',(17.8667713034602,15.4088780781264,37.0794114886103));
#54837=CARTESIAN_POINT('Ctrl Pts',(17.9022093886558,15.4046554363399,37.0084211488845));
#54838=CARTESIAN_POINT('Ctrl Pts',(17.9411223983249,15.4004327945535,36.9393909089532));
#54839=CARTESIAN_POINT('Ctrl Pts',(17.9800350763898,15.396210188751,36.8703612572753));
#54840=CARTESIAN_POINT('Ctrl Pts',(18.0224223886087,15.3919875829485,36.8032920798383));
#54841=CARTESIAN_POINT('Ctrl Pts',(18.068050504909,15.387764977146,36.738544312393));
#54842=CARTESIAN_POINT('Ctrl Pts',(18.1137239925146,15.383538172504,36.6737321616032));
#54843=CARTESIAN_POINT('Ctrl Pts',(18.1626444506268,15.3793113678621,36.6112464158093));
#54844=CARTESIAN_POINT('Ctrl Pts',(18.2145357442956,15.3750845632201,36.5514174763669));
#54845=CARTESIAN_POINT('Ctrl Pts',(18.266452183576,15.3708557103426,36.4915595448689));
#54846=CARTESIAN_POINT('Ctrl Pts',(18.3213420013016,15.3666268574652,36.4343613231174));
#54847=CARTESIAN_POINT('Ctrl Pts',(18.3788916926052,15.3623980045877,36.3801167782098));
#54848=CARTESIAN_POINT('Ctrl Pts',(18.4365448133155,15.3581615515349,36.3257747439678));
#54849=CARTESIAN_POINT('Ctrl Pts',(18.4968670015372,15.3539250984822,36.274397297954));
#54850=CARTESIAN_POINT('Ctrl Pts',(18.5595113142642,15.3496886454294,36.2262383323466));
#54851=CARTESIAN_POINT('Ctrl Pts',(18.6164470037892,15.3458382499952,36.1824679756406));
#54852=CARTESIAN_POINT('Ctrl Pts',(18.6753002715313,15.3419878545611,36.1413558540245));
#54853=CARTESIAN_POINT('Ctrl Pts',(18.7357920812526,15.3381374591269,36.1030601463548));
#54854=CARTESIAN_POINT('Ctrl Pts',(18.8023677514014,15.3338998167494,36.060912913305));
#54855=CARTESIAN_POINT('Ctrl Pts',(18.8711784054627,15.3296621743719,36.0220195410704));
#54856=CARTESIAN_POINT('Ctrl Pts',(18.9418728652621,15.3254245319944,35.9866241679173));
#54857=CARTESIAN_POINT('Ctrl Pts',(19.0124656636541,15.321192983513,35.9512796946997));
#54858=CARTESIAN_POINT('Ctrl Pts',(19.0849364722815,15.3169614350315,35.9194234390696));
#54859=CARTESIAN_POINT('Ctrl Pts',(19.1589062664445,15.31272988655,35.8912556118297));
#54860=CARTESIAN_POINT('Ctrl Pts',(19.2327906234526,15.3085032256239,35.8631203192082));
#54861=CARTESIAN_POINT('Ctrl Pts',(19.3081700894616,15.3042765646978,35.8386651547943));
#54862=CARTESIAN_POINT('Ctrl Pts',(19.3846436157027,15.3000499037717,35.8180431728));
#54863=CARTESIAN_POINT('Ctrl Pts',(19.4610688694711,15.2958259108457,35.7974342080434));
#54864=CARTESIAN_POINT('Ctrl Pts',(19.5385863612752,15.2916019179196,35.7806537447508));
#54865=CARTESIAN_POINT('Ctrl Pts',(19.6167789105024,15.2873779249936,35.7678053174179));
#54866=CARTESIAN_POINT('Ctrl Pts',(19.6949464480764,15.2831552832072,35.7549609999447));
#54867=CARTESIAN_POINT('Ctrl Pts',(19.7737881520378,15.2789326414207,35.7460462967408));
#54868=CARTESIAN_POINT('Ctrl Pts',(19.8528771166699,15.2747099996342,35.7411135470098));
#54869=CARTESIAN_POINT('Ctrl Pts',(19.9319654073316,15.2704873938317,35.7361808393142));
#54870=CARTESIAN_POINT('Ctrl Pts',(20.011300486522,15.2662647880292,35.7352300453764));
#54871=CARTESIAN_POINT('Ctrl Pts',(20.0904522949218,15.2620421822268,35.738261482881));
#54872=CARTESIAN_POINT('Ctrl Pts',(20.1696828096359,15.2578153775848,35.7412959347612));
#54873=CARTESIAN_POINT('Ctrl Pts',(20.2487292200167,15.2535885729428,35.7483205098561));
#54874=CARTESIAN_POINT('Ctrl Pts',(20.3271640530113,15.2493617683008,35.7592834167039));
#54875=CARTESIAN_POINT('Ctrl Pts',(20.4056368941516,15.2451329154233,35.7702516359843));
#54876=CARTESIAN_POINT('Ctrl Pts',(20.4834971065262,15.2409040625459,35.7851619005852));
#54877=CARTESIAN_POINT('Ctrl Pts',(20.5603274388273,15.2366752096684,35.8039112381711));
#54878=CARTESIAN_POINT('Ctrl Pts',(20.6372958520721,15.2324387566156,35.8226942724252));
#54879=CARTESIAN_POINT('Ctrl Pts',(20.7132302366212,15.2282023035628,35.8453300316111));
#54880=CARTESIAN_POINT('Ctrl Pts',(20.7877287571503,15.2239658505101,35.8716656790198));
#54881=CARTESIAN_POINT('Ctrl Pts',(20.8554384094741,15.220115455076,35.8956014232077));
#54882=CARTESIAN_POINT('Ctrl Pts',(20.9219619604967,15.2162650596419,35.9225927334175));
#54883=CARTESIAN_POINT('Ctrl Pts',(20.9870148297634,15.2124146642078,35.9524916375653));
#54884=CARTESIAN_POINT('Ctrl Pts',(21.0586102802312,15.2081770218304,35.9853975729234));
#54885=CARTESIAN_POINT('Ctrl Pts',(21.1286927534798,15.2039393794529,36.0219495558988));
#54886=CARTESIAN_POINT('Ctrl Pts',(21.1968662910727,15.1997017370754,36.0619858876363));
#54887=CARTESIAN_POINT('Ctrl Pts',(21.2649417924433,15.195470188594,36.1019646455575));
#54888=CARTESIAN_POINT('Ctrl Pts',(21.3311134088385,15.1912386401125,36.1454175661666));
#54889=CARTESIAN_POINT('Ctrl Pts',(21.395006873294,15.1870070916311,36.1921356797816));
#54890=CARTESIAN_POINT('Ctrl Pts',(21.4588265390337,15.182780430705,36.2387998326853));
#54891=CARTESIAN_POINT('Ctrl Pts',(21.5203729054523,15.1785537697789,36.2887214086112));
#54892=CARTESIAN_POINT('Ctrl Pts',(21.5792992752379,15.1743271088528,36.3416472935918));
#54893=CARTESIAN_POINT('Ctrl Pts',(21.6381884488626,15.1701031159268,36.3945397701045));
#54894=CARTESIAN_POINT('Ctrl Pts',(21.6944605606698,15.1658791230008,36.45043247908));
#54895=CARTESIAN_POINT('Ctrl Pts',(21.7478016726969,15.1616551300748,36.5090318187286));
#54896=CARTESIAN_POINT('Ctrl Pts',(21.8011257223643,15.1574324882883,36.5676124140547));
#54897=CARTESIAN_POINT('Ctrl Pts',(21.8515203187066,15.1532098465019,36.6288975743807));
#54898=CARTESIAN_POINT('Ctrl Pts',(21.8987091761125,15.1489872047154,36.6925576724263));
#54899=CARTESIAN_POINT('Ctrl Pts',(21.9458976313903,15.144764598913,36.7562172279812));
#54900=CARTESIAN_POINT('Ctrl Pts',(21.9898801240436,15.1405419931105,36.8222513035725));
#54901=CARTESIAN_POINT('Ctrl Pts',(22.0304222910095,15.136319387308,36.8902993093035));
#54902=CARTESIAN_POINT('Ctrl Pts',(22.0710047719568,15.1320925826661,36.9584149800422));
#54903=CARTESIAN_POINT('Ctrl Pts',(22.1081398533377,15.1278657780241,37.0285481774607));
#54904=CARTESIAN_POINT('Ctrl Pts',(22.1416382925597,15.1236389733821,37.1003121163373));
#54905=CARTESIAN_POINT('Ctrl Pts',(22.1751529645384,15.1194101205047,37.1721108307612));
#54906=CARTESIAN_POINT('Ctrl Pts',(22.2050273068634,15.1151812676272,37.2455414261018));
#54907=CARTESIAN_POINT('Ctrl Pts',(22.2311205749776,15.1109524147498,37.3201978322601));
#54908=CARTESIAN_POINT('Ctrl Pts',(22.2572607384126,15.106715961697,37.3949884123405));
#54909=CARTESIAN_POINT('Ctrl Pts',(22.2796061172186,15.1024795086443,37.4710087543335));
#54910=CARTESIAN_POINT('Ctrl Pts',(22.2980661879124,15.0982430555915,37.5478385771589));
#54911=CARTESIAN_POINT('Ctrl Pts',(22.3148440374552,15.0943926601573,37.617667085898));
#54912=CARTESIAN_POINT('Ctrl Pts',(22.3284130346181,15.0905422647231,37.6881638658518));
#54913=CARTESIAN_POINT('Ctrl Pts',(22.3387424011334,15.0866918692889,37.7590096452379));
#54914=CARTESIAN_POINT('Ctrl Pts',(22.3501106260407,15.0824542269114,37.8369806178621));
#54915=CARTESIAN_POINT('Ctrl Pts',(22.3575967325203,15.0782165845339,37.9156670762007));
#54916=CARTESIAN_POINT('Ctrl Pts',(22.3611208302554,15.0739789421564,37.9946488451231));
#54917=CARTESIAN_POINT('Ctrl Pts',(22.3646398601997,15.0697473936749,38.0735170351623));
#54918=CARTESIAN_POINT('Ctrl Pts',(22.3642081754316,15.0655158451935,38.1526792279952));
#54919=CARTESIAN_POINT('Ctrl Pts',(22.3597973470375,15.061284296712,38.2317077135734));
#54920=CARTESIAN_POINT('Ctrl Pts',(22.355391613272,15.0570576357859,38.3106449190683));
#54921=CARTESIAN_POINT('Ctrl Pts',(22.3470158953207,15.0528309748598,38.389448258535));
#54922=CARTESIAN_POINT('Ctrl Pts',(22.3346938026217,15.0486043139337,38.4676891199095));
#54923=CARTESIAN_POINT('Ctrl Pts',(22.3223794880116,15.0443803210077,38.5458805932142));
#54924=CARTESIAN_POINT('Ctrl Pts',(22.306123815899,15.0401563280817,38.6235098313147));
#54925=CARTESIAN_POINT('Ctrl Pts',(22.2860021917214,15.0359323351557,38.7001536639435));
#54926=CARTESIAN_POINT('Ctrl Pts',(22.2658870039,15.0317096933692,38.776772980311));
#54927=CARTESIAN_POINT('Ctrl Pts',(22.2419084386302,15.0274870515827,38.8524070640585));
#54928=CARTESIAN_POINT('Ctrl Pts',(22.214192617479,15.0232644097963,38.926644720301));
#54929=CARTESIAN_POINT('Ctrl Pts',(22.186477032513,15.0190418039938,39.0008817439143));
#54930=CARTESIAN_POINT('Ctrl Pts',(22.155024420285,15.0148191981913,39.0737219250184));
#54931=CARTESIAN_POINT('Ctrl Pts',(22.1200096958296,15.0105965923888,39.1447723821428));
#54932=CARTESIAN_POINT('Ctrl Pts',(22.0849601537249,15.0063697877468,39.2158934898276));
#54933=CARTESIAN_POINT('Ctrl Pts',(22.0463416318082,15.0021429831049,39.2852208972095));
#54934=CARTESIAN_POINT('Ctrl Pts',(22.0043755801985,14.9979161784629,39.3523853138727));
#54935=CARTESIAN_POINT('Ctrl Pts',(21.9623891925755,14.9936873255854,39.4195822772354));
#54936=CARTESIAN_POINT('Ctrl Pts',(21.9170523121701,14.989458472708,39.4846137768073));
#54937=CARTESIAN_POINT('Ctrl Pts',(21.8686289657637,14.9852296198305,39.5471407081584));
#54938=CARTESIAN_POINT('Ctrl Pts',(21.8201185919922,14.9809931667777,39.6097800141072));
#54939=CARTESIAN_POINT('Ctrl Pts',(21.7685109747064,14.976756713725,39.6699054013311));
#54940=CARTESIAN_POINT('Ctrl Pts',(21.714109398934,14.9725202606722,39.7272121586893));
#54941=CARTESIAN_POINT('Ctrl Pts',(21.664665305879,14.968669865238,39.7792966912284));
#54942=CARTESIAN_POINT('Ctrl Pts',(21.6129139293989,14.9648194698039,39.829053185278));
#54943=CARTESIAN_POINT('Ctrl Pts',(21.5591063425391,14.9609690743697,39.8762820309721));
#54944=CARTESIAN_POINT('Ctrl Pts',(21.4998871495476,14.9567314319922,39.9282608371432));
#54945=CARTESIAN_POINT('Ctrl Pts',(21.437954583786,14.9524937896147,39.9773725242892));
#54946=CARTESIAN_POINT('Ctrl Pts',(21.3736176294146,14.9482561472372,40.0233213587597));
#54947=CARTESIAN_POINT('Ctrl Pts',(21.3093731941084,14.9440245987557,40.0692041170032));
#54948=CARTESIAN_POINT('Ctrl Pts',(21.2427316149981,14.9397930502743,40.1119327848922));
#54949=CARTESIAN_POINT('Ctrl Pts',(21.1740362093125,14.9355615017928,40.1512506965564));
#54950=CARTESIAN_POINT('Ctrl Pts',(21.1054201487175,14.9313348408667,40.1905231949468));
#54951=CARTESIAN_POINT('Ctrl Pts',(21.0347553805461,14.9271081799406,40.2263925342439));
#54952=CARTESIAN_POINT('Ctrl Pts',(20.9624143050223,14.9228815190145,40.2586452108646));
#54953=CARTESIAN_POINT('Ctrl Pts',(20.8901188934396,14.9186575260884,40.2908775285907));
#54954=CARTESIAN_POINT('Ctrl Pts',(20.8161497018186,14.9144335331624,40.3194975246576));
#54955=CARTESIAN_POINT('Ctrl Pts',(20.7409027598398,14.9102095402364,40.3443381076304));
#54956=CARTESIAN_POINT('Ctrl Pts',(20.6656798872951,14.9059868984499,40.3691707447816));
#54957=CARTESIAN_POINT('Ctrl Pts',(20.5891805208482,14.9017642566634,40.3902262226906));
#54958=CARTESIAN_POINT('Ctrl Pts',(20.5118182510104,14.897541614877,40.4073865126659));
#54959=CARTESIAN_POINT('Ctrl Pts',(20.4344566404286,14.8933190090745,40.4245466564069));
#54960=CARTESIAN_POINT('Ctrl Pts',(20.3562325990354,14.889096403272,40.4378115780941));
#54961=CARTESIAN_POINT('Ctrl Pts',(20.27757091483,14.8848737974695,40.447114148937));
#54962=CARTESIAN_POINT('Ctrl Pts',(20.1988310116759,14.8806469928275,40.4564259699927));
#54963=CARTESIAN_POINT('Ctrl Pts',(20.1196530630481,14.8764201881855,40.461767514756));
#54964=CARTESIAN_POINT('Ctrl Pts',(20.040467397875,14.8721933835435,40.4631235326595));
#54965=CARTESIAN_POINT('Ctrl Pts',(19.9612433607161,14.867964530666,40.4644802076656));
#54966=CARTESIAN_POINT('Ctrl Pts',(19.8820120686772,14.8637356777886,40.4618475239913));
#54967=CARTESIAN_POINT('Ctrl Pts',(19.8032017046315,14.8595068249111,40.4552623785558));
#54968=CARTESIAN_POINT('Ctrl Pts',(19.7242497010912,14.8552703718583,40.4486653981708));
#54969=CARTESIAN_POINT('Ctrl Pts',(19.6457206027955,14.8510339188055,40.4381018253066));
#54970=CARTESIAN_POINT('Ctrl Pts',(19.5680351108609,14.8467974657527,40.4236602108422));
#54971=CARTESIAN_POINT('Ctrl Pts',(19.497428908052,14.8429470703187,40.4105346254289));
#54972=CARTESIAN_POINT('Ctrl Pts',(19.4275196849273,14.8390966748847,40.3942063006677));
#54973=CARTESIAN_POINT('Ctrl Pts',(19.3586115557134,14.8352462794506,40.3747771988561));
#54974=CARTESIAN_POINT('Ctrl Pts',(19.2827731091141,14.8310086370731,40.3533940483191));
#54975=CARTESIAN_POINT('Ctrl Pts',(19.2078628105288,14.8267709946956,40.3281740625552));
#54976=CARTESIAN_POINT('Ctrl Pts',(19.1342969323881,14.8225333523182,40.2992154600283));
#54977=CARTESIAN_POINT('Ctrl Pts',(19.0608368448671,14.8183018038367,40.2702985011082));
#54978=CARTESIAN_POINT('Ctrl Pts',(18.9887177709689,14.8140702553553,40.2376537725005));
#54979=CARTESIAN_POINT('Ctrl Pts',(18.9183418991389,14.8098387068738,40.2014295595479));
#54980=CARTESIAN_POINT('Ctrl Pts',(18.8480473133843,14.8056120459477,40.1652471865615));
#54981=CARTESIAN_POINT('Ctrl Pts',(18.7794923431636,14.8013853850216,40.125493758781));
#54982=CARTESIAN_POINT('Ctrl Pts',(18.7130588003859,14.7971587240956,40.0823654530979));
#54983=CARTESIAN_POINT('Ctrl Pts',(18.6466671925307,14.7929347311695,40.0392643713453));
#54984=CARTESIAN_POINT('Ctrl Pts',(18.582394746287,14.7887107382435,39.9927928947417));
#54985=CARTESIAN_POINT('Ctrl Pts',(18.5205972022698,14.7844867453175,39.9431922859453));
#54986=CARTESIAN_POINT('Ctrl Pts',(18.4588194255931,14.7802641035311,39.893607543024));
#54987=CARTESIAN_POINT('Ctrl Pts',(18.3995153443931,14.7760414617446,39.8408959487613));
#54988=CARTESIAN_POINT('Ctrl Pts',(18.3430091011241,14.7718188199582,39.7853402036214));
#54989=CARTESIAN_POINT('Ctrl Pts',(18.2865033393828,14.7675962141557,39.7297849319094));
#54990=CARTESIAN_POINT('Ctrl Pts',(18.2327957014365,14.7633736083532,39.6713858871789));
#54991=CARTESIAN_POINT('Ctrl Pts',(18.1821737266528,14.7591510025508,39.6104628697286));
#54992=CARTESIAN_POINT('Ctrl Pts',(18.1315014148125,14.7549241979088,39.5494792721569));
#54993=CARTESIAN_POINT('Ctrl Pts',(18.0839211953534,14.7506973932668,39.4859670499826));
#54994=CARTESIAN_POINT('Ctrl Pts',(18.0396801048077,14.7464705886248,39.4202788907702));
#54995=CARTESIAN_POINT('Ctrl Pts',(17.9954175758047,14.7422417357474,39.3545589002268));
#54996=CARTESIAN_POINT('Ctrl Pts',(17.9544976414061,14.73801288287,39.2866612741251));
#54997=CARTESIAN_POINT('Ctrl Pts',(17.9171224251338,14.7337840299925,39.2169652855034));
#54998=CARTESIAN_POINT('Ctrl Pts',(17.8796800374076,14.7295475769398,39.1471440379171));
#54999=CARTESIAN_POINT('Ctrl Pts',(17.8457952978973,14.725311123887,39.0755183946107));
#55000=CARTESIAN_POINT('Ctrl Pts',(17.815622926706,14.7210746708342,39.0024894695051));
#55001=CARTESIAN_POINT('Ctrl Pts',(17.788200090001,14.7172242754,38.9361154919606));
#55002=CARTESIAN_POINT('Ctrl Pts',(17.7638433183341,14.7133738799658,38.8685828232599));
#55003=CARTESIAN_POINT('Ctrl Pts',(17.7426326190174,14.7095234845316,38.8002020766719));
#55004=CARTESIAN_POINT('Ctrl Pts',(17.7143095978416,14.7043819835471,38.7088920588025));
#55005=CARTESIAN_POINT('Ctrl Pts',(17.691509480421,14.6992404825626,38.6157933314888));
#55006=CARTESIAN_POINT('Ctrl Pts',(17.6744210927045,14.6940989815781,38.5215129735158));
#55007=CARTESIAN_POINT('Ctrl Pts',(17.6575525340282,14.6890236220721,38.4284454602508));
#55008=CARTESIAN_POINT('Ctrl Pts',(17.6462497389265,14.683948262566,38.3342265316659));
#55009=CARTESIAN_POINT('Ctrl Pts',(17.6406481563961,14.6788729030599,38.2394608152235));
#55010=CARTESIAN_POINT('Ctrl Pts',(17.6379455876605,14.6764242186304,38.1937396531996));
#55011=CARTESIAN_POINT('Ctrl Pts',(17.6365694097498,14.6739755342008,38.1478915231381));
#55012=CARTESIAN_POINT('Ctrl Pts',(17.6365308344677,14.6715268497713,38.1019860710541));
#55013=CARTESIAN_POINT('',(17.6365303963904,13.8777768497283,38.0986311634849));
#55014=CARTESIAN_POINT('Ctrl Pts',(17.6365308344671,14.6715268497283,38.1019860702482));
#55015=CARTESIAN_POINT('Ctrl Pts',(17.6364646605814,14.6673262575168,38.0232376279563));
#55016=CARTESIAN_POINT('Ctrl Pts',(17.6403385060611,14.6631256653054,37.9444216968236));
#55017=CARTESIAN_POINT('Ctrl Pts',(17.6481459042837,14.6589250730939,37.8659642049545));
#55018=CARTESIAN_POINT('Ctrl Pts',(17.6559505594527,14.6547259567198,37.7875342783647));
#55019=CARTESIAN_POINT('Ctrl Pts',(17.6676859771048,14.6505268403457,37.7094630126979));
#55020=CARTESIAN_POINT('Ctrl Pts',(17.683293711496,14.6463277239716,37.632172666782));
#55021=CARTESIAN_POINT('Ctrl Pts',(17.6989009574053,14.642128739019,37.5548847398548));
#55022=CARTESIAN_POINT('Ctrl Pts',(17.7183801840557,14.6379297540664,37.4783781488536));
#55023=CARTESIAN_POINT('Ctrl Pts',(17.7416218588689,14.6337307691138,37.4030648433597));
#55024=CARTESIAN_POINT('Ctrl Pts',(17.7648867551708,14.6295275888232,37.3276762899725));
#55025=CARTESIAN_POINT('Ctrl Pts',(17.7919214685464,14.6253244085327,37.25348385805));
#55026=CARTESIAN_POINT('Ctrl Pts',(17.8225667841824,14.6211212282421,37.180883559306));
#55027=CARTESIAN_POINT('Ctrl Pts',(17.8532267747405,14.616916035202,37.1082484949309));
#55028=CARTESIAN_POINT('Ctrl Pts',(17.8875006042114,14.6127108421619,37.0372075097695));
#55029=CARTESIAN_POINT('Ctrl Pts',(17.9251822807059,14.6085056491219,36.9681334563637));
#55030=CARTESIAN_POINT('Ctrl Pts',(17.962933700464,14.6042926728854,36.8989315570028));
#55031=CARTESIAN_POINT('Ctrl Pts',(18.0041053208906,14.600079696649,36.8317042684717));
#55032=CARTESIAN_POINT('Ctrl Pts',(18.0484470026627,14.5958667204126,36.7667965873567));
#55033=CARTESIAN_POINT('Ctrl Pts',(18.0907787627588,14.5918447101459,36.7048310444285));
#55034=CARTESIAN_POINT('Ctrl Pts',(18.135999166347,14.5878226998792,36.6449796362851));
#55035=CARTESIAN_POINT('Ctrl Pts',(18.1838579015468,14.5838006896125,36.5875125391838));
#55036=CARTESIAN_POINT('Ctrl Pts',(18.2342824880017,14.579563047235,36.5269644575433));
#55037=CARTESIAN_POINT('Ctrl Pts',(18.2878329422262,14.5753254048575,36.4688271255746));
#55038=CARTESIAN_POINT('Ctrl Pts',(18.344249977709,14.57108776248,36.4134406904638));
#55039=CARTESIAN_POINT('Ctrl Pts',(18.4005858832808,14.5668562139985,36.3581339032201));
#55040=CARTESIAN_POINT('Ctrl Pts',(18.4597798519412,14.5626246655171,36.3055704824781));
#55041=CARTESIAN_POINT('Ctrl Pts',(18.5215326113407,14.5583931170356,36.256057316083));
#55042=CARTESIAN_POINT('Ctrl Pts',(18.5832140445977,14.5541664561095,36.2066013387624));
#55043=CARTESIAN_POINT('Ctrl Pts',(18.6474480314449,14.5499397951834,36.1601889062038));
#55044=CARTESIAN_POINT('Ctrl Pts',(18.7138998638877,14.5457131342573,36.1170887864577));
#55045=CARTESIAN_POINT('Ctrl Pts',(18.780309749863,14.5414891413313,36.0740158728503));
#55046=CARTESIAN_POINT('Ctrl Pts',(18.8489343103774,14.5372651484053,36.0342513763981));
#55047=CARTESIAN_POINT('Ctrl Pts',(18.9194082842053,14.5330411554793,35.998021887684));
#55048=CARTESIAN_POINT('Ctrl Pts',(18.9898597153405,14.5288185136928,35.9618039877903));
#55049=CARTESIAN_POINT('Ctrl Pts',(19.0621589684265,14.5245958719063,35.9291190643558));
#55050=CARTESIAN_POINT('Ctrl Pts',(19.1359158121418,14.5203732301199,35.9001479692503));
#55051=CARTESIAN_POINT('Ctrl Pts',(19.2096720273254,14.5161506243174,35.8711771210271));
#55052=CARTESIAN_POINT('Ctrl Pts',(19.2848853715982,14.5119280185149,35.8459202082597));
#55053=CARTESIAN_POINT('Ctrl Pts',(19.3611466441945,14.5077054127125,35.8245095406317));
#55054=CARTESIAN_POINT('Ctrl Pts',(19.4374837488383,14.5034786080705,35.8030775828429));
#55055=CARTESIAN_POINT('Ctrl Pts',(19.514870410893,14.4992518034285,35.785499636849));
#55056=CARTESIAN_POINT('Ctrl Pts',(19.5928838960292,14.4950249987865,35.771857624889));
#55057=CARTESIAN_POINT('Ctrl Pts',(19.6709351851333,14.4907961459091,35.758209002249));
#55058=CARTESIAN_POINT('Ctrl Pts',(19.7496134365798,14.4865672930316,35.7485001706613));
#55059=CARTESIAN_POINT('Ctrl Pts',(19.8284899342873,14.4823384401542,35.7427612046593));
#55060=CARTESIAN_POINT('Ctrl Pts',(19.9075081903462,14.4781019871014,35.7370119244778));
#55061=CARTESIAN_POINT('Ctrl Pts',(19.9867249348031,14.4738655340486,35.7352467762091));
#55062=CARTESIAN_POINT('Ctrl Pts',(20.0657108174142,14.4696290809959,35.7374436452489));
#55063=CARTESIAN_POINT('Ctrl Pts',(20.1374989094757,14.4657786855617,35.7394403189792));
#55064=CARTESIAN_POINT('Ctrl Pts',(20.2090960695186,14.4619282901276,35.7447091273303));
#55065=CARTESIAN_POINT('Ctrl Pts',(20.2801860349142,14.4580778946935,35.7531965939306));
#55066=CARTESIAN_POINT('Ctrl Pts',(20.3584257521403,14.453840252316,35.7625376729855));
#55067=CARTESIAN_POINT('Ctrl Pts',(20.4363446904957,14.4496026099385,35.7758131978984));
#55068=CARTESIAN_POINT('Ctrl Pts',(20.5135163726699,14.445364967561,35.792990815818));
#55069=CARTESIAN_POINT('Ctrl Pts',(20.5905770789364,14.4411334190795,35.8101437316489));
#55070=CARTESIAN_POINT('Ctrl Pts',(20.6668922092512,14.436901870598,35.8311874958296));
#55071=CARTESIAN_POINT('Ctrl Pts',(20.7420414207746,14.4326703221166,35.8560381084442));
#55072=CARTESIAN_POINT('Ctrl Pts',(20.8171038328835,14.4284436611905,35.880860017915));
#55073=CARTESIAN_POINT('Ctrl Pts',(20.8910025595526,14.4242170002644,35.9094798914121));
#55074=CARTESIAN_POINT('Ctrl Pts',(20.9633299465217,14.4199903393382,35.9417632532471));
#55075=CARTESIAN_POINT('Ctrl Pts',(21.0356116781902,14.4157663464122,35.974026236818));
#55076=CARTESIAN_POINT('Ctrl Pts',(21.1063236119807,14.4115423534862,36.0099479280856));
#55077=CARTESIAN_POINT('Ctrl Pts',(21.1750768437342,14.4073183605602,36.0493452625516));
#55078=CARTESIAN_POINT('Ctrl Pts',(21.2438080832135,14.4030957187737,36.0887299948902));
#55079=CARTESIAN_POINT('Ctrl Pts',(21.3105814583948,14.3988730769872,36.1315879297875));
#55080=CARTESIAN_POINT('Ctrl Pts',(21.3750328417326,14.3946504352008,36.1776901589346));
#55081=CARTESIAN_POINT('Ctrl Pts',(21.4394836758367,14.3904278293983,36.2237919952136));
#55082=CARTESIAN_POINT('Ctrl Pts',(21.5016121769995,14.3862052235958,36.2731377968842));
#55083=CARTESIAN_POINT('Ctrl Pts',(21.5610846124,14.3819826177933,36.3254563195492));
#55084=CARTESIAN_POINT('Ctrl Pts',(21.6206161855042,14.3777558131513,36.3778268662698));
#55085=CARTESIAN_POINT('Ctrl Pts',(21.6774860644205,14.3735290085093,36.43317572824));
#55086=CARTESIAN_POINT('Ctrl Pts',(21.7313954179226,14.3693022038673,36.4911928805178));
#55087=CARTESIAN_POINT('Ctrl Pts',(21.7853308949528,14.3650733509898,36.549238146891));
#55088=CARTESIAN_POINT('Ctrl Pts',(21.8363026868455,14.3608444981124,36.6099539199054));
#55089=CARTESIAN_POINT('Ctrl Pts',(21.884052199654,14.3566156452349,36.6729969341732));
#55090=CARTESIAN_POINT('Ctrl Pts',(21.9318875288007,14.3523791921821,36.7361532505528));
#55091=CARTESIAN_POINT('Ctrl Pts',(21.9764887431074,14.3481427391293,36.8016447769754));
#55092=CARTESIAN_POINT('Ctrl Pts',(22.0176406832059,14.3439062860765,36.8690993076725));
#55093=CARTESIAN_POINT('Ctrl Pts',(22.0550425475214,14.3400558906425,36.9304068717522));
#55094=CARTESIAN_POINT('Ctrl Pts',(22.0895955930787,14.3362054952084,36.9933354082853));
#55095=CARTESIAN_POINT('Ctrl Pts',(22.1211725264869,14.3323550997743,37.0575905057143));
#55096=CARTESIAN_POINT('Ctrl Pts',(22.1559252560319,14.3281174573968,37.1283079498045));
#55097=CARTESIAN_POINT('Ctrl Pts',(22.1872028951335,14.3238798150193,37.2008979615713));
#55098=CARTESIAN_POINT('Ctrl Pts',(22.214800436797,14.3196421726418,37.2749851722157));
#55099=CARTESIAN_POINT('Ctrl Pts',(22.2423582921125,14.3154106241604,37.3489658425438));
#55100=CARTESIAN_POINT('Ctrl Pts',(22.2662463973767,14.3111790756789,37.4244390003731));
#55101=CARTESIAN_POINT('Ctrl Pts',(22.2863064098537,14.3069475271975,37.501006309581));
#55102=CARTESIAN_POINT('Ctrl Pts',(22.3063432524623,14.3027208662714,37.5774851814321));
#55103=CARTESIAN_POINT('Ctrl Pts',(22.3225606708177,14.2984942053453,37.6550552420493));
#55104=CARTESIAN_POINT('Ctrl Pts',(22.3348495715185,14.2942675444192,37.7333013235912));
#55105=CARTESIAN_POINT('Ctrl Pts',(22.3471307150821,14.2900435514932,37.811498013768));
#55106=CARTESIAN_POINT('Ctrl Pts',(22.3554881905846,14.2858195585672,37.8903694159813));
#55107=CARTESIAN_POINT('Ctrl Pts',(22.3598638705481,14.2815955656412,37.9694896426265));
#55108=CARTESIAN_POINT('Ctrl Pts',(22.3642381508515,14.2773729238547,38.04858456088));
#55109=CARTESIAN_POINT('Ctrl Pts',(22.3646331390006,14.2731502820683,38.1279276777905));
#55110=CARTESIAN_POINT('Ctrl Pts',(22.3610426511955,14.2689276402818,38.2070889356365));
#55111=CARTESIAN_POINT('Ctrl Pts',(22.3574521939874,14.2647050344794,38.2862495188959));
#55112=CARTESIAN_POINT('Ctrl Pts',(22.3498763510219,14.2604824286769,38.3652277779459));
#55113=CARTESIAN_POINT('Ctrl Pts',(22.3383609978002,14.2562598228744,38.4435961071766));
#55114=CARTESIAN_POINT('Ctrl Pts',(22.3268341940376,14.2520330182324,38.5220423636523));
#55115=CARTESIAN_POINT('Ctrl Pts',(22.3113601234275,14.2478062135905,38.5998770139571));
#55116=CARTESIAN_POINT('Ctrl Pts',(22.2920361913906,14.2435794089485,38.6766806206694));
#55117=CARTESIAN_POINT('Ctrl Pts',(22.2727028953148,14.239350556071,38.7535214450639));
#55118=CARTESIAN_POINT('Ctrl Pts',(22.2495161586525,14.2351217031936,38.8293297817057));
#55119=CARTESIAN_POINT('Ctrl Pts',(22.2226231737379,14.2308928503162,38.9037018529674));
#55120=CARTESIAN_POINT('Ctrl Pts',(22.1956818562362,14.2266563972634,38.9782075871389));
#55121=CARTESIAN_POINT('Ctrl Pts',(22.1650211631008,14.2224199442106,39.0512714649937));
#55122=CARTESIAN_POINT('Ctrl Pts',(22.1308362067978,14.2181834911578,39.1225103914873));
#55123=CARTESIAN_POINT('Ctrl Pts',(22.0997664420612,14.2143330957237,39.1872574886205));
#55124=CARTESIAN_POINT('Ctrl Pts',(22.0657861828018,14.2104827002895,39.2504971569346));
#55125=CARTESIAN_POINT('Ctrl Pts',(22.0290731110171,14.2066323048553,39.311962355458));
#55126=CARTESIAN_POINT('Ctrl Pts',(21.9886676847534,14.2023946624778,39.379609311324));
#55127=CARTESIAN_POINT('Ctrl Pts',(21.9447998069588,14.1981570201003,39.4453604315721));
#55128=CARTESIAN_POINT('Ctrl Pts',(21.8976727697612,14.1939193777228,39.5088394159048));
#55129=CARTESIAN_POINT('Ctrl Pts',(21.8506135030923,14.1896878292413,39.5722271149671));
#55130=CARTESIAN_POINT('Ctrl Pts',(21.8003046616916,14.1854562807599,39.6333487936316));
#55131=CARTESIAN_POINT('Ctrl Pts',(21.7469942052441,14.1812247322784,39.6918547948049));
#55132=CARTESIAN_POINT('Ctrl Pts',(21.6937453238462,14.1769980713523,39.7502932199311));
#55133=CARTESIAN_POINT('Ctrl Pts',(21.6375020312322,14.1727714104262,39.8061216266631));
#55134=CARTESIAN_POINT('Ctrl Pts',(21.5785532148333,14.1685447495001,39.859022509475));
#55135=CARTESIAN_POINT('Ctrl Pts',(21.5196416087641,14.1643207565741,39.9118899996011));
#55136=CARTESIAN_POINT('Ctrl Pts',(21.4580282167,14.1600967636481,39.9618333214996));
#55137=CARTESIAN_POINT('Ctrl Pts',(21.3940386610968,14.155872770722,40.0085718881581));
#55138=CARTESIAN_POINT('Ctrl Pts',(21.3300695739986,14.1516501289356,40.0552955044302));
#55139=CARTESIAN_POINT('Ctrl Pts',(21.2637262109849,14.1474274871491,40.098816124839));
#55140=CARTESIAN_POINT('Ctrl Pts',(21.1953659674773,14.1432048453627,40.1388944662972));
#55141=CARTESIAN_POINT('Ctrl Pts',(21.1270063065133,14.1389822395602,40.1789724662208));
#55142=CARTESIAN_POINT('Ctrl Pts',(21.0566302043478,14.1347596337577,40.215608009662));
#55143=CARTESIAN_POINT('Ctrl Pts',(20.9846213371323,14.1305370279552,40.2486068191653));
#55144=CARTESIAN_POINT('Ctrl Pts',(20.9125408663408,14.1263102233132,40.2816384417492));
#55145=CARTESIAN_POINT('Ctrl Pts',(20.8388248145482,14.1220834186712,40.3110259111443));
#55146=CARTESIAN_POINT('Ctrl Pts',(20.7638780554441,14.1178566140293,40.3366226229096));
#55147=CARTESIAN_POINT('Ctrl Pts',(20.6888949784536,14.1136277611518,40.3622317383929));
#55148=CARTESIAN_POINT('Ctrl Pts',(20.6126804573469,14.1093989082743,40.3840463076975));
#55149=CARTESIAN_POINT('Ctrl Pts',(20.5356533301059,14.1051700553969,40.4019700151928));
#55150=CARTESIAN_POINT('Ctrl Pts',(20.4584877682375,14.1009336023441,40.4199259355182));
#55151=CARTESIAN_POINT('Ctrl Pts',(20.3805071445901,14.0966971492913,40.4339769385539));
#55152=CARTESIAN_POINT('Ctrl Pts',(20.3021390318273,14.0924606962386,40.4440781655795));
#55153=CARTESIAN_POINT('Ctrl Pts',(20.2309124137566,14.0886103008044,40.4532588924598));
#55154=CARTESIAN_POINT('Ctrl Pts',(20.1593660432827,14.0847599053703,40.4591775527539));
#55155=CARTESIAN_POINT('Ctrl Pts',(20.0878206510454,14.0809095099361,40.4618378382416));
#55156=CARTESIAN_POINT('Ctrl Pts',(20.0090797032014,14.0766718675586,40.4647656773979));
#55157=CARTESIAN_POINT('Ctrl Pts',(19.9300443750174,14.0724342251811,40.4637570075032));
#55158=CARTESIAN_POINT('Ctrl Pts',(19.8511409917448,14.0681965828037,40.458777530112));
#55159=CARTESIAN_POINT('Ctrl Pts',(19.7723510746336,14.0639650343222,40.4538052134047));
#55160=CARTESIAN_POINT('Ctrl Pts',(19.6936931896012,14.0597334858407,40.4448734583647));
#55161=CARTESIAN_POINT('Ctrl Pts',(19.6155956259171,14.0555019373593,40.4319999395553));
#55162=CARTESIAN_POINT('Ctrl Pts',(19.5375882670758,14.0512752764332,40.4191412900157));
#55163=CARTESIAN_POINT('Ctrl Pts',(19.4601404036507,14.047048615507,40.4023500002143));
#55164=CARTESIAN_POINT('Ctrl Pts',(19.3836756324295,14.0428219545809,40.3816955789147));
#55165=CARTESIAN_POINT('Ctrl Pts',(19.3072591281547,14.0385979616549,40.3610541953295));
#55166=CARTESIAN_POINT('Ctrl Pts',(19.231824935714,14.0343739687289,40.3365546423794));
#55167=CARTESIAN_POINT('Ctrl Pts',(19.1577856783303,14.0301499758029,40.3083173407086));
#55168=CARTESIAN_POINT('Ctrl Pts',(19.0837701040756,14.0259273340164,40.2800890713767));
#55169=CARTESIAN_POINT('Ctrl Pts',(19.0111490164942,14.0217046922299,40.2481255944814));
#55170=CARTESIAN_POINT('Ctrl Pts',(18.9403176854388,14.0174820504435,40.2125964671717));
#55171=CARTESIAN_POINT('Ctrl Pts',(18.8694869579849,14.013259444641,40.1770676426296));
#55172=CARTESIAN_POINT('Ctrl Pts',(18.8004463751051,14.0090368388385,40.1379734395443));
#55173=CARTESIAN_POINT('Ctrl Pts',(18.7335677584216,14.004814233036,40.0955299592817));
#55174=CARTESIAN_POINT('Ctrl Pts',(18.6666226395377,14.000587428394,40.0530442744256));
#55175=CARTESIAN_POINT('Ctrl Pts',(18.6018441777969,13.996360623752,40.0072029116203));
#55176=CARTESIAN_POINT('Ctrl Pts',(18.5395757420476,13.99213381911,39.9582657042749));
#55177=CARTESIAN_POINT('Ctrl Pts',(18.4772771321055,13.9879049662326,39.9093047828163));
#55178=CARTESIAN_POINT('Ctrl Pts',(18.4174913251768,13.9836761133551,39.8572453364943));
#55179=CARTESIAN_POINT('Ctrl Pts',(18.3605271057175,13.9794472604777,39.8023862868964));
#55180=CARTESIAN_POINT('Ctrl Pts',(18.3034605090727,13.9752108074249,39.7474286435647));
#55181=CARTESIAN_POINT('Ctrl Pts',(18.2492259538894,13.9709743543721,39.689661686099));
#55182=CARTESIAN_POINT('Ctrl Pts',(18.1980938136872,13.9667379013193,39.629419673153));
#55183=CARTESIAN_POINT('Ctrl Pts',(18.1516212205255,13.9628875058852,39.574667367699));
#55184=CARTESIAN_POINT('Ctrl Pts',(18.1077110166983,13.9590371104512,39.5178711735712));
#55185=CARTESIAN_POINT('Ctrl Pts',(18.0665346903742,13.9551867150171,39.4593021508751));
#55186=CARTESIAN_POINT('Ctrl Pts',(18.0207442084218,13.9509048502085,39.3941699738172));
#55187=CARTESIAN_POINT('Ctrl Pts',(17.9781648846182,13.9466229853999,39.326602749622));
#55188=CARTESIAN_POINT('Ctrl Pts',(17.9390618242376,13.9423411205913,39.2569460992567));
#55189=CARTESIAN_POINT('Ctrl Pts',(17.9000177586572,13.9380657158335,39.1873945399028));
#55190=CARTESIAN_POINT('Ctrl Pts',(17.864439760251,13.9337903110758,39.1157602097527));
#55191=CARTESIAN_POINT('Ctrl Pts',(17.8325504845345,13.929514906318,39.0424187173484));
#55192=CARTESIAN_POINT('Ctrl Pts',(17.8003919474075,13.9252034016022,38.968457956138));
#55193=CARTESIAN_POINT('Ctrl Pts',(17.7719850048456,13.9208918968864,38.8927614434773));
#55194=CARTESIAN_POINT('Ctrl Pts',(17.7475113669798,13.9165803921706,38.8157411536406));
#55195=CARTESIAN_POINT('Ctrl Pts',(17.7232972902773,13.9123146141745,38.7395377213607));
#55196=CARTESIAN_POINT('Ctrl Pts',(17.7029336313327,13.9080488361785,38.662038900109));
#55197=CARTESIAN_POINT('Ctrl Pts',(17.6865480274974,13.9037830581824,38.5836635316247));
#55198=CARTESIAN_POINT('Ctrl Pts',(17.6698989570979,13.8994486901067,38.5040279539194));
#55199=CARTESIAN_POINT('Ctrl Pts',(17.6573571699985,13.895114322031,38.4234878417123));
#55200=CARTESIAN_POINT('Ctrl Pts',(17.6490032228322,13.8907799539554,38.3424965868764));
#55201=CARTESIAN_POINT('Ctrl Pts',(17.6406492756659,13.8864455858797,38.2615053320404));
#55202=CARTESIAN_POINT('Ctrl Pts',(17.6364832337555,13.882111217804,38.1800634256563));
#55203=CARTESIAN_POINT('Ctrl Pts',(17.6365303963904,13.8777768497283,38.0986311634849));
#55204=CARTESIAN_POINT('',(17.6331851034168,13.0840268497283,38.0990226178629));
#55205=CARTESIAN_POINT('Ctrl Pts',(17.6395267864659,13.8777759447365,38.0986159178374));
#55206=CARTESIAN_POINT('Ctrl Pts',(17.637928747162,13.8616719365237,37.7964432487494));
#55207=CARTESIAN_POINT('Ctrl Pts',(17.8318962804384,13.8036603300046,36.7099019745982));
#55208=CARTESIAN_POINT('Ctrl Pts',(19.4641824064282,13.7037411251789,35.3606306468454));
#55209=CARTESIAN_POINT('Ctrl Pts',(22.0063036074145,13.5780183302599,36.1593839170346));
#55210=CARTESIAN_POINT('Ctrl Pts',(22.7200222714505,13.4522955353407,38.7266767822465));
#55211=CARTESIAN_POINT('Ctrl Pts',(20.9549059260135,13.3265727404216,40.7228609606787));
#55212=CARTESIAN_POINT('Ctrl Pts',(18.3817401264292,13.2038165118843,40.3380553789342));
#55213=CARTESIAN_POINT('Ctrl Pts',(17.6369894458825,13.1229678816531,38.8246886382043));
#55214=CARTESIAN_POINT('Ctrl Pts',(17.6331851034168,13.0840268497283,38.0990226178629));
#55215=CARTESIAN_POINT('',(17.6367489926442,12.2902768497283,38.1021344623069));
#55216=CARTESIAN_POINT('Ctrl Pts',(17.6331851034168,13.0840268497283,38.0990226178629));
#55217=CARTESIAN_POINT('Ctrl Pts',(17.6328952848397,13.0810602833467,38.0437406616896));
#55218=CARTESIAN_POINT('Ctrl Pts',(17.6596679510084,13.0361861186589,37.2077962582566));
#55219=CARTESIAN_POINT('Ctrl Pts',(18.6491954913026,12.9494043556642,35.657343223885));
#55220=CARTESIAN_POINT('Ctrl Pts',(21.3137747086376,12.8236815607454,35.6372290074956));
#55221=CARTESIAN_POINT('Ctrl Pts',(22.7810730152558,12.6979587658264,37.8615092655836));
#55222=CARTESIAN_POINT('Ctrl Pts',(21.713899002855,12.5722359709072,40.3031330315278));
#55223=CARTESIAN_POINT('Ctrl Pts',(19.0847992314011,12.4465131759882,40.7369779103628));
#55224=CARTESIAN_POINT('Ctrl Pts',(17.742876170108,12.3525268022618,39.2647846658353));
#55225=CARTESIAN_POINT('Ctrl Pts',(17.6350286938508,12.3004480268419,38.2924174207486));
#55226=CARTESIAN_POINT('Ctrl Pts',(17.6367489926442,12.2902768497283,38.1021344623069));
#55227=CARTESIAN_POINT('',(17.640153963339,11.4965268497283,38.0992943844365));
#55228=CARTESIAN_POINT('Ctrl Pts',(17.6367489926442,12.2902768497283,38.1021344623069));
#55229=CARTESIAN_POINT('Ctrl Pts',(17.6421167221093,12.2585404285355,37.5084076942567));
#55230=CARTESIAN_POINT('Ctrl Pts',(18.1692910103586,12.1848964090363,36.1221756123481));
#55231=CARTESIAN_POINT('Ctrl Pts',(20.4944013127005,12.0693447912309,35.3528537919161));
#55232=CARTESIAN_POINT('Ctrl Pts',(22.5736121140596,11.9436219963119,37.0193679474702));
#55233=CARTESIAN_POINT('Ctrl Pts',(22.307415719276,11.8178992013927,39.6706933644183));
#55234=CARTESIAN_POINT('Ctrl Pts',(19.9384046062531,11.6921764064736,40.8906004647851));
#55235=CARTESIAN_POINT('Ctrl Pts',(17.9676804027266,11.5850522892521,39.7631059729174));
#55236=CARTESIAN_POINT('Ctrl Pts',(17.641330657499,11.5198357703371,38.5369497808051));
#55237=CARTESIAN_POINT('Ctrl Pts',(17.640153963339,11.4965268497283,38.0992943844365));
#55238=CARTESIAN_POINT('',(17.6341963774677,10.7027768497283,38.0983734632106));
#55239=CARTESIAN_POINT('Ctrl Pts',(17.640153963339,11.4965268497283,38.0992943844365));
#55240=CARTESIAN_POINT('Ctrl Pts',(17.6392150543351,11.4779281720307,37.7500799443385));
#55241=CARTESIAN_POINT('Ctrl Pts',(17.8753171992425,11.4174218960267,36.615203052934));
#55242=CARTESIAN_POINT('Ctrl Pts',(19.6272936397288,11.3150080217165,35.3337145997561));
#55243=CARTESIAN_POINT('Ctrl Pts',(22.1176698466579,11.1892852267973,36.2815612830932));
#55244=CARTESIAN_POINT('Ctrl Pts',(22.6781522400348,11.0635624318782,38.8866037921257));
#55245=CARTESIAN_POINT('Ctrl Pts',(20.797956995228,10.9378396369591,40.7747915022213));
#55246=CARTESIAN_POINT('Ctrl Pts',(18.3038161317269,10.8175777762425,40.2492294011243));
#55247=CARTESIAN_POINT('Ctrl Pts',(17.6395514888341,10.7392235138322,38.7783215464619));
#55248=CARTESIAN_POINT('Ctrl Pts',(17.6341963774677,10.7027768497283,38.0983734632106));
#55249=CARTESIAN_POINT('',(17.6353503215415,9.9090268497283,38.1019939141643));
#55250=CARTESIAN_POINT('Ctrl Pts',(17.6341963774677,10.7027768497283,38.0983734632106));
#55251=CARTESIAN_POINT('Ctrl Pts',(17.6333940019544,10.6973159155259,37.9964944069241));
#55252=CARTESIAN_POINT('Ctrl Pts',(17.6855609843329,10.6499473830165,37.1136154527935));
#55253=CARTESIAN_POINT('Ctrl Pts',(18.7961706379081,10.5606712522025,35.581659313446));
#55254=CARTESIAN_POINT('Ctrl Pts',(21.4572672824637,10.4349484572826,35.7193242526437));
#55255=CARTESIAN_POINT('Ctrl Pts',(22.7903140813097,10.3092256623639,38.0265678937093));
#55256=CARTESIAN_POINT('Ctrl Pts',(21.5804669102173,10.1835028674447,40.400732338256));
#55257=CARTESIAN_POINT('Ctrl Pts',(18.9302945074246,10.0577800725256,40.6781728230947));
#55258=CARTESIAN_POINT('Ctrl Pts',(17.711117980681,9.96628806662015,39.1702307552347));
#55259=CARTESIAN_POINT('Ctrl Pts',(17.6340610761295,9.91670365902104,38.2453939776618));
#55260=CARTESIAN_POINT('Ctrl Pts',(17.6353503215415,9.9090268497283,38.1019939141643));
#55261=CARTESIAN_POINT('',(17.6403527334675,9.11527684972829,38.100042490769));
#55262=CARTESIAN_POINT('Ctrl Pts',(17.6353503215415,9.9090268497283,38.1019939141643));
#55263=CARTESIAN_POINT('Ctrl Pts',(17.6410990494308,9.87479606071468,37.4625749666653));
#55264=CARTESIAN_POINT('Ctrl Pts',(18.238503270141,9.79865767339471,36.0308725437426));
#55265=CARTESIAN_POINT('Ctrl Pts',(20.6561660623633,9.68061168776838,35.3869406484207));
#55266=CARTESIAN_POINT('Ctrl Pts',(22.6330720558258,9.55488889284928,37.1736218399495));
#55267=CARTESIAN_POINT('Ctrl Pts',(22.2103832875294,9.42916609793023,39.8045382567722));
#55268=CARTESIAN_POINT('Ctrl Pts',(19.7733082640224,9.30344330301114,40.8820596333343));
#55269=CARTESIAN_POINT('Ctrl Pts',(17.9170417702093,9.1988135536105,39.6687992359617));
#55270=CARTESIAN_POINT('Ctrl Pts',(17.6402897602495,9.13609140251621,38.4909451107544));
#55271=CARTESIAN_POINT('Ctrl Pts',(17.6403527334675,9.11527684972829,38.100042490769));
#55272=CARTESIAN_POINT('',(17.6355044646775,8.3215268497283,38.0979757353713));
#55273=CARTESIAN_POINT('Ctrl Pts',(17.6403527334675,9.11527684972829,38.100042490769));
#55274=CARTESIAN_POINT('Ctrl Pts',(17.640416549249,9.09418380420986,37.7039097061427));
#55275=CARTESIAN_POINT('Ctrl Pts',(17.9225004294726,9.03118316038505,36.5206561174594));
#55276=CARTESIAN_POINT('Ctrl Pts',(19.7917122341746,8.9262749182539,35.316501993319));
#55277=CARTESIAN_POINT('Ctrl Pts',(22.2216078271693,8.80055212333482,36.4101172795579));
#55278=CARTESIAN_POINT('Ctrl Pts',(22.6268879171577,8.67482932841574,39.0437715916894));
#55279=CARTESIAN_POINT('Ctrl Pts',(20.6382090299156,8.54910653349668,40.8173395409341));
#55280=CARTESIAN_POINT('Ctrl Pts',(18.2305512719002,8.43133904060083,40.1589894803223));
#55281=CARTESIAN_POINT('Ctrl Pts',(17.641248927774,8.35547914601139,38.7322993073621));
#55282=CARTESIAN_POINT('Ctrl Pts',(17.6355044646775,8.3215268497283,38.0979757353713));
#55283=CARTESIAN_POINT('',(17.6340647533427,7.52777684972829,38.1015653822901));
#55284=CARTESIAN_POINT('Ctrl Pts',(17.6355044646775,8.3215268497283,38.0979757353713));
#55285=CARTESIAN_POINT('Ctrl Pts',(17.6341584897687,8.31357154770503,37.9493485098786));
#55286=CARTESIAN_POINT('Ctrl Pts',(17.7145046251406,8.26370864737542,37.0192206278211));
#55287=CARTESIAN_POINT('Ctrl Pts',(18.9473685182804,8.17193814873941,35.5148091153107));
#55288=CARTESIAN_POINT('Ctrl Pts',(21.5956481253796,8.04621535382035,35.8097703157627));
#55289=CARTESIAN_POINT('Ctrl Pts',(22.789767420079,7.92049255890126,38.1918841033843));
#55290=CARTESIAN_POINT('Ctrl Pts',(21.4414909330391,7.79476976398219,40.4902612485993));
#55291=CARTESIAN_POINT('Ctrl Pts',(18.7795420440647,7.6690469690631,40.6103241472732));
#55292=CARTESIAN_POINT('Ctrl Pts',(17.6825210085457,7.58004933097848,39.07585822244));
#55293=CARTESIAN_POINT('Ctrl Pts',(17.6333245476966,7.53295929120021,38.1982348102183));
#55294=CARTESIAN_POINT('Ctrl Pts',(17.6340647533427,7.52777684972829,38.1015653822901));
#55295=CARTESIAN_POINT('',(17.6367873258724,6.73402689228867,38.100787309117));
#55296=CARTESIAN_POINT('Ctrl Pts',(17.6340647533427,7.52777684972829,38.1015653822901));
#55297=CARTESIAN_POINT('Ctrl Pts',(17.6393101899942,7.49105169289384,37.4165214853157));
#55298=CARTESIAN_POINT('Ctrl Pts',(18.3122833940378,7.41241893775303,35.9407788034475));
#55299=CARTESIAN_POINT('Ctrl Pts',(20.8156291448001,7.29187858430588,35.4305442418459));
#55300=CARTESIAN_POINT('Ctrl Pts',(22.6832958361958,7.16615578938679,37.3311252364372));
#55301=CARTESIAN_POINT('Ctrl Pts',(22.1055973813781,7.04043299446771,39.9324040531833));
#55302=CARTESIAN_POINT('Ctrl Pts',(19.6090070999777,6.91471019954863,40.863760029149));
#55303=CARTESIAN_POINT('Ctrl Pts',(17.8702883666026,6.81257501512464,39.5742316475738));
#55304=CARTESIAN_POINT('Ctrl Pts',(17.6390752763342,6.75234742900701,38.4447601330821));
#55305=CARTESIAN_POINT('Ctrl Pts',(17.6401044046334,6.73402744119574,38.1007965110423));
#55306=CARTESIAN_POINT('',(17.6365309617442,5.94027684968202,38.0978678400331));
#55307=CARTESIAN_POINT('Ctrl Pts',(17.636530130895,6.73402684972829,38.1007865956311));
#55308=CARTESIAN_POINT('Ctrl Pts',(17.6365030726185,6.72970315999644,38.0194850745859));
#55309=CARTESIAN_POINT('Ctrl Pts',(17.6406754204681,6.7253794702646,37.9382157103641));
#55310=CARTESIAN_POINT('Ctrl Pts',(17.6490110348502,6.72105578053275,37.8574276878044));
#55311=CARTESIAN_POINT('Ctrl Pts',(17.6573525203997,6.71672904542176,37.7765827624198));
#55312=CARTESIAN_POINT('Ctrl Pts',(17.6698630616553,6.71240231031076,37.6962202870288));
#55313=CARTESIAN_POINT('Ctrl Pts',(17.6864549718565,6.70807557519977,37.6167817846434));
#55314=CARTESIAN_POINT('Ctrl Pts',(17.7030761246116,6.70374121439748,37.5372032751902));
#55315=CARTESIAN_POINT('Ctrl Pts',(17.7237929189623,6.69940685359519,37.4585524180726));
#55316=CARTESIAN_POINT('Ctrl Pts',(17.7484670911131,6.6950724927929,37.3812580427585));
#55317=CARTESIAN_POINT('Ctrl Pts',(17.7731654827171,6.6907338775075,37.3038877975228));
#55318=CARTESIAN_POINT('Ctrl Pts',(17.8018288365831,6.6863952622221,37.2278770944096));
#55319=CARTESIAN_POINT('Ctrl Pts',(17.8342706913796,6.6820566469367,37.1536348470687));
#55320=CARTESIAN_POINT('Ctrl Pts',(17.86677938582,6.67770909284362,37.0792396391339));
#55321=CARTESIAN_POINT('Ctrl Pts',(17.9030819344239,6.67336153875053,37.0066205541054));
#55322=CARTESIAN_POINT('Ctrl Pts',(17.9429459095411,6.66901398465745,36.9361619915872));
#55323=CARTESIAN_POINT('Ctrl Pts',(17.9605184675755,6.66709752634179,36.905102942026));
#55324=CARTESIAN_POINT('Ctrl Pts',(17.9787825054123,6.66518106802613,36.8744633307563));
#55325=CARTESIAN_POINT('Ctrl Pts',(17.9977155506846,6.66326460971047,36.8442741441979));
#55326=CARTESIAN_POINT('Ctrl Pts',(18.0395800015446,6.65902696733297,36.7775202913974));
#55327=CARTESIAN_POINT('Ctrl Pts',(18.0848649312771,6.65478932495548,36.712736993741));
#55328=CARTESIAN_POINT('Ctrl Pts',(18.1333589265657,6.65055168257798,36.6502960495784));
#55329=CARTESIAN_POINT('Ctrl Pts',(18.1817831855859,6.64632013409652,36.5879448979439));
#55330=CARTESIAN_POINT('Ctrl Pts',(18.2334070605116,6.64208858561506,36.5279297776531));
#55331=CARTESIAN_POINT('Ctrl Pts',(18.2879750593924,6.6378570371336,36.4705948804433));
#55332=CARTESIAN_POINT('Ctrl Pts',(18.3424800307276,6.6336303762075,36.4133262066231));
#55333=CARTESIAN_POINT('Ctrl Pts',(18.3999220467381,6.6294037152814,36.3587319417326));
#55334=CARTESIAN_POINT('Ctrl Pts',(18.4600053953514,6.62517705435529,36.3071232450184));
#55335=CARTESIAN_POINT('Ctrl Pts',(18.5200508174828,6.62095306142927,36.2555471253219));
#55336=CARTESIAN_POINT('Ctrl Pts',(18.5827339081565,6.61672906850325,36.2069531377565));
#55337=CARTESIAN_POINT('Ctrl Pts',(18.6477230303954,6.61250507557723,36.1616147342757));
#55338=CARTESIAN_POINT('Ctrl Pts',(18.7126913643955,6.60828243379077,36.1162908333075));
#55339=CARTESIAN_POINT('Ctrl Pts',(18.7799638809766,6.60405979200431,36.0742207164835));
#55340=CARTESIAN_POINT('Ctrl Pts',(18.8491780743503,6.59983715021784,36.0356358518072));
#55341=CARTESIAN_POINT('Ctrl Pts',(18.9183916779033,6.59561454441536,35.9970513159385));
#55342=CARTESIAN_POINT('Ctrl Pts',(18.9895465152061,6.59139193861287,35.9619522001709));
#55343=CARTESIAN_POINT('Ctrl Pts',(19.0622547829605,6.58716933281038,35.9305244069547));
#55344=CARTESIAN_POINT('Ctrl Pts',(19.1350353497551,6.5829425281684,35.8990653628318));
#55345=CARTESIAN_POINT('Ctrl Pts',(19.2093720012243,6.57871572352641,35.8712851198941));
#55346=CARTESIAN_POINT('Ctrl Pts',(19.2848567764607,6.57448891888443,35.8473214586351));
#55347=CARTESIAN_POINT('Ctrl Pts',(19.3603781302965,6.57026006600698,35.8233461850058));
#55348=CARTESIAN_POINT('Ctrl Pts',(19.4370482622848,6.56603121312953,35.8031912967065));
#55349=CARTESIAN_POINT('Ctrl Pts',(19.5144463422357,6.56180236025208,35.7869439941213));
#55350=CARTESIAN_POINT('Ctrl Pts',(19.5919835234973,6.5575659071993,35.7706674915729));
#55351=CARTESIAN_POINT('Ctrl Pts',(19.6702508026572,6.55332945414652,35.758312680216));
#55352=CARTESIAN_POINT('Ctrl Pts',(19.7488197339795,6.54909300109374,35.7499151260302));
#55353=CARTESIAN_POINT('Ctrl Pts',(19.8202288705043,6.54524260565962,35.7422828204453));
#55354=CARTESIAN_POINT('Ctrl Pts',(19.8918868679174,6.54139221022551,35.737918754183));
#55355=CARTESIAN_POINT('Ctrl Pts',(19.9634731513095,6.53754181479139,35.7368122735964));
#55356=CARTESIAN_POINT('Ctrl Pts',(20.042259102867,6.5333041724139,35.7355945106149));
#55357=CARTESIAN_POINT('Ctrl Pts',(20.1212539077664,6.5290665300364,35.7383187196748));
#55358=CARTESIAN_POINT('Ctrl Pts',(20.2000305966432,6.52482888765891,35.7450099360493));
#55359=CARTESIAN_POINT('Ctrl Pts',(20.27869400155,6.52059733917745,35.751691530192));
#55360=CARTESIAN_POINT('Ctrl Pts',(20.3571394501003,6.51636579069598,35.7623287632727));
#55361=CARTESIAN_POINT('Ctrl Pts',(20.4349391376553,6.51213424221452,35.7768946671673));
#55362=CARTESIAN_POINT('Ctrl Pts',(20.5126489644227,6.50790758128842,35.7914437470407));
#55363=CARTESIAN_POINT('Ctrl Pts',(20.5897140539943,6.50368092036231,35.8099123943005));
#55364=CARTESIAN_POINT('Ctrl Pts',(20.6657124183755,6.49945425943621,35.8322219207073));
#55365=CARTESIAN_POINT('Ctrl Pts',(20.7416628102208,6.4952302665102,35.8545173646458));
#55366=CARTESIAN_POINT('Ctrl Pts',(20.8165473647843,6.49100627358418,35.8806487437084));
#55367=CARTESIAN_POINT('Ctrl Pts',(20.8899561702956,6.48678228065817,35.9104867079982));
#55368=CARTESIAN_POINT('Ctrl Pts',(20.9633414943422,6.48255963887172,35.9403151279411));
#55369=CARTESIAN_POINT('Ctrl Pts',(21.0352515727803,6.47833699708526,35.9738476022866));
#55370=CARTESIAN_POINT('Ctrl Pts',(21.1052949098236,6.47411435529881,36.0109060329372));
#55371=CARTESIAN_POINT('Ctrl Pts',(21.1753376499804,6.46989174949633,36.047964147788));
#55372=CARTESIAN_POINT('Ctrl Pts',(21.2435132666876,6.46566914369385,36.0885479387124));
#55373=CARTESIAN_POINT('Ctrl Pts',(21.3094547172913,6.46144653789137,36.1324332834022));
#55374=CARTESIAN_POINT('Ctrl Pts',(21.3754617382042,6.45721973324939,36.1763622664347));
#55375=CARTESIAN_POINT('Ctrl Pts',(21.4392297642179,6.45299292860741,36.2235991006603));
#55376=CARTESIAN_POINT('Ctrl Pts',(21.5004211481249,6.44876612396542,36.2738765597147));
#55377=CARTESIAN_POINT('Ctrl Pts',(21.5616421843044,6.44453727108797,36.3241783823448));
#55378=CARTESIAN_POINT('Ctrl Pts',(21.6202837438227,6.44030841821051,36.3775234492089));
#55379=CARTESIAN_POINT('Ctrl Pts',(21.6760436042791,6.43607956533306,36.433606205768));
#55380=CARTESIAN_POINT('Ctrl Pts',(21.731903677424,6.43184311228028,36.4897897553305));
#55381=CARTESIAN_POINT('Ctrl Pts',(21.7848713891656,6.4276066592275,36.5487204762121));
#55382=CARTESIAN_POINT('Ctrl Pts',(21.8346836861194,6.42337020617472,36.6100583189979));
#55383=CARTESIAN_POINT('Ctrl Pts',(21.8799567101245,6.41951981074058,36.6658065939959));
#55384=CARTESIAN_POINT('Ctrl Pts',(21.9226235779161,6.41566941530645,36.7235426491132));
#55385=CARTESIAN_POINT('Ctrl Pts',(21.9625187261799,6.41181901987231,36.7829917652903));
#55386=CARTESIAN_POINT('Ctrl Pts',(22.0064262608295,6.40758137749482,36.8484198747731));
#55387=CARTESIAN_POINT('Ctrl Pts',(22.047140689196,6.40334373511733,36.9161689399982));
#55388=CARTESIAN_POINT('Ctrl Pts',(22.0844085954045,6.39910609273984,36.9858944177935));
#55389=CARTESIAN_POINT('Ctrl Pts',(22.1216229089014,6.39487454425839,37.0555196276154));
#55390=CARTESIAN_POINT('Ctrl Pts',(22.1554003237148,6.39064299577694,37.1271151957349));
#55391=CARTESIAN_POINT('Ctrl Pts',(22.185530593265,6.38641144729549,37.2003075709984));
#55392=CARTESIAN_POINT('Ctrl Pts',(22.2156260615218,6.38218478636939,37.2734154070474));
#55393=CARTESIAN_POINT('Ctrl Pts',(22.2420825783761,6.37795812544329,37.3481159537538));
#55394=CARTESIAN_POINT('Ctrl Pts',(22.2647364497823,6.37373146451718,37.4240123862617));
#55395=CARTESIAN_POINT('Ctrl Pts',(22.2873760213589,6.36950747159117,37.4998609105762));
#55396=CARTESIAN_POINT('Ctrl Pts',(22.3062175781883,6.36528347866516,37.5769033743228));
#55397=CARTESIAN_POINT('Ctrl Pts',(22.3211464981653,6.36105948573914,37.6547255060584));
#55398=CARTESIAN_POINT('Ctrl Pts',(22.33607064279,6.35683684395268,37.7325227446273));
#55399=CARTESIAN_POINT('Ctrl Pts',(22.3470845476314,6.35261420216622,37.8110986958902));
#55400=CARTESIAN_POINT('Ctrl Pts',(22.3541245083443,6.34839156037976,37.8900280015987));
#55401=CARTESIAN_POINT('Ctrl Pts',(22.361164409065,6.34416895457728,37.9689566346973));
#55402=CARTESIAN_POINT('Ctrl Pts',(22.3642303927682,6.3399463487748,38.0482381492084));
#55403=CARTESIAN_POINT('Ctrl Pts',(22.3633106740363,6.33572374297231,38.1274426472103));
#55404=CARTESIAN_POINT('Ctrl Pts',(22.3623900407622,6.33149693833033,38.2067259039196));
#55405=CARTESIAN_POINT('Ctrl Pts',(22.3574757938599,6.32727013368835,38.2859315213133));
#55406=CARTESIAN_POINT('Ctrl Pts',(22.3486083074933,6.32304332904637,38.3646307972881));
#55407=CARTESIAN_POINT('Ctrl Pts',(22.3397365240982,6.31881447616892,38.443368209553));
#55408=CARTESIAN_POINT('Ctrl Pts',(22.3269077609558,6.31458562329147,38.5215983284183));
#55409=CARTESIAN_POINT('Ctrl Pts',(22.3102138274744,6.31035677041402,38.5989013051158));
#55410=CARTESIAN_POINT('Ctrl Pts',(22.2934898913362,6.30612031736125,38.6763432122026));
#55411=CARTESIAN_POINT('Ctrl Pts',(22.2728870271406,6.30188386430847,38.7528541940136));
#55412=CARTESIAN_POINT('Ctrl Pts',(22.2485473020164,6.29764741125569,38.8280284826122));
#55413=CARTESIAN_POINT('Ctrl Pts',(22.2264255965899,6.29379701582154,38.8963523219136));
#55414=CARTESIAN_POINT('Ctrl Pts',(22.2012177834238,6.28994662038738,38.9635719605848));
#55415=CARTESIAN_POINT('Ctrl Pts',(22.1730641934383,6.28609622495323,39.0293989735827));
#55416=CARTESIAN_POINT('Ctrl Pts',(22.1420791042334,6.28185858257573,39.1018464259636));
#55417=CARTESIAN_POINT('Ctrl Pts',(22.1074089192801,6.27762094019822,39.1728786636548));
#55418=CARTESIAN_POINT('Ctrl Pts',(22.0692047214133,6.27338329782073,39.2420955572021));
#55419=CARTESIAN_POINT('Ctrl Pts',(22.0310554626825,6.26915174933927,39.31121291414));
#55420=CARTESIAN_POINT('Ctrl Pts',(21.9893825081704,6.26492020085782,39.3785197041992));
#55421=CARTESIAN_POINT('Ctrl Pts',(21.9443847731485,6.26068865237637,39.443636221173));
#55422=CARTESIAN_POINT('Ctrl Pts',(21.8994390117532,6.25646199145027,39.5086775267716));
#55423=CARTESIAN_POINT('Ctrl Pts',(21.8511763664676,6.25223533052416,39.5715332029856));
#55424=CARTESIAN_POINT('Ctrl Pts',(21.7998406163161,6.24800866959806,39.6318499263175));
#55425=CARTESIAN_POINT('Ctrl Pts',(21.7485372708899,6.24378467667204,39.692128575854));
#55426=CARTESIAN_POINT('Ctrl Pts',(21.6941649739992,6.23956068374603,39.7498710975752));
#55427=CARTESIAN_POINT('Ctrl Pts',(21.6370088516455,6.23533669082002,39.8047558360464));
#55428=CARTESIAN_POINT('Ctrl Pts',(21.5798710119687,6.23111404903355,39.8596230183942));
#55429=CARTESIAN_POINT('Ctrl Pts',(21.5199514530048,6.22689140724709,39.9116339083146));
#55430=CARTESIAN_POINT('Ctrl Pts',(21.4575723174632,6.22266876546063,39.9605035286892));
#55431=CARTESIAN_POINT('Ctrl Pts',(21.3951937134964,6.21844615965815,40.0093727326128));
#55432=CARTESIAN_POINT('Ctrl Pts',(21.3303559445216,6.21422355385566,40.0551004322445));
#55433=CARTESIAN_POINT('Ctrl Pts',(21.2634132227497,6.21000094805318,40.097442732466));
#55434=CARTESIAN_POINT('Ctrl Pts',(21.196403935033,6.2057741434112,40.1398271366706));
#55435=CARTESIAN_POINT('Ctrl Pts',(21.127285910628,6.20154733876921,40.1788191660058));
#55436=CARTESIAN_POINT('Ctrl Pts',(21.0564407509257,6.19732053412722,40.2142193312624));
#55437=CARTESIAN_POINT('Ctrl Pts',(20.9855612609005,6.19309168124977,40.2496366508187));
#55438=CARTESIAN_POINT('Ctrl Pts',(20.9129533981948,6.18886282837232,40.2814584504973));
#55439=CARTESIAN_POINT('Ctrl Pts',(20.8390193354553,6.18463397549487,40.3095332076328));
#55440=CARTESIAN_POINT('Ctrl Pts',(20.7649523970032,6.18039752244209,40.3376584212592));
#55441=CARTESIAN_POINT('Ctrl Pts',(20.6895549432289,6.17616106938931,40.3620229921586));
#55442=CARTESIAN_POINT('Ctrl Pts',(20.6132446918886,6.17192461633653,40.3825252219352));
#55443=CARTESIAN_POINT('Ctrl Pts',(20.543888407356,6.16807422090241,40.4011591335915));
#55444=CARTESIAN_POINT('Ctrl Pts',(20.4737785228483,6.16422382546828,40.4166031538563));
#55445=CARTESIAN_POINT('Ctrl Pts',(20.4032333758916,6.16037343003415,40.4288180017913));
#55446=CARTESIAN_POINT('Ctrl Pts',(20.3255932712882,6.15613578765666,40.4422613371914));
#55447=CARTESIAN_POINT('Ctrl Pts',(20.2471344158678,6.15189814527916,40.4518430135706));
#55448=CARTESIAN_POINT('Ctrl Pts',(20.1682747050158,6.14766050290166,40.4574719647436));
#55449=CARTESIAN_POINT('Ctrl Pts',(20.089528397523,6.14342895442022,40.4630928212639));
#55450=CARTESIAN_POINT('Ctrl Pts',(20.0103828430872,6.13919740593877,40.4647722077209));
#55451=CARTESIAN_POINT('Ctrl Pts',(19.931264841588,6.13496585745733,40.4624703001092));
#55452=CARTESIAN_POINT('Ctrl Pts',(19.8522382235653,6.13073919653123,40.4601710512644));
#55453=CARTESIAN_POINT('Ctrl Pts',(19.7732395614395,6.12651253560512,40.4538996603001));
#55454=CARTESIAN_POINT('Ctrl Pts',(19.6946979444256,6.12228587467902,40.4436682990052));
#55455=CARTESIAN_POINT('Ctrl Pts',(19.6162059053278,6.118061881753,40.4334433960644));
#55456=CARTESIAN_POINT('Ctrl Pts',(19.5381708023289,6.11383788882699,40.419263544731));
#55457=CARTESIAN_POINT('Ctrl Pts',(19.4610176659607,6.10961389590098,40.4011928394842));
#55458=CARTESIAN_POINT('Ctrl Pts',(19.3838892087661,6.10539125411452,40.3831279145608));
#55459=CARTESIAN_POINT('Ctrl Pts',(19.3076426140659,6.10116861232806,40.3611747140345));
#55460=CARTESIAN_POINT('Ctrl Pts',(19.2326922936507,6.09694597054161,40.335448349812));
#55461=CARTESIAN_POINT('Ctrl Pts',(19.1577426119376,6.09272336473912,40.3097222048211));
#55462=CARTESIAN_POINT('Ctrl Pts',(19.0840896254625,6.08850075893664,40.2802231136058));
#55463=CARTESIAN_POINT('Ctrl Pts',(19.0121307402265,6.08427815313415,40.2471154525304));
#55464=CARTESIAN_POINT('Ctrl Pts',(18.9401003011151,6.08005134849217,40.2139748701354));
#55465=CARTESIAN_POINT('Ctrl Pts',(18.8697677550231,6.07582454385019,40.1772187467062));
#55466=CARTESIAN_POINT('Ctrl Pts',(18.8015081661781,6.07159773920821,40.1370586062169));
#55467=CARTESIAN_POINT('Ctrl Pts',(18.7332154999324,6.06736888633076,40.0968790048271));
#55468=CARTESIAN_POINT('Ctrl Pts',(18.6669981841135,6.06314003345332,40.0532923583951));
#55469=CARTESIAN_POINT('Ctrl Pts',(18.6032022430351,6.05891118057588,40.0065535573484));
#55470=CARTESIAN_POINT('Ctrl Pts',(18.5392916466703,6.0546747275231,39.9597307564339));
#55471=CARTESIAN_POINT('Ctrl Pts',(18.4778114848346,6.05043827447032,39.9097447778856));
#55472=CARTESIAN_POINT('Ctrl Pts',(18.4190744476327,6.04620182141754,39.8568906735401));
#55473=CARTESIAN_POINT('Ctrl Pts',(18.3656899731583,6.04235142598338,39.8088530346207));
#55474=CARTESIAN_POINT('Ctrl Pts',(18.3145711839386,6.03850103054923,39.7584468538845));
#55475=CARTESIAN_POINT('Ctrl Pts',(18.2659243139061,6.03465063511508,39.7059177923536));
#55476=CARTESIAN_POINT('Ctrl Pts',(18.2130172211904,6.03046304343466,39.6487885273707));
#55477=CARTESIAN_POINT('Ctrl Pts',(18.1628255204444,6.02627545175425,39.5889219903604));
#55478=CARTESIAN_POINT('Ctrl Pts',(18.1156500699753,6.02208786007384,39.5266098913564));
#55479=CARTESIAN_POINT('Ctrl Pts',(18.0685365912465,6.01790576939746,39.4643796482579));
#55480=CARTESIAN_POINT('Ctrl Pts',(18.0244317920978,6.01372367872109,39.3997105934865));
#55481=CARTESIAN_POINT('Ctrl Pts',(17.9835989233411,6.00954158804471,39.3329303057954));
#55482=CARTESIAN_POINT('Ctrl Pts',(17.9428062547143,6.00536361465408,39.2662157635766));
#55483=CARTESIAN_POINT('Ctrl Pts',(17.9052793751211,6.00118564126344,39.1973945197397));
#55484=CARTESIAN_POINT('Ctrl Pts',(17.8712395298754,5.99700766787281,39.1268248641979));
#55485=CARTESIAN_POINT('Ctrl Pts',(17.8372219986205,5.99283243325079,39.0563014688735));
#55486=CARTESIAN_POINT('Ctrl Pts',(17.8066871724102,5.98865719862876,38.9840323687656));
#55487=CARTESIAN_POINT('Ctrl Pts',(17.7798106199974,5.98448196400674,38.9104008624277));
#55488=CARTESIAN_POINT('Ctrl Pts',(17.7529350517411,5.98030688227206,38.8367720523035));
#55489=CARTESIAN_POINT('Ctrl Pts',(17.7297176706244,5.97613180053737,38.7617813810599));
#55490=CARTESIAN_POINT('Ctrl Pts',(17.7102855957909,5.97195671880268,38.6858313648631));
#55491=CARTESIAN_POINT('Ctrl Pts',(17.690854232713,5.96778178999237,38.609884130554));
#55492=CARTESIAN_POINT('Ctrl Pts',(17.6752080112612,5.96360686118205,38.5329780891183));
#55493=CARTESIAN_POINT('Ctrl Pts',(17.6634234014289,5.95943193237174,38.4555281140923));
#55494=CARTESIAN_POINT('Ctrl Pts',(17.6516296863262,5.95525377784107,38.3780182980553));
#55495=CARTESIAN_POINT('Ctrl Pts',(17.6437036009049,5.95107562331041,38.2999641866128));
#55496=CARTESIAN_POINT('Ctrl Pts',(17.6396698565796,5.94689746877974,38.2217869244251));
#55497=CARTESIAN_POINT('Ctrl Pts',(17.637539260058,5.94469059576259,38.1804942222977));
#55498=CARTESIAN_POINT('Ctrl Pts',(17.6364937042972,5.94248372274543,38.1391672076312));
#55499=CARTESIAN_POINT('Ctrl Pts',(17.6365309617434,5.94027684972828,38.0978678408989));
#55500=CARTESIAN_POINT('',(17.6365301680466,5.14652684968129,38.1008912610287));
#55501=CARTESIAN_POINT('Ctrl Pts',(17.6365309617442,5.94027684968202,38.0978678400331));
#55502=CARTESIAN_POINT('Ctrl Pts',(17.6366235326623,5.93479359199753,37.9952542921597));
#55503=CARTESIAN_POINT('Ctrl Pts',(17.6434025454018,5.92931033431303,37.8929359218963));
#55504=CARTESIAN_POINT('Ctrl Pts',(17.6567308745933,5.92382707662854,37.7916491498052));
#55505=CARTESIAN_POINT('Ctrl Pts',(17.6688028908594,5.91886066448436,37.6999095519417));
#55506=CARTESIAN_POINT('Ctrl Pts',(17.6862470647488,5.91389425234017,37.6090156628067));
#55507=CARTESIAN_POINT('Ctrl Pts',(17.7089286062922,5.90892784019599,37.5194982258133));
#55508=CARTESIAN_POINT('Ctrl Pts',(17.7282818655146,5.90469019781849,37.4431165495617));
#55509=CARTESIAN_POINT('Ctrl Pts',(17.751495345354,5.900452555441,37.3675603792653));
#55510=CARTESIAN_POINT('Ctrl Pts',(17.778481962481,5.8962149130635,37.2932484583978));
#55511=CARTESIAN_POINT('Ctrl Pts',(17.8054297717935,5.89198336458204,37.2190434009888));
#55512=CARTESIAN_POINT('Ctrl Pts',(17.83613978433,5.88775181610058,37.1460794766435));
#55513=CARTESIAN_POINT('Ctrl Pts',(17.8704744921261,5.88352026761912,37.0747626849288));
#55514=CARTESIAN_POINT('Ctrl Pts',(17.9047695423865,5.87929360669301,37.003528266078));
#55515=CARTESIAN_POINT('Ctrl Pts',(17.9426807657155,5.8750669457669,36.9339376193788));
#55516=CARTESIAN_POINT('Ctrl Pts',(17.9840222362744,5.87084028484079,36.8663776521708));
#55517=CARTESIAN_POINT('Ctrl Pts',(18.0253376108088,5.86661629191477,36.7988603309193));
#55518=CARTESIAN_POINT('Ctrl Pts',(18.0700786906955,5.86239229898875,36.7333715436769));
#55519=CARTESIAN_POINT('Ctrl Pts',(18.1180137851516,5.85816830606273,36.6702733380046));
#55520=CARTESIAN_POINT('Ctrl Pts',(18.1659335464848,5.85394566427627,36.6071953157188));
#55521=CARTESIAN_POINT('Ctrl Pts',(18.2170450101681,5.84972302248981,36.5465067295028));
#55522=CARTESIAN_POINT('Ctrl Pts',(18.2710742197591,5.84550038070334,36.4885391449624));
#55523=CARTESIAN_POINT('Ctrl Pts',(18.3251029689308,5.84127777490085,36.4305720544029));
#55524=CARTESIAN_POINT('Ctrl Pts',(18.3820490939087,5.83705516909836,36.3753262613571));
#55525=CARTESIAN_POINT('Ctrl Pts',(18.4416005755605,5.83283256329587,36.3230977306541));
#55526=CARTESIAN_POINT('Ctrl Pts',(18.5012112735172,5.82860575865388,36.270817265381));
#55527=CARTESIAN_POINT('Ctrl Pts',(18.5634321498163,5.8243789540119,36.2215603653372));
#55528=CARTESIAN_POINT('Ctrl Pts',(18.6279172297163,5.82015214936991,36.1755833838821));
#55529=CARTESIAN_POINT('Ctrl Pts',(18.6924335579561,5.81592329649245,36.1295841227874));
#55530=CARTESIAN_POINT('Ctrl Pts',(18.7592158801282,5.811694443615,36.0868681994476));
#55531=CARTESIAN_POINT('Ctrl Pts',(18.827890447833,5.80746559073754,36.0476477791035));
#55532=CARTESIAN_POINT('Ctrl Pts',(18.8966884387851,5.80322913768476,36.0083568710694));
#55533=CARTESIAN_POINT('Ctrl Pts',(18.9673850511148,5.79899268463198,35.972574230643));
#55534=CARTESIAN_POINT('Ctrl Pts',(19.0395834392595,5.79475623157919,35.9404652189058));
#55535=CARTESIAN_POINT('Ctrl Pts',(19.1052025646453,5.7909058361451,35.9112822229784));
#55536=CARTESIAN_POINT('Ctrl Pts',(19.1720617280285,5.78705544071101,35.8851333044687));
#55537=CARTESIAN_POINT('Ctrl Pts',(19.2398525600461,5.78320504527692,35.8621067249684));
#55538=CARTESIAN_POINT('Ctrl Pts',(19.3144613391911,5.77896740289943,35.8367642865698));
#55539=CARTESIAN_POINT('Ctrl Pts',(19.3904788833851,5.77472976052194,35.815109414351));
#55540=CARTESIAN_POINT('Ctrl Pts',(19.4675065197498,5.77049211814445,35.7972969938807));
#55541=CARTESIAN_POINT('Ctrl Pts',(19.5444233873506,5.76626056966299,35.77951018837));
#55542=CARTESIAN_POINT('Ctrl Pts',(19.6223470095406,5.76202902118154,35.7655549660279));
#55543=CARTESIAN_POINT('Ctrl Pts',(19.7008619559717,5.75779747270009,35.7555369758695));
#55544=CARTESIAN_POINT('Ctrl Pts',(19.7792862154715,5.75357081177399,35.7455305567665));
#55545=CARTESIAN_POINT('Ctrl Pts',(19.8582999792779,5.74934415084789,35.7394523916293));
#55546=CARTESIAN_POINT('Ctrl Pts',(19.9374774773243,5.74511748992178,35.7373571207103));
#55547=CARTESIAN_POINT('Ctrl Pts',(20.0166049960666,5.74089349699577,35.7352631723916));
#55548=CARTESIAN_POINT('Ctrl Pts',(20.0958955765188,5.73666950406976,35.737147140395));
#55549=CARTESIAN_POINT('Ctrl Pts',(20.1749193911915,5.73244551114374,35.7430117421834));
#55550=CARTESIAN_POINT('Ctrl Pts',(20.2539179283118,5.72822286935729,35.7488744680465));
#55551=CARTESIAN_POINT('Ctrl Pts',(20.3326494019525,5.72400022757083,35.7587152645124));
#55552=CARTESIAN_POINT('Ctrl Pts',(20.4106865482482,5.71977758578438,35.7724848013412));
#55553=CARTESIAN_POINT('Ctrl Pts',(20.4887230295368,5.71555497998189,35.7862542208304));
#55554=CARTESIAN_POINT('Ctrl Pts',(20.5660647338519,5.71133237417941,35.8039522312514));
#55555=CARTESIAN_POINT('Ctrl Pts',(20.6422935427912,5.70710976837693,35.8254781940398));
#55556=CARTESIAN_POINT('Ctrl Pts',(20.7185981514971,5.70288296373495,35.8470255616352));
#55557=CARTESIAN_POINT('Ctrl Pts',(20.7937872021454,5.69865615909297,35.8724083572244));
#55558=CARTESIAN_POINT('Ctrl Pts',(20.8674573218677,5.69442935445099,35.9014758960525));
#55559=CARTESIAN_POINT('Ctrl Pts',(20.9411631408391,5.69020050157354,35.9305575205005));
#55560=CARTESIAN_POINT('Ctrl Pts',(21.0133481351976,5.6859716486961,35.9633272512121));
#55561=CARTESIAN_POINT('Ctrl Pts',(21.083630881866,5.68174279581865,35.9995870518476));
#55562=CARTESIAN_POINT('Ctrl Pts',(21.1540399420318,5.67750634276588,36.0359120192907));
#55563=CARTESIAN_POINT('Ctrl Pts',(21.222539517287,5.6732698897131,36.0757393533793));
#55564=CARTESIAN_POINT('Ctrl Pts',(21.2887748744403,5.66903343666033,36.1188261651457));
#55565=CARTESIAN_POINT('Ctrl Pts',(21.3489743652848,5.66518304122616,36.1579865810009));
#55566=CARTESIAN_POINT('Ctrl Pts',(21.4073036636659,5.66133264579199,36.1998387806815));
#55567=CARTESIAN_POINT('Ctrl Pts',(21.463520873394,5.65748225035783,36.2441721270441));
#55568=CARTESIAN_POINT('Ctrl Pts',(21.5253920329571,5.65324460798033,36.2929642239843));
#55569=CARTESIAN_POINT('Ctrl Pts',(21.5849366536444,5.64900696560284,36.3449453615566));
#55570=CARTESIAN_POINT('Ctrl Pts',(21.6418077951597,5.64476932322535,36.3998654157236));
#55571=CARTESIAN_POINT('Ctrl Pts',(21.6985971537418,5.64053777474389,36.4547064926974));
#55572=CARTESIAN_POINT('Ctrl Pts',(21.7527203336871,5.63630622626243,36.5124777703227));
#55573=CARTESIAN_POINT('Ctrl Pts',(21.8038625759622,5.63207467778097,36.5728882660581));
#55574=CARTESIAN_POINT('Ctrl Pts',(21.8549457475351,5.62784801685487,36.6332289860026));
#55575=CARTESIAN_POINT('Ctrl Pts',(21.9030545223185,5.62362135592877,36.6962025102102));
#55576=CARTESIAN_POINT('Ctrl Pts',(21.9479113026009,5.61939469500266,36.7614814166028));
#55577=CARTESIAN_POINT('Ctrl Pts',(21.9927397678858,5.61517070207664,36.8267191169155));
#55578=CARTESIAN_POINT('Ctrl Pts',(22.0343200483831,5.61094670915063,36.8942589256039));
#55579=CARTESIAN_POINT('Ctrl Pts',(22.0724158941268,5.60672271622461,36.9637417535302));
#55580=CARTESIAN_POINT('Ctrl Pts',(22.1104995540536,5.60250007443815,37.0332023558044));
#55581=CARTESIAN_POINT('Ctrl Pts',(22.1451007673485,5.59827743265169,37.1046043323545));
#55582=CARTESIAN_POINT('Ctrl Pts',(22.1760283406479,5.59405479086523,37.1775624131699));
#55583=CARTESIAN_POINT('Ctrl Pts',(22.2069556503927,5.58983218506275,37.2505198722603));
#55584=CARTESIAN_POINT('Ctrl Pts',(22.2342092007462,5.58560957926027,37.3250329770968));
#55585=CARTESIAN_POINT('Ctrl Pts',(22.2576458174357,5.58138697345778,37.4006962005573));
#55586=CARTESIAN_POINT('Ctrl Pts',(22.2811057388325,5.5771601688158,37.4764346613822));
#55587=CARTESIAN_POINT('Ctrl Pts',(22.3007410061124,5.57293336417381,37.5533250764427));
#55588=CARTESIAN_POINT('Ctrl Pts',(22.3164584536478,5.56870655953183,37.6309470462476));
#55589=CARTESIAN_POINT('Ctrl Pts',(22.3321835175828,5.56447770665438,37.708606630299));
#55590=CARTESIAN_POINT('Ctrl Pts',(22.34398690984,5.56024885377693,37.7869980111561));
#55591=CARTESIAN_POINT('Ctrl Pts',(22.3518271345525,5.55602000089948,37.8656934271461));
#55592=CARTESIAN_POINT('Ctrl Pts',(22.359681449867,5.5517835478467,37.9445302760439));
#55593=CARTESIAN_POINT('Ctrl Pts',(22.3635583428394,5.54754709479392,38.0236717825474));
#55594=CARTESIAN_POINT('Ctrl Pts',(22.3634684712725,5.54331064174114,38.1026881593849));
#55595=CARTESIAN_POINT('Ctrl Pts',(22.3633867894819,5.53946024630701,38.1745039668083));
#55596=CARTESIAN_POINT('Ctrl Pts',(22.3600290452797,5.53560985087289,38.2462161639682));
#55597=CARTESIAN_POINT('Ctrl Pts',(22.3534402626473,5.53175945543876,38.3175071747104));
#55598=CARTESIAN_POINT('Ctrl Pts',(22.346188824457,5.52752181306127,38.3959681570753));
#55599=CARTESIAN_POINT('Ctrl Pts',(22.3349957856703,5.52328417068377,38.4742133895104));
#55600=CARTESIAN_POINT('Ctrl Pts',(22.319882115305,5.51904652830628,38.5518156836456));
#55601=CARTESIAN_POINT('Ctrl Pts',(22.3047901789907,5.51481497982482,38.6293063826365));
#55602=CARTESIAN_POINT('Ctrl Pts',(22.2857888965608,5.51058343134337,38.7061555231122));
#55603=CARTESIAN_POINT('Ctrl Pts',(22.2629510293121,5.50635188286191,38.7819406717855));
#55604=CARTESIAN_POINT('Ctrl Pts',(22.2401395404308,5.50212522193581,38.8576382865193));
#55605=CARTESIAN_POINT('Ctrl Pts',(22.213500407533,5.4978985610097,38.9322739050989));
#55606=CARTESIAN_POINT('Ctrl Pts',(22.1831571880899,5.4936719000836,39.0054364323306));
#55607=CARTESIAN_POINT('Ctrl Pts',(22.1528331222324,5.48944790715758,39.0785527770953));
#55608=CARTESIAN_POINT('Ctrl Pts',(22.1188097898846,5.48522391423156,39.1501974443069));
#55609=CARTESIAN_POINT('Ctrl Pts',(22.0812598200345,5.48099992130555,39.2199767865495));
#55610=CARTESIAN_POINT('Ctrl Pts',(22.0437218613905,5.47677727951909,39.2897338082933));
#55611=CARTESIAN_POINT('Ctrl Pts',(22.002659727355,5.47255463773263,39.3576262774278));
#55612=CARTESIAN_POINT('Ctrl Pts',(21.9582925351113,5.46833199594617,39.4232840918817));
#55613=CARTESIAN_POINT('Ctrl Pts',(21.9139257209504,5.46410939014368,39.4889413468213));
#55614=CARTESIAN_POINT('Ctrl Pts',(21.8662541682268,5.4598867843412,39.5523635973345));
#55615=CARTESIAN_POINT('Ctrl Pts',(21.8155401256557,5.45566417853871,39.6132099963436));
#55616=CARTESIAN_POINT('Ctrl Pts',(21.7647756544783,5.45143737389673,39.6741168992869));
#55617=CARTESIAN_POINT('Ctrl Pts',(21.7109629511014,5.44721056925474,39.732442473477));
#55618=CARTESIAN_POINT('Ctrl Pts',(21.6544039616708,5.44298376461276,39.7878797269083));
#55619=CARTESIAN_POINT('Ctrl Pts',(21.5978175647449,5.43875491173531,39.8433438442612));
#55620=CARTESIAN_POINT('Ctrl Pts',(21.5384825819637,5.43452605885786,39.8959165413559));
#55621=CARTESIAN_POINT('Ctrl Pts',(21.4767352610551,5.43029720598041,39.9453301627775));
#55622=CARTESIAN_POINT('Ctrl Pts',(21.4148769666796,5.42606075292763,39.9948325913053));
#55623=CARTESIAN_POINT('Ctrl Pts',(21.3505980526119,5.42182429987485,40.0411643251066));
#55624=CARTESIAN_POINT('Ctrl Pts',(21.2842648548844,5.41758784682207,40.0841003561838));
#55625=CARTESIAN_POINT('Ctrl Pts',(21.2239764394388,5.41373745138794,40.1231237316256));
#55626=CARTESIAN_POINT('Ctrl Pts',(21.1619916621134,5.4098870559538,40.1593425257466));
#55627=CARTESIAN_POINT('Ctrl Pts',(21.0986014354038,5.40603666051967,40.1926216397211));
#55628=CARTESIAN_POINT('Ctrl Pts',(21.028835844929,5.40179901814217,40.2292477437346));
#55629=CARTESIAN_POINT('Ctrl Pts',(20.9571056868249,5.39756137576468,40.2624499264109));
#55630=CARTESIAN_POINT('Ctrl Pts',(20.8837807297505,5.39332373338719,40.2920132441712));
#55631=CARTESIAN_POINT('Ctrl Pts',(20.8105612168419,5.38909218490573,40.3215340487203));
#55632=CARTESIAN_POINT('Ctrl Pts',(20.7357518905846,5.38486063642427,40.3474262064284));
#55633=CARTESIAN_POINT('Ctrl Pts',(20.6597467231307,5.38062908794282,40.3695208089415));
#55634=CARTESIAN_POINT('Ctrl Pts',(20.5838293437441,5.37640242701671,40.3915898915785));
#55635=CARTESIAN_POINT('Ctrl Pts',(20.5067193158726,5.37217576609061,40.4098700054719));
#55636=CARTESIAN_POINT('Ctrl Pts',(20.4288287506712,5.36794910516451,40.4242410252592));
#55637=CARTESIAN_POINT('Ctrl Pts',(20.3509873524219,5.36372511223849,40.4386029736109));
#55638=CARTESIAN_POINT('Ctrl Pts',(20.2723668545833,5.35950111931247,40.4490606408231));
#55639=CARTESIAN_POINT('Ctrl Pts',(20.1933914433055,5.35527712638646,40.4555445634834));
#55640=CARTESIAN_POINT('Ctrl Pts',(20.114441294097,5.3510544846,40.4620264121146));
#55641=CARTESIAN_POINT('Ctrl Pts',(20.0351369237563,5.34683184281354,40.4645370020018));
#55642=CARTESIAN_POINT('Ctrl Pts',(19.9559080721833,5.34260920102708,40.4630586837405));
#55643=CARTESIAN_POINT('Ctrl Pts',(19.8766798957726,5.3383865952246,40.461580378077));
#55644=CARTESIAN_POINT('Ctrl Pts',(19.7975277055146,5.33416398942211,40.4561132420264));
#55645=CARTESIAN_POINT('Ctrl Pts',(19.7188801782686,5.32994138361963,40.4466917323606));
#55646=CARTESIAN_POINT('Ctrl Pts',(19.6401544461512,5.32571457897764,40.4372608542128));
#55647=CARTESIAN_POINT('Ctrl Pts',(19.5619348459664,5.32148777433566,40.4238678039155));
#55648=CARTESIAN_POINT('Ctrl Pts',(19.484643263373,5.31726096969368,40.4065987676475));
#55649=CARTESIAN_POINT('Ctrl Pts',(19.4073142266329,5.31303211681622,40.3893213631072));
#55650=CARTESIAN_POINT('Ctrl Pts',(19.3309145556901,5.30880326393877,40.3681643561995));
#55651=CARTESIAN_POINT('Ctrl Pts',(19.2558518095822,5.30457441106132,40.3432641198927));
#55652=CARTESIAN_POINT('Ctrl Pts',(19.1806541592704,5.30033795800854,40.3183191324046));
#55653=CARTESIAN_POINT('Ctrl Pts',(19.1067986726909,5.29610150495576,40.2896176437174));
#55654=CARTESIAN_POINT('Ctrl Pts',(19.0346735114784,5.29186505190298,40.2573444814073));
#55655=CARTESIAN_POINT('Ctrl Pts',(18.9691209400327,5.28801465646886,40.2280122935474));
#55656=CARTESIAN_POINT('Ctrl Pts',(18.9049976509105,5.28416426103473,40.1957304494275));
#55657=CARTESIAN_POINT('Ctrl Pts',(18.8425753281453,5.2803138656006,40.1606694470201));
#55658=CARTESIAN_POINT('Ctrl Pts',(18.7738749869007,5.27607622322311,40.1220822441884));
#55659=CARTESIAN_POINT('Ctrl Pts',(18.7069774783263,5.27183858084562,40.07998326721));
#55660=CARTESIAN_POINT('Ctrl Pts',(18.6422643898427,5.26760093846813,40.0345657016009));
#55661=CARTESIAN_POINT('Ctrl Pts',(18.5776443613199,5.26336938998668,39.9892134482336));
#55662=CARTESIAN_POINT('Ctrl Pts',(18.515202895127,5.25913784150523,39.9405523505732));
#55663=CARTESIAN_POINT('Ctrl Pts',(18.4552961360479,5.25490629302378,39.8888209562703));
#55664=CARTESIAN_POINT('Ctrl Pts',(18.3954585709299,5.25067963209768,39.8371493131562));
#55665=CARTESIAN_POINT('Ctrl Pts',(18.3381502479364,5.24645297117158,39.7824147255725));
#55666=CARTESIAN_POINT('Ctrl Pts',(18.2836962630847,5.24222631024548,39.7248975117067));
#55667=CARTESIAN_POINT('Ctrl Pts',(18.2292766512852,5.23800231731946,39.6674166044986));
#55668=CARTESIAN_POINT('Ctrl Pts',(18.1777081227993,5.23377832439344,39.6071568969513));
#55669=CARTESIAN_POINT('Ctrl Pts',(18.129279847825,5.22955433146743,39.5444364136737));
#55670=CARTESIAN_POINT('Ctrl Pts',(18.0808670637285,5.22533168968097,39.4817359929595));
#55671=CARTESIAN_POINT('Ctrl Pts',(18.0355928247275,5.22110904789452,39.4165767303823));
#55672=CARTESIAN_POINT('Ctrl Pts',(17.9937058590316,5.21688640610806,39.3493095136178));
#55673=CARTESIAN_POINT('Ctrl Pts',(17.9518192502828,5.21266380030557,39.2820428700825));
#55674=CARTESIAN_POINT('Ctrl Pts',(17.9133201040219,5.20844119450308,39.2126687067619));
#55675=CARTESIAN_POINT('Ctrl Pts',(17.8784128596257,5.2042185887006,39.1415653828245));
#55676=CARTESIAN_POINT('Ctrl Pts',(17.8434709044553,5.19999178405862,39.0703913557576));
#55677=CARTESIAN_POINT('Ctrl Pts',(17.8121281926727,5.19576497941664,38.9974851552844));
#55678=CARTESIAN_POINT('Ctrl Pts',(17.7845420728401,5.19153817477466,38.9232476018091));
#55679=CARTESIAN_POINT('Ctrl Pts',(17.7569425852572,5.18730932189721,38.8489740741162));
#55680=CARTESIAN_POINT('Ctrl Pts',(17.7331034571786,5.18308046901976,38.7733683558542));
#55681=CARTESIAN_POINT('Ctrl Pts',(17.7131321386065,5.17885161614231,38.6968465677422));
#55682=CARTESIAN_POINT('Ctrl Pts',(17.6931249271985,5.17461516308954,38.620187253208));
#55683=CARTESIAN_POINT('Ctrl Pts',(17.6769995102976,5.17037871003676,38.5426090392524));
#55684=CARTESIAN_POINT('Ctrl Pts',(17.6648121322106,5.16614225698399,38.4645381503067));
#55685=CARTESIAN_POINT('Ctrl Pts',(17.6537353601193,5.16229186154983,38.3935816707724));
#55686=CARTESIAN_POINT('Ctrl Pts',(17.6459109682121,5.15844146611567,38.3222185671474));
#55687=CARTESIAN_POINT('Ctrl Pts',(17.6413438185386,5.15459107068152,38.250769554466));
#55688=CARTESIAN_POINT('Ctrl Pts',(17.6381553577927,5.15190299703044,38.200888909304));
#55689=CARTESIAN_POINT('Ctrl Pts',(17.6365490285732,5.14921492337936,38.1509060607469));
#55690=CARTESIAN_POINT('Ctrl Pts',(17.6365301680469,5.14652684972828,38.100891261903));
#55691=CARTESIAN_POINT('',(17.6365304347554,4.35277684975661,38.1014335489659));
#55692=CARTESIAN_POINT('Ctrl Pts',(17.6365301680466,5.14652684968129,38.1008912610287));
#55693=CARTESIAN_POINT('Ctrl Pts',(17.6365007172957,5.14232941297597,38.0227929721683));
#55694=CARTESIAN_POINT('Ctrl Pts',(17.6403465262968,5.13813197627065,37.944538778742));
#55695=CARTESIAN_POINT('Ctrl Pts',(17.6480877422875,5.13393453956532,37.8665494208153));
#55696=CARTESIAN_POINT('Ctrl Pts',(17.6561615253538,5.12955677857354,37.7852095953753));
#55697=CARTESIAN_POINT('Ctrl Pts',(17.6684730614319,5.12517901758175,37.7041583895631));
#55698=CARTESIAN_POINT('Ctrl Pts',(17.6849847219665,5.12080125658996,37.6238753279115));
#55699=CARTESIAN_POINT('Ctrl Pts',(17.7007772898864,5.11661414968722,37.5470886412364));
#55700=CARTESIAN_POINT('Ctrl Pts',(17.7204116738816,5.11242704278448,37.4710051167982));
#55701=CARTESIAN_POINT('Ctrl Pts',(17.7438020749889,5.10823993588174,37.3960388049932));
#55702=CARTESIAN_POINT('Ctrl Pts',(17.7671799540606,5.10405507054387,37.321112626353));
#55703=CARTESIAN_POINT('Ctrl Pts',(17.7943097185199,5.09987020520601,37.2473029294767));
#55704=CARTESIAN_POINT('Ctrl Pts',(17.8250551809499,5.09568533986814,37.1750105541211));
#55705=CARTESIAN_POINT('Ctrl Pts',(17.8557942006474,5.09150135147166,37.102733327682));
#55706=CARTESIAN_POINT('Ctrl Pts',(17.8901472264574,5.08731736307517,37.03197323143));
#55707=CARTESIAN_POINT('Ctrl Pts',(17.927929795733,5.08313337467868,36.9631114788649));
#55708=CARTESIAN_POINT('Ctrl Pts',(17.9657167571783,5.07894889989951,36.8942417212192));
#55709=CARTESIAN_POINT('Ctrl Pts',(18.0069338210219,5.07476442512034,36.8272711634052));
#55710=CARTESIAN_POINT('Ctrl Pts',(18.0513511975692,5.07057995034116,36.7625553149064));
#55711=CARTESIAN_POINT('Ctrl Pts',(18.0958154486267,5.06639105960543,36.6977711705304));
#55712=CARTESIAN_POINT('Ctrl Pts',(18.1434864789077,5.06220216886969,36.6352468772897));
#55713=CARTESIAN_POINT('Ctrl Pts',(18.194092390071,5.05801327813396,36.5753071964161));
#55714=CARTESIAN_POINT('Ctrl Pts',(18.244729818509,5.05382177856426,36.515330185212));
#55715=CARTESIAN_POINT('Ctrl Pts',(18.2983054368241,5.04963027899456,36.4579413368638));
#55716=CARTESIAN_POINT('Ctrl Pts',(18.3545102414385,5.04543877942486,36.4034287827005));
#55717=CARTESIAN_POINT('Ctrl Pts',(18.4108053900339,5.04124054241054,36.3488286046909));
#55718=CARTESIAN_POINT('Ctrl Pts',(18.4697377955761,5.03704230539623,36.2971142568638));
#55719=CARTESIAN_POINT('Ctrl Pts',(18.5309657889771,5.03284406838192,36.2485333036362));
#55720=CARTESIAN_POINT('Ctrl Pts',(18.5502937277793,5.03151880417543,36.233197676274));
#55721=CARTESIAN_POINT('Ctrl Pts',(18.569850209863,5.03019353996893,36.2181739573338));
#55722=CARTESIAN_POINT('Ctrl Pts',(18.5896239431852,5.02886827576244,36.2034690038748));
#55723=CARTESIAN_POINT('Ctrl Pts',(18.6528520979012,5.02463063338495,36.1564486937875));
#55724=CARTESIAN_POINT('Ctrl Pts',(18.7185529135914,5.02039299100746,36.1125055107695));
#55725=CARTESIAN_POINT('Ctrl Pts',(18.7863945055933,5.01615534862996,36.0719092365365));
#55726=CARTESIAN_POINT('Ctrl Pts',(18.8541385387237,5.0119238001485,36.031371341339));
#55727=CARTESIAN_POINT('Ctrl Pts',(18.9240168355792,5.00769225166704,35.994171035501));
#55728=CARTESIAN_POINT('Ctrl Pts',(18.9956664497596,5.00346070318558,35.9605363848007));
#55729=CARTESIAN_POINT('Ctrl Pts',(19.0672333066569,4.99923404225947,35.9269405830509));
#55730=CARTESIAN_POINT('Ctrl Pts',(19.1405669929246,4.99500738133337,35.8969024502745));
#55731=CARTESIAN_POINT('Ctrl Pts',(19.215279064378,4.99078072040726,35.8706046797177));
#55732=CARTESIAN_POINT('Ctrl Pts',(19.2899439752438,4.98655672748124,35.8443235091332));
#55733=CARTESIAN_POINT('Ctrl Pts',(19.3659851032591,4.98233273455522,35.8217781696134));
#55734=CARTESIAN_POINT('Ctrl Pts',(19.442994204912,4.9781087416292,35.8031031836109));
#55735=CARTESIAN_POINT('Ctrl Pts',(19.519978673464,4.97388609984274,35.7844341712246));
#55736=CARTESIAN_POINT('Ctrl Pts',(19.5979300455523,4.96966345805628,35.76963316429));
#55737=CARTESIAN_POINT('Ctrl Pts',(19.6764265414123,4.96544081626982,35.7587843632426));
#55738=CARTESIAN_POINT('Ctrl Pts',(19.7549223683509,4.96121821046733,35.747935654645));
#55739=CARTESIAN_POINT('Ctrl Pts',(19.8339628452702,4.95699560466484,35.7410391477315));
#55740=CARTESIAN_POINT('Ctrl Pts',(19.9131191472081,4.95277299886236,35.7381274043001));
#55741=CARTESIAN_POINT('Ctrl Pts',(19.9923541599286,4.94854619422037,35.7352127655136));
#55742=CARTESIAN_POINT('Ctrl Pts',(20.0717047581808,4.94431938957838,35.7362908222652));
#55743=CARTESIAN_POINT('Ctrl Pts',(20.1507407889469,4.9400925849364,35.7413419799709));
#55744=CARTESIAN_POINT('Ctrl Pts',(20.2298151191886,4.93586373205895,35.7463955853791));
#55745=CARTESIAN_POINT('Ctrl Pts',(20.3085741119602,4.9316348791815,35.7554260736865));
#55746=CARTESIAN_POINT('Ctrl Pts',(20.3865939697747,4.92740602630405,35.7683620470935));
#55747=CARTESIAN_POINT('Ctrl Pts',(20.4647540463709,4.92316957325127,35.7813212692796));
#55748=CARTESIAN_POINT('Ctrl Pts',(20.5421718746618,4.91893312019849,35.7981999011402));
#55749=CARTESIAN_POINT('Ctrl Pts',(20.6184352910172,4.91469666714571,35.818875665001));
#55750=CARTESIAN_POINT('Ctrl Pts',(20.6877490085225,4.91084627171159,35.8376672970043));
#55751=CARTESIAN_POINT('Ctrl Pts',(20.7561090637551,4.90699587627747,35.8595948257343));
#55752=CARTESIAN_POINT('Ctrl Pts',(20.8232205826439,4.90314548084336,35.8845320329079));
#55753=CARTESIAN_POINT('Ctrl Pts',(20.8970817279021,4.89890783846587,35.9119772570941));
#55754=CARTESIAN_POINT('Ctrl Pts',(20.9697075282217,4.89467019608838,35.9431717060236));
#55755=CARTESIAN_POINT('Ctrl Pts',(21.0406910158519,4.89043255371089,35.9779838241839));
#55756=CARTESIAN_POINT('Ctrl Pts',(21.1115724264413,4.88620100522944,36.0127458811522));
#55757=CARTESIAN_POINT('Ctrl Pts',(21.1808157970728,4.88196945674798,36.0511150712587));
#55758=CARTESIAN_POINT('Ctrl Pts',(21.2480322461359,4.87773790826653,36.0929110748387));
#55759=CARTESIAN_POINT('Ctrl Pts',(21.3151710583441,4.87351124734042,36.1346588028804));
#55760=CARTESIAN_POINT('Ctrl Pts',(21.3802872053651,4.86928458641432,36.179825232443));
#55761=CARTESIAN_POINT('Ctrl Pts',(21.4430159877848,4.86505792548821,36.2281839567154));
#55762=CARTESIAN_POINT('Ctrl Pts',(21.5057051738423,4.8608339325622,36.2765121554541));
#55763=CARTESIAN_POINT('Ctrl Pts',(21.5660096161983,4.85660993963618,36.3280283637388));
#55764=CARTESIAN_POINT('Ctrl Pts',(21.6235942468787,4.85238594671016,36.3824633446699));
#55765=CARTESIAN_POINT('Ctrl Pts',(21.6811604578141,4.8481633049237,36.4368809133427));
#55766=CARTESIAN_POINT('Ctrl Pts',(21.7360082442959,4.84394066313724,36.494215078853));
#55767=CARTESIAN_POINT('Ctrl Pts',(21.787837383596,4.83971802135078,36.5541578571159));
#55768=CARTESIAN_POINT('Ctrl Pts',(21.8396660812251,4.8354954155483,36.614100124566));
#55769=CARTESIAN_POINT('Ctrl Pts',(21.888475877297,4.83127280974582,36.6766506050328));
#55770=CARTESIAN_POINT('Ctrl Pts',(21.9340060321114,4.82705020394334,36.7414672956985));
#55771=CARTESIAN_POINT('Ctrl Pts',(21.979581460821,4.82282339930136,36.8063484382439));
#55772=CARTESIAN_POINT('Ctrl Pts',(22.0218704639672,4.81859659465938,36.8734999077903));
#55773=CARTESIAN_POINT('Ctrl Pts',(22.0606553312402,4.81436979001739,36.9425501968848));
#55774=CARTESIAN_POINT('Ctrl Pts',(22.0994589929802,4.81014093713994,37.0116339465395));
#55775=CARTESIAN_POINT('Ctrl Pts',(22.1347549271662,4.80591208426249,37.0826179284749));
#55776=CARTESIAN_POINT('Ctrl Pts',(22.166372339068,4.80168323138504,37.1551077683561));
#55777=CARTESIAN_POINT('Ctrl Pts',(22.1980465743876,4.79744677833226,37.2277278883651));
#55778=CARTESIAN_POINT('Ctrl Pts',(22.2260289118425,4.79321032527948,37.3018588342739));
#55779=CARTESIAN_POINT('Ctrl Pts',(22.2501975709019,4.7889738722267,37.3770882952895));
#55780=CARTESIAN_POINT('Ctrl Pts',(22.272163799096,4.78512347679256,37.4454622792801));
#55781=CARTESIAN_POINT('Ctrl Pts',(22.2909803129078,4.78127308135842,37.5147432469093));
#55782=CARTESIAN_POINT('Ctrl Pts',(22.3065924823299,4.77742268592428,37.5846151327803));
#55783=CARTESIAN_POINT('Ctrl Pts',(22.3237748190222,4.77318504354679,37.6615142642142));
#55784=CARTESIAN_POINT('Ctrl Pts',(22.3371396104549,4.7689474011693,37.7394179410598));
#55785=CARTESIAN_POINT('Ctrl Pts',(22.3465756872768,4.76470975879181,37.8179131609216));
#55786=CARTESIAN_POINT('Ctrl Pts',(22.35599819465,4.76047821031035,37.8962955015771));
#55787=CARTESIAN_POINT('Ctrl Pts',(22.3615031515985,4.75624666182888,37.9752672343355));
#55788=CARTESIAN_POINT('Ctrl Pts',(22.3630301403667,4.75201511334742,38.0544039846177));
#55789=CARTESIAN_POINT('Ctrl Pts',(22.3645553654206,4.74778845242132,38.1334493297678));
#55790=CARTESIAN_POINT('Ctrl Pts',(22.3621117440479,4.74356179149521,38.2126588473581));
#55791=CARTESIAN_POINT('Ctrl Pts',(22.3556906827349,4.73933513056911,38.291603361599));
#55792=CARTESIAN_POINT('Ctrl Pts',(22.3492736745959,4.73511113764309,38.3704980436024));
#55793=CARTESIAN_POINT('Ctrl Pts',(22.3388842478505,4.73088714471707,38.4491275882775));
#55794=CARTESIAN_POINT('Ctrl Pts',(22.3245658672038,4.72666315179105,38.5270643627503));
#55795=CARTESIAN_POINT('Ctrl Pts',(22.3102520666145,4.7224405100046,38.6049762073851));
#55796=CARTESIAN_POINT('Ctrl Pts',(22.2920118924536,4.71821786821814,38.6821952611433));
#55797=CARTESIAN_POINT('Ctrl Pts',(22.2699402806896,4.71399522643168,38.7583020302285));
#55798=CARTESIAN_POINT('Ctrl Pts',(22.2478688570126,4.7097726206292,38.8344081507568));
#55799=CARTESIAN_POINT('Ctrl Pts',(22.2219661925922,4.70555001482671,38.9094015556345));
#55800=CARTESIAN_POINT('Ctrl Pts',(22.1923772526242,4.70132740902423,38.9828773544928));
#55801=CARTESIAN_POINT('Ctrl Pts',(22.1627588902531,4.69710060438224,39.0564262156023));
#55802=CARTESIAN_POINT('Ctrl Pts',(22.1294471059438,4.69287379974026,39.1284540204798));
#55803=CARTESIAN_POINT('Ctrl Pts',(22.0926350378,4.68864699509828,39.1985759142962));
#55804=CARTESIAN_POINT('Ctrl Pts',(22.0558051311731,4.68441814222083,39.2687317879535));
#55805=CARTESIAN_POINT('Ctrl Pts',(22.0154718005368,4.68018928934339,39.3369795066057));
#55806=CARTESIAN_POINT('Ctrl Pts',(21.9718729040978,4.67596043646594,39.4029611241265));
#55807=CARTESIAN_POINT('Ctrl Pts',(21.9281956508876,4.67172398341317,39.4690613250733));
#55808=CARTESIAN_POINT('Ctrl Pts',(21.8812413836156,4.66748753036039,39.5328869087816));
#55809=CARTESIAN_POINT('Ctrl Pts',(21.8312896869721,4.66325107730761,39.594111282097));
#55810=CARTESIAN_POINT('Ctrl Pts',(21.7858899664306,4.65940068187347,39.6497564278203));
#55811=CARTESIAN_POINT('Ctrl Pts',(21.7380149052619,4.65555028643934,39.7032530836573));
#55812=CARTESIAN_POINT('Ctrl Pts',(21.6878999034291,4.6516998910052,39.7543833766404));
#55813=CARTESIAN_POINT('Ctrl Pts',(21.6327446708958,4.6474622486277,39.810656011497));
#55814=CARTESIAN_POINT('Ctrl Pts',(21.5746687322511,4.64322460625021,39.8642730411299));
#55815=CARTESIAN_POINT('Ctrl Pts',(21.5139580283905,4.63898696387271,39.9149163972955));
#55816=CARTESIAN_POINT('Ctrl Pts',(21.4533346289045,4.63475541539125,39.9654869263275));
#55817=CARTESIAN_POINT('Ctrl Pts',(21.3900843455973,4.6305238669098,40.0130919763475));
#55818=CARTESIAN_POINT('Ctrl Pts',(21.3245302850174,4.62629231842834,40.0574498626968));
#55819=CARTESIAN_POINT('Ctrl Pts',(21.2590519411876,4.62206565750224,40.1017565144625));
#55820=CARTESIAN_POINT('Ctrl Pts',(21.191275494293,4.61783899657613,40.1428231944919));
#55821=CARTESIAN_POINT('Ctrl Pts',(21.121556288238,4.61361233565003,40.1804090783338));
#55822=CARTESIAN_POINT('Ctrl Pts',(21.0518810911186,4.60938834272402,40.2179712367946));
#55823=CARTESIAN_POINT('Ctrl Pts',(20.9802659805198,4.605164349798,40.2520567383726));
#55824=CARTESIAN_POINT('Ctrl Pts',(20.9070933431826,4.60094035687199,40.2824692684329));
#55825=CARTESIAN_POINT('Ctrl Pts',(20.8339441117663,4.59671771508553,40.3128720703584));
#55826=CARTESIAN_POINT('Ctrl Pts',(20.7592387755196,4.59249507329907,40.3396040540671));
#55827=CARTESIAN_POINT('Ctrl Pts',(20.6833809112124,4.58827243151261,40.3625165128879));
#55828=CARTESIAN_POINT('Ctrl Pts',(20.607523693341,4.58404982571011,40.3854287764563));
#55829=CARTESIAN_POINT('Ctrl Pts',(20.5305144160999,4.57982721990762,40.4045214456795));
#55830=CARTESIAN_POINT('Ctrl Pts',(20.4527716386031,4.57560461410512,40.4196957309476));
#55831=CARTESIAN_POINT('Ctrl Pts',(20.3749515558925,4.57137780946314,40.4348851050949));
#55832=CARTESIAN_POINT('Ctrl Pts',(20.2963969771635,4.56715100482115,40.4461482223384));
#55833=CARTESIAN_POINT('Ctrl Pts',(20.2175358765903,4.56292420017917,40.4534376098159));
#55834=CARTESIAN_POINT('Ctrl Pts',(20.1386365613096,4.55869534730172,40.4607305296029));
#55835=CARTESIAN_POINT('Ctrl Pts',(20.0594308972479,4.55446649442428,40.4640458639742));
#55836=CARTESIAN_POINT('Ctrl Pts',(19.9803486284817,4.55023764154683,40.4633883016757));
#55837=CARTESIAN_POINT('Ctrl Pts',(19.9011242315485,4.54600118849405,40.4627295575936));
#55838=CARTESIAN_POINT('Ctrl Pts',(19.8220241421029,4.54176473544127,40.4580836776483));
#55839=CARTESIAN_POINT('Ctrl Pts',(19.7434745164375,4.53752828238849,40.4495074201166));
#55840=CARTESIAN_POINT('Ctrl Pts',(19.6720829262921,4.53367788695437,40.4417126959853));
#55841=CARTESIAN_POINT('Ctrl Pts',(19.6011462188211,4.52982749152024,40.4306719894504));
#55842=CARTESIAN_POINT('Ctrl Pts',(19.5309752971593,4.52597709608612,40.4164641739136));
#55843=CARTESIAN_POINT('Ctrl Pts',(19.4537470549203,4.52173945370862,40.4008274315996));
#55844=CARTESIAN_POINT('Ctrl Pts',(19.3771566697186,4.51750181133113,40.3812950633162));
#55845=CARTESIAN_POINT('Ctrl Pts',(19.3016266064833,4.51326416895363,40.3579337997665));
#55846=CARTESIAN_POINT('Ctrl Pts',(19.2262051584429,4.50903262047217,40.3346061306305));
#55847=CARTESIAN_POINT('Ctrl Pts',(19.1518414484292,4.50480107199071,40.3074606382079));
#55848=CARTESIAN_POINT('Ctrl Pts',(19.0789476509468,4.50056952350924,40.2766150351414));
#55849=CARTESIAN_POINT('Ctrl Pts',(19.0061380478138,4.49634286258314,40.2458050595984));
#55850=CARTESIAN_POINT('Ctrl Pts',(18.9347954128044,4.49211620165704,40.211303648146));
#55851=CARTESIAN_POINT('Ctrl Pts',(18.865315192058,4.48788954073094,40.1732777979629));
#55852=CARTESIAN_POINT('Ctrl Pts',(18.7958788293922,4.48366554780492,40.1352759508813));
#55853=CARTESIAN_POINT('Ctrl Pts',(18.7283029576661,4.47944155487891,40.0937543053894));
#55854=CARTESIAN_POINT('Ctrl Pts',(18.6629604055536,4.47521756195289,40.0489267722987));
#55855=CARTESIAN_POINT('Ctrl Pts',(18.5976387547325,4.47099492016643,40.0041135783071));
#55856=CARTESIAN_POINT('Ctrl Pts',(18.5345493911858,4.46677227837997,39.9559968616279));
#55857=CARTESIAN_POINT('Ctrl Pts',(18.4740367412951,4.46254963659351,39.9048342234074));
#55858=CARTESIAN_POINT('Ctrl Pts',(18.4135246070734,4.45832703079102,39.8536720211782));
#55859=CARTESIAN_POINT('Ctrl Pts',(18.3555894998982,4.45410442498852,39.7994642527695));
#55860=CARTESIAN_POINT('Ctrl Pts',(18.3005421277688,4.44988181918603,39.7425082591608));
#55861=CARTESIAN_POINT('Ctrl Pts',(18.2454400180932,4.44565501454405,39.6854956301268));
#55862=CARTESIAN_POINT('Ctrl Pts',(18.1932317057957,4.44142820990206,39.6257296550541));
#55863=CARTESIAN_POINT('Ctrl Pts',(18.1441899758712,4.43720140526008,39.5635435064402));
#55864=CARTESIAN_POINT('Ctrl Pts',(18.0951244811839,4.43297255238264,39.5013272235084));
#55865=CARTESIAN_POINT('Ctrl Pts',(18.0492288974533,4.42874369950519,39.4366888134454));
#55866=CARTESIAN_POINT('Ctrl Pts',(18.0067332164128,4.42451484662775,39.369991326879));
#55867=CARTESIAN_POINT('Ctrl Pts',(17.964161161321,4.42027839357497,39.3031739703132));
#55868=CARTESIAN_POINT('Ctrl Pts',(17.9250014502555,4.4160419405222,39.2342905515535));
#55869=CARTESIAN_POINT('Ctrl Pts',(17.8894384425492,4.41180548746942,39.1637294548478));
#55870=CARTESIAN_POINT('Ctrl Pts',(17.8571162048682,4.40795509203529,39.0995984185309));
#55871=CARTESIAN_POINT('Ctrl Pts',(17.8277645254185,4.40410469660117,39.0340820649915));
#55872=CARTESIAN_POINT('Ctrl Pts',(17.8014864754825,4.40025430116704,38.9674841343872));
#55873=CARTESIAN_POINT('Ctrl Pts',(17.7688461216759,4.39547166814932,38.8847618615015));
#55874=CARTESIAN_POINT('Ctrl Pts',(17.7408451901343,4.3906890351316,38.8001111929199));
#55875=CARTESIAN_POINT('Ctrl Pts',(17.7176868255926,4.38590640211389,38.7140333987874));
#55876=CARTESIAN_POINT('Ctrl Pts',(17.6946140719736,4.38114144934406,38.6282738136273));
#55877=CARTESIAN_POINT('Ctrl Pts',(17.6763482843133,4.37637649657422,38.5410978479686));
#55878=CARTESIAN_POINT('Ctrl Pts',(17.6630436254456,4.37161154380439,38.4530231498492));
#55879=CARTESIAN_POINT('Ctrl Pts',(17.6498224692232,4.36687649681154,38.365501225788));
#55880=CARTESIAN_POINT('Ctrl Pts',(17.6415004770565,4.36214144981869,38.2770920449245));
#55881=CARTESIAN_POINT('Ctrl Pts',(17.6381808545965,4.35740640282584,38.1883219412461));
#55882=CARTESIAN_POINT('Ctrl Pts',(17.6370989668228,4.35586321846943,38.159391154388));
#55883=CARTESIAN_POINT('Ctrl Pts',(17.6365480176339,4.35432003411302,38.1304221633823));
#55884=CARTESIAN_POINT('Ctrl Pts',(17.6365304347554,4.35277684975661,38.1014335489659));
#55885=CARTESIAN_POINT('',(17.6365308065437,3.55902684968247,38.098047441927));
#55886=CARTESIAN_POINT('Ctrl Pts',(17.6365304347551,4.35277684972829,38.1014335484339));
#55887=CARTESIAN_POINT('Ctrl Pts',(17.6364819365156,4.34852033665357,38.0214752364084));
#55888=CARTESIAN_POINT('Ctrl Pts',(17.6404953682683,4.34426382357884,37.941502555969));
#55889=CARTESIAN_POINT('Ctrl Pts',(17.6485485953399,4.34000731050412,37.8619522476012));
#55890=CARTESIAN_POINT('Ctrl Pts',(17.6566030235322,4.33575016258004,37.7823900744838));
#55891=CARTESIAN_POINT('Ctrl Pts',(17.6686983974036,4.33149301465597,37.7032508543268));
#55892=CARTESIAN_POINT('Ctrl Pts',(17.6847607875601,4.32723586673189,37.6249654432773));
#55893=CARTESIAN_POINT('Ctrl Pts',(17.7013320933604,4.32284383669156,37.5441996622471));
#55894=CARTESIAN_POINT('Ctrl Pts',(17.7221259304715,4.31845180665124,37.4643432170031));
#55895=CARTESIAN_POINT('Ctrl Pts',(17.7470048447539,4.31405977661091,37.385854866755));
#55896=CARTESIAN_POINT('Ctrl Pts',(17.771164415336,4.30979473680437,37.3096359121751));
#55897=CARTESIAN_POINT('Ctrl Pts',(17.7991758114773,4.30552969699783,37.2347074253263));
#55898=CARTESIAN_POINT('Ctrl Pts',(17.8308639407526,4.30126465719129,37.1614696609206));
#55899=CARTESIAN_POINT('Ctrl Pts',(17.8639673263188,4.29680913203407,37.0849609490282));
#55900=CARTESIAN_POINT('Ctrl Pts',(17.9010832925184,4.29235360687685,37.0102980217581));
#55901=CARTESIAN_POINT('Ctrl Pts',(17.9419595175657,4.28789808171962,36.937907140732));
#55902=CARTESIAN_POINT('Ctrl Pts',(17.9828357426131,4.2834425565624,36.8655162597058));
#55903=CARTESIAN_POINT('Ctrl Pts',(18.0274718595266,4.27898703140518,36.7953978564748));
#55904=CARTESIAN_POINT('Ctrl Pts',(18.0755666504899,4.27453150624796,36.7279406994618));
#55905=CARTESIAN_POINT('Ctrl Pts',(18.1213095241425,4.27029386387047,36.6637823124848));
#55906=CARTESIAN_POINT('Ctrl Pts',(18.170350220126,4.26605622149298,36.6017935179042));
#55907=CARTESIAN_POINT('Ctrl Pts',(18.2224556853443,4.26181857911549,36.542332946251));
#55908=CARTESIAN_POINT('Ctrl Pts',(18.2744862208587,4.25758703063405,36.4829578812334));
#55909=CARTESIAN_POINT('Ctrl Pts',(18.3295724668039,4.25335548215261,36.4261041686591));
#55910=CARTESIAN_POINT('Ctrl Pts',(18.3874390030781,4.24912393367117,36.372100271397));
#55911=CARTESIAN_POINT('Ctrl Pts',(18.445238701905,4.24489727274507,36.3181587501275));
#55912=CARTESIAN_POINT('Ctrl Pts',(18.5058119683969,4.24067061181897,36.2670608211206));
#55913=CARTESIAN_POINT('Ctrl Pts',(18.5688451884037,4.23644395089287,36.2190995916464));
#55914=CARTESIAN_POINT('Ctrl Pts',(18.6318386198778,4.23221995796685,36.1711686367948));
#55915=CARTESIAN_POINT('Ctrl Pts',(18.6972885506477,4.22799596504084,36.1263707345436));
#55916=CARTESIAN_POINT('Ctrl Pts',(18.7648477369498,4.22377197211483,36.0849592242384));
#55917=CARTESIAN_POINT('Ctrl Pts',(18.83238531292,4.21954933032837,36.0435609603402));
#55918=CARTESIAN_POINT('Ctrl Pts',(18.9020304052379,4.21532668854191,36.0055471821441));
#55919=CARTESIAN_POINT('Ctrl Pts',(18.9734074409312,4.21110404675546,35.9711274912376));
#55920=CARTESIAN_POINT('Ctrl Pts',(19.0447838683725,4.20688144095298,35.9367080936444));
#55921=CARTESIAN_POINT('Ctrl Pts',(19.1178917869802,4.20265883515051,35.9058829247715));
#55922=CARTESIAN_POINT('Ctrl Pts',(19.1923330681351,4.19843622934803,35.8788146029492));
#55923=CARTESIAN_POINT('Ctrl Pts',(19.2668483715896,4.19420942470606,35.851719365155));
#55924=CARTESIAN_POINT('Ctrl Pts',(19.3426992444218,4.18998262006408,35.8283885970594));
#55925=CARTESIAN_POINT('Ctrl Pts',(19.4194702845906,4.1857558154221,35.8089356860999));
#55926=CARTESIAN_POINT('Ctrl Pts',(19.4962785266604,4.18152696254465,35.7894733486005));
#55927=CARTESIAN_POINT('Ctrl Pts',(19.5740073641273,4.1772981096672,35.7738927039572));
#55928=CARTESIAN_POINT('Ctrl Pts',(19.6522315425966,4.17306925678975,35.7622558863436));
#55929=CARTESIAN_POINT('Ctrl Pts',(19.7305963070566,4.16883280373698,35.7505981548186));
#55930=CARTESIAN_POINT('Ctrl Pts',(19.8094577236358,4.1645963506842,35.7428984583384));
#55931=CARTESIAN_POINT('Ctrl Pts',(19.8883859925219,4.16035989763142,35.7391669363899));
#55932=CARTESIAN_POINT('Ctrl Pts',(19.9601217210574,4.15650950219724,35.7357754589218));
#55933=CARTESIAN_POINT('Ctrl Pts',(20.0319123932756,4.15265910676306,35.7356612213296));
#55934=CARTESIAN_POINT('Ctrl Pts',(20.1034386272148,4.14880871132888,35.738794610522));
#55935=CARTESIAN_POINT('Ctrl Pts',(20.1821584899466,4.1445710689514,35.7422431349798));
#55936=CARTESIAN_POINT('Ctrl Pts',(20.2608534738069,4.14033342657392,35.7496390819302));
#55937=CARTESIAN_POINT('Ctrl Pts',(20.3390958761865,4.13609578419645,35.760982166025));
#55938=CARTESIAN_POINT('Ctrl Pts',(20.4172257629209,4.13186423571501,35.7723089383196));
#55939=CARTESIAN_POINT('Ctrl Pts',(20.4949039005721,4.12763268723357,35.787571508773));
#55940=CARTESIAN_POINT('Ctrl Pts',(20.5717048313383,4.12340113875213,35.8067176303986));
#55941=CARTESIAN_POINT('Ctrl Pts',(20.6484170549086,4.11917447782605,35.8258416377251));
#55942=CARTESIAN_POINT('Ctrl Pts',(20.7242536325234,4.11494781689996,35.8488401693719));
#55943=CARTESIAN_POINT('Ctrl Pts',(20.7987979746695,4.11072115597388,35.8756096932948));
#55944=CARTESIAN_POINT('Ctrl Pts',(20.8732952621039,4.10649716304788,35.9023623194601));
#55945=CARTESIAN_POINT('Ctrl Pts',(20.9465014931087,4.10227317012188,35.9328810551143));
#55946=CARTESIAN_POINT('Ctrl Pts',(21.0180151323997,4.09804917719588,35.9670125103261));
#55947=CARTESIAN_POINT('Ctrl Pts',(21.0895058964376,4.09382653540944,36.001133047821));
#55948=CARTESIAN_POINT('Ctrl Pts',(21.1593047211482,4.089603893623,36.0388638082917));
#55949=CARTESIAN_POINT('Ctrl Pts',(21.2270313408399,4.08538125183656,36.0800038293361));
#55950=CARTESIAN_POINT('Ctrl Pts',(21.2947573833875,4.0811586460341,36.1211434997988));
#55951=CARTESIAN_POINT('Ctrl Pts',(21.3604108561213,4.07693604023163,36.1656921284776));
#55952=CARTESIAN_POINT('Ctrl Pts',(21.4236386282416,4.07271343442917,36.2134042571133));
#55953=CARTESIAN_POINT('Ctrl Pts',(21.4869292722659,4.0684866297872,36.261163829337));
#55954=CARTESIAN_POINT('Ctrl Pts',(21.5477890225405,4.06425982514524,36.3120929020342));
#55955=CARTESIAN_POINT('Ctrl Pts',(21.6058966439289,4.06003302050328,36.3659047287078));
#55956=CARTESIAN_POINT('Ctrl Pts',(21.6640324232525,4.05580416762584,36.4197426316498));
#55957=CARTESIAN_POINT('Ctrl Pts',(21.7194130890371,4.05157531474841,36.4764657355728));
#55958=CARTESIAN_POINT('Ctrl Pts',(21.7717550378619,4.04734646187097,36.5357511301871));
#55959=CARTESIAN_POINT('Ctrl Pts',(21.8241910566387,4.04311000881822,36.5951430736471));
#55960=CARTESIAN_POINT('Ctrl Pts',(21.8735771534998,4.03887355576546,36.657106141579));
#55961=CARTESIAN_POINT('Ctrl Pts',(21.9196708674492,4.0346371027127,36.7212853081341));
#55962=CARTESIAN_POINT('Ctrl Pts',(21.961564173838,4.0307867072784,36.7796159840094));
#55963=CARTESIAN_POINT('Ctrl Pts',(22.0007382177158,4.0269363118441,36.8397766684666));
#55964=CARTESIAN_POINT('Ctrl Pts',(22.0370439895952,4.0230859164098,36.901483322872));
#55965=CARTESIAN_POINT('Ctrl Pts',(22.077001152461,4.01884827403225,36.9693960186319));
#55966=CARTESIAN_POINT('Ctrl Pts',(22.1136334080881,4.01461063165471,37.0394365666303));
#55967=CARTESIAN_POINT('Ctrl Pts',(22.1467081821194,4.01037298927716,37.1112460256861));
#55968=CARTESIAN_POINT('Ctrl Pts',(22.1797353933276,4.00614144079566,37.1829522199216));
#55969=CARTESIAN_POINT('Ctrl Pts',(22.2092150879509,4.00190989231416,37.2564218512728));
#55970=CARTESIAN_POINT('Ctrl Pts',(22.2349595024946,3.99767834383266,37.3312695770889));
#55971=CARTESIAN_POINT('Ctrl Pts',(22.2606741815285,3.9934516829065,37.4060308517147));
#55972=CARTESIAN_POINT('Ctrl Pts',(22.2826620024857,3.98922502198035,37.4821666165824));
#55973=CARTESIAN_POINT('Ctrl Pts',(22.3007830505684,3.98499836105419,37.5592710520814));
#55974=CARTESIAN_POINT('Ctrl Pts',(22.3188926600809,3.98077436812812,37.6363268168581));
#55975=CARTESIAN_POINT('Ctrl Pts',(22.3331402345238,3.97655037520206,37.7143495834492));
#55976=CARTESIAN_POINT('Ctrl Pts',(22.3434358778168,3.97232638227599,37.7929190213299));
#55977=CARTESIAN_POINT('Ctrl Pts',(22.3537282278157,3.96810374048948,37.8714633270011));
#55978=CARTESIAN_POINT('Ctrl Pts',(22.3600710960833,3.96388109870296,37.9505534922494));
#55979=CARTESIAN_POINT('Ctrl Pts',(22.3624260713381,3.95965845691644,38.0297611335359));
#55980=CARTESIAN_POINT('Ctrl Pts',(22.3647810265245,3.95543585111392,38.1089680998404));
#55981=CARTESIAN_POINT('Ctrl Pts',(22.3631481437654,3.95121324531139,38.1882920715844));
#55982=CARTESIAN_POINT('Ctrl Pts',(22.3575411083972,3.94699063950886,38.2673032071336));
#55983=CARTESIAN_POINT('Ctrl Pts',(22.3519284975521,3.94276383486683,38.3463929091162));
#55984=CARTESIAN_POINT('Ctrl Pts',(22.3423338736503,3.9385370302248,38.4251686848449));
#55985=CARTESIAN_POINT('Ctrl Pts',(22.328822919336,3.93431022558277,38.5032049742689));
#55986=CARTESIAN_POINT('Ctrl Pts',(22.31530541785,3.93008137270527,38.5812790787115));
#55987=CARTESIAN_POINT('Ctrl Pts',(22.2978679085859,3.92585251982777,38.6586125251126));
#55988=CARTESIAN_POINT('Ctrl Pts',(22.276626895101,3.92162366695026,38.7347916362105));
#55989=CARTESIAN_POINT('Ctrl Pts',(22.2553477068602,3.91738721389744,38.8111076578648));
#55990=CARTESIAN_POINT('Ctrl Pts',(22.2302515047706,3.91315076084461,38.8862647532822));
#55991=CARTESIAN_POINT('Ctrl Pts',(22.2015041283749,3.90891430779179,38.9598662766083));
#55992=CARTESIAN_POINT('Ctrl Pts',(22.1753764301744,3.9050639123581,39.026760672886));
#55993=CARTESIAN_POINT('Ctrl Pts',(22.1462334058879,3.90121351692441,39.0923701066734));
#55994=CARTESIAN_POINT('Ctrl Pts',(22.1142322151604,3.89736312149072,39.1564149664209));
#55995=CARTESIAN_POINT('Ctrl Pts',(22.0790125593376,3.89312547911326,39.2269010285406));
#55996=CARTESIAN_POINT('Ctrl Pts',(22.040198052094,3.88888783673581,39.2957561993228));
#55997=CARTESIAN_POINT('Ctrl Pts',(21.997963199066,3.88465019435835,39.3625899952391));
#55998=CARTESIAN_POINT('Ctrl Pts',(21.9557890814143,3.88041864587694,39.429327681534));
#55999=CARTESIAN_POINT('Ctrl Pts',(21.9102046341999,3.87618709739552,39.4940493726268));
#56000=CARTESIAN_POINT('Ctrl Pts',(21.8614309025415,3.8719555489141,39.5563878041111));
#56001=CARTESIAN_POINT('Ctrl Pts',(21.8127135058901,3.86772888798804,39.6186542329856));
#56002=CARTESIAN_POINT('Ctrl Pts',(21.7608144326559,3.86350222706197,39.6785425052902));
#56003=CARTESIAN_POINT('Ctrl Pts',(21.7059979511609,3.8592755661359,39.7357143490031));
#56004=CARTESIAN_POINT('Ctrl Pts',(21.6512160715373,3.85505157320992,39.7928501040667));
#56005=CARTESIAN_POINT('Ctrl Pts',(21.593520762525,3.85082758028395,39.8472724965332));
#56006=CARTESIAN_POINT('Ctrl Pts',(21.5332156921468,3.84660358735797,39.8986773146551));
#56007=CARTESIAN_POINT('Ctrl Pts',(21.4729299117075,3.84238094557154,39.9500656897848));
#56008=CARTESIAN_POINT('Ctrl Pts',(21.4100363841272,3.83815830378511,39.998438103464));
#56009=CARTESIAN_POINT('Ctrl Pts',(21.3448735578467,3.83393566199869,40.0435291493324));
#56010=CARTESIAN_POINT('Ctrl Pts',(21.2797112868624,3.82971305619623,40.0886198109498));
#56011=CARTESIAN_POINT('Ctrl Pts',(21.2122801419229,3.82549045039378,40.1304288947869));
#56012=CARTESIAN_POINT('Ctrl Pts',(21.1429481526579,3.82126784459132,40.1687339029551));
#56013=CARTESIAN_POINT('Ctrl Pts',(21.0735472216284,3.81704103994938,40.2070770005374));
#56014=CARTESIAN_POINT('Ctrl Pts',(21.0022420819679,3.81281423530743,40.2419088352182));
#56015=CARTESIAN_POINT('Ctrl Pts',(20.9294254756064,3.80858743066548,40.2730528585825));
#56016=CARTESIAN_POINT('Ctrl Pts',(20.8565735835934,3.80435857778806,40.3042119737949));
#56017=CARTESIAN_POINT('Ctrl Pts',(20.7822092060908,3.80012972491065,40.33167955505));
#56018=CARTESIAN_POINT('Ctrl Pts',(20.706742780571,3.79590087203323,40.3553281541742));
#56019=CARTESIAN_POINT('Ctrl Pts',(20.6311407253468,3.79166441898049,40.3790192550134));
#56020=CARTESIAN_POINT('Ctrl Pts',(20.5544331195204,3.78742796592774,40.3988775419244));
#56021=CARTESIAN_POINT('Ctrl Pts',(20.4770429687982,3.783191512875,40.4148262238925));
#56022=CARTESIAN_POINT('Ctrl Pts',(20.40670519347,3.77934111744054,40.4293215414307));
#56023=CARTESIAN_POINT('Ctrl Pts',(20.3358039824011,3.77549072200609,40.4405879489081));
#56024=CARTESIAN_POINT('Ctrl Pts',(20.2646594402364,3.77164032657164,40.4486050799557));
#56025=CARTESIAN_POINT('Ctrl Pts',(20.1863596572844,3.76740268419425,40.4574285202623));
#56026=CARTESIAN_POINT('Ctrl Pts',(20.1074711708587,3.76316504181687,40.462348604127));
#56027=CARTESIAN_POINT('Ctrl Pts',(20.0284165345531,3.75892739943948,40.4632991646137));
#56028=CARTESIAN_POINT('Ctrl Pts',(19.9494755819169,3.75469585095813,40.4642483581572));
#56029=CARTESIAN_POINT('Ctrl Pts',(19.8703694187606,3.75046430247677,40.4612393589484));
#56030=CARTESIAN_POINT('Ctrl Pts',(19.7915264540029,3.74623275399542,40.4542576795074));
#56031=CARTESIAN_POINT('Ctrl Pts',(19.7127745550468,3.74200609306943,40.4472840640989));
#56032=CARTESIAN_POINT('Ctrl Pts',(19.6342857149448,3.73777943214344,40.4363469282115));
#56033=CARTESIAN_POINT('Ctrl Pts',(19.5564875497691,3.73355277121744,40.4214838244946));
#56034=CARTESIAN_POINT('Ctrl Pts',(19.4787384932196,3.72932877829153,40.406630102832));
#56035=CARTESIAN_POINT('Ctrl Pts',(19.4016797054743,3.72510478536563,40.3878554200163));
#56036=CARTESIAN_POINT('Ctrl Pts',(19.3257316772024,3.72088079243972,40.3652489200465));
#56037=CARTESIAN_POINT('Ctrl Pts',(19.2498079426231,3.71665815065337,40.3426496512764));
#56038=CARTESIAN_POINT('Ctrl Pts',(19.1749947109268,3.71243550886702,40.3162211329756));
#56039=CARTESIAN_POINT('Ctrl Pts',(19.1016988524184,3.70821286708068,40.2861028084593));
#56040=CARTESIAN_POINT('Ctrl Pts',(19.0284036185131,3.70399026127829,40.2559847406015));
#56041=CARTESIAN_POINT('Ctrl Pts',(18.9566261651361,3.69976765547591,40.2221771085391));
#56042=CARTESIAN_POINT('Ctrl Pts',(18.8867534701583,3.69554504967352,40.1848675268936));
#56043=CARTESIAN_POINT('Ctrl Pts',(18.8168112957537,3.69131824503165,40.147520845658));
#56044=CARTESIAN_POINT('Ctrl Pts',(18.7487780775739,3.68709144038978,40.1066654803662));
#56045=CARTESIAN_POINT('Ctrl Pts',(18.6830156997487,3.68286463574791,40.0625347879189));
#56046=CARTESIAN_POINT('Ctrl Pts',(18.6172214546275,3.67863578287057,40.0183827105111));
#56047=CARTESIAN_POINT('Ctrl Pts',(18.5537006181006,3.67440692999322,39.9709524249533));
#56048=CARTESIAN_POINT('Ctrl Pts',(18.4927835180097,3.67017807711588,39.9205188593686));
#56049=CARTESIAN_POINT('Ctrl Pts',(18.4317569365406,3.66594162406321,39.8699946536146));
#56050=CARTESIAN_POINT('Ctrl Pts',(18.3733437879723,3.66170517101055,39.81645670049));
#56051=CARTESIAN_POINT('Ctrl Pts',(18.3178387468338,3.65746871795788,39.7602180456935));
#56052=CARTESIAN_POINT('Ctrl Pts',(18.2673917445024,3.65361832252277,39.7091042821246));
#56053=CARTESIAN_POINT('Ctrl Pts',(18.2193466720729,3.64976792708767,39.6557602601024));
#56054=CARTESIAN_POINT('Ctrl Pts',(18.1738948585642,3.64591753165256,39.6004434189005));
#56055=CARTESIAN_POINT('Ctrl Pts',(18.1241097958789,3.64170005025189,39.5398528242862));
#56056=CARTESIAN_POINT('Ctrl Pts',(18.0772440232761,3.63748256885122,39.4766604032495));
#56057=CARTESIAN_POINT('Ctrl Pts',(18.0335827029836,3.63326508745055,39.4111801763659));
#56058=CARTESIAN_POINT('Ctrl Pts',(17.9899812417688,3.62905338815965,39.3457897219848));
#56059=CARTESIAN_POINT('Ctrl Pts',(17.9495757753076,3.62484168886876,39.2781180754439));
#56060=CARTESIAN_POINT('Ctrl Pts',(17.9126116513043,3.62062998957786,39.2085126623677));
#56061=CARTESIAN_POINT('Ctrl Pts',(17.8756864262643,3.61642272244221,39.1389804981099));
#56062=CARTESIAN_POINT('Ctrl Pts',(17.8421955755532,3.61221545530655,39.0675190224678));
#56063=CARTESIAN_POINT('Ctrl Pts',(17.8123406269042,3.6080081881709,38.9945037217397));
#56064=CARTESIAN_POINT('Ctrl Pts',(17.7825040763327,3.60380351375873,38.9215334166059));
#56065=CARTESIAN_POINT('Ctrl Pts',(17.7562991624995,3.59959883934656,38.8470116224974));
#56066=CARTESIAN_POINT('Ctrl Pts',(17.7338803767706,3.59539416493439,38.7713362005097));
#56067=CARTESIAN_POINT('Ctrl Pts',(17.7114705086883,3.59119116303922,38.6956908803603));
#56068=CARTESIAN_POINT('Ctrl Pts',(17.6928439091955,3.58698816114405,38.6188932980639));
#56069=CARTESIAN_POINT('Ctrl Pts',(17.6781054904817,3.58278515924888,38.5413573694509));
#56070=CARTESIAN_POINT('Ctrl Pts',(17.6633617670978,3.57858064460402,38.4637935340098));
#56071=CARTESIAN_POINT('Ctrl Pts',(17.6525091147608,3.57437612995915,38.385491285794));
#56072=CARTESIAN_POINT('Ctrl Pts',(17.6456012848616,3.57017161531429,38.3068746747539));
#56073=CARTESIAN_POINT('Ctrl Pts',(17.6394978340523,3.56645669345229,38.2374125389932));
#56074=CARTESIAN_POINT('Ctrl Pts',(17.6364732593455,3.56274177159029,38.1677053393348));
#56075=CARTESIAN_POINT('Ctrl Pts',(17.636530806543,3.55902684972829,38.0980474427862));
#56076=CARTESIAN_POINT('',(17.6365300009389,2.76527684969598,38.1000666180705));
#56077=CARTESIAN_POINT('Ctrl Pts',(17.6365308065437,3.55902684968247,38.098047441927));
#56078=CARTESIAN_POINT('Ctrl Pts',(17.6366087562975,3.55399485629477,38.0036933510878));
#56079=CARTESIAN_POINT('Ctrl Pts',(17.6423407577314,3.54896286290708,37.9095808518187));
#56080=CARTESIAN_POINT('Ctrl Pts',(17.6536172651267,3.54393086951938,37.8163126679098));
#56081=CARTESIAN_POINT('Ctrl Pts',(17.6650358770517,3.53883546385085,37.7218691350258));
#56082=CARTESIAN_POINT('Ctrl Pts',(17.6821395347456,3.53374005818232,37.6282913753209));
#56083=CARTESIAN_POINT('Ctrl Pts',(17.7047654113372,3.5286446525138,37.5361838740284));
#56084=CARTESIAN_POINT('Ctrl Pts',(17.7172725445006,3.52582801392036,37.4852686849811));
#56085=CARTESIAN_POINT('Ctrl Pts',(17.7314662234869,3.52301137532692,37.4348023773383));
#56086=CARTESIAN_POINT('Ctrl Pts',(17.7473127371145,3.52019473673349,37.3848842495559));
#56087=CARTESIAN_POINT('Ctrl Pts',(17.7711538709519,3.51595709435636,37.3097822559346));
#56088=CARTESIAN_POINT('Ctrl Pts',(17.7987995848625,3.51171945197924,37.2357328466356));
#56089=CARTESIAN_POINT('Ctrl Pts',(17.8301381585128,3.50748180960211,37.16314887535));
#56090=CARTESIAN_POINT('Ctrl Pts',(17.8614316660644,3.50325026112103,37.0906692826637));
#56091=CARTESIAN_POINT('Ctrl Pts',(17.8964073029588,3.49901871263994,37.0196513697913));
#56092=CARTESIAN_POINT('Ctrl Pts',(17.9349037671089,3.49478716415886,36.950492283715));
#56093=CARTESIAN_POINT('Ctrl Pts',(17.9733557667798,3.49056050323311,36.8814130782928));
#56094=CARTESIAN_POINT('Ctrl Pts',(18.0153202854038,3.48633384230737,36.8141888405654));
#56095=CARTESIAN_POINT('Ctrl Pts',(18.0605888182041,3.48210718138163,36.7491947924201));
#56096=CARTESIAN_POINT('Ctrl Pts',(18.1058287760958,3.47788318845598,36.6842417705434));
#56097=CARTESIAN_POINT('Ctrl Pts',(18.1543683412653,3.47365919553032,36.6215165276491));
#56098=CARTESIAN_POINT('Ctrl Pts',(18.2059547959636,3.46943520260466,36.5613667601491));
#56099=CARTESIAN_POINT('Ctrl Pts',(18.2575247495691,3.46521256081856,36.501236232911));
#56100=CARTESIAN_POINT('Ctrl Pts',(18.3121393523534,3.46098991903246,36.443679900692));
#56101=CARTESIAN_POINT('Ctrl Pts',(18.369505499578,3.45676727724635,36.3890125292705));
#56102=CARTESIAN_POINT('Ctrl Pts',(18.4268711579469,3.45254467144422,36.3343456237064));
#56103=CARTESIAN_POINT('Ctrl Pts',(18.4869879737899,3.44832206564209,36.282567952349));
#56104=CARTESIAN_POINT('Ctrl Pts',(18.549526954012,3.44409945983996,36.233956489317));
#56105=CARTESIAN_POINT('Ctrl Pts',(18.6121281212232,3.43987265519832,36.1852966884241));
#56106=CARTESIAN_POINT('Ctrl Pts',(18.6771558928925,3.43564585055668,36.1398096731329));
#56107=CARTESIAN_POINT('Ctrl Pts',(18.7442497248806,3.43141904591504,36.0977308653836));
#56108=CARTESIAN_POINT('Ctrl Pts',(18.8113760693641,3.42719019303793,36.0556316669813));
#56109=CARTESIAN_POINT('Ctrl Pts',(18.8805700589422,3.42296134016082,36.0169441952786));
#56110=CARTESIAN_POINT('Ctrl Pts',(18.9514460404782,3.41873248728371,35.9818581173889));
#56111=CARTESIAN_POINT('Ctrl Pts',(19.022449401685,3.41449603423126,35.9467089821285));
#56112=CARTESIAN_POINT('Ctrl Pts',(19.0951403638434,3.41025958117881,35.9151743603576));
#56113=CARTESIAN_POINT('Ctrl Pts',(19.169112987984,3.40602312812636,35.8873958297601));
#56114=CARTESIAN_POINT('Ctrl Pts',(19.2363446676346,3.40217273268904,35.8621486887806));
#56115=CARTESIAN_POINT('Ctrl Pts',(19.3046345921318,3.39832233725172,35.840003714446));
#56116=CARTESIAN_POINT('Ctrl Pts',(19.3736697078406,3.3944719418144,35.8210307579909));
#56117=CARTESIAN_POINT('Ctrl Pts',(19.4496479123088,3.39023429943751,35.8001496288712));
#56118=CARTESIAN_POINT('Ctrl Pts',(19.526814106019,3.38599665706063,35.7830329977053));
#56119=CARTESIAN_POINT('Ctrl Pts',(19.604761146044,3.38175901468375,35.7698118768598));
#56120=CARTESIAN_POINT('Ctrl Pts',(19.6825960951665,3.37752746620291,35.756609768505));
#56121=CARTESIAN_POINT('Ctrl Pts',(19.7612092022994,3.37329591772207,35.7472921233669));
#56122=CARTESIAN_POINT('Ctrl Pts',(19.8401795112546,3.36906436924124,35.7419398115661));
#56123=CARTESIAN_POINT('Ctrl Pts',(19.919058607322,3.36483770831576,35.7365936818332));
#56124=CARTESIAN_POINT('Ctrl Pts',(19.9982936199824,3.36061104739028,35.7352038152258));
#56125=CARTESIAN_POINT('Ctrl Pts',(20.077456291198,3.3563843864648,35.7377995504501));
#56126=CARTESIAN_POINT('Ctrl Pts',(20.1565689924686,3.35216039353941,35.7403936471654));
#56127=CARTESIAN_POINT('Ctrl Pts',(20.2356089756367,3.34793640061402,35.746968336733));
#56128=CARTESIAN_POINT('Ctrl Pts',(20.3141470062023,3.34371240768863,35.7575008859353));
#56129=CARTESIAN_POINT('Ctrl Pts',(20.3926599146046,3.33948976590281,35.7680300660637));
#56130=CARTESIAN_POINT('Ctrl Pts',(20.4706707249675,3.33526712411698,35.7825145295162));
#56131=CARTESIAN_POINT('Ctrl Pts',(20.5477558431582,3.33104448233115,35.8008797384247));
#56132=CARTESIAN_POINT('Ctrl Pts',(20.6248403044547,3.3268218765293,35.8192447908309));
#56133=CARTESIAN_POINT('Ctrl Pts',(20.7009986335855,3.32259927072744,35.8414904129059));
#56134=CARTESIAN_POINT('Ctrl Pts',(20.7758194033088,3.31837666492559,35.8674913898599));
#56135=CARTESIAN_POINT('Ctrl Pts',(20.8507145726844,3.31414986028424,35.8935182214483));
#56136=CARTESIAN_POINT('Ctrl Pts',(20.9242690820816,3.30992305564289,35.9233077127991));
#56137=CARTESIAN_POINT('Ctrl Pts',(20.9960891866796,3.30569625100154,35.9566855636468));
#56138=CARTESIAN_POINT('Ctrl Pts',(21.0679440940418,3.30146739812472,35.9900795888162));
#56139=CARTESIAN_POINT('Ctrl Pts',(21.1380625071475,3.2972385452479,36.0270652185019));
#56140=CARTESIAN_POINT('Ctrl Pts',(21.2060753956977,3.29300969237108,36.0674221833365));
#56141=CARTESIAN_POINT('Ctrl Pts',(21.2742105183131,3.28877323931893,36.1078516784808));
#56142=CARTESIAN_POINT('Ctrl Pts',(21.3402321638762,3.28453678626677,36.1516643554831));
#56143=CARTESIAN_POINT('Ctrl Pts',(21.4038006004526,3.28030033321462,36.1985967510628));
#56144=CARTESIAN_POINT('Ctrl Pts',(21.4615762007705,3.27644993777486,36.2412523121402));
#56145=CARTESIAN_POINT('Ctrl Pts',(21.5173255343056,3.27259954233509,36.2864842200498));
#56146=CARTESIAN_POINT('Ctrl Pts',(21.5708195989041,3.26874914689532,36.3340678867525));
#56147=CARTESIAN_POINT('Ctrl Pts',(21.6296937376197,3.26451150451514,36.3864371994057));
#56148=CARTESIAN_POINT('Ctrl Pts',(21.6860566257664,3.26027386213496,36.4418522277241));
#56149=CARTESIAN_POINT('Ctrl Pts',(21.7395767389552,3.25603621975477,36.5000427473879));
#56150=CARTESIAN_POINT('Ctrl Pts',(21.793019888121,3.25180467127062,36.558149586801));
#56151=CARTESIAN_POINT('Ctrl Pts',(21.8436280660461,3.24757312278648,36.6190236490969));
#56152=CARTESIAN_POINT('Ctrl Pts',(21.8911042919975,3.24334157430233,36.6823558282529));
#56153=CARTESIAN_POINT('Ctrl Pts',(21.9385256815969,3.23911491337353,36.7456148569931));
#56154=CARTESIAN_POINT('Ctrl Pts',(21.9828220283333,3.23488825244474,36.8113259872177));
#56155=CARTESIAN_POINT('Ctrl Pts',(22.0237356048506,3.23066159151594,36.879145937239));
#56156=CARTESIAN_POINT('Ctrl Pts',(22.0646233554434,3.22643759858724,36.9469230771944));
#56157=CARTESIAN_POINT('Ctrl Pts',(22.1021323326594,3.22221360565854,37.0168059944153));
#56158=CARTESIAN_POINT('Ctrl Pts',(22.1360479590686,3.21798961272984,37.0884222434933));
#56159=CARTESIAN_POINT('Ctrl Pts',(22.1699527367984,3.2137669709407,37.1600155844961));
#56160=CARTESIAN_POINT('Ctrl Pts',(22.2002662457384,3.20954432915156,37.2333407329763));
#56161=CARTESIAN_POINT('Ctrl Pts',(22.226820435953,3.20532168736243,37.308001775935));
#56162=CARTESIAN_POINT('Ctrl Pts',(22.2533743998814,3.20109908155728,37.3826621826565));
#56163=CARTESIAN_POINT('Ctrl Pts',(22.2761689530424,3.19687647575212,37.4586580190729));
#56164=CARTESIAN_POINT('Ctrl Pts',(22.2950851795987,3.19265386994697,37.5355759933468));
#56165=CARTESIAN_POINT('Ctrl Pts',(22.3140202159142,3.18842706530236,37.612570452673));
#56166=CARTESIAN_POINT('Ctrl Pts',(22.3290691100442,3.18420026065775,37.6904884251957));
#56167=CARTESIAN_POINT('Ctrl Pts',(22.3401637475359,3.17997345601313,37.7689047333189));
#56168=CARTESIAN_POINT('Ctrl Pts',(22.3512637612945,3.17574460313307,37.8473590406107));
#56169=CARTESIAN_POINT('Ctrl Pts',(22.3584056589073,3.171515750253,37.9263116971043));
#56170=CARTESIAN_POINT('Ctrl Pts',(22.3615733409036,3.16728689737293,38.0053332347993));
#56171=CARTESIAN_POINT('Ctrl Pts',(22.3647467159185,3.1630504443176,38.0844967915132));
#56172=CARTESIAN_POINT('Ctrl Pts',(22.3639316086702,3.15881399126226,38.1637290069214));
#56173=CARTESIAN_POINT('Ctrl Pts',(22.3591641018022,3.15457753820693,38.2426014784904));
#56174=CARTESIAN_POINT('Ctrl Pts',(22.3548310462195,3.1507271427967,38.3142864938926));
#56175=CARTESIAN_POINT('Ctrl Pts',(22.3472338078296,3.14687674738647,38.3856741368903));
#56176=CARTESIAN_POINT('Ctrl Pts',(22.3364361322485,3.14302635197624,38.4564500537572));
#56177=CARTESIAN_POINT('Ctrl Pts',(22.3245524988267,3.13878870960212,38.5343441379816));
#56178=CARTESIAN_POINT('Ctrl Pts',(22.3087469503506,3.13455106722801,38.6117895067555));
#56179=CARTESIAN_POINT('Ctrl Pts',(22.2890657087384,3.13031342485389,38.6883609623164));
#56180=CARTESIAN_POINT('Ctrl Pts',(22.269412769524,3.1260818763758,38.7648223051195));
#56181=CARTESIAN_POINT('Ctrl Pts',(22.2458953211595,3.12185032789771,38.8404117801773));
#56182=CARTESIAN_POINT('Ctrl Pts',(22.2186110055028,3.11761877941962,38.9147120025886));
#56183=CARTESIAN_POINT('Ctrl Pts',(22.191358203984,3.11339211849684,38.9889264061917));
#56184=CARTESIAN_POINT('Ctrl Pts',(22.1603473421512,3.10916545757407,39.0618540785945));
#56185=CARTESIAN_POINT('Ctrl Pts',(22.1257260977279,3.10493879665129,39.1330919602526));
#56186=CARTESIAN_POINT('Ctrl Pts',(22.0911267073128,3.10071480372859,39.2042848743403));
#56187=CARTESIAN_POINT('Ctrl Pts',(22.0529216622112,3.09649081080588,39.2737896943469));
#56188=CARTESIAN_POINT('Ctrl Pts',(22.0113065926847,3.09226681788317,39.3412236829528));
#56189=CARTESIAN_POINT('Ctrl Pts',(21.969704834678,3.08804417609999,39.4086361012746));
#56190=CARTESIAN_POINT('Ctrl Pts',(21.9246954643149,3.08382153431681,39.4739786049584));
#56191=CARTESIAN_POINT('Ctrl Pts',(21.8765191246263,3.07959889253363,39.5368947128485));
#56192=CARTESIAN_POINT('Ctrl Pts',(21.8283431954803,3.0753762867344,39.5998102845884));
#56193=CARTESIAN_POINT('Ctrl Pts',(21.7770006367988,3.07115368093516,39.6602991303254));
#56194=CARTESIAN_POINT('Ctrl Pts',(21.7227734155927,3.06693107513593,39.7180365259867));
#56195=CARTESIAN_POINT('Ctrl Pts',(21.6684922723741,3.06270427049713,39.7758313340785));
#56196=CARTESIAN_POINT('Ctrl Pts',(21.611321058605,3.05847746585832,39.830868884503));
#56197=CARTESIAN_POINT('Ctrl Pts',(21.5515793648724,3.05425066121952,39.8828605989819));
#56198=CARTESIAN_POINT('Ctrl Pts',(21.4918087213613,3.05002180834521,39.9348775077352));
#56199=CARTESIAN_POINT('Ctrl Pts',(21.4294654856099,3.04579295547091,39.9838453503306));
#56200=CARTESIAN_POINT('Ctrl Pts',(21.3649011608889,3.0415641025966,40.0295168467531));
#56201=CARTESIAN_POINT('Ctrl Pts',(21.3002207999264,3.03732764954688,40.0752704248642));
#56202=CARTESIAN_POINT('Ctrl Pts',(21.2333117708055,3.03309119649715,40.117715567856));
#56203=CARTESIAN_POINT('Ctrl Pts',(21.1645530875906,3.02885474344742,40.1566493495692));
#56204=CARTESIAN_POINT('Ctrl Pts',(21.1020602147053,3.02500434798401,40.1920351911499));
#56205=CARTESIAN_POINT('Ctrl Pts',(21.0380399871679,3.02115395252059,40.2245209451278));
#56206=CARTESIAN_POINT('Ctrl Pts',(20.9727908051473,3.01730355705717,40.2539889717269));
#56207=CARTESIAN_POINT('Ctrl Pts',(20.9009792987033,3.01306591468266,40.286420694493));
#56208=CARTESIAN_POINT('Ctrl Pts',(20.827409367394,3.00882827230814,40.3153181980759));
#56209=CARTESIAN_POINT('Ctrl Pts',(20.7524628560726,3.00459062993362,40.3404888062945));
#56210=CARTESIAN_POINT('Ctrl Pts',(20.6776241207765,3.00035908145519,40.3656232181905));
#56211=CARTESIAN_POINT('Ctrl Pts',(20.6014131774329,2.99612753297676,40.3870412300264));
#56212=CARTESIAN_POINT('Ctrl Pts',(20.5242333066394,2.99189598449833,40.4045975529602));
#56213=CARTESIAN_POINT('Ctrl Pts',(20.4471425807292,2.9876693235753,40.4221335978558));
#56214=CARTESIAN_POINT('Ctrl Pts',(20.3690856061609,2.98344266265227,40.4358167142507));
#56215=CARTESIAN_POINT('Ctrl Pts',(20.2904808827541,2.97921600172925,40.4455513845692));
#56216=CARTESIAN_POINT('Ctrl Pts',(20.2119257770988,2.97499200880635,40.4552799100603));
#56217=CARTESIAN_POINT('Ctrl Pts',(20.1328240728952,2.97076801588344,40.461064879115));
#56218=CARTESIAN_POINT('Ctrl Pts',(20.0536033245773,2.96654402296054,40.4628620620964));
#56219=CARTESIAN_POINT('Ctrl Pts',(19.9744079168059,2.96232138117722,40.4646586702082));
#56220=CARTESIAN_POINT('Ctrl Pts',(19.8950940088524,2.9580987393939,40.4624700146794));
#56221=CARTESIAN_POINT('Ctrl Pts',(19.8160916317561,2.95387609761059,40.4563039177894));
#56222=CARTESIAN_POINT('Ctrl Pts',(19.7370899278926,2.94965349181126,40.450137873445));
#56223=CARTESIAN_POINT('Ctrl Pts',(19.6584002168479,2.94543088601194,40.4399944930337));
#56224=CARTESIAN_POINT('Ctrl Pts',(19.5804483837839,2.94120828021262,40.4259335506911));
#56225=CARTESIAN_POINT('Ctrl Pts',(19.5024190376273,2.93698147557381,40.4118586265461));
#56226=CARTESIAN_POINT('Ctrl Pts',(19.4251294974711,2.93275467093501,40.3938584425738));
#56227=CARTESIAN_POINT('Ctrl Pts',(19.3489958067916,2.9285278662962,40.3720440095485));
#56228=CARTESIAN_POINT('Ctrl Pts',(19.2728252230598,2.92429901342194,40.3502190056312));
#56229=CARTESIAN_POINT('Ctrl Pts',(19.1978120487375,2.92007016054768,40.3245762224212));
#56230=CARTESIAN_POINT('Ctrl Pts',(19.1243550547343,2.91584130767342,40.2952759213208));
#56231=CARTESIAN_POINT('Ctrl Pts',(19.0507660424153,2.91160485462381,40.2659229611582));
#56232=CARTESIAN_POINT('Ctrl Pts',(18.9787392258186,2.90736840157421,40.2328995447266));
#56233=CARTESIAN_POINT('Ctrl Pts',(18.9086511439443,2.9031319485246,40.1964131547207));
#56234=CARTESIAN_POINT('Ctrl Pts',(18.8449500172609,2.89928155306243,40.1632516800472));
#56235=CARTESIAN_POINT('Ctrl Pts',(18.782850286663,2.89543115760026,40.1272303363376));
#56236=CARTESIAN_POINT('Ctrl Pts',(18.7226130661596,2.89158076213809,40.0885354063114));
#56237=CARTESIAN_POINT('Ctrl Pts',(18.6563175902903,2.88734311974163,40.0459487999178));
#56238=CARTESIAN_POINT('Ctrl Pts',(18.5920296832405,2.88310547734517,39.9999633067943));
#56239=CARTESIAN_POINT('Ctrl Pts',(18.530118826536,2.87886783494872,39.950794363725));
#56240=CARTESIAN_POINT('Ctrl Pts',(18.4682970000719,2.87463628644825,39.9016961275245));
#56241=CARTESIAN_POINT('Ctrl Pts',(18.4088457995984,2.87040473794778,39.8494238218444));
#56242=CARTESIAN_POINT('Ctrl Pts',(18.3521066231758,2.86617318944731,39.7942366598321));
#56243=CARTESIAN_POINT('Ctrl Pts',(18.2954329820687,2.8619465285022,39.7391132405158));
#56244=CARTESIAN_POINT('Ctrl Pts',(18.2414654743572,2.85771986755709,39.6810819806166));
#56245=CARTESIAN_POINT('Ctrl Pts',(18.1905120309623,2.85349320661199,39.6204419524624));
#56246=CARTESIAN_POINT('Ctrl Pts',(18.1395907509687,2.84926921366698,39.5598402021837));
#56247=CARTESIAN_POINT('Ctrl Pts',(18.091680059675,2.84504522072198,39.4966333101958));
#56248=CARTESIAN_POINT('Ctrl Pts',(18.047049792961,2.84082122777698,39.4311558622965));
#56249=CARTESIAN_POINT('Ctrl Pts',(18.0024338022463,2.83659858597157,39.3656993588386));
#56250=CARTESIAN_POINT('Ctrl Pts',(17.9610964162059,2.83237594416617,39.2979741288062));
#56251=CARTESIAN_POINT('Ctrl Pts',(17.9232651541579,2.82815330236077,39.228345169248));
#56252=CARTESIAN_POINT('Ctrl Pts',(17.8854342144962,2.8239306965394,39.1587168030461));
#56253=CARTESIAN_POINT('Ctrl Pts',(17.8511095619611,2.81970809071804,39.0871851521587));
#56254=CARTESIAN_POINT('Ctrl Pts',(17.8204728783943,2.81548548489668,39.0141400150334));
#56255=CARTESIAN_POINT('Ctrl Pts',(17.7898057305799,2.81125868023606,38.9410222438991));
#56256=CARTESIAN_POINT('Ctrl Pts',(17.7628340587385,2.80703187557543,38.8663884136422));
#56257=CARTESIAN_POINT('Ctrl Pts',(17.7396912067772,2.80280507091481,38.7906479567622));
#56258=CARTESIAN_POINT('Ctrl Pts',(17.716537140196,2.79857621801882,38.714870797386));
#56259=CARTESIAN_POINT('Ctrl Pts',(17.6972157040253,2.79434736512283,38.637986398329));
#56260=CARTESIAN_POINT('Ctrl Pts',(17.6818095253449,2.79011851222684,38.5604165115612));
#56261=CARTESIAN_POINT('Ctrl Pts',(17.6663756583868,2.78588205915591,38.482707214716));
#56262=CARTESIAN_POINT('Ctrl Pts',(17.6548711769025,2.78164560608498,38.4043104334678));
#56263=CARTESIAN_POINT('Ctrl Pts',(17.6473269939418,2.77740915301404,38.3256549743858));
#56264=CARTESIAN_POINT('Ctrl Pts',(17.6404702942772,2.77355875774903,38.2541671986106));
#56265=CARTESIAN_POINT('Ctrl Pts',(17.6368843425059,2.76970836248401,38.1824660538048));
#56266=CARTESIAN_POINT('Ctrl Pts',(17.6365550057291,2.765857967219,38.1108719802996));
#56267=CARTESIAN_POINT('Ctrl Pts',(17.6365384374421,2.76566426138876,38.107270222949));
#56268=CARTESIAN_POINT('Ctrl Pts',(17.6365301024624,2.76547055555852,38.1036684276956));
#56269=CARTESIAN_POINT('Ctrl Pts',(17.6365300009389,2.76527684972828,38.1000666186711));
#56270=CARTESIAN_POINT('',(17.6365307642293,1.97152684977754,38.1019006486528));
#56271=CARTESIAN_POINT('Ctrl Pts',(17.6365300009389,2.76527684969598,38.1000666180705));
#56272=CARTESIAN_POINT('Ctrl Pts',(17.6365277817899,2.7610426970283,38.0213358474423));
#56273=CARTESIAN_POINT('Ctrl Pts',(17.6404638294913,2.75680854436061,37.9424559890261));
#56274=CARTESIAN_POINT('Ctrl Pts',(17.6483568759924,2.75257439169293,37.8638537355627));
#56275=CARTESIAN_POINT('Ctrl Pts',(17.656238569863,2.74834632904014,37.7853645363352));
#56276=CARTESIAN_POINT('Ctrl Pts',(17.6680659139453,2.74411826638735,37.7071526125758));
#56277=CARTESIAN_POINT('Ctrl Pts',(17.6838056298472,2.73989020373455,37.6296447294093));
#56278=CARTESIAN_POINT('Ctrl Pts',(17.6995272028678,2.73566701469187,37.5522261881552));
#56279=CARTESIAN_POINT('Ctrl Pts',(17.7191520931642,2.73144382564918,37.4755105327649));
#56280=CARTESIAN_POINT('Ctrl Pts',(17.7425953940227,2.72722063660649,37.3999179435147));
#56281=CARTESIAN_POINT('Ctrl Pts',(17.7660239611144,2.72300010177547,37.3243728630856));
#56282=CARTESIAN_POINT('Ctrl Pts',(17.7932660368616,2.71877956694445,37.2499498952732));
#56283=CARTESIAN_POINT('Ctrl Pts',(17.8241862410376,2.71455903211343,37.1770563791814));
#56284=CARTESIAN_POINT('Ctrl Pts',(17.8550966835537,2.71033982972592,37.1041858759295));
#56285=CARTESIAN_POINT('Ctrl Pts',(17.8896827653708,2.70612062733841,37.032844297629));
#56286=CARTESIAN_POINT('Ctrl Pts',(17.9277606465776,2.7019014249509,36.963419821118));
#56287=CARTESIAN_POINT('Ctrl Pts',(17.9658384161765,2.69768223493006,36.893995548093));
#56288=CARTESIAN_POINT('Ctrl Pts',(18.0074077376034,2.69346304490922,36.8264887767218));
#56289=CARTESIAN_POINT('Ctrl Pts',(18.0522391338228,2.68924385488838,36.7612625167388));
#56290=CARTESIAN_POINT('Ctrl Pts',(18.0971152043896,2.68502046045775,36.6959712589898));
#56291=CARTESIAN_POINT('Ctrl Pts',(18.1452595758028,2.68079706602713,36.6329654395846));
#56292=CARTESIAN_POINT('Ctrl Pts',(18.1964001430807,2.67657367159651,36.5725779898729));
#56293=CARTESIAN_POINT('Ctrl Pts',(18.2475658828021,2.67234819832392,36.5121608162112));
#56294=CARTESIAN_POINT('Ctrl Pts',(18.3017304344297,2.66812272505133,36.4543649224505));
#56295=CARTESIAN_POINT('Ctrl Pts',(18.358583940748,2.66389725177874,36.3994872063611));
#56296=CARTESIAN_POINT('Ctrl Pts',(18.4155388995487,2.6596642383423,36.3445115634966));
#56297=CARTESIAN_POINT('Ctrl Pts',(18.4751920449262,2.65543122490587,36.2924648114215));
#56298=CARTESIAN_POINT('Ctrl Pts',(18.5371996944003,2.65119821146943,36.2436041082686));
#56299=CARTESIAN_POINT('Ctrl Pts',(18.5912189776084,2.64751053174626,36.2010380670825));
#56300=CARTESIAN_POINT('Ctrl Pts',(18.6470245249846,2.6438228520231,36.1608894951088));
#56301=CARTESIAN_POINT('Ctrl Pts',(18.704372763647,2.64013517229993,36.1233006031972));
#56302=CARTESIAN_POINT('Ctrl Pts',(18.7702736401,2.63589752993283,36.0801058865043));
#56303=CARTESIAN_POINT('Ctrl Pts',(18.8384606739486,2.63165988756574,36.040129282216));
#56304=CARTESIAN_POINT('Ctrl Pts',(18.9085865914612,2.62742224519864,36.0036204512156));
#56305=CARTESIAN_POINT('Ctrl Pts',(18.9786116651466,2.62319069672792,35.9671641213499));
#56306=CARTESIAN_POINT('Ctrl Pts',(19.0505696730441,2.6189591482572,35.934165876144));
#56307=CARTESIAN_POINT('Ctrl Pts',(19.124084803758,2.61472759978647,35.9048318948444));
#56308=CARTESIAN_POINT('Ctrl Pts',(19.1975150224579,2.61050093887155,35.8755317951065));
#56309=CARTESIAN_POINT('Ctrl Pts',(19.272498356674,2.60627427795662,35.8498877214283));
#56310=CARTESIAN_POINT('Ctrl Pts',(19.3486362280133,2.6020476170417,35.8280590506258));
#56311=CARTESIAN_POINT('Ctrl Pts',(19.4247260387507,2.59782362412713,35.806244158762));
#56312=CARTESIAN_POINT('Ctrl Pts',(19.5019684906233,2.59359963121257,35.7882400182171));
#56313=CARTESIAN_POINT('Ctrl Pts',(19.5799480923609,2.589375638298,35.7741567473734));
#56314=CARTESIAN_POINT('Ctrl Pts',(19.6579027505566,2.58515299652323,35.7600779813828));
#56315=CARTESIAN_POINT('Ctrl Pts',(19.7365936293992,2.58093035474847,35.7499176777952));
#56316=CARTESIAN_POINT('Ctrl Pts',(19.8155947041848,2.57670771297371,35.7437349198837));
#56317=CARTESIAN_POINT('Ctrl Pts',(19.8945951057447,2.57248510718315,35.7375522146601));
#56318=CARTESIAN_POINT('Ctrl Pts',(19.9739052305367,2.56826250139259,35.7353470228679));
#56319=CARTESIAN_POINT('Ctrl Pts',(20.053095078038,2.56403989560204,35.7371264626332));
#56320=CARTESIAN_POINT('Ctrl Pts',(20.1323636696737,2.55981309097225,35.7389076718229));
#56321=CARTESIAN_POINT('Ctrl Pts',(20.211511275372,2.55558628634247,35.744681416536));
#56322=CARTESIAN_POINT('Ctrl Pts',(20.290109656557,2.55135948171269,35.7544026713708));
#56323=CARTESIAN_POINT('Ctrl Pts',(20.3687461251371,2.54713062884761,35.764128636955));
#56324=CARTESIAN_POINT('Ctrl Pts',(20.4468323766782,2.54290177598254,35.7778058423894));
#56325=CARTESIAN_POINT('Ctrl Pts',(20.5239495837537,2.53867292311746,35.7953379261627));
#56326=CARTESIAN_POINT('Ctrl Pts',(20.6012053873477,2.53443647007719,35.8129015189319));
#56327=CARTESIAN_POINT('Ctrl Pts',(20.6774882142496,2.53020001703692,35.8343337058813));
#56328=CARTESIAN_POINT('Ctrl Pts',(20.7523938625888,2.52596356399665,35.8594880235895));
#56329=CARTESIAN_POINT('Ctrl Pts',(20.8204735442091,2.52211316845805,35.8823500904553));
#56330=CARTESIAN_POINT('Ctrl Pts',(20.8874155900921,2.51826277291945,35.908286097158));
#56331=CARTESIAN_POINT('Ctrl Pts',(20.9529331154744,2.51441237738085,35.9371525901413));
#56332=CARTESIAN_POINT('Ctrl Pts',(21.0250399543103,2.51017473487319,35.9689222814592));
#56333=CARTESIAN_POINT('Ctrl Pts',(21.0956916594874,2.50593709236553,36.0043614892623));
#56334=CARTESIAN_POINT('Ctrl Pts',(21.1644897651357,2.50169944985788,36.0433147961357));
#56335=CARTESIAN_POINT('Ctrl Pts',(21.2331889364188,2.49746790124579,36.0822120866312));
#56336=CARTESIAN_POINT('Ctrl Pts',(21.3000393971506,2.49323635263371,36.1246132115312));
#56337=CARTESIAN_POINT('Ctrl Pts',(21.3646636227348,2.48900480402162,36.1703151455006));
#56338=CARTESIAN_POINT('Ctrl Pts',(21.4292132055571,2.48477814296483,36.2159642924765));
#56339=CARTESIAN_POINT('Ctrl Pts',(21.491541282378,2.48055148190803,36.2649064027758));
#56340=CARTESIAN_POINT('Ctrl Pts',(21.5512971967595,2.47632482085123,36.3168938763422));
#56341=CARTESIAN_POINT('Ctrl Pts',(21.6110153913467,2.47210082779454,36.3688485337961));
#56342=CARTESIAN_POINT('Ctrl Pts',(21.6681642934807,2.46787683473784,36.423844432027));
#56343=CARTESIAN_POINT('Ctrl Pts',(21.7224253617482,2.46365284168114,36.4815929701998));
#56344=CARTESIAN_POINT('Ctrl Pts',(21.7766690733852,2.45943019976421,36.5393230361959));
#56345=CARTESIAN_POINT('Ctrl Pts',(21.8280264647536,2.45520755784727,36.5998036522649));
#56346=CARTESIAN_POINT('Ctrl Pts',(21.8762160724176,2.45098491593033,36.6627096011933));
#56347=CARTESIAN_POINT('Ctrl Pts',(21.9244052694213,2.44676230999774,36.7256150140523));
#56348=CARTESIAN_POINT('Ctrl Pts',(21.9694264524563,2.44253970406515,36.7909453456766));
#56349=CARTESIAN_POINT('Ctrl Pts',(22.0110395857854,2.43831709813256,36.8583437571919));
#56350=CARTESIAN_POINT('Ctrl Pts',(22.0526940980185,2.43409029336196,36.925809187751));
#56351=CARTESIAN_POINT('Ctrl Pts',(22.090933544425,2.42986348859136,36.9953464061484));
#56352=CARTESIAN_POINT('Ctrl Pts',(22.1255625898733,2.42563668382077,37.0665716679754));
#56353=CARTESIAN_POINT('Ctrl Pts',(22.1602084159447,2.42140783081532,37.1378314443048));
#56354=CARTESIAN_POINT('Ctrl Pts',(22.1912401720431,2.41717897780988,37.2107804616895));
#56355=CARTESIAN_POINT('Ctrl Pts',(22.2185107100584,2.41295012480443,37.28501492636));
#56356=CARTESIAN_POINT('Ctrl Pts',(22.2458302591889,2.40871367162619,37.3593828065828));
#56357=CARTESIAN_POINT('Ctrl Pts',(22.2693749440146,2.40447721844794,37.4350403014924));
#56358=CARTESIAN_POINT('Ctrl Pts',(22.2890476065036,2.40024076526969,37.5115686139742));
#56359=CARTESIAN_POINT('Ctrl Pts',(22.3069275413742,2.39639037100038,37.5811230651677));
#56360=CARTESIAN_POINT('Ctrl Pts',(22.3216095942983,2.39253997673108,37.6513964447735));
#56361=CARTESIAN_POINT('Ctrl Pts',(22.33305794227,2.38868958246177,37.7220700079234));
#56362=CARTESIAN_POINT('Ctrl Pts',(22.3456576913936,2.38445194031984,37.7998514631659));
#56363=CARTESIAN_POINT('Ctrl Pts',(22.3543871217923,2.38021429817791,37.8784097021737));
#56364=CARTESIAN_POINT('Ctrl Pts',(22.3591597089427,2.37597665603598,37.9573258656897));
#56365=CARTESIAN_POINT('Ctrl Pts',(22.3639254329255,2.3717451077898,38.0361285446649));
#56366=CARTESIAN_POINT('Ctrl Pts',(22.3647455855991,2.36751355954361,38.1152876619303));
#56367=CARTESIAN_POINT('Ctrl Pts',(22.3615849782599,2.36328201129742,38.1943760104973));
#56368=CARTESIAN_POINT('Ctrl Pts',(22.3584280215084,2.35905535060505,38.2733730098612));
#56369=CARTESIAN_POINT('Ctrl Pts',(22.3512994605252,2.35482868991268,38.3522989369354));
#56370=CARTESIAN_POINT('Ctrl Pts',(22.3402161241884,2.35060202922031,38.4307248599495));
#56371=CARTESIAN_POINT('Ctrl Pts',(22.3291397839965,2.346378036527,38.5091012780936));
#56372=CARTESIAN_POINT('Ctrl Pts',(22.3141136889076,2.34215404383368,38.5869778556978));
#56373=CARTESIAN_POINT('Ctrl Pts',(22.2952065433738,2.33793005114037,38.6639302830618));
#56374=CARTESIAN_POINT('Ctrl Pts',(22.2763054457119,2.33370740958526,38.7408580954768));
#56375=CARTESIAN_POINT('Ctrl Pts',(22.2535258746306,2.32948476803015,38.8168618897691));
#56376=CARTESIAN_POINT('Ctrl Pts',(22.2269874337358,2.32526212647504,38.8915285281548));
#56377=CARTESIAN_POINT('Ctrl Pts',(22.2004492189825,2.32103952090225,38.9661945302851));
#56378=CARTESIAN_POINT('Ctrl Pts',(22.1701523564412,2.31681691532946,39.0395229579402));
#56379=CARTESIAN_POINT('Ctrl Pts',(22.1362655266727,2.31259430975666,39.1111182128958));
#56380=CARTESIAN_POINT('Ctrl Pts',(22.102345000766,2.30836750534019,39.1827846602182));
#56381=CARTESIAN_POINT('Ctrl Pts',(22.0648275780222,2.30414070092371,39.2527140676081));
#56382=CARTESIAN_POINT('Ctrl Pts',(22.0239288413109,2.29991389650723,39.3205336890925));
#56383=CARTESIAN_POINT('Ctrl Pts',(21.9830102857687,2.29568504385335,39.38838617481));
#56384=CARTESIAN_POINT('Ctrl Pts',(21.9387074144306,2.29145619119947,39.4541264487122));
#56385=CARTESIAN_POINT('Ctrl Pts',(21.8912788588317,2.2872273385456,39.5174112737792));
#56386=CARTESIAN_POINT('Ctrl Pts',(21.8437650636547,2.28299088571053,39.5808098356387));
#56387=CARTESIAN_POINT('Ctrl Pts',(21.7931146601845,2.27875443287547,39.6417437697455));
#56388=CARTESIAN_POINT('Ctrl Pts',(21.7396260771504,2.27451798004041,39.6999036072834));
#56389=CARTESIAN_POINT('Ctrl Pts',(21.6910117494637,2.27066758254117,39.7527635119563));
#56390=CARTESIAN_POINT('Ctrl Pts',(21.6400536112878,2.26681718504193,39.8033321516061));
#56391=CARTESIAN_POINT('Ctrl Pts',(21.5869995482967,2.26296678754269,39.8514059708149));
#56392=CARTESIAN_POINT('Ctrl Pts',(21.5286096947538,2.25872914515703,39.9043147039938));
#56393=CARTESIAN_POINT('Ctrl Pts',(21.4674614702668,2.25449150277136,39.9543995829428));
#56394=CARTESIAN_POINT('Ctrl Pts',(21.4038591439485,2.2502538603857,40.0013600250485));
#56395=CARTESIAN_POINT('Ctrl Pts',(21.3403482803063,2.24602231189841,40.0482529361698));
#56396=CARTESIAN_POINT('Ctrl Pts',(21.274390697293,2.24179076341113,40.0920300571151));
#56397=CARTESIAN_POINT('Ctrl Pts',(21.206325610573,2.23755921492384,40.1324293252597));
#56398=CARTESIAN_POINT('Ctrl Pts',(21.1383391409639,2.2333325539954,40.1727819311007));
#56399=CARTESIAN_POINT('Ctrl Pts',(21.0682504061431,2.22910589306696,40.2097641993818));
#56400=CARTESIAN_POINT('Ctrl Pts',(20.9964283836556,2.22487923213852,40.2431567644821));
#56401=CARTESIAN_POINT('Ctrl Pts',(20.924651697503,2.2206552392123,40.2765282511379));
#56402=CARTESIAN_POINT('Ctrl Pts',(20.8511443193274,2.21643124628608,40.3063143351266));
#56403=CARTESIAN_POINT('Ctrl Pts',(20.776299587088,2.21220725335986,40.3323416835214));
#56404=CARTESIAN_POINT('Ctrl Pts',(20.7014787956642,2.2079846115753,40.3583607064678));
#56405=CARTESIAN_POINT('Ctrl Pts',(20.6253219421162,2.20376196979073,40.380623227526));
#56406=CARTESIAN_POINT('Ctrl Pts',(20.5482406988636,2.19953932800617,40.3990046926898));
#56407=CARTESIAN_POINT('Ctrl Pts',(20.4711601125105,2.19531672220768,40.4173860012036));
#56408=CARTESIAN_POINT('Ctrl Pts',(20.3931556084345,2.19109411640919,40.4318862122382));
#56409=CARTESIAN_POINT('Ctrl Pts',(20.3146508600194,2.18687151061071,40.4424314882594));
#56410=CARTESIAN_POINT('Ctrl Pts',(20.2360680487678,2.18264470597593,40.4529872501961));
#56411=CARTESIAN_POINT('Ctrl Pts',(20.1569844652424,2.17841790134116,40.4595801590354));
#56412=CARTESIAN_POINT('Ctrl Pts',(20.0778301434093,2.17419109670638,40.4621881613616));
#56413=CARTESIAN_POINT('Ctrl Pts',(19.998637464812,2.16996224383792,40.4647974274789));
#56414=CARTESIAN_POINT('Ctrl Pts',(19.9193744489222,2.16573339096945,40.4634179484446));
#56415=CARTESIAN_POINT('Ctrl Pts',(19.840469808524,2.16150453810098,40.4580798457448));
#56416=CARTESIAN_POINT('Ctrl Pts',(19.7614233592487,2.15726808506003,40.4527321493081));
#56417=CARTESIAN_POINT('Ctrl Pts',(19.6827370390208,2.15303163201909,40.4434116689938));
#56418=CARTESIAN_POINT('Ctrl Pts',(19.6048328966024,2.14879517897814,40.4302002920977));
#56419=CARTESIAN_POINT('Ctrl Pts',(19.534027967875,2.14494478352663,40.4181928356201));
#56420=CARTESIAN_POINT('Ctrl Pts',(19.4638692871082,2.14109438807512,40.4029720189242));
#56421=CARTESIAN_POINT('Ctrl Pts',(19.3946625428323,2.13724399262361,40.3846349826285));
#56422=CARTESIAN_POINT('Ctrl Pts',(19.3184954332277,2.13300634937881,40.3644537261921));
#56423=CARTESIAN_POINT('Ctrl Pts',(19.2431956849316,2.128768706134,40.3404214360633));
#56424=CARTESIAN_POINT('Ctrl Pts',(19.1691810715687,2.12453106288919,40.3126297360969));
#56425=CARTESIAN_POINT('Ctrl Pts',(19.0952728940357,2.12029951353659,40.2848780016524));
#56426=CARTESIAN_POINT('Ctrl Pts',(19.0226466165638,2.11606796418399,40.253377756956));
#56427=CARTESIAN_POINT('Ctrl Pts',(18.951706722241,2.11183641483139,40.2182709091864));
#56428=CARTESIAN_POINT('Ctrl Pts',(18.880848765411,2.1076097530325,40.1832046107736));
#56429=CARTESIAN_POINT('Ctrl Pts',(18.8116737389392,2.10338309123362,40.1445401944964));
#56430=CARTESIAN_POINT('Ctrl Pts',(18.7445665092171,2.09915642943474,40.1024677753014));
#56431=CARTESIAN_POINT('Ctrl Pts',(18.6775016396513,2.09493243563535,40.0604219135171));
#56432=CARTESIAN_POINT('Ctrl Pts',(18.6125023721764,2.09070844183596,40.0149725671351));
#56433=CARTESIAN_POINT('Ctrl Pts',(18.5499282180774,2.08648444803657,39.9663553434895));
#56434=CARTESIAN_POINT('Ctrl Pts',(18.4873740797401,2.08226180537735,39.917753671165));
#56435=CARTESIAN_POINT('Ctrl Pts',(18.4272438842452,2.07803916271813,39.8659864212264));
#56436=CARTESIAN_POINT('Ctrl Pts',(18.3698662039139,2.07381652005892,39.8113311332872));
#56437=CARTESIAN_POINT('Ctrl Pts',(18.3124890125612,2.06959391338551,39.7566763111261));
#56438=CARTESIAN_POINT('Ctrl Pts',(18.2578646281728,2.06537130671209,39.699133824258));
#56439=CARTESIAN_POINT('Ctrl Pts',(18.2062856112127,2.06114870003868,39.63901888629));
#56440=CARTESIAN_POINT('Ctrl Pts',(18.1546553056601,2.0569218945347,39.5788441718715));
#56441=CARTESIAN_POINT('Ctrl Pts',(18.1060767223792,2.05269508903072,39.5160922533979));
#56442=CARTESIAN_POINT('Ctrl Pts',(18.0608024441042,2.04846828352674,39.4511118680953));
#56443=CARTESIAN_POINT('Ctrl Pts',(18.0155062267494,2.04423942979081,39.386099994497));
#56444=CARTESIAN_POINT('Ctrl Pts',(17.9735177527947,2.04001057605487,39.3188579009626));
#56445=CARTESIAN_POINT('Ctrl Pts',(17.9350451179742,2.03578172231894,39.2497616170746));
#56446=CARTESIAN_POINT('Ctrl Pts',(17.8965033395575,2.03154526842365,39.180541152309));
#56447=CARTESIAN_POINT('Ctrl Pts',(17.8614902333218,2.02730881452837,39.1094602602954));
#56448=CARTESIAN_POINT('Ctrl Pts',(17.8301668428778,2.02307236063308,39.0369175583546));
#56449=CARTESIAN_POINT('Ctrl Pts',(17.8016979397624,2.01922197299023,38.9709856421728));
#56450=CARTESIAN_POINT('Ctrl Pts',(17.776276383819,2.01537158534738,38.9038467014695));
#56451=CARTESIAN_POINT('Ctrl Pts',(17.7539870835865,2.01152119770453,38.83581004356));
#56452=CARTESIAN_POINT('Ctrl Pts',(17.7247520329228,2.00647095940009,38.7465719284007));
#56453=CARTESIAN_POINT('Ctrl Pts',(17.7008157486621,2.00142072109565,38.6555178360481));
#56454=CARTESIAN_POINT('Ctrl Pts',(17.6823695053237,1.99637048279121,38.5632270836712));
#56455=CARTESIAN_POINT('Ctrl Pts',(17.6641279904338,1.99137629532779,38.4719606343029));
#56456=CARTESIAN_POINT('Ctrl Pts',(17.651255385937,1.98638210786438,38.3794848941208));
#56457=CARTESIAN_POINT('Ctrl Pts',(17.6438903546904,1.98138792040096,38.2863807398292));
#56458=CARTESIAN_POINT('Ctrl Pts',(17.6390429132866,1.97810089685982,38.2251023939168));
#56459=CARTESIAN_POINT('Ctrl Pts',(17.6365803430543,1.97481387331868,38.1635522471656));
#56460=CARTESIAN_POINT('Ctrl Pts',(17.6365307642293,1.97152684977754,38.1019006486528));
#56461=CARTESIAN_POINT('',(17.6365304902263,1.17777684969959,38.0984777417075));
#56462=CARTESIAN_POINT('Ctrl Pts',(17.6365307642285,1.97152684972829,38.1019006477291));
#56463=CARTESIAN_POINT('Ctrl Pts',(17.6364672651918,1.96731692886144,38.0229391350386));
#56464=CARTESIAN_POINT('Ctrl Pts',(17.6403651241089,1.96310700799459,37.9439206442699));
#56465=CARTESIAN_POINT('Ctrl Pts',(17.6482147911937,1.95889708712774,37.8652729829355));
#56466=CARTESIAN_POINT('Ctrl Pts',(17.6560624232589,1.95468825767937,37.7866457109418));
#56467=CARTESIAN_POINT('Ctrl Pts',(17.6678597823381,1.950479428231,37.7083895466702));
#56468=CARTESIAN_POINT('Ctrl Pts',(17.6835453668716,1.94627059878263,37.6309281786783));
#56469=CARTESIAN_POINT('Ctrl Pts',(17.6992318422657,1.94206153029438,37.5534624112789));
#56470=CARTESIAN_POINT('Ctrl Pts',(17.7188068863251,1.93785246180614,37.4767919918292));
#56471=CARTESIAN_POINT('Ctrl Pts',(17.7421579940123,1.93364339331789,37.4013298940864));
#56472=CARTESIAN_POINT('Ctrl Pts',(17.7655341420198,1.9294298112783,37.3257868753385));
#56473=CARTESIAN_POINT('Ctrl Pts',(17.7926942992056,1.92521622923872,37.2514552172083));
#56474=CARTESIAN_POINT('Ctrl Pts',(17.8234764060496,1.92100264719913,37.1787315885817));
#56475=CARTESIAN_POINT('Ctrl Pts',(17.8542754425718,1.91678674775519,37.1059679630946));
#56476=CARTESIAN_POINT('Ctrl Pts',(17.8887001887314,1.91257084831125,37.0348145525808));
#56477=CARTESIAN_POINT('Ctrl Pts',(17.9265419786131,1.90835494886731,36.965644555509));
#56478=CARTESIAN_POINT('Ctrl Pts',(17.9644524925575,1.90413139297429,36.8963489395585));
#56479=CARTESIAN_POINT('Ctrl Pts',(18.0057921972571,1.89990783708127,36.8290443336176));
#56480=CARTESIAN_POINT('Ctrl Pts',(18.0503085452814,1.89568428118824,36.7640757235916));
#56481=CARTESIAN_POINT('Ctrl Pts',(18.0850409851694,1.89238898838731,36.713386068162));
#56482=CARTESIAN_POINT('Ctrl Pts',(18.1217062669699,1.88909369558638,36.664117868854));
#56483=CARTESIAN_POINT('Ctrl Pts',(18.160168207798,1.88579840278545,36.6164200671002));
#56484=CARTESIAN_POINT('Ctrl Pts',(18.2096290557138,1.88156075974001,36.5550821921084));
#56485=CARTESIAN_POINT('Ctrl Pts',(18.2622535021514,1.87732311669457,36.4961053368348));
#56486=CARTESIAN_POINT('Ctrl Pts',(18.3177876717066,1.87308547364912,36.4398337060892));
#56487=CARTESIAN_POINT('Ctrl Pts',(18.3732419807513,1.86885392451558,36.3836429963548));
#56488=CARTESIAN_POINT('Ctrl Pts',(18.4315973767101,1.86462237538204,36.3301501164099));
#56489=CARTESIAN_POINT('Ctrl Pts',(18.4925594774106,1.8603908262485,36.279666648178));
#56490=CARTESIAN_POINT('Ctrl Pts',(18.5534511648287,1.85616416469693,36.2292414900547));
#56491=CARTESIAN_POINT('Ctrl Pts',(18.6169432144885,1.85193750314536,36.1818191334874));
#56492=CARTESIAN_POINT('Ctrl Pts',(18.682705210216,1.84771084159379,36.137673605715));
#56493=CARTESIAN_POINT('Ctrl Pts',(18.7484256946727,1.84348684805876,36.0935559441429));
#56494=CARTESIAN_POINT('Ctrl Pts',(18.816412892918,1.83926285452372,36.0527112663131));
#56495=CARTESIAN_POINT('Ctrl Pts',(18.8863051724119,1.83503886098868,36.015371910411));
#56496=CARTESIAN_POINT('Ctrl Pts',(18.956175095001,1.83081621861034,35.9780444984952));
#56497=CARTESIAN_POINT('Ctrl Pts',(19.0279484755394,1.826593576232,35.9442204026176));
#56498=CARTESIAN_POINT('Ctrl Pts',(19.1012379912428,1.82237093385366,35.9140866228245));
#56499=CARTESIAN_POINT('Ctrl Pts',(19.1745268820873,1.81814832747714,35.883953099949));
#56500=CARTESIAN_POINT('Ctrl Pts',(19.2493314482957,1.81392572110061,35.8575100075387));
#56501=CARTESIAN_POINT('Ctrl Pts',(19.3252446324073,1.80970311472409,35.8348961094897));
#56502=CARTESIAN_POINT('Ctrl Pts',(19.4012333018571,1.80547630953975,35.8122597249944));
#56503=CARTESIAN_POINT('Ctrl Pts',(19.478332340891,1.80124950435542,35.7934602747277));
#56504=CARTESIAN_POINT('Ctrl Pts',(19.556120363395,1.79702269917109,35.7785863554491));
#56505=CARTESIAN_POINT('Ctrl Pts',(19.6339460803034,1.79279384576777,35.7637052285887));
#56506=CARTESIAN_POINT('Ctrl Pts',(19.7124609809109,1.78856499236445,35.7527534870205));
#56507=CARTESIAN_POINT('Ctrl Pts',(19.7912368782203,1.78433613896113,35.7457679808726));
#56508=CARTESIAN_POINT('Ctrl Pts',(19.8701543524351,1.78009968541616,35.7387699202965));
#56509=CARTESIAN_POINT('Ctrl Pts',(19.9493332910468,1.77586323187119,35.735752355794));
#56510=CARTESIAN_POINT('Ctrl Pts',(20.0283440476992,1.77162677832622,35.7366999649092));
#56511=CARTESIAN_POINT('Ctrl Pts',(20.1001546402594,1.76777638817293,35.7375612194392));
#56512=CARTESIAN_POINT('Ctrl Pts',(20.1718260670583,1.76392599801965,35.7416972098081));
#56513=CARTESIAN_POINT('Ctrl Pts',(20.2430412607103,1.76007560786637,35.7490594676827));
#56514=CARTESIAN_POINT('Ctrl Pts',(20.3214190114522,1.75583795991208,35.7571621938428));
#56515=CARTESIAN_POINT('Ctrl Pts',(20.3995382347593,1.75160031195779,35.7692039567637));
#56516=CARTESIAN_POINT('Ctrl Pts',(20.4769719941166,1.74736266400351,35.7851591506697));
#56517=CARTESIAN_POINT('Ctrl Pts',(20.5542944013986,1.74313110991445,35.8010914005269));
#56518=CARTESIAN_POINT('Ctrl Pts',(20.6309328469414,1.7388995558254,35.820925811592));
#56519=CARTESIAN_POINT('Ctrl Pts',(20.706465711346,1.73466800173634,35.8445850404876));
#56520=CARTESIAN_POINT('Ctrl Pts',(20.7819113336741,1.73044133518291,35.868216942467));
#56521=CARTESIAN_POINT('Ctrl Pts',(20.8562534674485,1.72621466862947,35.8956647436907));
#56522=CARTESIAN_POINT('Ctrl Pts',(20.9290823821772,1.72198800207604,35.9268004306949));
#56523=CARTESIAN_POINT('Ctrl Pts',(21.0018653252485,1.71776400351329,35.9579164639786));
#56524=CARTESIAN_POINT('Ctrl Pts',(21.0731365153078,1.71354000495054,35.9927155786309));
#56525=CARTESIAN_POINT('Ctrl Pts',(21.1425042013522,1.70931600638779,36.0310208819825));
#56526=CARTESIAN_POINT('Ctrl Pts',(21.2118496986302,1.70509335896307,36.0693139325479));
#56527=CARTESIAN_POINT('Ctrl Pts',(21.2792924909367,1.70087071153834,36.111110718232));
#56528=CARTESIAN_POINT('Ctrl Pts',(21.3444648759035,1.69664806411361,36.1561881165191));
#56529=CARTESIAN_POINT('Ctrl Pts',(21.409636705396,1.69242545267916,36.2012651306044));
#56530=CARTESIAN_POINT('Ctrl Pts',(21.4725377813014,1.68820284124471,36.2496224338601));
#56531=CARTESIAN_POINT('Ctrl Pts',(21.5328301227423,1.68398022981027,36.3009940923627));
#56532=CARTESIAN_POINT('Ctrl Pts',(21.5931824163948,1.67975341958559,36.3524168327186));
#56533=CARTESIAN_POINT('Ctrl Pts',(21.6509204363752,1.67552660936091,36.4068596108128));
#56534=CARTESIAN_POINT('Ctrl Pts',(21.7057404858179,1.67129979913624,36.4640171651446));
#56535=CARTESIAN_POINT('Ctrl Pts',(21.7605870998265,1.66707094069418,36.5212024167445));
#56536=CARTESIAN_POINT('Ctrl Pts',(21.812512619037,1.66284208225211,36.581104710582));
#56537=CARTESIAN_POINT('Ctrl Pts',(21.8612530531965,1.65861322381005,36.6433849125913));
#56538=CARTESIAN_POINT('Ctrl Pts',(21.9100810833794,1.65437676528832,36.7057770442156));
#56539=CARTESIAN_POINT('Ctrl Pts',(21.9557123203718,1.65014030676659,36.7705552388603));
#56540=CARTESIAN_POINT('Ctrl Pts',(21.9979257454302,1.64590384824486,36.837350738864));
#56541=CARTESIAN_POINT('Ctrl Pts',(22.0362918130926,1.64205350314567,36.8980584561161));
#56542=CARTESIAN_POINT('Ctrl Pts',(22.071835123553,1.63820315804648,36.9604319462386));
#56543=CARTESIAN_POINT('Ctrl Pts',(22.1044237487931,1.63435281294729,37.0241788594681));
#56544=CARTESIAN_POINT('Ctrl Pts',(22.1402902674161,1.63011518484278,37.0943376904606));
#56545=CARTESIAN_POINT('Ctrl Pts',(22.1727117659432,1.62587755673826,37.1664237990782));
#56546=CARTESIAN_POINT('Ctrl Pts',(22.2014773272519,1.62163992863375,37.2400651079902));
#56547=CARTESIAN_POINT('Ctrl Pts',(22.2302015223787,1.61740839443066,37.3136005173599));
#56548=CARTESIAN_POINT('Ctrl Pts',(22.2552800518491,1.61317686022756,37.3886862526061));
#56549=CARTESIAN_POINT('Ctrl Pts',(22.2765482936958,1.60894532602447,37.4649265338793));
#56550=CARTESIAN_POINT('Ctrl Pts',(22.2977919703461,1.60471867931841,37.5410787562757));
#56551=CARTESIAN_POINT('Ctrl Pts',(22.3152339798406,1.60049203261236,37.6183824254067));
#56552=CARTESIAN_POINT('Ctrl Pts',(22.3287586771763,1.59626538590631,37.6964241528833));
#56553=CARTESIAN_POINT('Ctrl Pts',(22.3422748374071,1.59204140715842,37.7744166185981));
#56554=CARTESIAN_POINT('Ctrl Pts',(22.3518785136756,1.58781742841053,37.8531457572553));
#56555=CARTESIAN_POINT('Ctrl Pts',(22.357504850999,1.58359344966264,37.9321866560246));
#56556=CARTESIAN_POINT('Ctrl Pts',(22.3631293886866,1.57937082199321,38.0112022728352));
#56557=CARTESIAN_POINT('Ctrl Pts',(22.364779080483,1.57514819432379,38.0905289844784));
#56558=CARTESIAN_POINT('Ctrl Pts',(22.3624409426436,1.57092556665437,38.1697368870928));
#56559=CARTESIAN_POINT('Ctrl Pts',(22.3601028246846,1.56670297488862,38.2489441162272));
#56560=CARTESIAN_POINT('Ctrl Pts',(22.3537769597684,1.56248038312288,38.3280320698116));
#56561=CARTESIAN_POINT('Ctrl Pts',(22.343502455719,1.55825779135713,38.4065724725726));
#56562=CARTESIAN_POINT('Ctrl Pts',(22.3332177344175,1.55403100052894,38.4851909780898));
#56563=CARTESIAN_POINT('Ctrl Pts',(22.3189765914572,1.54980420970075,38.5632603792459));
#56564=CARTESIAN_POINT('Ctrl Pts',(22.3008697873043,1.54557741887256,38.6403597531));
#56565=CARTESIAN_POINT('Ctrl Pts',(22.2827542084542,1.54134857970887,38.7174964899065));
#56566=CARTESIAN_POINT('Ctrl Pts',(22.2607693666919,1.53711974054519,38.7936618119859));
#56567=CARTESIAN_POINT('Ctrl Pts',(22.2350560507775,1.5328909013815,38.8684496670459));
#56568=CARTESIAN_POINT('Ctrl Pts',(22.2092965202539,1.52865446171425,38.9433719385112));
#56569=CARTESIAN_POINT('Ctrl Pts',(22.1797953008886,1.524418022047,39.0169113601128));
#56570=CARTESIAN_POINT('Ctrl Pts',(22.1467414226089,1.52018158237975,39.0886818018732));
#56571=CARTESIAN_POINT('Ctrl Pts',(22.1166985853834,1.51633106092923,39.1539143195573));
#56572=CARTESIAN_POINT('Ctrl Pts',(22.0837215876223,1.51248053947872,39.2176855272462));
#56573=CARTESIAN_POINT('Ctrl Pts',(22.0479838852922,1.50863001802821,39.2797255810076));
#56574=CARTESIAN_POINT('Ctrl Pts',(22.0086531267125,1.50439236648092,39.3480031203474));
#56575=CARTESIAN_POINT('Ctrl Pts',(21.9658303594803,1.50015471493363,39.4144398044524));
#56576=CARTESIAN_POINT('Ctrl Pts',(21.9197129007478,1.49591706338634,39.4786561643871));
#56577=CARTESIAN_POINT('Ctrl Pts',(21.8736617617226,1.49168550583941,39.542780177295));
#56578=CARTESIAN_POINT('Ctrl Pts',(21.8243256115447,1.48745394829248,39.6046898293475));
#56579=CARTESIAN_POINT('Ctrl Pts',(21.7719468506317,1.48322239074554,39.6640315851787));
#56580=CARTESIAN_POINT('Ctrl Pts',(21.7196285909442,1.47899572095108,39.7233047970257));
#56581=CARTESIAN_POINT('Ctrl Pts',(21.6642750132269,1.47476905115662,39.7800156573782));
#56582=CARTESIAN_POINT('Ctrl Pts',(21.6061699489185,1.47054238136216,39.8338421312482));
#56583=CARTESIAN_POINT('Ctrl Pts',(21.5481015639615,1.46631837969153,39.8876346266658));
#56584=CARTESIAN_POINT('Ctrl Pts',(21.4872854829616,1.4620943780209,39.9385460319441));
#56585=CARTESIAN_POINT('Ctrl Pts',(21.4240428515956,1.45787037635027,39.9862906450808));
#56586=CARTESIAN_POINT('Ctrl Pts',(21.3608204517885,1.45364772595388,40.0340199845338));
#56587=CARTESIAN_POINT('Ctrl Pts',(21.2951734169776,1.44942507555749,40.0785842613587));
#56588=CARTESIAN_POINT('Ctrl Pts',(21.2274553150098,1.4452024251611,40.1197385698536));
#56589=CARTESIAN_POINT('Ctrl Pts',(21.1597377924494,1.44097981089442,40.1608925262253));
#56590=CARTESIAN_POINT('Ctrl Pts',(21.0899496393029,1.43675719662773,40.1986363300461));
#56591=CARTESIAN_POINT('Ctrl Pts',(21.0184714126016,1.43253458236105,40.2327696599992));
#56592=CARTESIAN_POINT('Ctrl Pts',(20.9469221149502,1.42830776954018,40.2669369287936));
#56593=CARTESIAN_POINT('Ctrl Pts',(20.8736798110474,1.4240809567193,40.2974863504011));
#56594=CARTESIAN_POINT('Ctrl Pts',(20.7991470067265,1.41985414389843,40.3242649353303));
#56595=CARTESIAN_POINT('Ctrl Pts',(20.7245780877089,1.41562528298525,40.3510564957606));
#56596=CARTESIAN_POINT('Ctrl Pts',(20.648717871736,1.41139642207206,40.3740734433361));
#56597=CARTESIAN_POINT('Ctrl Pts',(20.5719836225394,1.40716756115888,40.3932128502271));
#56598=CARTESIAN_POINT('Ctrl Pts',(20.4951114713913,1.40293110040366,40.4123866532527));
#56599=CARTESIAN_POINT('Ctrl Pts',(20.4173626095551,1.39869463964843,40.427668901285));
#56600=CARTESIAN_POINT('Ctrl Pts',(20.3391638481552,1.39445817889321,40.4390079788245));
#56601=CARTESIAN_POINT('Ctrl Pts',(20.2680926964329,1.39060786029852,40.4493135295234));
#56602=CARTESIAN_POINT('Ctrl Pts',(20.1966502644901,1.38675754170382,40.4563626067236));
#56603=CARTESIAN_POINT('Ctrl Pts',(20.1251572814483,1.38290722310913,40.4601538288426));
#56604=CARTESIAN_POINT('Ctrl Pts',(20.0464718075153,1.37866954647953,40.4643264636457));
#56605=CARTESIAN_POINT('Ctrl Pts',(19.9674297554087,1.37443186984992,40.4645676688016));
#56606=CARTESIAN_POINT('Ctrl Pts',(19.8884568612947,1.37019419322032,40.4608364130341));
#56607=CARTESIAN_POINT('Ctrl Pts',(19.8095975279049,1.36596261024642,40.4571105227039));
#56608=CARTESIAN_POINT('Ctrl Pts',(19.7308076193892,1.36173102727252,40.4494235374622));
#56609=CARTESIAN_POINT('Ctrl Pts',(19.6525156568587,1.35749944429862,40.4377863615334));
#56610=CARTESIAN_POINT('Ctrl Pts',(19.574314119327,1.35327274868318,40.4261626262131));
#56611=CARTESIAN_POINT('Ctrl Pts',(19.4966098462091,1.34904605306774,40.4105978353342));
#56612=CARTESIAN_POINT('Ctrl Pts',(19.4198274858161,1.3448193574523,40.3911547950074));
#56613=CARTESIAN_POINT('Ctrl Pts',(19.3430935905616,1.34059532973333,40.3717240271562));
#56614=CARTESIAN_POINT('Ctrl Pts',(19.2672809062322,1.33637130201436,40.3484199835529));
#56615=CARTESIAN_POINT('Ctrl Pts',(19.1928039135692,1.33214727429539,40.3213565492624));
#56616=CARTESIAN_POINT('Ctrl Pts',(19.1183507428936,1.32792459766125,40.2943017714008));
#56617=CARTESIAN_POINT('Ctrl Pts',(19.0452328557494,1.32370192102712,40.263490150698));
#56618=CARTESIAN_POINT('Ctrl Pts',(18.973848158353,1.31947924439298,40.229084976882));
#56619=CARTESIAN_POINT('Ctrl Pts',(18.9024640691693,1.31525660373695,40.1946800962053));
#56620=CARTESIAN_POINT('Ctrl Pts',(18.8328135620277,1.31103396308091,40.1566819281047));
#56621=CARTESIAN_POINT('Ctrl Pts',(18.7652718336524,1.30681132242487,40.1153006713957));
#56622=CARTESIAN_POINT('Ctrl Pts',(18.6976629480153,1.30258448316465,40.0738782689838));
#56623=CARTESIAN_POINT('Ctrl Pts',(18.632167430101,1.29835764390443,40.0290663041574));
#56624=CARTESIAN_POINT('Ctrl Pts',(18.5691327188234,1.2941308046442,39.9811191521428));
#56625=CARTESIAN_POINT('Ctrl Pts',(18.5060674633782,1.28990191722219,39.9331487668044));
#56626=CARTESIAN_POINT('Ctrl Pts',(18.4454657487965,1.28567302980018,39.882040470467));
#56627=CARTESIAN_POINT('Ctrl Pts',(18.3876410520472,1.28144414237817,39.8280882685374));
#56628=CARTESIAN_POINT('Ctrl Pts',(18.3297124397358,1.27720765531035,39.7740391102257));
#56629=CARTESIAN_POINT('Ctrl Pts',(18.2745711437923,1.27297116824253,39.7171361720341));
#56630=CARTESIAN_POINT('Ctrl Pts',(18.2224927938629,1.26873468117471,39.6577093994166));
#56631=CARTESIAN_POINT('Ctrl Pts',(18.1751644211586,1.26488459684649,39.6037028410892));
#56632=CARTESIAN_POINT('Ctrl Pts',(18.1303653946041,1.26103451251827,39.547612476359));
#56633=CARTESIAN_POINT('Ctrl Pts',(18.0882714251047,1.25718442819005,39.4897065506174));
#56634=CARTESIAN_POINT('Ctrl Pts',(18.0416356896263,1.25291893561627,39.4255528139269));
#56635=CARTESIAN_POINT('Ctrl Pts',(17.9981457106074,1.24865344304249,39.3589293252204));
#56636=CARTESIAN_POINT('Ctrl Pts',(17.9580708299778,1.24438795046871,39.290174653365));
#56637=CARTESIAN_POINT('Ctrl Pts',(17.9180549133786,1.24012873391197,39.2215211434468));
#56638=CARTESIAN_POINT('Ctrl Pts',(17.8814443465497,1.23586951735523,39.1507430715146));
#56639=CARTESIAN_POINT('Ctrl Pts',(17.8484665606069,1.23161030079849,39.0782097423729));
#56640=CARTESIAN_POINT('Ctrl Pts',(17.8155274888571,1.22735608433886,39.0057615635597));
#56641=CARTESIAN_POINT('Ctrl Pts',(17.786212915632,1.22310186787923,38.9315626377535));
#56642=CARTESIAN_POINT('Ctrl Pts',(17.7607047949425,1.2188476514196,38.8560075565141));
#56643=CARTESIAN_POINT('Ctrl Pts',(17.7352203500755,1.21459738358774,38.7805226030866));
#56644=CARTESIAN_POINT('Ctrl Pts',(17.7135354803532,1.21034711575588,38.7036844317353));
#56645=CARTESIAN_POINT('Ctrl Pts',(17.6957838047055,1.20609684792401,38.6259069939093));
#56646=CARTESIAN_POINT('Ctrl Pts',(17.6780415344963,1.20184883202787,38.5481707652017));
#56647=CARTESIAN_POINT('Ctrl Pts',(17.6642284180863,1.19760081613173,38.4694967075477));
#56648=CARTESIAN_POINT('Ctrl Pts',(17.6544277166018,1.19335280023559,38.3903120807924));
#56649=CARTESIAN_POINT('Ctrl Pts',(17.6446283443218,1.18910536046987,38.3111381933266));
#56650=CARTESIAN_POINT('Ctrl Pts',(17.6388403639534,1.18485792070415,38.231454330974));
#56651=CARTESIAN_POINT('Ctrl Pts',(17.6370954127973,1.18061048093843,38.1516948031864));
#56652=CARTESIAN_POINT('Ctrl Pts',(17.6367073713473,1.17966593720172,38.133957915421));
#56653=CARTESIAN_POINT('Ctrl Pts',(17.6365190645752,1.178721393465,38.1162172986552));
#56654=CARTESIAN_POINT('Ctrl Pts',(17.636530490226,1.17777684972829,38.0984777422465));
#56655=CARTESIAN_POINT('Ctrl Pts',(17.6365304902264,1.17777684969959,38.0984777417075));
#56656=CARTESIAN_POINT('Ctrl Pts',(17.6365882237607,1.1730040949641,38.0088402283102));
#56657=CARTESIAN_POINT('Ctrl Pts',(17.6417494431323,1.16823134022862,37.9193966228562));
#56658=CARTESIAN_POINT('Ctrl Pts',(17.6519239320934,1.16345858549314,37.8306875045147));
#56659=CARTESIAN_POINT('Ctrl Pts',(17.6621469747597,1.15866305468241,37.7415550571597));
#56660=CARTESIAN_POINT('Ctrl Pts',(17.6774311176323,1.15386752387167,37.6531643358699));
#56661=CARTESIAN_POINT('Ctrl Pts',(17.697635314948,1.14907199306094,37.5660456031409));
#56662=CARTESIAN_POINT('Ctrl Pts',(17.7179521886893,1.14424971814043,37.4784410195136));
#56663=CARTESIAN_POINT('Ctrl Pts',(17.7432440262356,1.13942744321992,37.3921228568976));
#56664=CARTESIAN_POINT('Ctrl Pts',(17.7733193362406,1.1346051682994,37.3076088954691));
#56665=CARTESIAN_POINT('Ctrl Pts',(17.7798544807557,1.13355732328992,37.2892446308483));
#56666=CARTESIAN_POINT('Ctrl Pts',(17.7866153068068,1.13250947828044,37.2709654671663));
#56667=CARTESIAN_POINT('Ctrl Pts',(17.7935995603932,1.13146163327096,37.2527765696094));
#56668=CARTESIAN_POINT('Ctrl Pts',(17.8218455723972,1.12722389442741,37.1792162653646));
#56669=CARTESIAN_POINT('Ctrl Pts',(17.8538273169042,1.12298615558387,37.1069320076802));
#56670=CARTESIAN_POINT('Ctrl Pts',(17.8894088186085,1.11874841674032,37.0363293244936));
#56671=CARTESIAN_POINT('Ctrl Pts',(17.9249391483456,1.11451677245216,36.9658281794099));
#56672=CARTESIAN_POINT('Ctrl Pts',(17.9640587449404,1.110285128164,36.8970042212857));
#56673=CARTESIAN_POINT('Ctrl Pts',(18.0065830683766,1.10605348387584,36.8302443630299));
#56674=CARTESIAN_POINT('Ctrl Pts',(18.0490582618386,1.10182672856787,36.7635616349869));
#56675=CARTESIAN_POINT('Ctrl Pts',(18.0949301144955,1.09759997325989,36.6989386610957));
#56676=CARTESIAN_POINT('Ctrl Pts',(18.1439682646889,1.09337321795192,36.6367376727265));
#56677=CARTESIAN_POINT('Ctrl Pts',(18.1929754506256,1.08914913155245,36.5745759600509));
#56678=CARTESIAN_POINT('Ctrl Pts',(18.2451446762482,1.08492504515298,36.5148335645099));
#56679=CARTESIAN_POINT('Ctrl Pts',(18.3002030740553,1.08070095875351,36.4578426228132));
#56680=CARTESIAN_POINT('Ctrl Pts',(18.3552438471663,1.07647822452269,36.4008699244376));
#56681=CARTESIAN_POINT('Ctrl Pts',(18.4131716304322,1.07225549029186,36.3466472677579));
#56682=CARTESIAN_POINT('Ctrl Pts',(18.4736751895664,1.06803275606103,36.2954715258675));
#56683=CARTESIAN_POINT('Ctrl Pts',(18.5341782166333,1.06381005896487,36.2442962340158));
#56684=CARTESIAN_POINT('Ctrl Pts',(18.5972566157142,1.05958736186871,36.196168105306));
#56685=CARTESIAN_POINT('Ctrl Pts',(18.6625655639975,1.05536466477255,36.1513441632));
#56686=CARTESIAN_POINT('Ctrl Pts',(18.7279394147492,1.05113777126116,36.1064756761341));
#56687=CARTESIAN_POINT('Ctrl Pts',(18.7955478551298,1.04691087774978,36.0649182005989));
#56688=CARTESIAN_POINT('Ctrl Pts',(18.8650170261336,1.04268398423839,36.0268854132168));
#56689=CARTESIAN_POINT('Ctrl Pts',(18.9345198404873,1.03845504367714,35.9888342068676));
#56690=CARTESIAN_POINT('Ctrl Pts',(19.0058847581297,1.03422610311589,35.954311293574));
#56691=CARTESIAN_POINT('Ctrl Pts',(19.0787155627366,1.02999716255464,35.9234831894616));
#56692=CARTESIAN_POINT('Ctrl Pts',(19.1516772057252,1.02576062482701,35.8925997035739));
#56693=CARTESIAN_POINT('Ctrl Pts',(19.2261095561485,1.02152408709938,35.8654244506196));
#56694=CARTESIAN_POINT('Ctrl Pts',(19.3015989934079,1.01728754937175,35.8420747410751));
#56695=CARTESIAN_POINT('Ctrl Pts',(19.370193189267,1.0134379790318,35.8208578051978));
#56696=CARTESIAN_POINT('Ctrl Pts',(19.4396597441982,1.00958840869185,35.8027988984575));
#56697=CARTESIAN_POINT('Ctrl Pts',(19.5096822305933,1.0057388383519,35.7879491947831));
#56698=CARTESIAN_POINT('Ctrl Pts',(19.5867672127342,1.00150099882088,35.7716017441074));
#56699=CARTESIAN_POINT('Ctrl Pts',(19.6648152223334,0.997263159289865,35.7590829273399));
#56700=CARTESIAN_POINT('Ctrl Pts',(19.7434120318108,0.99302531975885,35.7504994029623));
#56701=CARTESIAN_POINT('Ctrl Pts',(19.8218958550916,0.988793572299183,35.7419282177595));
#56702=CARTESIAN_POINT('Ctrl Pts',(19.9009264494113,0.984561824839515,35.7372811408079));
#56703=CARTESIAN_POINT('Ctrl Pts',(19.9800787707609,0.980330077379848,35.7366139575758));
#56704=CARTESIAN_POINT('Ctrl Pts',(20.0591397067108,0.976103215688868,35.7359475446409));
#56705=CARTESIAN_POINT('Ctrl Pts',(20.1383216240653,0.971876353997889,35.7392518979301));
#56706=CARTESIAN_POINT('Ctrl Pts',(20.2171952439491,0.967649492306909,35.7465309292651));
#56707=CARTESIAN_POINT('Ctrl Pts',(20.2960190972292,0.96342529762362,35.7538053677759));
#56708=CARTESIAN_POINT('Ctrl Pts',(20.3745345736319,0.959201102940331,35.7650494634725));
#56709=CARTESIAN_POINT('Ctrl Pts',(20.4523145051818,0.954976908257042,35.7802150898624));
#56710=CARTESIAN_POINT('Ctrl Pts',(20.5300695712347,0.950754064008214,35.7953758679472));
#56711=CARTESIAN_POINT('Ctrl Pts',(20.6070890996636,0.946531219759387,35.8144555975261));
#56712=CARTESIAN_POINT('Ctrl Pts',(20.6829546220782,0.942308375510559,35.8373547725987));
#56713=CARTESIAN_POINT('Ctrl Pts',(20.7588195055433,0.938085566827086,35.8602537548114));
#56714=CARTESIAN_POINT('Ctrl Pts',(20.833529954006,0.933862758143614,35.8869719817455));
#56715=CARTESIAN_POINT('Ctrl Pts',(20.9066826462485,0.929639949460142,35.9173600801113));
#56716=CARTESIAN_POINT('Ctrl Pts',(20.9799080625471,0.925412942711408,35.9477783885172));
#56717=CARTESIAN_POINT('Ctrl Pts',(21.0515721953663,0.921185935962673,35.9818736757559));
#56718=CARTESIAN_POINT('Ctrl Pts',(21.1212922818258,0.916958929213939,36.0194486164437));
#56719=CARTESIAN_POINT('Ctrl Pts',(21.1910461501188,0.912729874331789,36.0570417635117));
#56720=CARTESIAN_POINT('Ctrl Pts',(21.2588536941375,0.908500819449638,36.0981176796145));
#56721=CARTESIAN_POINT('Ctrl Pts',(21.3243595437161,0.904271764567488,36.1424346141526));
#56722=CARTESIAN_POINT('Ctrl Pts',(21.3899830765645,0.900035112058414,36.1868311654241));
#56723=CARTESIAN_POINT('Ctrl Pts',(21.4532962773062,0.89579845954934,36.2344800867139));
#56724=CARTESIAN_POINT('Ctrl Pts',(21.5139755799051,0.891561807040266,36.2850982438845));
#56725=CARTESIAN_POINT('Ctrl Pts',(21.5690968407095,0.887713219171115,36.3310799299511));
#56726=CARTESIAN_POINT('Ctrl Pts',(21.6220448664736,0.883864631301964,36.3795111358586));
#56727=CARTESIAN_POINT('Ctrl Pts',(21.6726046576235,0.880016043432813,36.430154468163));
#56728=CARTESIAN_POINT('Ctrl Pts',(21.7282653304164,0.875779178817131,36.4859071104193));
#56729=CARTESIAN_POINT('Ctrl Pts',(21.7812400674091,0.87154231420145,36.5445506652308));
#56730=CARTESIAN_POINT('Ctrl Pts',(21.8312139615278,0.867305449585769,36.605795908182));
#56731=CARTESIAN_POINT('Ctrl Pts',(21.8811159619345,0.863074680231024,36.6669530421728));
#56732=CARTESIAN_POINT('Ctrl Pts',(21.9280253986868,0.858843910876279,36.7307040710797));
#56733=CARTESIAN_POINT('Ctrl Pts',(21.971664141373,0.854613141521535,36.7967229939404));
#56734=CARTESIAN_POINT('Ctrl Pts',(22.0152524871653,0.850387258137864,36.8626656738011));
#56735=CARTESIAN_POINT('Ctrl Pts',(22.055577387786,0.846161374754194,36.9308706536058));
#56736=CARTESIAN_POINT('Ctrl Pts',(22.0924019147194,0.841935491370524,37.0009801329463));
#56737=CARTESIAN_POINT('Ctrl Pts',(22.1292032040468,0.83771227467184,37.0710453706742));
#56738=CARTESIAN_POINT('Ctrl Pts',(22.1625082864791,0.833489057973156,37.1430123084224));
#56739=CARTESIAN_POINT('Ctrl Pts',(22.1921250309563,0.829265841274472,37.2164965820355));
#56740=CARTESIAN_POINT('Ctrl Pts',(22.2217323167283,0.825043973345284,37.2899573869626));
#56741=CARTESIAN_POINT('Ctrl Pts',(22.2476534285012,0.820822105416095,37.3649341308112));
#56742=CARTESIAN_POINT('Ctrl Pts',(22.2697440688809,0.816600237486907,37.4410217737437));
#56743=CARTESIAN_POINT('Ctrl Pts',(22.2918345389071,0.812378402114952,37.517108829921));
#56744=CARTESIAN_POINT('Ctrl Pts',(22.3100944668947,0.808156566742998,37.5943063173825));
#56745=CARTESIAN_POINT('Ctrl Pts',(22.3244296318692,0.803934731371043,37.6721947553052));
#56746=CARTESIAN_POINT('Ctrl Pts',(22.3387790902978,0.799708686447955,37.7501608550346));
#56747=CARTESIAN_POINT('Ctrl Pts',(22.3491958837366,0.795482641524868,37.8288188190892));
#56748=CARTESIAN_POINT('Ctrl Pts',(22.3556372071988,0.79125659660178,37.9077403085395));
#56749=CARTESIAN_POINT('Ctrl Pts',(22.3620816596615,0.787028498793719,37.9867001356655));
#56750=CARTESIAN_POINT('Ctrl Pts',(22.3645467805294,0.782800400985658,38.0659232738646));
#56751=CARTESIAN_POINT('Ctrl Pts',(22.363041942897,0.778572303177597,38.1449801846302));
#56752=CARTESIAN_POINT('Ctrl Pts',(22.3615343943348,0.774336588549943,38.2241795145768));
#56753=CARTESIAN_POINT('Ctrl Pts',(22.3560426299536,0.77010087392229,38.3032115498097));
#56754=CARTESIAN_POINT('Ctrl Pts',(22.3466280503898,0.765865159294637,38.3816509080826));
#56755=CARTESIAN_POINT('Ctrl Pts',(22.3380545522257,0.762007855701003,38.4530826368805));
#56756=CARTESIAN_POINT('Ctrl Pts',(22.3262285401886,0.758150552107369,38.5240226863687));
#56757=CARTESIAN_POINT('Ctrl Pts',(22.3112327910835,0.754293248513735,38.5941593126921));
#56758=CARTESIAN_POINT('Ctrl Pts',(22.2947549221081,0.750054704459074,38.6712279626701));
#56759=CARTESIAN_POINT('Ctrl Pts',(22.2743871480269,0.745816160404412,38.7476159526973));
#56760=CARTESIAN_POINT('Ctrl Pts',(22.2502008691845,0.74157761634975,38.8229014381097));
#56761=CARTESIAN_POINT('Ctrl Pts',(22.2260493863507,0.73734517014983,38.898078612756));
#56762=CARTESIAN_POINT('Ctrl Pts',(22.1980904507105,0.733112723949911,38.9721559903171));
#56763=CARTESIAN_POINT('Ctrl Pts',(22.1664463281365,0.728880277749991,39.0447225773761));
#56764=CARTESIAN_POINT('Ctrl Pts',(22.1348388228573,0.724652729165109,39.1172051933244));
#56765=CARTESIAN_POINT('Ctrl Pts',(22.0995547914582,0.720425180580228,39.1881800656599));
#56766=CARTESIAN_POINT('Ctrl Pts',(22.0607655974215,0.716197631995346,39.2572534698086));
#56767=CARTESIAN_POINT('Ctrl Pts',(22.0220009430105,0.711972757930074,39.3262831753054));
#56768=CARTESIAN_POINT('Ctrl Pts',(21.9797357563619,0.707747883864801,39.393413392886));
#56769=CARTESIAN_POINT('Ctrl Pts',(21.9341880649202,0.703523009799529,39.4582735256274));
#56770=CARTESIAN_POINT('Ctrl Pts',(21.8886550226854,0.699299494552947,39.5231127978272));
#56771=CARTESIAN_POINT('Ctrl Pts',(21.8398418412436,0.695075979306365,39.58568305189));
#56772=CARTESIAN_POINT('Ctrl Pts',(21.7880099274264,0.690852464059783,39.6456425655127));
#56773=CARTESIAN_POINT('Ctrl Pts',(21.736178563767,0.686628993642725,39.7056014427091));
#56774=CARTESIAN_POINT('Ctrl Pts',(21.681328838936,0.682405523225666,39.7629492810137));
#56775=CARTESIAN_POINT('Ctrl Pts',(21.6237615331349,0.678182052808608,39.8173785035371));
#56776=CARTESIAN_POINT('Ctrl Pts',(21.5661372653819,0.673954403333392,39.871861582928));
#56777=CARTESIAN_POINT('Ctrl Pts',(21.5057903865848,0.669726753858176,39.9234199551932));
#56778=CARTESIAN_POINT('Ctrl Pts',(21.4430570967569,0.665499104382961,39.9717843509335));
#56779=CARTESIAN_POINT('Ctrl Pts',(21.3802935543493,0.661269416160799,40.0201720699802));
#56780=CARTESIAN_POINT('Ctrl Pts',(21.3151416937638,0.657039727938637,40.0653624766099));
#56781=CARTESIAN_POINT('Ctrl Pts',(21.2479671343398,0.652810039716476,40.1071294110017));
#56782=CARTESIAN_POINT('Ctrl Pts',(21.180672278697,0.648572776967528,40.1489711416305));
#56783=CARTESIAN_POINT('Ctrl Pts',(21.1113478974067,0.644335514218581,40.1873769224907));
#56784=CARTESIAN_POINT('Ctrl Pts',(21.040384453305,0.640098251469634,40.222166494463));
#56785=CARTESIAN_POINT('Ctrl Pts',(20.9760306248562,0.636255652177974,40.2537157262521));
#56786=CARTESIAN_POINT('Ctrl Pts',(20.910329365219,0.632413052886314,40.2822915244999));
#56787=CARTESIAN_POINT('Ctrl Pts',(20.8435835715002,0.628570453594655,40.3077946459748));
#56788=CARTESIAN_POINT('Ctrl Pts',(20.7699581473124,0.624331789447159,40.3359264282503));
#56789=CARTESIAN_POINT('Ctrl Pts',(20.6947864120994,0.620093125299663,40.360423862717));
#56790=CARTESIAN_POINT('Ctrl Pts',(20.6184612006793,0.615854461152167,40.3811173104762));
#56791=CARTESIAN_POINT('Ctrl Pts',(20.5422454777903,0.611621877369241,40.4017810734805));
#56792=CARTESIAN_POINT('Ctrl Pts',(20.4648800132238,0.607389293586315,40.41865156511));
#56793=CARTESIAN_POINT('Ctrl Pts',(20.3867762105732,0.60315670980339,40.4316077294079));
#56794=CARTESIAN_POINT('Ctrl Pts',(20.3087623158836,0.598928998292557,40.4445489794216));
#56795=CARTESIAN_POINT('Ctrl Pts',(20.2300122320118,0.594701286781725,40.4535847803177));
#56796=CARTESIAN_POINT('Ctrl Pts',(20.1509495880502,0.590473575270893,40.4586446664912));
#56797=CARTESIAN_POINT('Ctrl Pts',(20.0719366740902,0.586248522969131,40.463701370022));
#56798=CARTESIAN_POINT('Ctrl Pts',(19.992612056607,0.58202347066737,40.4647870929481));
#56799=CARTESIAN_POINT('Ctrl Pts',(19.913405348292,0.577798418365609,40.4618831061667));
#56800=CARTESIAN_POINT('Ctrl Pts',(19.83422383386,0.573574709958516,40.4589800430786));
#56801=CARTESIAN_POINT('Ctrl Pts',(19.7551606219727,0.569351001551423,40.4520898075416));
#56802=CARTESIAN_POINT('Ctrl Pts',(19.676644700725,0.565127293144331,40.4412457776429));
#56803=CARTESIAN_POINT('Ctrl Pts',(19.5981293423155,0.560903615014718,40.4304018254792));
#56804=CARTESIAN_POINT('Ctrl Pts',(19.5201617306439,0.556679936885105,40.4156042008339));
#56805=CARTESIAN_POINT('Ctrl Pts',(19.4431636280474,0.552456258755492,40.3969378954971));
#56806=CARTESIAN_POINT('Ctrl Pts',(19.3660889562055,0.548228380472418,40.3782530278209));
#56807=CARTESIAN_POINT('Ctrl Pts',(19.289986175618,0.544000502189343,40.3556919054373));
#56808=CARTESIAN_POINT('Ctrl Pts',(19.215264182522,0.539772623906269,40.3293900819882));
#56809=CARTESIAN_POINT('Ctrl Pts',(19.1405059468101,0.53554269496364,40.3030755012925));
#56810=CARTESIAN_POINT('Ctrl Pts',(19.0671302668755,0.531312766021011,40.2730167828784));
#56811=CARTESIAN_POINT('Ctrl Pts',(18.9955258770044,0.527082837078382,40.2393976201567));
#56812=CARTESIAN_POINT('Ctrl Pts',(18.923792977181,0.522845316590492,40.2057181203942));
#56813=CARTESIAN_POINT('Ctrl Pts',(18.8538381338368,0.518607796102602,40.1684656291719));
#56814=CARTESIAN_POINT('Ctrl Pts',(18.7860250899914,0.514370275614712,40.1278696602025));
#56815=CARTESIAN_POINT('Ctrl Pts',(18.7245596072136,0.510529403301667,40.0910736296744));
#56816=CARTESIAN_POINT('Ctrl Pts',(18.6648535817497,0.506688530988621,40.0515314697525));
#56817=CARTESIAN_POINT('Ctrl Pts',(18.607154751171,0.502847658675575,40.0094429956703));
#56818=CARTESIAN_POINT('Ctrl Pts',(18.5440944950677,0.498649889166365,39.9634436239674));
#56819=CARTESIAN_POINT('Ctrl Pts',(18.4831856799924,0.494452119657154,39.9142221837444));
#56820=CARTESIAN_POINT('Ctrl Pts',(18.424780789985,0.490254350147943,39.8620087631167));
#56821=CARTESIAN_POINT('Ctrl Pts',(18.3664603959426,0.486062653667637,39.8098708810844));
#56822=CARTESIAN_POINT('Ctrl Pts',(18.3106370903089,0.481870957187332,39.754749926423));
#56823=CARTESIAN_POINT('Ctrl Pts',(18.2576331101625,0.477679260707026,39.6969183016354));
#56824=CARTESIAN_POINT('Ctrl Pts',(18.2046896945328,0.473492353830652,39.6391527576288));
#56825=CARTESIAN_POINT('Ctrl Pts',(18.154559527168,0.469305446954278,39.5786830466592));
#56826=CARTESIAN_POINT('Ctrl Pts',(18.1075293268368,0.465118540077904,39.5158196184957));
#56827=CARTESIAN_POINT('Ctrl Pts',(18.0605277904194,0.46093418503284,39.4529945042639));
#56828=CARTESIAN_POINT('Ctrl Pts',(18.016622758633,0.456749829987776,39.3877789494164));
#56829=CARTESIAN_POINT('Ctrl Pts',(17.9760609471667,0.452565474942712,39.3205167558524));
#56830=CARTESIAN_POINT('Ctrl Pts',(17.935510634744,0.448382306138573,39.2532736307388));
#56831=CARTESIAN_POINT('Ctrl Pts',(17.8983019079526,0.444199137334434,39.1839854283694));
#56832=CARTESIAN_POINT('Ctrl Pts',(17.8646374777929,0.440015968530295,39.1130238593703));
#56833=CARTESIAN_POINT('Ctrl Pts',(17.8309716174094,0.435832622005396,39.0420592755888));
#56834=CARTESIAN_POINT('Ctrl Pts',(17.8008505554083,0.431649275480497,38.9694216174508));
#56835=CARTESIAN_POINT('Ctrl Pts',(17.7744297561447,0.427465928955598,38.8955045760811));
#56836=CARTESIAN_POINT('Ctrl Pts',(17.7479829229321,0.423278460336241,38.8215146999547));
#56837=CARTESIAN_POINT('Ctrl Pts',(17.725243790005,0.419090991716885,38.7462433761688));
#56838=CARTESIAN_POINT('Ctrl Pts',(17.7063183315099,0.414903523097528,38.6701007319173));
#56839=CARTESIAN_POINT('Ctrl Pts',(17.6873823111652,0.410713717551214,38.5939155942613));
#56840=CARTESIAN_POINT('Ctrl Pts',(17.6722642913954,0.4065239120049,38.5168586381407));
#56841=CARTESIAN_POINT('Ctrl Pts',(17.6610188679983,0.402334106458586,38.4393489428891));
#56842=CARTESIAN_POINT('Ctrl Pts',(17.6497553295379,0.398137551625042,38.3617143885742));
#56843=CARTESIAN_POINT('Ctrl Pts',(17.6423768800543,0.3939409967915,38.2836261155568));
#56844=CARTESIAN_POINT('Ctrl Pts',(17.6388860990133,0.389744441957957,38.2055063385164));
#56845=CARTESIAN_POINT('Ctrl Pts',(17.6373007618979,0.387838577896013,38.1700282662658));
#56846=CARTESIAN_POINT('Ctrl Pts',(17.6365165509045,0.38593271383407,38.1345436670864));
#56847=CARTESIAN_POINT('Ctrl Pts',(17.6365301745119,0.384026849772126,38.099091756019));
#56848=CARTESIAN_POINT('Origin',(20.,-1.3495818343519,38.1));
#56849=CARTESIAN_POINT('',(18.0708707491416,21.2722931656887,38.0982998874535));
#56850=CARTESIAN_POINT('Ctrl Pts',(19.3941040087494,21.1141809091495,36.2684889831927));
#56851=CARTESIAN_POINT('Ctrl Pts',(19.3627036109449,21.1163561899284,36.2788767859298));
#56852=CARTESIAN_POINT('Ctrl Pts',(19.3315975445805,21.1185314707073,36.2900633660934));
#56853=CARTESIAN_POINT('Ctrl Pts',(19.3008283950407,21.1207067514863,36.3020284697141));
#56854=CARTESIAN_POINT('Ctrl Pts',(19.2377524129147,21.1251660223333,36.3265566309862));
#56855=CARTESIAN_POINT('Ctrl Pts',(19.175844332916,21.1296252931803,36.3544564075852));
#56856=CARTESIAN_POINT('Ctrl Pts',(19.1154887940643,21.1340845640273,36.3855955892864));
#56857=CARTESIAN_POINT('Ctrl Pts',(19.0521316315247,21.1387656049598,36.4182833961378));
#56858=CARTESIAN_POINT('Ctrl Pts',(18.9904859997409,21.1434466458922,36.4545411133358));
#56859=CARTESIAN_POINT('Ctrl Pts',(18.9309759297778,21.1481276868246,36.4941575126478));
#56860=CARTESIAN_POINT('Ctrl Pts',(18.8744391227793,21.15257485195,36.5317945835379));
#56861=CARTESIAN_POINT('Ctrl Pts',(18.8198300706574,21.1570220170753,36.572462458363));
#56862=CARTESIAN_POINT('Ctrl Pts',(18.7674873179353,21.1614691822007,36.6159329376846));
#56863=CARTESIAN_POINT('Ctrl Pts',(18.7151762470697,21.1659136555599,36.6593771053313));
#56864=CARTESIAN_POINT('Ctrl Pts',(18.6651291328328,21.1703581289192,36.7056201980804));
#56865=CARTESIAN_POINT('Ctrl Pts',(18.6176531092621,21.1748026022785,36.7543924678543));
#56866=CARTESIAN_POINT('Ctrl Pts',(18.5701894778516,21.1792459155442,36.8031520071227));
#56867=CARTESIAN_POINT('Ctrl Pts',(18.5252959483506,21.18368922881,36.8544390596418));
#56868=CARTESIAN_POINT('Ctrl Pts',(18.4832429671676,21.1881325420758,36.907946871883));
#56869=CARTESIAN_POINT('Ctrl Pts',(18.4411864860854,21.1925762251405,36.9614591373626));
#56870=CARTESIAN_POINT('Ctrl Pts',(18.4019713250343,21.1970199082052,37.017192140241));
#56871=CARTESIAN_POINT('Ctrl Pts',(18.3658266378197,21.2014635912699,37.0748073453052));
#56872=CARTESIAN_POINT('Ctrl Pts',(18.3296431725879,21.2059120417633,37.1324843631441));
#56873=CARTESIAN_POINT('Ctrl Pts',(18.2965370163799,21.2103604922567,37.1920471940158));
#56874=CARTESIAN_POINT('Ctrl Pts',(18.2666925266657,21.2148089427501,37.2531306123235));
#56875=CARTESIAN_POINT('Ctrl Pts',(18.2368294566097,21.2192601627239,37.3142520594534));
#56876=CARTESIAN_POINT('Ctrl Pts',(18.2102322864395,21.2237113826978,37.3768955242203));
#56877=CARTESIAN_POINT('Ctrl Pts',(18.1870370415035,21.2281626026716,37.4406762039639));
#56878=CARTESIAN_POINT('Ctrl Pts',(18.1638027062202,21.2326213241715,37.5045643716398));
#56879=CARTESIAN_POINT('Ctrl Pts',(18.1439818790603,21.2370800456714,37.5695931074238));
#56880=CARTESIAN_POINT('Ctrl Pts',(18.1276603449738,21.2415387671712,37.6353638271547));
#56881=CARTESIAN_POINT('Ctrl Pts',(18.1216926387617,21.243169026916,37.6594118321176));
#56882=CARTESIAN_POINT('Ctrl Pts',(18.1161922483818,21.2447992866606,37.6835589537376));
#56883=CARTESIAN_POINT('Ctrl Pts',(18.1111616393731,21.2464295464053,37.7077855123479));
#56884=CARTESIAN_POINT('Ctrl Pts',(18.0918301223393,21.2526942737912,37.8008828152065));
#56885=CARTESIAN_POINT('Ctrl Pts',(18.0793762649212,21.258959001177,37.8954539813234));
#56886=CARTESIAN_POINT('Ctrl Pts',(18.0739715027794,21.2652237285629,37.9906529159316));
#56887=CARTESIAN_POINT('Ctrl Pts',(18.0719384999277,21.2675802075913,38.0264620228749));
#56888=CARTESIAN_POINT('Ctrl Pts',(18.0709024226888,21.2699366866197,38.06235971154));
#56889=CARTESIAN_POINT('Ctrl Pts',(18.0708707491422,21.2722931656481,38.098299886834));
#56890=CARTESIAN_POINT('',(21.5476173497497,21.75,36.9482955693174));
#56891=CARTESIAN_POINT('Ctrl Pts',(18.0708707491416,21.2722931656887,38.0982998874535));
#56892=CARTESIAN_POINT('Ctrl Pts',(18.0708117642268,21.2766815837971,38.1652304708287));
#56893=CARTESIAN_POINT('Ctrl Pts',(18.0742402209119,21.2810700019056,38.2322696432489));
#56894=CARTESIAN_POINT('Ctrl Pts',(18.0811633913888,21.285458420014,38.2990191607702));
#56895=CARTESIAN_POINT('Ctrl Pts',(18.0880808002805,21.289843186003,38.3657131281579));
#56896=CARTESIAN_POINT('Ctrl Pts',(18.0984871082126,21.294227951992,38.4321174151031));
#56897=CARTESIAN_POINT('Ctrl Pts',(18.1123375584943,21.2986127179809,38.4978354733163));
#56898=CARTESIAN_POINT('Ctrl Pts',(18.1261815683776,21.302995445073,38.5635229729216));
#56899=CARTESIAN_POINT('Ctrl Pts',(18.1434664408058,21.3073781721651,38.6285243800003));
#56900=CARTESIAN_POINT('Ctrl Pts',(18.1640960781561,21.3117608992572,38.6924519783564));
#56901=CARTESIAN_POINT('Ctrl Pts',(18.1847236974656,21.3161431976203,38.7563733231606));
#56902=CARTESIAN_POINT('Ctrl Pts',(18.2086952744819,21.3205254959835,38.8192205848984));
#56903=CARTESIAN_POINT('Ctrl Pts',(18.2358650602611,21.3249077943466,38.8806218491001));
#56904=CARTESIAN_POINT('Ctrl Pts',(18.2630601717377,21.3292941775695,38.9420803470929));
#56905=CARTESIAN_POINT('Ctrl Pts',(18.2934592370428,21.3336805607923,39.0020896913925));
#56906=CARTESIAN_POINT('Ctrl Pts',(18.3268691145082,21.3380669440151,39.0602997432642));
#56907=CARTESIAN_POINT('Ctrl Pts',(18.3602957555656,21.3424555281302,39.1185390023536));
#56908=CARTESIAN_POINT('Ctrl Pts',(18.3967359379642,21.3468441122452,39.1749767463128));
#56909=CARTESIAN_POINT('Ctrl Pts',(18.4359530809998,21.3512326963603,39.2292917214192));
#56910=CARTESIAN_POINT('Ctrl Pts',(18.4752380586776,21.3556288714932,39.2837006461767));
#56911=CARTESIAN_POINT('Ctrl Pts',(18.5173092640418,21.3600250466261,39.3359790791136));
#56912=CARTESIAN_POINT('Ctrl Pts',(18.5618904093106,21.364421221759,39.3858395553362));
#56913=CARTESIAN_POINT('Ctrl Pts',(18.5880238968701,21.3669982616141,39.4150677890933));
#56914=CARTESIAN_POINT('Ctrl Pts',(18.6150191785668,21.3695753014693,39.4434658355131));
#56915=CARTESIAN_POINT('Ctrl Pts',(18.6428152478348,21.3721523413244,39.4709821681518));
#56916=CARTESIAN_POINT('Ctrl Pts',(18.6908402055143,21.3766048496553,39.5185238078611));
#56917=CARTESIAN_POINT('Ctrl Pts',(18.7414626085893,21.3810573579862,39.5636343380257));
#56918=CARTESIAN_POINT('Ctrl Pts',(18.7944061999614,21.385509866317,39.6060166487156));
#56919=CARTESIAN_POINT('Ctrl Pts',(18.8472699163602,21.3899556572346,39.6483350180323));
#56920=CARTESIAN_POINT('Ctrl Pts',(18.902447488726,21.3944014481522,39.6879330292911));
#56921=CARTESIAN_POINT('Ctrl Pts',(18.9596262385859,21.3988472390698,39.7245507051062));
#56922=CARTESIAN_POINT('Ctrl Pts',(19.0167381012465,21.4032878293402,39.7611255458857));
#56923=CARTESIAN_POINT('Ctrl Pts',(19.0758460782621,21.4077284196106,39.7947267089443));
#56924=CARTESIAN_POINT('Ctrl Pts',(19.1366063571682,21.412169009881,39.8251359292582));
#56925=CARTESIAN_POINT('Ctrl Pts',(19.1973289329325,21.4166068446637,39.8555262799559));
#56926=CARTESIAN_POINT('Ctrl Pts',(19.2597013356713,21.4210446794463,39.8827283956558));
#56927=CARTESIAN_POINT('Ctrl Pts',(19.3233542501424,21.425482514229,39.9065694246554));
#56928=CARTESIAN_POINT('Ctrl Pts',(19.38698975622,21.4299191353112,39.9304039333877));
#56929=CARTESIAN_POINT('Ctrl Pts',(19.4519046159155,21.4343557563933,39.9508790067391));
#56930=CARTESIAN_POINT('Ctrl Pts',(19.5177103068475,21.4387923774755,39.9678702333885));
#56931=CARTESIAN_POINT('Ctrl Pts',(19.5835208368066,21.4432293248049,39.9848627094893));
#56932=CARTESIAN_POINT('Ctrl Pts',(19.6502218485231,21.4476662721344,39.998370709307));
#56933=CARTESIAN_POINT('Ctrl Pts',(19.7174122649928,21.4521032194638,40.008320394725));
#56934=CARTESIAN_POINT('Ctrl Pts',(19.7846756128002,21.4565449828448,40.0182808799551));
#56935=CARTESIAN_POINT('Ctrl Pts',(19.852428935245,21.4609867462257,40.024675271164));
#56936=CARTESIAN_POINT('Ctrl Pts',(19.920264669978,21.4654285096066,40.0274814743718));
#56937=CARTESIAN_POINT('Ctrl Pts',(19.9881423296492,21.469873018158,40.0302894119146));
#56938=CARTESIAN_POINT('Ctrl Pts',(20.0561020084809,21.4743175267094,40.0295047546418));
#56939=CARTESIAN_POINT('Ctrl Pts',(20.123737637891,21.4787620352608,40.0251575400131));
#56940=CARTESIAN_POINT('Ctrl Pts',(20.1914905344253,21.483214249732,40.0208027881535));
#56941=CARTESIAN_POINT('Ctrl Pts',(20.2589177697175,21.4876664642032,40.0128732109645));
#56942=CARTESIAN_POINT('Ctrl Pts',(20.3256208080778,21.4921186786744,40.0014504059393));
#56943=CARTESIAN_POINT('Ctrl Pts',(20.3543685404356,21.4940374978641,39.996527395688));
#56944=CARTESIAN_POINT('Ctrl Pts',(20.3829819219436,21.4959563170538,39.9909561758273));
#56945=CARTESIAN_POINT('Ctrl Pts',(20.4114299415252,21.4978751362435,39.984746126171));
#56946=CARTESIAN_POINT('Ctrl Pts',(20.4776508976573,21.5023417403606,39.9702904476417));
#56947=CARTESIAN_POINT('Ctrl Pts',(20.5432377940952,21.5068083444777,39.952312427416));
#56948=CARTESIAN_POINT('Ctrl Pts',(20.6077891663749,21.5112749485948,39.9308836353349));
#56949=CARTESIAN_POINT('Ctrl Pts',(20.6754263324151,21.5159550728685,39.9084304679298));
#56950=CARTESIAN_POINT('Ctrl Pts',(20.7419259401755,21.5206351971421,39.8821883482491));
#56951=CARTESIAN_POINT('Ctrl Pts',(20.8068377368834,21.5253153214158,39.8523000380188));
#56952=CARTESIAN_POINT('Ctrl Pts',(20.8686190326334,21.529769737355,39.8238531512054));
#56953=CARTESIAN_POINT('Ctrl Pts',(20.9289616178721,21.5342241532942,39.7921038646062));
#56954=CARTESIAN_POINT('Ctrl Pts',(20.9874947374449,21.5386785692334,39.757225603356));
#56955=CARTESIAN_POINT('Ctrl Pts',(21.045991836734,21.543130244001,39.722368805593));
#56956=CARTESIAN_POINT('Ctrl Pts',(21.102681258503,21.5475819187686,39.6843871042582));
#56957=CARTESIAN_POINT('Ctrl Pts',(21.157216832345,21.5520335935361,39.6434998412172));
#56958=CARTESIAN_POINT('Ctrl Pts',(21.2117374550972,21.5564840478638,39.602623787541));
#56959=CARTESIAN_POINT('Ctrl Pts',(21.2641050095886,21.5609345021915,39.5588440483339));
#56960=CARTESIAN_POINT('Ctrl Pts',(21.3140038091691,21.5653849565192,39.5124222266692));
#56961=CARTESIAN_POINT('Ctrl Pts',(21.3639059550048,21.5698357092981,39.4659972919183));
#56962=CARTESIAN_POINT('Ctrl Pts',(21.4113386595033,21.574286462077,39.4169302594691));
#56963=CARTESIAN_POINT('Ctrl Pts',(21.4560220645719,21.5787372148559,39.3655205665575));
#56964=CARTESIAN_POINT('Ctrl Pts',(21.5007518148429,21.5831925839132,39.3140575520017));
#56965=CARTESIAN_POINT('Ctrl Pts',(21.5427262529987,21.5876479529705,39.2602473999785));
#56966=CARTESIAN_POINT('Ctrl Pts',(21.5817056006401,21.5921033220278,39.2044229035128));
#56967=CARTESIAN_POINT('Ctrl Pts',(21.6207084830151,21.596561381123,39.1485647016434));
#56968=CARTESIAN_POINT('Ctrl Pts',(21.6567124160615,21.6010194402183,39.0906901516005));
#56969=CARTESIAN_POINT('Ctrl Pts',(21.6895222800999,21.6054774993135,39.0311589670654));
#56970=CARTESIAN_POINT('Ctrl Pts',(21.7223860199728,21.6099428788186,38.9715300286277));
#56971=CARTESIAN_POINT('Ctrl Pts',(21.7520450113432,21.6144082583238,38.9102394691559));
#56972=CARTESIAN_POINT('Ctrl Pts',(21.7783515883805,21.618873637829,38.8476684994063));
#56973=CARTESIAN_POINT('Ctrl Pts',(21.7876288876848,21.6204484022735,38.8256021692523));
#56974=CARTESIAN_POINT('Ctrl Pts',(21.7964896994039,21.6220231667181,38.8033767407199));
#56975=CARTESIAN_POINT('Ctrl Pts',(21.8049290351548,21.6235979311626,38.7810093501232));
#56976=CARTESIAN_POINT('Ctrl Pts',(21.8288495946408,21.6280614633273,38.7176109366569));
#56977=CARTESIAN_POINT('Ctrl Pts',(21.8494717851415,21.632524995492,38.652828802607));
#56978=CARTESIAN_POINT('Ctrl Pts',(21.866637600227,21.6369885276567,38.5870386291853));
#56979=CARTESIAN_POINT('Ctrl Pts',(21.8846378602152,21.6416690359244,38.5180503393572));
#56980=CARTESIAN_POINT('Ctrl Pts',(21.8988368583806,21.6463495441921,38.4479539776668));
#56981=CARTESIAN_POINT('Ctrl Pts',(21.9091096038987,21.6510300524598,38.3772058390467));
#56982=CARTESIAN_POINT('Ctrl Pts',(21.9188801237923,21.6554817347351,38.3099165156038));
#56983=CARTESIAN_POINT('Ctrl Pts',(21.9250992104239,21.6599334170103,38.2420382053687));
#56984=CARTESIAN_POINT('Ctrl Pts',(21.9277111001389,21.6643850992856,38.1739761535979));
#56985=CARTESIAN_POINT('Ctrl Pts',(21.9303214576001,21.6688341700006,38.1059540301361));
#56986=CARTESIAN_POINT('Ctrl Pts',(21.9293287975894,21.6732832407157,38.0377488693417));
#56987=CARTESIAN_POINT('Ctrl Pts',(21.9247292680504,21.6777323114308,37.96977019692));
#56988=CARTESIAN_POINT('Ctrl Pts',(21.9201308633023,21.6821802941488,37.9018081483282));
#56989=CARTESIAN_POINT('Ctrl Pts',(21.9119273736502,21.6866282768668,37.834072968505));
#56990=CARTESIAN_POINT('Ctrl Pts',(21.9001669892711,21.6910762595848,37.7669715180585));
#56991=CARTESIAN_POINT('Ctrl Pts',(21.888405457762,21.6955246761675,37.69986352241));
#56992=CARTESIAN_POINT('Ctrl Pts',(21.8730864303068,21.6999730927501,37.6333898626534));
#56993=CARTESIAN_POINT('Ctrl Pts',(21.8543093192622,21.7044215093328,37.5679478358305));
#56994=CARTESIAN_POINT('Ctrl Pts',(21.835511817859,21.7088747565206,37.5024347444871));
#56995=CARTESIAN_POINT('Ctrl Pts',(21.8132488761256,21.7133280037083,37.437955994717));
#56996=CARTESIAN_POINT('Ctrl Pts',(21.7876696778375,21.7177812508961,37.3748933320949));
#56997=CARTESIAN_POINT('Ctrl Pts',(21.7620743308935,21.7222373095073,37.3117908567617));
#56998=CARTESIAN_POINT('Ctrl Pts',(21.733158769686,21.7266933681184,37.2501066927458));
#56999=CARTESIAN_POINT('Ctrl Pts',(21.701119016288,21.7311494267296,37.1901996651334));
#57000=CARTESIAN_POINT('Ctrl Pts',(21.6690252080924,21.7356130032309,37.1301915673846));
#57001=CARTESIAN_POINT('Ctrl Pts',(21.6337969447907,21.7400765797321,37.0719670086048));
#57002=CARTESIAN_POINT('Ctrl Pts',(21.5956740511215,21.7445401562334,37.0158566148901));
#57003=CARTESIAN_POINT('Ctrl Pts',(21.582063951989,21.7461336795162,36.9958248715643));
#57004=CARTESIAN_POINT('Ctrl Pts',(21.5680852976313,21.7477272027989,36.9760622789677));
#57005=CARTESIAN_POINT('Ctrl Pts',(21.553750203327,21.7493207260817,36.9565828134224));
#57006=CARTESIAN_POINT('Ctrl Pts',(21.5517133215352,21.7495471507211,36.953814964963));
#57007=CARTESIAN_POINT('Ctrl Pts',(21.5496690309495,21.7497735753606,36.9510525417979));
#57008=CARTESIAN_POINT('Ctrl Pts',(21.5476173497497,21.75,36.9482955693174));
#57009=CARTESIAN_POINT('',(21.45785946511,21.75,39.3634034735148));
#57010=CARTESIAN_POINT('Origin',(20.,21.75,38.1));
#57011=CARTESIAN_POINT('',(18.0708701150598,21.4433318344123,38.100666281098));
#57012=CARTESIAN_POINT('Ctrl Pts',(18.0708701150598,21.4433318344123,38.100666281098));
#57013=CARTESIAN_POINT('Ctrl Pts',(18.0708957469507,21.4481676676054,38.1748800730484));
#57014=CARTESIAN_POINT('Ctrl Pts',(18.0752081170122,21.4530035007986,38.2489637478113));
#57015=CARTESIAN_POINT('Ctrl Pts',(18.0837371745069,21.4578393339917,38.3224395210687));
#57016=CARTESIAN_POINT('Ctrl Pts',(18.0922900823321,21.462688689924,38.3961207591715));
#57017=CARTESIAN_POINT('Ctrl Pts',(18.105083161469,21.4675380458563,38.469190363243));
#57018=CARTESIAN_POINT('Ctrl Pts',(18.1219954280233,21.4723874017887,38.541181804401));
#57019=CARTESIAN_POINT('Ctrl Pts',(18.1389805387895,21.4772576447801,38.6134833258064));
#57020=CARTESIAN_POINT('Ctrl Pts',(18.160120250225,21.4821278877716,38.684697057785));
#57021=CARTESIAN_POINT('Ctrl Pts',(18.1852433867281,21.486998130763,38.7543706835472));
#57022=CARTESIAN_POINT('Ctrl Pts',(18.2051143996883,21.490850223896,38.8094786721667));
#57023=CARTESIAN_POINT('Ctrl Pts',(18.2274764284197,21.4947023170289,38.8636235298763));
#57024=CARTESIAN_POINT('Ctrl Pts',(18.252224385491,21.4985544101619,38.9165922839629));
#57025=CARTESIAN_POINT('Ctrl Pts',(18.2805717918491,21.5029667682831,38.9772650413967));
#57026=CARTESIAN_POINT('Ctrl Pts',(18.3121450401223,21.5073791264044,39.0365939290971));
#57027=CARTESIAN_POINT('Ctrl Pts',(18.3467935985325,21.5117914845257,39.0942088065628));
#57028=CARTESIAN_POINT('Ctrl Pts',(18.3813893343138,21.5161971158922,39.1517358486485));
#57029=CARTESIAN_POINT('Ctrl Pts',(18.4190508245653,21.5206027472587,39.2075536347135));
#57030=CARTESIAN_POINT('Ctrl Pts',(18.4595803006785,21.5250083786252,39.2613137848326));
#57031=CARTESIAN_POINT('Ctrl Pts',(18.5000634584664,21.5294089751014,39.3150124962074));
#57032=CARTESIAN_POINT('Ctrl Pts',(18.5434077962888,21.5338095715776,39.366657837327));
#57033=CARTESIAN_POINT('Ctrl Pts',(18.5893716704543,21.5382101680538,39.415929433056));
#57034=CARTESIAN_POINT('Ctrl Pts',(18.6353079755125,21.5426081250545,39.4651714757082));
#57035=CARTESIAN_POINT('Ctrl Pts',(18.6838603595823,21.5470060820553,39.5120422270587));
#57036=CARTESIAN_POINT('Ctrl Pts',(18.7347473629116,21.5514040390561,39.5562548956968));
#57037=CARTESIAN_POINT('Ctrl Pts',(18.7856222591027,21.5558009496861,39.6004570451678));
#57038=CARTESIAN_POINT('Ctrl Pts',(18.8388302921501,21.5601978603161,39.6420020359081));
#57039=CARTESIAN_POINT('Ctrl Pts',(18.8940551187641,21.5645947709461,39.6806417926172));
#57040=CARTESIAN_POINT('Ctrl Pts',(18.9492867909995,21.5689922266133,39.7192863390769));
#57041=CARTESIAN_POINT('Ctrl Pts',(19.0065353380151,21.5733896822805,39.7550246503077));
#57042=CARTESIAN_POINT('Ctrl Pts',(19.0654551368492,21.5777871379478,39.7876517578157));
#57043=CARTESIAN_POINT('Ctrl Pts',(19.1244473456659,21.5821899979051,39.820318962682));
#57044=CARTESIAN_POINT('Ctrl Pts',(19.1851144618776,21.5865928578625,39.8498670911014));
#57045=CARTESIAN_POINT('Ctrl Pts',(19.2470869161592,21.5909957178198,39.8761375073686));
#57046=CARTESIAN_POINT('Ctrl Pts',(19.3091017949215,21.5954015918429,39.9024259075736));
#57047=CARTESIAN_POINT('Ctrl Pts',(19.3724233142563,21.5998074658659,39.9254319640702));
#57048=CARTESIAN_POINT('Ctrl Pts',(19.436665530953,21.6042133398889,39.9450465665895));
#57049=CARTESIAN_POINT('Ctrl Pts',(19.5010320913046,21.6086277416762,39.9646991340404));
#57050=CARTESIAN_POINT('Ctrl Pts',(19.5663224156939,21.6130421434635,39.980947030881));
#57051=CARTESIAN_POINT('Ctrl Pts',(19.6321400638034,21.6174565452508,39.9937321944355));
#57052=CARTESIAN_POINT('Ctrl Pts',(19.6660381856185,21.6197300985275,40.0003169485864));
#57053=CARTESIAN_POINT('Ctrl Pts',(19.7000760964438,21.6220036518042,40.0059840359317));
#57054=CARTESIAN_POINT('Ctrl Pts',(19.7341994520756,21.6242772050809,40.0107309139759));
#57055=CARTESIAN_POINT('Ctrl Pts',(19.802951938091,21.6288580101328,40.0202950280646));
#57056=CARTESIAN_POINT('Ctrl Pts',(19.8723324705866,21.6334388151846,40.0261595313805));
#57057=CARTESIAN_POINT('Ctrl Pts',(19.9419211784638,21.6380196202364,40.0282555347746));
#57058=CARTESIAN_POINT('Ctrl Pts',(20.01280182287,21.6426854693932,40.0303904511395));
#57059=CARTESIAN_POINT('Ctrl Pts',(20.0838979863156,21.64735131855,40.0286153721321));
#57060=CARTESIAN_POINT('Ctrl Pts',(20.1547573315076,21.6520171677069,40.0229125630784));
#57061=CARTESIAN_POINT('Ctrl Pts',(20.2240947373107,21.6565828022823,40.0173322407581));
#57062=CARTESIAN_POINT('Ctrl Pts',(20.2932049107954,21.6611484368578,40.0079912596888));
#57063=CARTESIAN_POINT('Ctrl Pts',(20.3616628893468,21.6657140714332,39.9949254632754));
#57064=CARTESIAN_POINT('Ctrl Pts',(20.4300562009068,21.6702753932045,39.9818720091157));
#57065=CARTESIAN_POINT('Ctrl Pts',(20.4977980913606,21.6748367149759,39.9651008177934));
#57066=CARTESIAN_POINT('Ctrl Pts',(20.5644705860265,21.6793980367472,39.9446993018947));
#57067=CARTESIAN_POINT('Ctrl Pts',(20.631098306068,21.6839562953143,39.9243114868515));
#57068=CARTESIAN_POINT('Ctrl Pts',(20.6966576187536,21.6885145538814,39.9002983283355));
#57069=CARTESIAN_POINT('Ctrl Pts',(20.7607439627118,21.6930728124485,39.8727975575619));
#57070=CARTESIAN_POINT('Ctrl Pts',(20.8274407664053,21.6978167447444,39.8441765847241));
#57071=CARTESIAN_POINT('Ctrl Pts',(20.8925415197652,21.7025606770404,39.8117779140257));
#57072=CARTESIAN_POINT('Ctrl Pts',(20.9556123210989,21.7073046093363,39.7758125338665));
#57073=CARTESIAN_POINT('Ctrl Pts',(21.0161992792482,21.7118617169266,39.7412635359712));
#57074=CARTESIAN_POINT('Ctrl Pts',(21.0749127748468,21.7164188245168,39.7034237799828));
#57075=CARTESIAN_POINT('Ctrl Pts',(21.1313942764615,21.720975932107,39.6625266551615));
#57076=CARTESIAN_POINT('Ctrl Pts',(21.1878812173633,21.7255334785562,39.6216255918612));
#57077=CARTESIAN_POINT('Ctrl Pts',(21.2421353687718,21.7300910250055,39.577666850821));
#57078=CARTESIAN_POINT('Ctrl Pts',(21.2938295118927,21.7346485714547,39.5309254875973));
#57079=CARTESIAN_POINT('Ctrl Pts',(21.3455582994798,21.7392091722879,39.4841527991696));
#57080=CARTESIAN_POINT('Ctrl Pts',(21.3947233205039,21.7437697731212,39.4345940833591));
#57081=CARTESIAN_POINT('Ctrl Pts',(21.441033354978,21.7483303739544,39.3825620557076));
#57082=CARTESIAN_POINT('Ctrl Pts',(21.4466846892762,21.7488869159696,39.3762124516571));
#57083=CARTESIAN_POINT('Ctrl Pts',(21.4522935554523,21.7494434579848,39.3698260568356));
#57084=CARTESIAN_POINT('Ctrl Pts',(21.45785946511,21.75,39.3634034735148));
#57085=CARTESIAN_POINT('Ctrl Pts',(18.0708700849959,21.444817201297,38.1005726573522));
#57086=CARTESIAN_POINT('Ctrl Pts',(18.0708621447113,21.4431312111911,38.0738239558221));
#57087=CARTESIAN_POINT('Ctrl Pts',(18.0714105371302,21.4414297588578,38.0470788578902));
#57088=CARTESIAN_POINT('Ctrl Pts',(18.0728453930802,21.4391969107969,38.0123541562582));
#57089=CARTESIAN_POINT('Ctrl Pts',(18.0732257813741,21.438680981368,38.0043559712711));
#57090=CARTESIAN_POINT('Ctrl Pts',(18.073992734373,21.4377584137641,37.9901006430405));
#57091=CARTESIAN_POINT('Ctrl Pts',(18.0743600285079,21.4373523687922,37.9838425439747));
#57092=CARTESIAN_POINT('Ctrl Pts',(18.0751569577228,21.4365370228772,37.9713089544374));
#57093=CARTESIAN_POINT('Ctrl Pts',(18.0755867960074,21.436127720581,37.9650335546474));
#57094=CARTESIAN_POINT('Ctrl Pts',(18.0765727849264,21.4352493641535,37.9516025025255));
#57095=CARTESIAN_POINT('Ctrl Pts',(18.0771381923196,21.4347800319043,37.9444476448115));
#57096=CARTESIAN_POINT('Ctrl Pts',(18.0787389410611,21.4335356335069,37.9255356745032));
#57097=CARTESIAN_POINT('Ctrl Pts',(18.0798422632143,21.4327584961842,37.9137847668753));
#57098=CARTESIAN_POINT('Ctrl Pts',(18.0850286803668,21.4294161828354,37.8635084173905));
#57099=CARTESIAN_POINT('Ctrl Pts',(18.0901637139054,21.4268191404273,37.8251028789182));
#57100=CARTESIAN_POINT('Ctrl Pts',(18.1216694805466,21.4136383917863,37.6335699464261));
#57101=CARTESIAN_POINT('Ctrl Pts',(18.1653144164803,21.4025341672775,37.4838857843554));
#57102=CARTESIAN_POINT('Ctrl Pts',(18.2558626995096,21.3862392303953,37.2722743844936));
#57103=CARTESIAN_POINT('Ctrl Pts',(18.2892901562238,21.3809912022391,37.2052269950852));
#57104=CARTESIAN_POINT('Ctrl Pts',(18.333534336177,21.374975598533,37.1280777750873));
#57105=CARTESIAN_POINT('Ctrl Pts',(18.3406693203647,21.3740304301354,37.115945965412));
#57106=CARTESIAN_POINT('Ctrl Pts',(18.3507486549677,21.3727302879657,37.0992291893859));
#57107=CARTESIAN_POINT('Ctrl Pts',(18.3535804122822,21.3723687334392,37.0945773240205));
#57108=CARTESIAN_POINT('Ctrl Pts',(18.3584105676622,21.3717583594154,37.0867177222553));
#57109=CARTESIAN_POINT('Ctrl Pts',(18.3603987412837,21.371508906987,37.083503786643));
#57110=CARTESIAN_POINT('Ctrl Pts',(18.36418960164,21.3710366822543,37.0774158192065));
#57111=CARTESIAN_POINT('Ctrl Pts',(18.3659904051399,21.37081380124,37.0745407320344));
#57112=CARTESIAN_POINT('Ctrl Pts',(18.3707638299532,21.3702267695268,37.0669641833853));
#57113=CARTESIAN_POINT('Ctrl Pts',(18.3737492241718,21.3698634419188,37.0622707905371));
#57114=CARTESIAN_POINT('Ctrl Pts',(18.3843722057136,21.3685837511249,37.0457286357568));
#57115=CARTESIAN_POINT('Ctrl Pts',(18.3921195428945,21.3676741976809,37.0339504034153));
#57116=CARTESIAN_POINT('Ctrl Pts',(18.4740450669705,21.3582870123036,36.9123246602368));
#57117=CARTESIAN_POINT('Ctrl Pts',(18.5592388113022,21.3504410898259,36.8102989275548));
#57118=CARTESIAN_POINT('Ctrl Pts',(18.7211152388735,21.3369263369857,36.6526888317364));
#57119=CARTESIAN_POINT('Ctrl Pts',(18.7926282984253,21.3313211867468,36.5925161895644));
#57120=CARTESIAN_POINT('Ctrl Pts',(18.8940316318945,21.3235546398041,36.5190531102441));
#57121=CARTESIAN_POINT('Ctrl Pts',(18.9203098247461,21.3215577163147,36.500991539715));
#57122=CARTESIAN_POINT('Ctrl Pts',(18.959926887435,21.3185618140299,36.4751838048304));
#57123=CARTESIAN_POINT('Ctrl Pts',(18.9729312209725,21.3175806979886,36.4669325030817));
#57124=CARTESIAN_POINT('Ctrl Pts',(18.9938730382735,21.316003560162,36.4539939155586));
#57125=CARTESIAN_POINT('Ctrl Pts',(19.0017479069026,21.3154111298052,36.4492061767031));
#57126=CARTESIAN_POINT('Ctrl Pts',(19.0167546023702,21.3142831780889,36.4402290958583));
#57127=CARTESIAN_POINT('Ctrl Pts',(19.023879674651,21.3137480614945,36.4360288244223));
#57128=CARTESIAN_POINT('Ctrl Pts',(19.0365197796093,21.3127993908049,36.4286865323672));
#57129=CARTESIAN_POINT('Ctrl Pts',(19.0420237565756,21.3123865175655,36.4255256473703));
#57130=CARTESIAN_POINT('Ctrl Pts',(19.0528328874467,21.3115760538106,36.4193887962615));
#57131=CARTESIAN_POINT('Ctrl Pts',(19.0581367202113,21.311178547083,36.4164106444847));
#57132=CARTESIAN_POINT('Ctrl Pts',(19.0708300795819,21.3102275794654,36.4093619577762));
#57133=CARTESIAN_POINT('Ctrl Pts',(19.0782323473301,21.3096733036281,36.4053147426393));
#57134=CARTESIAN_POINT('Ctrl Pts',(19.1049635197194,21.3076725702162,36.3909263326198));
#57135=CARTESIAN_POINT('Ctrl Pts',(19.1244412025445,21.306216346879,36.3808665476503));
#57136=CARTESIAN_POINT('Ctrl Pts',(19.2249999922806,21.2987033875505,36.3310824162271));
#57137=CARTESIAN_POINT('Ctrl Pts',(19.3085497672861,21.2924705746517,36.2967918114816));
#57138=CARTESIAN_POINT('Ctrl Pts',(19.3941043260691,21.2861174117667,36.2684888782178));
#57139=CARTESIAN_POINT('Origin',(20.,21.75,38.1));
#57140=CARTESIAN_POINT('',(17.883581703528,21.75,39.1520285334812));
#57141=CARTESIAN_POINT('Origin',(20.,21.75,38.1));
#57142=CARTESIAN_POINT('Ctrl Pts',(17.883581703528,21.75,39.1520285334812));
#57143=CARTESIAN_POINT('Ctrl Pts',(17.9277932180658,21.7500000000001,39.22297989717));
#57144=CARTESIAN_POINT('Ctrl Pts',(17.9760877855519,21.7500000000001,39.2913445416396));
#57145=CARTESIAN_POINT('Ctrl Pts',(18.0281130771647,21.7500000000001,39.3569276629741));
#57146=CARTESIAN_POINT('Ctrl Pts',(18.0729426874247,21.7500000000001,39.4134399030387));
#57147=CARTESIAN_POINT('Ctrl Pts',(18.1205434589414,21.7500000000001,39.4678864547816));
#57148=CARTESIAN_POINT('Ctrl Pts',(18.1707077965432,21.7500000000001,39.5201173219611));
#57149=CARTESIAN_POINT('Ctrl Pts',(18.1818183450819,21.7500000000001,39.5316855716931));
#57150=CARTESIAN_POINT('Ctrl Pts',(18.1930524042112,21.7500000000001,39.5431425628877));
#57151=CARTESIAN_POINT('Ctrl Pts',(18.2044015768659,21.7500000000001,39.554480823305));
#57152=CARTESIAN_POINT('Ctrl Pts',(18.2631474317285,21.75,39.6131701939873));
#57153=CARTESIAN_POINT('Ctrl Pts',(18.325021894181,21.7500000000001,39.6687306291731));
#57154=CARTESIAN_POINT('Ctrl Pts',(18.3896927432761,21.7500000000001,39.7209522333743));
#57155=CARTESIAN_POINT('Ctrl Pts',(18.4364046733552,21.75,39.7586720400291));
#57156=CARTESIAN_POINT('Ctrl Pts',(18.4845762623831,21.75,39.7946490527158));
#57157=CARTESIAN_POINT('Ctrl Pts',(18.5340885148965,21.7500000000001,39.8287884171533));
#57158=CARTESIAN_POINT('Ctrl Pts',(18.5462898292441,21.7500000000001,39.8372013875997));
#57159=CARTESIAN_POINT('Ctrl Pts',(18.5585725745402,21.75,39.8455026943682));
#57160=CARTESIAN_POINT('Ctrl Pts',(18.570934994616,21.75,39.8536907833519));
#57161=CARTESIAN_POINT('Ctrl Pts',(18.582644131702,21.75,39.8614461788));
#57162=CARTESIAN_POINT('Ctrl Pts',(18.5944162834139,21.7500000000001,39.8690943988968));
#57163=CARTESIAN_POINT('Ctrl Pts',(18.6062494302586,21.7500000000001,39.8766343834877));
#57164=CARTESIAN_POINT('Ctrl Pts',(18.674676426647,21.75,39.9202355071059));
#57165=CARTESIAN_POINT('Ctrl Pts',(18.7451450843928,21.75,39.9602236491718));
#57166=CARTESIAN_POINT('Ctrl Pts',(18.8173443875306,21.75,39.99641011754));
#57167=CARTESIAN_POINT('Ctrl Pts',(18.8887220445928,21.75,40.0321847748735));
#57168=CARTESIAN_POINT('Ctrl Pts',(18.9617921137688,21.75,40.0642440963409));
#57169=CARTESIAN_POINT('Ctrl Pts',(19.0362665833562,21.75,40.0923568791639));
#57170=CARTESIAN_POINT('Ctrl Pts',(19.1085593322196,21.7500000000001,40.1196461013596));
#57171=CARTESIAN_POINT('Ctrl Pts',(19.1821761823731,21.7500000000001,40.1432167252266));
#57172=CARTESIAN_POINT('Ctrl Pts',(19.256853078291,21.75,40.1628082746128));
#57173=CARTESIAN_POINT('Ctrl Pts',(19.2785430184841,21.75,40.1684986495173));
#57174=CARTESIAN_POINT('Ctrl Pts',(19.3003223413584,21.75,40.1738530151002));
#57175=CARTESIAN_POINT('Ctrl Pts',(19.322184426739,21.75,40.1788641632569));
#57176=CARTESIAN_POINT('Ctrl Pts',(19.3343537500359,21.75,40.1816535715383));
#57177=CARTESIAN_POINT('Ctrl Pts',(19.3465487155545,21.75,40.1843366275288));
#57178=CARTESIAN_POINT('Ctrl Pts',(19.3587681675008,21.75,40.1869120359227));
#57179=CARTESIAN_POINT('Ctrl Pts',(19.3718709904236,21.75,40.1896736262369));
#57180=CARTESIAN_POINT('Ctrl Pts',(19.3849932065373,21.75,40.1923095652966));
#57181=CARTESIAN_POINT('Ctrl Pts',(19.3981287272652,21.75,40.1948179331189));
#57182=CARTESIAN_POINT('Ctrl Pts',(19.4729976305839,21.75,40.2091149489636));
#57183=CARTESIAN_POINT('Ctrl Pts',(19.548347373974,21.75,40.2192819902038));
#57184=CARTESIAN_POINT('Ctrl Pts',(19.6239185624981,21.75,40.2251172383339));
#57185=CARTESIAN_POINT('Ctrl Pts',(19.6505037576844,21.75,40.2271700207968));
#57186=CARTESIAN_POINT('Ctrl Pts',(19.6771163593369,21.75,40.2286862521491));
#57187=CARTESIAN_POINT('Ctrl Pts',(19.703744980525,21.75,40.2296555953342));
#57188=CARTESIAN_POINT('Ctrl Pts',(19.7813518609821,21.75,40.2324806646516));
#57189=CARTESIAN_POINT('Ctrl Pts',(19.8590961441614,21.75,40.2306641911219));
#57190=CARTESIAN_POINT('Ctrl Pts',(19.9366408209257,21.75,40.2243619036731));
#57191=CARTESIAN_POINT('Ctrl Pts',(20.0110102784872,21.75,40.2183176757708));
#57192=CARTESIAN_POINT('Ctrl Pts',(20.0851968055271,21.75,40.2081466928086));
#57193=CARTESIAN_POINT('Ctrl Pts',(20.1588811181686,21.75,40.1939470315399));
#57194=CARTESIAN_POINT('Ctrl Pts',(20.1744047711941,21.75,40.1909554773445));
#57195=CARTESIAN_POINT('Ctrl Pts',(20.1899095582806,21.75,40.1877841069774));
#57196=CARTESIAN_POINT('Ctrl Pts',(20.2053667593194,21.75,40.184439537327));
#57197=CARTESIAN_POINT('Ctrl Pts',(20.2795029508407,21.75,40.1683982336304));
#57198=CARTESIAN_POINT('Ctrl Pts',(20.3526602952137,21.75,40.1483566584602));
#57199=CARTESIAN_POINT('Ctrl Pts',(20.4245337957823,21.75,40.1244889058307));
#57200=CARTESIAN_POINT('Ctrl Pts',(20.4961137461482,21.75,40.1007186353549));
#57201=CARTESIAN_POINT('Ctrl Pts',(20.566421180313,21.75,40.0731527585199));
#57202=CARTESIAN_POINT('Ctrl Pts',(20.6351295047781,21.75,40.0419190370673));
#57203=CARTESIAN_POINT('Ctrl Pts',(20.7032602977131,21.75,40.0109478523462));
#57204=CARTESIAN_POINT('Ctrl Pts',(20.7698195230793,21.75,39.9763696283126));
#57205=CARTESIAN_POINT('Ctrl Pts',(20.8344517025453,21.75,39.9382744436647));
#57206=CARTESIAN_POINT('Ctrl Pts',(20.8581546852447,21.75,39.9243035469674));
#57207=CARTESIAN_POINT('Ctrl Pts',(20.881598069502,21.75,39.9098593416072));
#57208=CARTESIAN_POINT('Ctrl Pts',(20.9047627456548,21.75,39.8949453334425));
#57209=CARTESIAN_POINT('Ctrl Pts',(20.9147055515707,21.75,39.8885439018995));
#57210=CARTESIAN_POINT('Ctrl Pts',(20.924595831536,21.75,39.8820565812407));
#57211=CARTESIAN_POINT('Ctrl Pts',(20.9344220826436,21.75,39.8754905971792));
#57212=CARTESIAN_POINT('Ctrl Pts',(20.9953083722281,21.75,39.8348058637445));
#57213=CARTESIAN_POINT('Ctrl Pts',(21.0538466168534,21.75,39.7910353867451));
#57214=CARTESIAN_POINT('Ctrl Pts',(21.109739867734,21.75,39.7443037617988));
#57215=CARTESIAN_POINT('Ctrl Pts',(21.164047120997,21.75,39.6988981689703));
#57216=CARTESIAN_POINT('Ctrl Pts',(21.2158578668268,21.75,39.6506964389093));
#57217=CARTESIAN_POINT('Ctrl Pts',(21.2648614302667,21.75,39.5997839374079));
#57218=CARTESIAN_POINT('Ctrl Pts',(21.3132198492097,21.75,39.5495417120633));
#57219=CARTESIAN_POINT('Ctrl Pts',(21.3588450296455,21.75,39.4966591220955));
#57220=CARTESIAN_POINT('Ctrl Pts',(21.4013929325376,21.75,39.4411979346476));
#57221=CARTESIAN_POINT('Ctrl Pts',(21.4208730776474,21.75,39.4158055673156));
#57222=CARTESIAN_POINT('Ctrl Pts',(21.4397074908361,21.75,39.3898724435325));
#57223=CARTESIAN_POINT('Ctrl Pts',(21.45785946511,21.75,39.3634034735148));
#57224=CARTESIAN_POINT('Ctrl Pts',(21.5504048836412,21.75,36.9462211449553));
#57225=CARTESIAN_POINT('Ctrl Pts',(21.5152004352802,21.75,36.885761931632));
#57226=CARTESIAN_POINT('Ctrl Pts',(21.4764419646285,21.75,36.8275241874393));
#57227=CARTESIAN_POINT('Ctrl Pts',(21.434486940511,21.75,36.7716059964527));
#57228=CARTESIAN_POINT('Ctrl Pts',(21.3986418022227,21.75,36.7238311391881));
#57229=CARTESIAN_POINT('Ctrl Pts',(21.3604621811875,21.75,36.6777494040042));
#57230=CARTESIAN_POINT('Ctrl Pts',(21.3201424774326,21.75,36.63343135754));
#57231=CARTESIAN_POINT('Ctrl Pts',(21.3089460542563,21.75,36.62112463015));
#57232=CARTESIAN_POINT('Ctrl Pts',(21.2975828442927,21.75,36.6089522848169));
#57233=CARTESIAN_POINT('Ctrl Pts',(21.286061915094,21.75,36.5969214204494));
#57234=CARTESIAN_POINT('Ctrl Pts',(21.2354736072089,21.75,36.54409399132));
#57235=CARTESIAN_POINT('Ctrl Pts',(21.1819369929417,21.75,36.494083574989));
#57236=CARTESIAN_POINT('Ctrl Pts',(21.1258151639906,21.75,36.4470065366406));
#57237=CARTESIAN_POINT('Ctrl Pts',(21.0820213593962,21.75,36.4102706950465));
#57238=CARTESIAN_POINT('Ctrl Pts',(21.0366521413219,21.75,36.3753212937733));
#57239=CARTESIAN_POINT('Ctrl Pts',(20.9898607439523,21.75,36.3422241650772));
#57240=CARTESIAN_POINT('Ctrl Pts',(20.9774656288495,21.75,36.3334566833857));
#57241=CARTESIAN_POINT('Ctrl Pts',(20.9649706346163,21.75,36.3248192401923));
#57242=CARTESIAN_POINT('Ctrl Pts',(20.9523784433775,21.75,36.316313194054));
#57243=CARTESIAN_POINT('Ctrl Pts',(20.9403661339154,21.75,36.3081988590208));
#57244=CARTESIAN_POINT('Ctrl Pts',(20.928272392671,21.75,36.3002088768254));
#57245=CARTESIAN_POINT('Ctrl Pts',(20.9161036367489,21.75,36.2923464263246));
#57246=CARTESIAN_POINT('Ctrl Pts',(20.8521530733458,21.75,36.251026825334));
#57247=CARTESIAN_POINT('Ctrl Pts',(20.7861025993975,21.75,36.2132056325107));
#57248=CARTESIAN_POINT('Ctrl Pts',(20.7183291552492,21.75,36.1790042619072));
#57249=CARTESIAN_POINT('Ctrl Pts',(20.6505632332243,21.75,36.1448066872879));
#57250=CARTESIAN_POINT('Ctrl Pts',(20.5810738836283,21.7499999999999,36.1142275037117));
#57251=CARTESIAN_POINT('Ctrl Pts',(20.5101966664877,21.75,36.0874199201387));
#57252=CARTESIAN_POINT('Ctrl Pts',(20.4392415021213,21.75,36.0605828549234));
#57253=CARTESIAN_POINT('Ctrl Pts',(20.3668945577923,21.75,36.0375250306173));
#57254=CARTESIAN_POINT('Ctrl Pts',(20.2934638749207,21.75,36.0184417253472));
#57255=CARTESIAN_POINT('Ctrl Pts',(20.2698818894381,21.7499999999999,36.0123131941905));
#57256=CARTESIAN_POINT('Ctrl Pts',(20.2461879660648,21.7499999999999,36.0065949361045));
#57257=CARTESIAN_POINT('Ctrl Pts',(20.2223919096731,21.7499999999999,36.0012945023363));
#57258=CARTESIAN_POINT('Ctrl Pts',(20.2103027038764,21.7499999999999,35.9986017017486));
#57259=CARTESIAN_POINT('Ctrl Pts',(20.1981910225857,21.7499999999999,35.9960176758035));
#57260=CARTESIAN_POINT('Ctrl Pts',(20.1860677365327,21.75,35.9935450303039));
#57261=CARTESIAN_POINT('Ctrl Pts',(20.1090016189117,21.75,35.9778267516066));
#57262=CARTESIAN_POINT('Ctrl Pts',(20.0313570587203,21.75,35.9665807998749));
#57263=CARTESIAN_POINT('Ctrl Pts',(19.9534981235114,21.75,35.9599575860445));
#57264=CARTESIAN_POINT('Ctrl Pts',(19.9266953868611,21.75,35.9576775618494));
#57265=CARTESIAN_POINT('Ctrl Pts',(19.8998669686043,21.75,35.9559457213365));
#57266=CARTESIAN_POINT('Ctrl Pts',(19.873026956781,21.75,35.9547694100208));
#57267=CARTESIAN_POINT('Ctrl Pts',(19.796957402718,21.75,35.9514355263469));
#57268=CARTESIAN_POINT('Ctrl Pts',(19.7207955629966,21.75,35.9525599283831));
#57269=CARTESIAN_POINT('Ctrl Pts',(19.6448113276275,21.75,35.9579222236047));
#57270=CARTESIAN_POINT('Ctrl Pts',(19.5688270922584,21.75,35.9632845188263));
#57271=CARTESIAN_POINT('Ctrl Pts',(19.4930196712211,21.75,35.9728849486848));
#57272=CARTESIAN_POINT('Ctrl Pts',(19.4176534273628,21.75,35.9865551032572));
#57273=CARTESIAN_POINT('Ctrl Pts',(19.4003670978281,21.75,35.9896905493751));
#57274=CARTESIAN_POINT('Ctrl Pts',(19.3830988100698,21.75,35.9930415012686));
#57275=CARTESIAN_POINT('Ctrl Pts',(19.3658826346092,21.75,35.9965995273322));
#57276=CARTESIAN_POINT('Ctrl Pts',(19.2892535472449,21.75,36.0124362786883));
#57277=CARTESIAN_POINT('Ctrl Pts',(19.2135567969655,21.75,36.0323869962119));
#57278=CARTESIAN_POINT('Ctrl Pts',(19.1390725001544,21.75,36.0561990525511));
#57279=CARTESIAN_POINT('Ctrl Pts',(19.0622735673651,21.75,36.0807510801953));
#57280=CARTESIAN_POINT('Ctrl Pts',(18.9867627690563,21.75,36.1094081944649));
#57281=CARTESIAN_POINT('Ctrl Pts',(18.912841317696,21.75,36.1419496464839));
#57282=CARTESIAN_POINT('Ctrl Pts',(18.8389198663356,21.75,36.1744910985028));
#57283=CARTESIAN_POINT('Ctrl Pts',(18.7665868250202,21.75,36.2109172193929));
#57284=CARTESIAN_POINT('Ctrl Pts',(18.6961512285367,21.75,36.2510593784398));
#57285=CARTESIAN_POINT('Ctrl Pts',(18.6664445302591,21.75,36.2679896106882));
#57286=CARTESIAN_POINT('Ctrl Pts',(18.6370755244225,21.75,36.2855814538998));
#57287=CARTESIAN_POINT('Ctrl Pts',(18.6080684406704,21.75,36.3038248169416));
#57288=CARTESIAN_POINT('Ctrl Pts',(18.5950040138221,21.75,36.3120413989311));
#57289=CARTESIAN_POINT('Ctrl Pts',(18.5820114468336,21.75,36.320391318453));
#57290=CARTESIAN_POINT('Ctrl Pts',(18.5691115639433,21.75,36.3288611784974));
#57291=CARTESIAN_POINT('Ctrl Pts',(18.4992480227799,21.75,36.37473247988));
#57292=CARTESIAN_POINT('Ctrl Pts',(18.4319799898637,21.75,36.4241928678248));
#57293=CARTESIAN_POINT('Ctrl Pts',(18.3676173103639,21.75,36.4770057143139));
#57294=CARTESIAN_POINT('Ctrl Pts',(18.3032905441657,21.75,36.5297890921157));
#57295=CARTESIAN_POINT('Ctrl Pts',(18.2418649238884,21.75,36.5859215783093));
#57296=CARTESIAN_POINT('Ctrl Pts',(18.1836636252436,21.75,36.6452170871453));
#57297=CARTESIAN_POINT('Ctrl Pts',(18.1266152525058,21.75,36.7033379945567));
#57298=CARTESIAN_POINT('Ctrl Pts',(18.072663886905,21.75,36.7644983503434));
#57299=CARTESIAN_POINT('Ctrl Pts',(18.0221403945991,21.75,36.8285642992791));
#57300=CARTESIAN_POINT('Ctrl Pts',(17.9954862842875,21.75,36.862362851046));
#57301=CARTESIAN_POINT('Ctrl Pts',(17.9697867357093,21.75,36.8969707358832));
#57302=CARTESIAN_POINT('Ctrl Pts',(17.9450946017473,21.75,36.932372385933));
#57303=CARTESIAN_POINT('Ctrl Pts',(19.1114077309894,-0.12774359558736,36.3915666551543));
#57304=CARTESIAN_POINT('Ctrl Pts',(18.5446637169267,-0.0858359972810003,
36.6863421879098));
#57305=CARTESIAN_POINT('Ctrl Pts',(17.7372336080694,-0.00202080066828049,
37.8791160387151));
#57306=CARTESIAN_POINT('Ctrl Pts',(18.5843637960128,0.123701994250799,39.8818024076985));
#57307=CARTESIAN_POINT('Ctrl Pts',(20.7234950721292,0.249424789169879,40.2555031365194));
#57308=CARTESIAN_POINT('Ctrl Pts',(22.202317510923,0.375147584088957,38.6673870046074));
#57309=CARTESIAN_POINT('Ctrl Pts',(21.6746022358962,0.500870379008037,36.5608878176203));
#57310=CARTESIAN_POINT('Ctrl Pts',(19.6205166436687,0.626593173927117,35.8576992053172));
#57311=CARTESIAN_POINT('Ctrl Pts',(17.9123977241599,0.752315968846196,37.1976370239046));
#57312=CARTESIAN_POINT('Ctrl Pts',(18.1067028033701,0.878038763765275,39.3601034488986));
#57313=CARTESIAN_POINT('Ctrl Pts',(20.0264596815545,1.00376155868435,40.3741087222362));
#57314=CARTESIAN_POINT('Ctrl Pts',(21.9220848862426,1.12948435360343,39.3157005884543));
#57315=CARTESIAN_POINT('Ctrl Pts',(22.0660679021208,1.25520714852251,37.1493647266486));
#57316=CARTESIAN_POINT('Ctrl Pts',(20.3271786047828,1.38092994344159,35.8493829925345));
#57317=CARTESIAN_POINT('Ctrl Pts',(18.2901244766361,1.50665273836067,36.6004471178591));
#57318=CARTESIAN_POINT('Ctrl Pts',(17.8113281044618,1.63237553327975,38.7181005585794));
#57319=CARTESIAN_POINT('Ctrl Pts',(19.3271324331515,1.75809832819883,40.2724593299136));
#57320=CARTESIAN_POINT('Ctrl Pts',(21.4561401039683,1.88382112311791,39.8469939456022));
#57321=CARTESIAN_POINT('Ctrl Pts',(22.2581253366117,2.00954391803699,37.8294419590792));
#57322=CARTESIAN_POINT('Ctrl Pts',(21.0022155117262,2.13526671295606,36.0584575842664));
#57323=CARTESIAN_POINT('Ctrl Pts',(18.8329577355021,2.26098950787515,36.1479897686354));
#57324=CARTESIAN_POINT('Ctrl Pts',(17.7272593230923,2.38671230279422,38.0164454289377));
#57325=CARTESIAN_POINT('Ctrl Pts',(18.6927752719204,2.51243509771331,39.9610467549065));
#57326=CARTESIAN_POINT('Ctrl Pts',(20.8496029381568,2.63815789263238,40.2096223341063));
#57327=CARTESIAN_POINT('Ctrl Pts',(22.2321628639168,2.76388068755146,38.5356380220699));
#57328=CARTESIAN_POINT('Ctrl Pts',(21.5804881745105,2.88960348247054,36.4646441783065));
#57329=CARTESIAN_POINT('Ctrl Pts',(19.4884688755281,3.01532627738962,35.8839974173462));
#57330=CARTESIAN_POINT('Ctrl Pts',(17.8626226927863,3.1410490723087,37.3228579390602));
#57331=CARTESIAN_POINT('Ctrl Pts',(18.1846303029432,3.26677186722778,39.4699505096519));
#57332=CARTESIAN_POINT('Ctrl Pts',(20.1610368520708,3.39249466214686,40.3685675367379));
#57333=CARTESIAN_POINT('Ctrl Pts',(21.9906858577964,3.51821745706594,39.1997733183766));
#57334=CARTESIAN_POINT('Ctrl Pts',(22.0061652337193,3.64394025198502,37.0287238492198));
#57335=CARTESIAN_POINT('Ctrl Pts',(20.1933681766596,3.7696630469041,35.8339593374025));
#57336=CARTESIAN_POINT('Ctrl Pts',(18.2043491044069,3.89538584182318,36.7043032573617));
#57337=CARTESIAN_POINT('Ctrl Pts',(17.851758656844,4.02110863674226,38.8465860083142));
#57338=CARTESIAN_POINT('Ctrl Pts',(19.4569227122844,4.14683143166134,40.3084833247801));
#57339=CARTESIAN_POINT('Ctrl Pts',(21.5570088158898,4.27255422658041,39.7577258770679));
#57340=CARTESIAN_POINT('Ctrl Pts',(22.2381477279983,4.3982770214995,37.6962348654038));
#57341=CARTESIAN_POINT('Ctrl Pts',(20.8795978468344,4.52399981641858,36.0027067052734));
#57342=CARTESIAN_POINT('Ctrl Pts',(18.7194449935648,4.64972261133765,36.2205026172528));
#57343=CARTESIAN_POINT('Ctrl Pts',(17.7262989750634,4.77544540625674,38.1511388840565));
#57344=CARTESIAN_POINT('Ctrl Pts',(18.8052424981953,4.90116820117581,40.0351708059346));
#57345=CARTESIAN_POINT('Ctrl Pts',(20.9730031072704,5.0268909960949,40.1556255713292));
#57346=CARTESIAN_POINT('Ctrl Pts',(22.2540378273918,5.15261379101397,38.40272926675));
#57347=CARTESIAN_POINT('Ctrl Pts',(21.4809026468269,5.27833658593306,36.373947020836));
#57348=CARTESIAN_POINT('Ctrl Pts',(19.3581780290348,5.40405938085213,35.9181668043027));
#57349=CARTESIAN_POINT('Ctrl Pts',(17.8203643467799,5.52978217577121,37.4507543180954));
#57350=CARTESIAN_POINT('Ctrl Pts',(18.2689157107976,5.65550497069029,39.5750182100357));
#57351=CARTESIAN_POINT('Ctrl Pts',(20.2950542826331,5.78122776560936,40.3550553222838));
#57352=CARTESIAN_POINT('Ctrl Pts',(22.0523013482622,5.90695056052845,39.0799952613055));
#57353=CARTESIAN_POINT('Ctrl Pts',(21.9392268045967,6.03267335544753,36.9118371590588));
#57354=CARTESIAN_POINT('Ctrl Pts',(20.0588787554923,6.15839615036661,35.8264862374703));
#57355=CARTESIAN_POINT('Ctrl Pts',(18.1248727926419,6.28411894528568,36.8130541998647));
#57356=CARTESIAN_POINT('Ctrl Pts',(17.8997245173177,6.40984174020477,38.9724531122665));
#57357=CARTESIAN_POINT('Ctrl Pts',(19.5886180682867,6.53556453512385,40.3367602559326));
#57358=CARTESIAN_POINT('Ctrl Pts',(21.6524158784223,6.66128733004292,39.6626430497711));
#57359=CARTESIAN_POINT('Ctrl Pts',(22.2103192800337,6.78701012496201,37.5644440117305));
#57360=CARTESIAN_POINT('Ctrl Pts',(20.7538947583175,6.91273291988108,35.9543126440133));
#57361=CARTESIAN_POINT('Ctrl Pts',(18.6104241267262,7.03845571480017,36.2996082568853));
#57362=CARTESIAN_POINT('Ctrl Pts',(17.7333142007588,7.16417850971926,38.2856529659826));
#57363=CARTESIAN_POINT('Ctrl Pts',(18.921900638238,7.28990130463832,40.1025067546524));
#57364=CARTESIAN_POINT('Ctrl Pts',(21.0929902227223,7.41562409955741,40.0944181881676));
#57365=CARTESIAN_POINT('Ctrl Pts',(22.2680061876885,7.5413468944765,38.2687586112371));
#57366=CARTESIAN_POINT('Ctrl Pts',(21.376122481006,7.66706968939556,36.2893044282569));
#57367=CARTESIAN_POINT('Ctrl Pts',(19.2301385343949,7.79279248431465,35.9599895187087));
#57368=CARTESIAN_POINT('Ctrl Pts',(17.7857516200634,7.91851527923373,37.5809280895596));
#57369=CARTESIAN_POINT('Ctrl Pts',(18.3592733315035,8.0442380741528,39.6749119135826));
#57370=CARTESIAN_POINT('Ctrl Pts',(20.4280367361936,8.16996086907188,40.3336329350923));
#57371=CARTESIAN_POINT('Ctrl Pts',(22.1067178764283,8.29568366399096,38.956779624756));
#57372=CARTESIAN_POINT('Ctrl Pts',(21.8654860505154,8.42140645891005,36.7991182484206));
#57373=CARTESIAN_POINT('Ctrl Pts',(19.9241828023082,8.54712925382911,35.8269880579295));
#57374=CARTESIAN_POINT('Ctrl Pts',(18.0519739603972,8.6728520487482,36.9263194279151));
#57375=CARTESIAN_POINT('Ctrl Pts',(17.9550576214233,8.79857484366728,39.0952598678542));
#57376=CARTESIAN_POINT('Ctrl Pts',(19.7217564497116,8.92429763858637,40.3571911888414));
#57377=CARTESIAN_POINT('Ctrl Pts',(21.7420266773424,9.05002043350544,39.5620788595995));
#57378=CARTESIAN_POINT('Ctrl Pts',(22.1747375821867,9.17574322842452,37.4345317551639));
#57379=CARTESIAN_POINT('Ctrl Pts',(20.6255471946341,9.30146602334358,35.9134451199328));
#57380=CARTESIAN_POINT('Ctrl Pts',(18.5062775461834,9.42718881826269,36.3850292226326));
#57381=CARTESIAN_POINT('Ctrl Pts',(17.7482803960562,9.55291161318175,38.4195158235133));
#57382=CARTESIAN_POINT('Ctrl Pts',(19.0423404825012,9.67863440810083,40.1628184081019));
#57383=CARTESIAN_POINT('Ctrl Pts',(21.2091434005197,9.80435720301992,40.0262148824157));
#57384=CARTESIAN_POINT('Ctrl Pts',(22.274018946789,9.93007999793899,38.1341959925202));
#57385=CARTESIAN_POINT('Ctrl Pts',(21.2665152200408,10.0558027928581,36.2110133050587));
#57386=CARTESIAN_POINT('Ctrl Pts',(19.1047995221564,10.1815255877772,36.0093188572313));
#57387=CARTESIAN_POINT('Ctrl Pts',(17.758905925534,10.3072483826963,37.7129226360877));
#57388=CARTESIAN_POINT('Ctrl Pts',(18.455386212983,10.4329711776153,39.7692812181347));
#57389=CARTESIAN_POINT('Ctrl Pts',(20.5595177434226,10.5586939725344,40.3043755195192));
#57390=CARTESIAN_POINT('Ctrl Pts',(22.1537445626494,10.6844167674535,38.8305586185368));
#57391=CARTESIAN_POINT('Ctrl Pts',(21.7852016356913,10.8101395623726,36.6909625071754));
#57392=CARTESIAN_POINT('Ctrl Pts',(19.7897527969826,10.9358623572916,35.8354630385256));
#57393=CARTESIAN_POINT('Ctrl Pts',(17.9859083186327,11.0615851522108,37.0437016352813));
#57394=CARTESIAN_POINT('Ctrl Pts',(18.0175638744037,11.1873079471298,39.2145754995472));
#57395=CARTESIAN_POINT('Ctrl Pts',(19.8558708402556,11.3130307420489,40.3697044568779));
#57396=CARTESIAN_POINT('Ctrl Pts',(21.8255268802713,11.438753536968,39.4563860607021));
#57397=CARTESIAN_POINT('Ctrl Pts',(22.1315274461966,11.564476331887,37.3069537955639));
#57398=CARTESIAN_POINT('Ctrl Pts',(20.4950053670916,11.6901991268062,35.8802474861349));
#57399=CARTESIAN_POINT('Ctrl Pts',(18.4073705722187,11.8159219217252,36.476465879008));
#57400=CARTESIAN_POINT('Ctrl Pts',(17.7711450632678,11.9416447166443,38.5522578990629));
#57401=CARTESIAN_POINT('Ctrl Pts',(19.1661395579888,12.0673675115634,40.2158942080144));
#57402=CARTESIAN_POINT('Ctrl Pts',(21.3210552042258,12.1930903064825,39.951254894294));
#57403=CARTESIAN_POINT('Ctrl Pts',(22.272055013431,12.3188131014015,37.9995134227731));
#57404=CARTESIAN_POINT('Ctrl Pts',(21.1524653389212,12.4445358963206,36.1393482770146));
#57405=CARTESIAN_POINT('Ctrl Pts',(18.9826006503776,12.5702586912397,36.0659817848288));
#57406=CARTESIAN_POINT('Ctrl Pts',(17.7399214312059,12.6959814861588,37.8462749536643));
#57407=CARTESIAN_POINT('Ctrl Pts',(18.5569172151707,12.8217042810779,39.8577950996602));
#57408=CARTESIAN_POINT('Ctrl Pts',(20.6890361016724,12.9474270759969,40.2673857032961));
#57409=CARTESIAN_POINT('Ctrl Pts',(22.1932164490149,13.073149870916,38.7017749945208));
#57410=CARTESIAN_POINT('Ctrl Pts',(21.6986551778685,13.1988726658351,36.5877493187435));
#57411=CARTESIAN_POINT('Ctrl Pts',(19.6560602865144,13.3245954607542,35.8518814511358));
#57412=CARTESIAN_POINT('Ctrl Pts',(17.926907609176,13.4503182556732,37.1647890743968));
#57413=CARTESIAN_POINT('Ctrl Pts',(18.0870240198812,13.5760410505923,39.3299814778073));
#57414=CARTESIAN_POINT('Ctrl Pts',(19.9904908000181,13.7017638455114,40.3742561666127));
#57415=CARTESIAN_POINT('Ctrl Pts',(21.9026235892807,13.8274866404305,39.3459353971103));
#57416=CARTESIAN_POINT('Ctrl Pts',(22.0808404424659,13.9532094353496,37.1821576446587));
#57417=CARTESIAN_POINT('Ctrl Pts',(20.3627271839287,14.0789322302686,35.8548361916556));
#57418=CARTESIAN_POINT('Ctrl Pts',(18.3140501458789,14.2046550251877,36.5735974889797));
#57419=CARTESIAN_POINT('Ctrl Pts',(17.8018279988321,14.3303778201068,38.6834135664704));
#57420=CARTESIAN_POINT('Ctrl Pts',(19.2928636083578,14.4561006150259,40.2615479776945));
#57421=CARTESIAN_POINT('Ctrl Pts',(21.4283330750883,14.581823409945,39.8698011647836));
#57422=CARTESIAN_POINT('Ctrl Pts',(22.262121276604,14.707546204864,37.8651833349275));
#57423=CARTESIAN_POINT('Ctrl Pts',(21.0343728962431,14.8332689997831,36.0745607272056));
#57424=CARTESIAN_POINT('Ctrl Pts',(18.863970562285,14.9589917947022,36.1297795420549));
#57425=CARTESIAN_POINT('Ctrl Pts',(17.7288647299603,15.0847145896213,37.9805172755509));
#57426=CARTESIAN_POINT('Ctrl Pts',(18.663510192582,15.2104373845404,39.9401430734941));
#57427=CARTESIAN_POINT('Ctrl Pts',(20.8161374927797,15.3361601794594,40.2227932374915));
#57428=CARTESIAN_POINT('Ctrl Pts',(22.2249950779723,15.4618829743785,38.5708804936067));
#57429=CARTESIAN_POINT('Ctrl Pts',(21.6061502604796,15.5876057692976,36.4898407292998));
#57430=CARTESIAN_POINT('Ctrl Pts',(19.5235742309539,15.7133285642167,35.8761857040551));
#57431=CARTESIAN_POINT('Ctrl Pts',(17.8751787918303,15.8390513591358,37.2891570006639));
#57432=CARTESIAN_POINT('Ctrl Pts',(18.1631944089545,15.9647741540548,39.4410729871876));
#57433=CARTESIAN_POINT('Ctrl Pts',(20.1251441156871,16.0904969489739,40.3708303517809));
#57434=CARTESIAN_POINT('Ctrl Pts',(21.9730463683049,16.216219743893,39.2311143022607));
#57435=CARTESIAN_POINT('Ctrl Pts',(22.0228543683874,16.3419425388121,37.0605810562838));
#57436=CARTESIAN_POINT('Ctrl Pts',(20.2291766440881,16.4676653337312,35.8373003729914));
#57437=CARTESIAN_POINT('Ctrl Pts',(18.2266436119918,16.5933881286502,36.6760833390361));
#57438=CARTESIAN_POINT('Ctrl Pts',(17.8402215746481,16.7191109235693,38.8125227642993));
#57439=CARTESIAN_POINT('Ctrl Pts',(19.4220681171815,16.8448337184884,40.2996195750816));
#57440=CARTESIAN_POINT('Ctrl Pts',(21.5306007090374,16.9705565134075,39.7821394132931));
#57441=CARTESIAN_POINT('Ctrl Pts',(22.2442525813841,17.0962793083265,37.7316769254967));
#57442=CARTESIAN_POINT('Ctrl Pts',(20.9126521309017,17.2220021032456,36.0168779142305));
#57443=CARTESIAN_POINT('Ctrl Pts',(18.7493253827009,17.3477248981647,36.2004883422566));
#57444=CARTESIAN_POINT('Ctrl Pts',(17.7257746059519,17.4734476930838,38.1151787130956));
#57445=CARTESIAN_POINT('Ctrl Pts',(18.7747912435853,17.5991704880029,40.0160362834403));
#57446=CARTESIAN_POINT('Ctrl Pts',(20.9403760766967,17.7248932829219,40.1707545413767));
#57447=CARTESIAN_POINT('Ctrl Pts',(22.2489689780076,17.850616077841,38.4383342611231));
#57448=CARTESIAN_POINT('Ctrl Pts',(21.5080113677371,17.9763388727601,36.3975801778086));
#57449=CARTESIAN_POINT('Ctrl Pts',(19.3927593584336,18.1020616676792,35.9082905440105));
#57450=CARTESIAN_POINT('Ctrl Pts',(17.8309033183622,18.2277844625983,37.416369162359));
#57451=CARTESIAN_POINT('Ctrl Pts',(18.2458078549532,18.3535072575174,39.5474603463113));
#57452=CARTESIAN_POINT('Ctrl Pts',(20.2593584567611,18.4792300524364,40.3594390293124));
#57453=CARTESIAN_POINT('Ctrl Pts',(22.0365481921237,18.6049528473555,39.1123255399277));
#57454=CARTESIAN_POINT('Ctrl Pts',(21.9577726239778,18.7306756422746,36.9426504909417));
#57455=CARTESIAN_POINT('Ctrl Pts',(20.0948222109758,18.8563984371937,35.8277015412522));
#57456=CARTESIAN_POINT('Ctrl Pts',(18.1454575682997,18.9821212321127,36.7835639346676));
#57457=CARTESIAN_POINT('Ctrl Pts',(17.8861911206918,19.1078440270318,38.9391326089534));
#57458=CARTESIAN_POINT('Ctrl Pts',(19.5532998573488,19.2335668219509,40.329975455778));
#57459=CARTESIAN_POINT('Ctrl Pts',(21.6274993957651,19.35928961687,39.6885771329276));
#57460=CARTESIAN_POINT('Ctrl Pts',(22.2185115696939,19.4850124117891,37.5994625065813));
#57461=CARTESIAN_POINT('Ctrl Pts',(20.787730080782,19.6107352067082,35.9665021656478));
#57462=CARTESIAN_POINT('Ctrl Pts',(18.6390671193433,19.7364580016272,36.2778601747661));
#57463=CARTESIAN_POINT('Ctrl Pts',(17.7306621680414,19.8621807965463,38.2497868722107));
#57464=CARTESIAN_POINT('Ctrl Pts',(18.8903694996679,19.9879035914654,40.0852085833905));
#57465=CARTESIAN_POINT('Ctrl Pts',(21.0613170676605,20.1136263863845,40.1114520212098));
#57466=CARTESIAN_POINT('Ctrl Pts',(22.2650520927181,20.2393491813036,38.3046014931365));
#57467=CARTESIAN_POINT('Ctrl Pts',(21.4045865489703,20.3650719762226,36.3112907934586));
#57468=CARTESIAN_POINT('Ctrl Pts',(19.2640671650938,20.4907947711417,35.948084320147));
#57469=CARTESIAN_POINT('Ctrl Pts',(17.7942507800659,20.6165175660608,37.5459774606941));
#57470=CARTESIAN_POINT('Ctrl Pts',(18.334546885942,20.7422403609799,39.648773999513));
#57471=CARTESIAN_POINT('Ctrl Pts',(20.3927166898407,20.867963155899,40.3401151319165));
#57472=CARTESIAN_POINT('Ctrl Pts',(22.0928023143269,20.993685950818,38.9899994071434));
#57473=CARTESIAN_POINT('Ctrl Pts',(21.8860250841065,21.1194087457371,36.8287532338137));
#57474=CARTESIAN_POINT('Ctrl Pts',(19.9597442617979,21.2451315406562,35.8261244740626));
#57475=CARTESIAN_POINT('Ctrl Pts',(18.071536445263,21.3708543355753,36.895563530529));
#57476=CARTESIAN_POINT('Ctrl Pts',(17.9380830578744,21.4965771304943,39.0629871265469));
#57477=CARTESIAN_POINT('Ctrl Pts',(19.6894213454275,21.622316577962,40.3523470934528));
#57478=CARTESIAN_POINT('Ctrl Pts',(21.0374380936755,21.7061484271234,39.8437203447635));
#57479=CARTESIAN_POINT('Ctrl Pts',(21.4557699665296,21.7480726779785,39.3605849726844));
#57480=CARTESIAN_POINT('Ctrl Pts',(19.0436064803604,-0.0429106862021636,
36.2612099984105));
#57481=CARTESIAN_POINT('Ctrl Pts',(18.4336188389561,-0.00100308789580381,
36.5784774551593));
#57482=CARTESIAN_POINT('Ctrl Pts',(17.5645803039565,0.0828121087169158,
37.8622621797055));
#57483=CARTESIAN_POINT('Ctrl Pts',(18.4763481082636,0.208534903635996,40.017757261042));
#57484=CARTESIAN_POINT('Ctrl Pts',(20.7786990981206,0.334257698555075,40.4199720538028));
#57485=CARTESIAN_POINT('Ctrl Pts',(22.3703584524549,0.459980493474155,38.7106796933293));
#57486=CARTESIAN_POINT('Ctrl Pts',(21.8023775158073,0.585703288393234,36.4434506819814));
#57487=CARTESIAN_POINT('Ctrl Pts',(19.5915613544439,0.711426083312313,35.6866074645181));
#57488=CARTESIAN_POINT('Ctrl Pts',(17.753109769432,0.837148878231393,37.1287850425919));
#57489=CARTESIAN_POINT('Ctrl Pts',(17.9622406892819,0.962871673150472,39.4562516967922));
#57490=CARTESIAN_POINT('Ctrl Pts',(20.0284786047021,1.08859446806955,40.5476274673468));
#57491=CARTESIAN_POINT('Ctrl Pts',(22.0687435548436,1.21431726298863,39.4084608151208));
#57492=CARTESIAN_POINT('Ctrl Pts',(22.2237127438928,1.34004005790771,37.0768294788493));
#57493=CARTESIAN_POINT('Ctrl Pts',(20.3521429437231,1.46576285282679,35.6776567091597));
#57494=CARTESIAN_POINT('Ctrl Pts',(18.1596577789763,1.59148564774587,36.4860284307524));
#57495=CARTESIAN_POINT('Ctrl Pts',(17.6443283488832,1.71720844266495,38.7652627862372));
#57496=CARTESIAN_POINT('Ctrl Pts',(19.2757913804202,1.84293123758403,40.4382220364387));
#57497=CARTESIAN_POINT('Ctrl Pts',(21.5672463149755,1.96865403250311,39.9802928482416));
#57498=CARTESIAN_POINT('Ctrl Pts',(22.4304245195311,2.09437682742219,37.8087978749678));
#57499=CARTESIAN_POINT('Ctrl Pts',(21.0786864281009,2.22009962234127,35.9026840829364));
#57500=CARTESIAN_POINT('Ctrl Pts',(18.7439102298808,2.34582241726035,35.9990477402805));
#57501=CARTESIAN_POINT('Ctrl Pts',(17.5538449623967,2.47154521217943,38.0100700590282));
#57502=CARTESIAN_POINT('Ctrl Pts',(18.5930315823703,2.59726800709851,40.1030481000252));
#57503=CARTESIAN_POINT('Ctrl Pts',(20.9144292299826,2.72299080201759,40.3705904604286));
#57504=CARTESIAN_POINT('Ctrl Pts',(22.4024810616538,2.84871359693667,38.5688780172262));
#57505=CARTESIAN_POINT('Ctrl Pts',(21.7010823756679,2.97443639185575,36.3398634731384));
#57506=CARTESIAN_POINT('Ctrl Pts',(19.4494380948377,3.10015918677483,35.714912279268));
#57507=CARTESIAN_POINT('Ctrl Pts',(17.6995368101505,3.22588198169391,37.2635605475731));
#57508=CARTESIAN_POINT('Ctrl Pts',(18.0461142026948,3.35160477661299,39.574480293551));
#57509=CARTESIAN_POINT('Ctrl Pts',(20.1733242648118,3.47732757153206,40.5416634790403));
#57510=CARTESIAN_POINT('Ctrl Pts',(22.1425789087208,3.60305036645114,39.283688077704));
#57511=CARTESIAN_POINT('Ctrl Pts',(22.1592393899528,3.72877316137022,36.9469834770324));
#57512=CARTESIAN_POINT('Ctrl Pts',(20.2081225298838,3.85449595628931,35.661056200319));
#57513=CARTESIAN_POINT('Ctrl Pts',(18.0673375855584,3.98021875120838,36.5978089877741));
#57514=CARTESIAN_POINT('Ctrl Pts',(17.6878438279644,4.10594154612746,38.9035519158862));
#57515=CARTESIAN_POINT('Ctrl Pts',(19.4154849003888,4.23166434104654,40.4769947294314));
#57516=CARTESIAN_POINT('Ctrl Pts',(21.6758114981089,4.35738713596562,39.8842134592636));
#57517=CARTESIAN_POINT('Ctrl Pts',(22.4089225820486,4.4831099308847,37.6654268311222));
#57518=CARTESIAN_POINT('Ctrl Pts',(20.9467128062435,4.60883272580378,35.842679307695));
#57519=CARTESIAN_POINT('Ctrl Pts',(18.6217362536136,4.73455552072286,36.0770934547515));
#57520=CARTESIAN_POINT('Ctrl Pts',(17.5528113380187,4.86027831564194,38.1550408764728));
#57521=CARTESIAN_POINT('Ctrl Pts',(18.7140802681763,4.98600111056102,40.1828279546616));
#57522=CARTESIAN_POINT('Ctrl Pts',(21.0472450625962,5.1117239054801,40.3124736437482));
#57523=CARTESIAN_POINT('Ctrl Pts',(22.4260251257194,5.23744670039918,38.4258280755102));
#57524=CARTESIAN_POINT('Ctrl Pts',(21.5938982861276,5.36316949531825,36.2422459530679));
#57525=CARTESIAN_POINT('Ctrl Pts',(19.3092058132839,5.48889229023733,35.7516888543014));
#57526=CARTESIAN_POINT('Ctrl Pts',(17.6540540733761,5.61461508515642,37.4012156593273));
#57527=CARTESIAN_POINT('Ctrl Pts',(18.1368307446719,5.74033788007549,39.6875648558131));
#57528=CARTESIAN_POINT('Ctrl Pts',(20.317567475763,5.86606067499458,40.527120257373));
#57529=CARTESIAN_POINT('Ctrl Pts',(22.2088957762494,5.99178346991365,39.1547707310503));
#57530=CARTESIAN_POINT('Ctrl Pts',(22.087193433601,6.11750626483274,36.821178113987));
#57531=CARTESIAN_POINT('Ctrl Pts',(20.0633713145625,6.24322905975181,35.6530128888971));
#57532=CARTESIAN_POINT('Ctrl Pts',(17.9817970826894,6.36895185467089,36.7148578304118));
#57533=CARTESIAN_POINT('Ctrl Pts',(17.7394695732254,6.49467464958997,39.0390229150768));
#57534=CARTESIAN_POINT('Ctrl Pts',(19.5572288581518,6.62039744450905,40.5074292432716));
#57535=CARTESIAN_POINT('Ctrl Pts',(21.7784982977988,6.74612023942813,39.7818756345639));
#57536=CARTESIAN_POINT('Ctrl Pts',(22.3789707715017,6.87184303434721,37.5235800890376));
#57537=CARTESIAN_POINT('Ctrl Pts',(20.8114183371727,6.99756582926629,35.7905926891272));
#57538=CARTESIAN_POINT('Ctrl Pts',(18.504396890909,7.12328862418536,36.1622350025119));
#57539=CARTESIAN_POINT('Ctrl Pts',(17.5603618385438,7.24901141910446,38.2998186342149));
#57540=CARTESIAN_POINT('Ctrl Pts',(18.8396396423022,7.37473421402352,40.2553017620966));
#57541=CARTESIAN_POINT('Ctrl Pts',(21.1763874191757,7.50045700894261,40.2465960228738));
#57542=CARTESIAN_POINT('Ctrl Pts',(22.4410592980093,7.62617980386168,38.2816352086321));
#57543=CARTESIAN_POINT('Ctrl Pts',(21.481123197853,7.75190259878077,36.1511449725044));
#57544=CARTESIAN_POINT('Ctrl Pts',(19.1713966659368,7.87762539369984,35.7967027199703));
#57545=CARTESIAN_POINT('Ctrl Pts',(17.6168003309307,8.00334818861892,37.5413219328085));
#57546=CARTESIAN_POINT('Ctrl Pts',(18.2340828206879,8.129070983538,39.795080635611));
#57547=CARTESIAN_POINT('Ctrl Pts',(20.4606967390331,8.25479377845708,40.504063302007));
#57548=CARTESIAN_POINT('Ctrl Pts',(22.2674643872022,8.38051657337616,39.0221535111804));
#57549=CARTESIAN_POINT('Ctrl Pts',(22.0078261221847,8.50623936829525,36.6998585398304));
#57550=CARTESIAN_POINT('Ctrl Pts',(19.9183978084455,8.63196216321431,35.6535529991953));
#57551=CARTESIAN_POINT('Ctrl Pts',(17.903335933319,8.75768495813341,36.8367654070199));
#57552=CARTESIAN_POINT('Ctrl Pts',(17.7990246965748,8.88340775305248,39.1712000556036));
#57553=CARTESIAN_POINT('Ctrl Pts',(19.7005259468737,9.00913054797156,40.5294190945403));
#57554=CARTESIAN_POINT('Ctrl Pts',(21.8749465681312,9.13485334289064,39.673638208759));
#57555=CARTESIAN_POINT('Ctrl Pts',(22.3406741236175,9.26057613780971,37.383755284529));
#57556=CARTESIAN_POINT('Ctrl Pts',(20.6732776145384,9.3862989327288,35.7466068965907));
#57557=CARTESIAN_POINT('Ctrl Pts',(18.3923037316531,9.51202172764788,36.2541737475709));
#57558=CARTESIAN_POINT('Ctrl Pts',(17.5764699825097,9.63774452256696,38.4438954779233));
#57559=CARTESIAN_POINT('Ctrl Pts',(18.9692692717474,9.76346731748603,40.3202153074079));
#57560=CARTESIAN_POINT('Ctrl Pts',(21.3014033014935,9.88919011240512,40.1731886774423));
#57561=CARTESIAN_POINT('Ctrl Pts',(22.4475308418653,10.0149129073242,38.1368052106512));
#57562=CARTESIAN_POINT('Ctrl Pts',(21.363152698054,10.1406357022433,36.0668800903044));
#57563=CARTESIAN_POINT('Ctrl Pts',(19.036494052845,10.2663584971624,35.8497959792033));
#57564=CARTESIAN_POINT('Ctrl Pts',(17.5879062597423,10.3920812920814,37.6833879098936));
#57565=CARTESIAN_POINT('Ctrl Pts',(18.3375292946295,10.5178040870005,39.8966504944474));
#57566=CARTESIAN_POINT('Ctrl Pts',(20.6022099928108,10.6435268819196,40.4725734909528));
#57567=CARTESIAN_POINT('Ctrl Pts',(22.3180792974602,10.7692496768387,38.8863016063186));
#57568=CARTESIAN_POINT('Ctrl Pts',(21.9214158564827,10.8949724717578,36.5834503134188));
#57569=CARTESIAN_POINT('Ctrl Pts',(19.7737105425055,11.0206952666768,35.6626746366478));
#57570=CARTESIAN_POINT('Ctrl Pts',(17.8322293596317,11.1464180615959,36.9631040961593));
#57571=CARTESIAN_POINT('Ctrl Pts',(17.8663002934623,11.272140856515,39.2996196929586));
#57572=CARTESIAN_POINT('Ctrl Pts',(19.8448735160344,11.3978636514341,40.5428871483115));
#57573=CARTESIAN_POINT('Ctrl Pts',(21.9648179925797,11.5235864463532,39.5598808517986));
#57574=CARTESIAN_POINT('Ctrl Pts',(22.2941669735052,11.6493092412722,37.246442888208));
#57575=CARTESIAN_POINT('Ctrl Pts',(20.532775201612,11.7750320361913,35.7108762212978));
#57576=CARTESIAN_POINT('Ctrl Pts',(18.2858499707485,11.9007548311104,36.3525871916946));
#57577=CARTESIAN_POINT('Ctrl Pts',(17.6010792665565,12.0264776260295,38.5867660218912));
#57578=CARTESIAN_POINT('Ctrl Pts',(19.1025144480368,12.1522004209485,40.377340890036));
#57579=CARTESIAN_POINT('Ctrl Pts',(21.4218541849508,12.2779232158676,40.09250910215));
#57580=CARTESIAN_POINT('Ctrl Pts',(22.4454170567221,12.4036460107867,37.9918461091523));
#57581=CARTESIAN_POINT('Ctrl Pts',(21.2404005978811,12.5293688057058,35.9897468867008));
#57582=CARTESIAN_POINT('Ctrl Pts',(18.9049711787976,12.6550916006249,35.910782394062));
#57583=CARTESIAN_POINT('Ctrl Pts',(17.567473213021,12.780814395544,37.8269152584955));
#57584=CARTESIAN_POINT('Ctrl Pts',(18.4468073020141,12.906537190463,39.9919181505383));
#57585=CARTESIAN_POINT('Ctrl Pts',(20.7416108438247,13.0322599853821,40.4327612826292));
#57586=CARTESIAN_POINT('Ctrl Pts',(22.3605629625162,13.1579827803012,38.7476915511336));
#57587=CARTESIAN_POINT('Ctrl Pts',(21.8282657421995,13.2837055752202,36.472361765836));
#57588=CARTESIAN_POINT('Ctrl Pts',(19.6298170436588,13.4094283701394,35.680345804821));
#57589=CARTESIAN_POINT('Ctrl Pts',(17.7687267857893,13.5351511650584,37.0934307331541));
#57590=CARTESIAN_POINT('Ctrl Pts',(17.9410603778394,13.6608739599775,39.423831363018));
#57591=CARTESIAN_POINT('Ctrl Pts',(19.9897652302897,13.7865967548966,40.5477861620047));
#57592=CARTESIAN_POINT('Ctrl Pts',(22.0477973245563,13.9123195498157,39.4410025961767));
#57593=CARTESIAN_POINT('Ctrl Pts',(22.2396124566716,14.0380423447347,37.1121245577836));
#57594=CARTESIAN_POINT('Ctrl Pts',(20.3904039458871,14.1637651396538,35.683525997564));
#57595=CARTESIAN_POINT('Ctrl Pts',(18.1854090214921,14.2894879345729,36.457130125016));
#57596=CARTESIAN_POINT('Ctrl Pts',(17.6341033674412,14.415210729492,38.7279291118112));
#57597=CARTESIAN_POINT('Ctrl Pts',(19.238907780257,14.5409335244111,40.4264781276555));
#57598=CARTESIAN_POINT('Ctrl Pts',(21.5373175578291,14.6666563193301,40.004840300866));
#57599=CARTESIAN_POINT('Ctrl Pts',(22.434725357212,14.7923791142492,37.8472663845829));
#57600=CARTESIAN_POINT('Ctrl Pts',(21.1132974811485,14.9181019091683,35.9200159257734));
#57601=CARTESIAN_POINT('Ctrl Pts',(18.7772893933007,15.0438247040874,35.9794480393827));
#57602=CARTESIAN_POINT('Ctrl Pts',(17.5555728648087,15.1695474990065,37.9714005203993));
#57603=CARTESIAN_POINT('Ctrl Pts',(18.5615335227911,15.2952702939255,40.0805494286584));
#57604=CARTESIAN_POINT('Ctrl Pts',(20.8784103085867,15.4209930888446,40.3847663283543));
#57605=CARTESIAN_POINT('Ctrl Pts',(22.3947663602474,15.5467158837637,38.6068095551986));
#57606=CARTESIAN_POINT('Ctrl Pts',(21.7287025267509,15.6724386786828,36.3669825680571));
#57607=CARTESIAN_POINT('Ctrl Pts',(19.4872220544836,15.7981614736018,35.7065045176552));
#57608=CARTESIAN_POINT('Ctrl Pts',(17.7130509630151,15.9238842685209,37.2272881646004));
#57609=CARTESIAN_POINT('Ctrl Pts',(18.0230427099378,16.04960706344,39.5433993621595));
#57610=CARTESIAN_POINT('Ctrl Pts',(20.1346928455696,16.1753298583591,40.5440989510993));
#57611=CARTESIAN_POINT('Ctrl Pts',(22.1235934932184,16.3010526532782,39.3174204372251));
#57612=CARTESIAN_POINT('Ctrl Pts',(22.1772019367829,16.4267754481972,36.9812714485266));
#57613=CARTESIAN_POINT('Ctrl Pts',(20.2466632502921,16.5524982431163,35.6646521631667));
#57614=CARTESIAN_POINT('Ctrl Pts',(18.0913332057336,16.6782210380354,36.5674358369459));
#57615=CARTESIAN_POINT('Ctrl Pts',(17.6754264448377,16.8039438329545,38.8668895826994));
#57616=CARTESIAN_POINT('Ctrl Pts',(19.377970834547,16.9296666278735,40.4674546590671));
#57617=CARTESIAN_POINT('Ctrl Pts',(21.647388403355,17.0553894227927,39.9104897939243));
#57618=CARTESIAN_POINT('Ctrl Pts',(22.4154932471558,17.1811122177117,37.7035731866305));
#57619=CARTESIAN_POINT('Ctrl Pts',(20.9822891939532,17.3068350126308,35.8579318063771));
#57620=CARTESIAN_POINT('Ctrl Pts',(18.653896572278,17.4325578075499,36.0555520531726));
#57621=CARTESIAN_POINT('Ctrl Pts',(17.552246958564,17.558280602469,38.1163368772691));
#57622=CARTESIAN_POINT('Ctrl Pts',(18.6813055259356,17.684003397388,40.1622334323443));
#57623=CARTESIAN_POINT('Ctrl Pts',(21.0121285286199,17.8097261923071,40.3287569824818));
#57624=CARTESIAN_POINT('Ctrl Pts',(22.4205695136552,17.9354489872262,38.4641497974886));
#57625=CARTESIAN_POINT('Ctrl Pts',(21.623075453101,18.0611717821453,36.2676823640807));
#57626=CARTESIAN_POINT('Ctrl Pts',(19.3464257627376,18.1868945770644,35.7410590168932));
#57627=CARTESIAN_POINT('Ctrl Pts',(17.6653971881842,18.3126173719835,37.364206851953));
#57628=CARTESIAN_POINT('Ctrl Pts',(18.1119597162451,18.4383401669025,39.6579042755893));
#57629=CARTESIAN_POINT('Ctrl Pts',(20.2791479916725,18.5640629618216,40.5318384494398));
#57630=CARTESIAN_POINT('Ctrl Pts',(22.1919406248596,18.6897857567407,39.1895678703468));
#57631=CARTESIAN_POINT('Ctrl Pts',(22.1071543336573,18.8155085516598,36.8543425606733));
#57632=CARTESIAN_POINT('Ctrl Pts',(20.1020573228665,18.9412313465789,35.6543209226286));
#57633=CARTESIAN_POINT('Ctrl Pts',(18.0039525151963,19.0669541414979,36.6831174028719));
#57634=CARTESIAN_POINT('Ctrl Pts',(17.7249035531474,19.192676936417,39.0031599950952));
#57635=CARTESIAN_POINT('Ctrl Pts',(19.5192158017205,19.3183997313361,40.5001267501863));
#57636=CARTESIAN_POINT('Ctrl Pts',(21.7516806409536,19.4441225262551,39.809788536728));
#57637=CARTESIAN_POINT('Ctrl Pts',(22.3877881481717,19.5698453211742,37.561270560484));
#57638=CARTESIAN_POINT('Ctrl Pts',(20.8478353579689,19.6955681160933,35.8037122940409));
#57639=CARTESIAN_POINT('Ctrl Pts',(18.5352253973877,19.8212909110124,36.1388275010866));
#57640=CARTESIAN_POINT('Ctrl Pts',(17.5575074507744,19.9470137059315,38.2612158904656));
#57641=CARTESIAN_POINT('Ctrl Pts',(18.8057026189372,20.0727365008505,40.2366837080424));
#57642=CARTESIAN_POINT('Ctrl Pts',(21.1422975431955,20.1984592957697,40.2649295692081));
#57643=CARTESIAN_POINT('Ctrl Pts',(22.4378798000725,20.3241820906887,38.3202129693996));
#57644=CARTESIAN_POINT('Ctrl Pts',(21.5117591273934,20.4499048856078,36.1748089384568));
#57645=CARTESIAN_POINT('Ctrl Pts',(19.2079141145602,20.5756276805269,35.7838891325111));
#57646=CARTESIAN_POINT('Ctrl Pts',(17.6259479927237,20.701350475446,37.5037045056489));
#57647=CARTESIAN_POINT('Ctrl Pts',(18.207469701124,20.827073270365,39.766948349854));
#57648=CARTESIAN_POINT('Ctrl Pts',(20.4226817071412,20.9527960652841,40.5110401025622));
#57649=CARTESIAN_POINT('Ctrl Pts',(22.2524870417086,21.0785188602032,39.0579080250413));
#57650=CARTESIAN_POINT('Ctrl Pts',(22.0299323224199,21.2042416551223,36.7317547299878));
#57651=CARTESIAN_POINT('Ctrl Pts',(19.9566726737475,21.3299644500414,35.6526235222652));
#57652=CARTESIAN_POINT('Ctrl Pts',(17.9243910723363,21.4556872449604,36.8036627771902));
#57653=CARTESIAN_POINT('Ctrl Pts',(17.780754942107,21.5814100398795,39.1364648438266));
#57654=CARTESIAN_POINT('Ctrl Pts',(19.6657236137085,21.7071494873473,40.5242053856216));
#57655=CARTESIAN_POINT('Ctrl Pts',(21.1165965588731,21.7909813365086,39.9767694655415));
#57656=CARTESIAN_POINT('Ctrl Pts',(21.5668479353584,21.8329055873637,39.4567699617426));
#57657=CARTESIAN_POINT('Ctrl Pts',(18.9758052297315,0.0419222231830331,
36.1308533416667));
#57658=CARTESIAN_POINT('Ctrl Pts',(18.3225739609854,0.083829821489393,36.4706127224088));
#57659=CARTESIAN_POINT('Ctrl Pts',(17.3919269998435,0.167645018102112,37.8454083206958));
#57660=CARTESIAN_POINT('Ctrl Pts',(18.3683324205143,0.293367813021192,40.1537121143855));
#57661=CARTESIAN_POINT('Ctrl Pts',(20.833903124112,0.419090607940272,40.5844409710861));
#57662=CARTESIAN_POINT('Ctrl Pts',(22.5383993939867,0.544813402859351,38.7539723820513));
#57663=CARTESIAN_POINT('Ctrl Pts',(21.9301527957185,0.67053619777843,36.3260135463425));
#57664=CARTESIAN_POINT('Ctrl Pts',(19.5626060652191,0.79625899269751,35.515515723719));
#57665=CARTESIAN_POINT('Ctrl Pts',(17.5938218147042,0.921981787616588,37.0599330612793));
#57666=CARTESIAN_POINT('Ctrl Pts',(17.8177785751937,1.04770458253567,39.5523999446856));
#57667=CARTESIAN_POINT('Ctrl Pts',(20.0304975278497,1.17342737745475,40.7211462124573));
#57668=CARTESIAN_POINT('Ctrl Pts',(22.2154022234444,1.29915017237383,39.5012210417873));
#57669=CARTESIAN_POINT('Ctrl Pts',(22.3813575856649,1.42487296729291,37.0042942310502));
#57670=CARTESIAN_POINT('Ctrl Pts',(20.3771072826633,1.55059576221199,35.5059304257848));
#57671=CARTESIAN_POINT('Ctrl Pts',(18.0291910813165,1.67631855713107,36.3716097436458));
#57672=CARTESIAN_POINT('Ctrl Pts',(17.4773285933046,1.80204135205015,38.8124250138951));
#57673=CARTESIAN_POINT('Ctrl Pts',(19.2244503276889,1.92776414696923,40.603984742964));
#57674=CARTESIAN_POINT('Ctrl Pts',(21.6783525259826,2.05348694188831,40.1135917508809));
#57675=CARTESIAN_POINT('Ctrl Pts',(22.6027237024506,2.17920973680738,37.7881537908565));
#57676=CARTESIAN_POINT('Ctrl Pts',(21.1551573444755,2.30493253172647,35.7469105816062));
#57677=CARTESIAN_POINT('Ctrl Pts',(18.6548627242596,2.43065532664554,35.8501057119256));
#57678=CARTESIAN_POINT('Ctrl Pts',(17.3804306017012,2.55637812156462,38.0036946891185));
#57679=CARTESIAN_POINT('Ctrl Pts',(18.4932878928202,2.6821009164837,40.2450494451438));
#57680=CARTESIAN_POINT('Ctrl Pts',(20.9792555218084,2.80782371140278,40.5315585867508));
#57681=CARTESIAN_POINT('Ctrl Pts',(22.5727992593908,2.93354650632186,38.6021180123824));
#57682=CARTESIAN_POINT('Ctrl Pts',(21.8216765768254,3.05926930124094,36.2150827679703));
#57683=CARTESIAN_POINT('Ctrl Pts',(19.4104073141475,3.18499209616002,35.54582714119));
#57684=CARTESIAN_POINT('Ctrl Pts',(17.5364509275148,3.3107148910791,37.2042631560859));
#57685=CARTESIAN_POINT('Ctrl Pts',(17.9075981024465,3.43643768599817,39.6790100774501));
#57686=CARTESIAN_POINT('Ctrl Pts',(20.1856116775528,3.56216048091726,40.7147594213426));
#57687=CARTESIAN_POINT('Ctrl Pts',(22.2944719596453,3.68788327583633,39.3676028370313));
#57688=CARTESIAN_POINT('Ctrl Pts',(22.3123135461862,3.81360607075542,36.865243104845));
#57689=CARTESIAN_POINT('Ctrl Pts',(20.2228768831082,3.9393288656745,35.4881530632354));
#57690=CARTESIAN_POINT('Ctrl Pts',(17.93032606671,4.06505166059357,36.4913147181865));
#57691=CARTESIAN_POINT('Ctrl Pts',(17.5239289990847,4.19077445551266,38.9605178234583));
#57692=CARTESIAN_POINT('Ctrl Pts',(19.374047088493,4.31649725043174,40.6455061340825));
#57693=CARTESIAN_POINT('Ctrl Pts',(21.7946141803279,4.44222004535081,40.0107010414595));
#57694=CARTESIAN_POINT('Ctrl Pts',(22.5796974360989,4.56794284026989,37.6346187968407));
#57695=CARTESIAN_POINT('Ctrl Pts',(21.0138277656526,4.69366563518897,35.6826519101167));
#57696=CARTESIAN_POINT('Ctrl Pts',(18.5240275136623,4.81938843010805,35.93368429225));
#57697=CARTESIAN_POINT('Ctrl Pts',(17.3793237009739,4.94511122502714,38.158942868889));
#57698=CARTESIAN_POINT('Ctrl Pts',(18.6229180381575,5.0708340199462,40.3304851033885));
#57699=CARTESIAN_POINT('Ctrl Pts',(21.121487017922,5.1965568148653,40.4693217161674));
#57700=CARTESIAN_POINT('Ctrl Pts',(22.5980124240472,5.32227960978436,38.4489268842704));
#57701=CARTESIAN_POINT('Ctrl Pts',(21.7068939254283,5.44800240470346,36.1105448853));
#57702=CARTESIAN_POINT('Ctrl Pts',(19.260233597533,5.57372519962252,35.5852109043001));
#57703=CARTESIAN_POINT('Ctrl Pts',(17.4877437999723,5.69944799454161,37.3516770005591));
#57704=CARTESIAN_POINT('Ctrl Pts',(18.004745778546,5.82517078946069,39.8001115015904));
#57705=CARTESIAN_POINT('Ctrl Pts',(20.3400806688929,5.95089358437976,40.6991851924624));
#57706=CARTESIAN_POINT('Ctrl Pts',(22.3654902042366,6.07661637929885,39.2295462007951));
#57707=CARTESIAN_POINT('Ctrl Pts',(22.2351600626052,6.20233917421792,36.7305190689153));
#57708=CARTESIAN_POINT('Ctrl Pts',(20.0678638736327,6.32806196913701,35.479539540324));
#57709=CARTESIAN_POINT('Ctrl Pts',(17.8387213727366,6.45378476405608,36.6166614609588));
#57710=CARTESIAN_POINT('Ctrl Pts',(17.5792146291333,6.57950755897517,39.1055927178871));
#57711=CARTESIAN_POINT('Ctrl Pts',(19.5258396480168,6.70523035389424,40.6780982306105));
#57712=CARTESIAN_POINT('Ctrl Pts',(21.9045807171753,6.83095314881333,39.9011082193567));
#57713=CARTESIAN_POINT('Ctrl Pts',(22.5476222629695,6.95667594373239,37.4827161663445));
#57714=CARTESIAN_POINT('Ctrl Pts',(20.8689419160278,7.08239873865149,35.6268727342411));
#57715=CARTESIAN_POINT('Ctrl Pts',(18.3983696550917,7.20812153357055,36.0248617481384));
#57716=CARTESIAN_POINT('Ctrl Pts',(17.3874094763289,7.33384432848965,38.3139843024473));
#57717=CARTESIAN_POINT('Ctrl Pts',(18.7573786463665,7.45956712340871,40.4080967695405));
#57718=CARTESIAN_POINT('Ctrl Pts',(21.2597846156292,7.58528991832781,40.3987738575802));
#57719=CARTESIAN_POINT('Ctrl Pts',(22.6141124083302,7.71101271324687,38.2945118060269));
#57720=CARTESIAN_POINT('Ctrl Pts',(21.5861239146998,7.83673550816597,36.0129855167519));
#57721=CARTESIAN_POINT('Ctrl Pts',(19.1126547974788,7.96245830308503,35.6334159212318));
#57722=CARTESIAN_POINT('Ctrl Pts',(17.447849041798,8.08818109800412,37.5017157760575));
#57723=CARTESIAN_POINT('Ctrl Pts',(18.1088923098723,8.21390389292319,39.9152493576393));
#57724=CARTESIAN_POINT('Ctrl Pts',(20.4933567418726,8.33962668784228,40.6744936689219));
#57725=CARTESIAN_POINT('Ctrl Pts',(22.4282108979761,8.46534948276135,39.0875273976046));
#57726=CARTESIAN_POINT('Ctrl Pts',(22.1501661938539,8.59107227768044,36.6005988312404));
#57727=CARTESIAN_POINT('Ctrl Pts',(19.9126128145828,8.71679507259951,35.4801179404609));
#57728=CARTESIAN_POINT('Ctrl Pts',(17.7546979062407,8.8425178675186,36.7472113861249));
#57729=CARTESIAN_POINT('Ctrl Pts',(17.6429917717263,8.96824066243768,39.2471402433529));
#57730=CARTESIAN_POINT('Ctrl Pts',(19.6792954440358,9.09396345735676,40.7016470002393));
#57731=CARTESIAN_POINT('Ctrl Pts',(22.00786645892,9.21968625227583,39.7851975579183));
#57732=CARTESIAN_POINT('Ctrl Pts',(22.5066106650485,9.34540904719491,37.3329788138943));
#57733=CARTESIAN_POINT('Ctrl Pts',(20.7210080344426,9.47113184211399,35.5797686732486));
#57734=CARTESIAN_POINT('Ctrl Pts',(18.2783299171228,9.59685463703307,36.1233182725093));
#57735=CARTESIAN_POINT('Ctrl Pts',(17.4046595689631,9.72257743195216,38.4682751323334));
#57736=CARTESIAN_POINT('Ctrl Pts',(18.8961980609935,9.84830022687122,40.477612206714));
#57737=CARTESIAN_POINT('Ctrl Pts',(21.3936632024671,9.97402302179031,40.3201624724688));
#57738=CARTESIAN_POINT('Ctrl Pts',(22.6210427369415,10.0997458167094,38.1394144287822));
#57739=CARTESIAN_POINT('Ctrl Pts',(21.4597901760673,10.2254686116285,35.92274687555));
#57740=CARTESIAN_POINT('Ctrl Pts',(18.9681885835334,10.3511914065475,35.6902731011753));
#57741=CARTESIAN_POINT('Ctrl Pts',(17.4169065939508,10.4769142014666,37.6538531836996));
#57742=CARTESIAN_POINT('Ctrl Pts',(18.219672376276,10.6026369963857,40.0240197707599));
#57743=CARTESIAN_POINT('Ctrl Pts',(20.6449022421991,10.7283597913048,40.6407714623863));
#57744=CARTESIAN_POINT('Ctrl Pts',(22.4824140322711,10.8540825862239,38.9420445941005));
#57745=CARTESIAN_POINT('Ctrl Pts',(22.0576300772742,10.9798053811429,36.4759381196621));
#57746=CARTESIAN_POINT('Ctrl Pts',(19.7576682880285,11.105528176062,35.48988623477));
#57747=CARTESIAN_POINT('Ctrl Pts',(17.6785504006306,11.2312509709811,36.8825065570371));
#57748=CARTESIAN_POINT('Ctrl Pts',(17.715036712521,11.3569737659002,39.38466388637));
#57749=CARTESIAN_POINT('Ctrl Pts',(19.8338761918132,11.4826965608193,40.716069839745));
#57750=CARTESIAN_POINT('Ctrl Pts',(22.104109104888,11.6084193557383,39.6633756428951));
#57751=CARTESIAN_POINT('Ctrl Pts',(22.4568065008138,11.7341421506574,37.1859319808521));
#57752=CARTESIAN_POINT('Ctrl Pts',(20.5705450361326,11.8598649455765,35.5415049564609));
#57753=CARTESIAN_POINT('Ctrl Pts',(18.1643293692783,11.9855877404956,36.2287085043811));
#57754=CARTESIAN_POINT('Ctrl Pts',(17.4310134698452,12.1113105354147,38.6212741447195));
#57755=CARTESIAN_POINT('Ctrl Pts',(19.0388893380848,12.2370333303337,40.5387875720576));
#57756=CARTESIAN_POINT('Ctrl Pts',(21.5226531656758,12.3627561252528,40.233763310006));
#57757=CARTESIAN_POINT('Ctrl Pts',(22.6187791000131,12.4884789201719,37.9841787955316));
#57758=CARTESIAN_POINT('Ctrl Pts',(21.3283358568412,12.614201715091,35.840145496387));
#57759=CARTESIAN_POINT('Ctrl Pts',(18.8273417072175,12.7399245100101,35.7555830032952));
#57760=CARTESIAN_POINT('Ctrl Pts',(17.3950249948361,12.8656473049291,37.8075555633267));
#57761=CARTESIAN_POINT('Ctrl Pts',(18.3366973888574,12.9913700998482,40.1260412014163));
#57762=CARTESIAN_POINT('Ctrl Pts',(20.7941855859771,13.1170928947673,40.5981368619626));
#57763=CARTESIAN_POINT('Ctrl Pts',(22.5279094760174,13.2428156896864,38.7936081077463));
#57764=CARTESIAN_POINT('Ctrl Pts',(21.9578763065307,13.3685384846054,36.3569742129286));
#57765=CARTESIAN_POINT('Ctrl Pts',(19.6035738008031,13.4942612795245,35.5088101585062));
#57766=CARTESIAN_POINT('Ctrl Pts',(17.6105459624027,13.6199840744436,37.0220723919115));
#57767=CARTESIAN_POINT('Ctrl Pts',(17.7950967357975,13.7457068693627,39.5176812482286));
#57768=CARTESIAN_POINT('Ctrl Pts',(19.9890396605614,13.8714296642818,40.7213161573968));
#57769=CARTESIAN_POINT('Ctrl Pts',(22.1929710598319,13.9971524592008,39.5360697952432));
#57770=CARTESIAN_POINT('Ctrl Pts',(22.3983844708772,14.1228752541199,37.0420914709082));
#57771=CARTESIAN_POINT('Ctrl Pts',(20.4180807078455,14.248598049039,35.5122158034726));
#57772=CARTESIAN_POINT('Ctrl Pts',(18.0567678971051,14.3743208439581,36.3406627610522));
#57773=CARTESIAN_POINT('Ctrl Pts',(17.4663787360504,14.5000436388772,38.7724446571519));
#57774=CARTESIAN_POINT('Ctrl Pts',(19.1849519521561,14.6257664337962,40.5914082776165));
#57775=CARTESIAN_POINT('Ctrl Pts',(21.6463020405699,14.7514892287153,40.1398794369485));
#57776=CARTESIAN_POINT('Ctrl Pts',(22.60732943782,14.8772120236344,37.8293494342383));
#57777=CARTESIAN_POINT('Ctrl Pts',(21.192222066054,15.0029348185535,35.7654711243414));
#57778=CARTESIAN_POINT('Ctrl Pts',(18.6906082243163,15.1286576134725,35.8291165367105));
#57779=CARTESIAN_POINT('Ctrl Pts',(17.3822809996572,15.2543804083917,37.9622837652478));
#57780=CARTESIAN_POINT('Ctrl Pts',(18.4595568530001,15.3801032033107,40.2209557838228));
#57781=CARTESIAN_POINT('Ctrl Pts',(20.9406831243936,15.5058259982298,40.5467394192171));
#57782=CARTESIAN_POINT('Ctrl Pts',(22.5645376425225,15.6315487931489,38.6427386167903));
#57783=CARTESIAN_POINT('Ctrl Pts',(21.8512547930222,15.7572715880679,36.2441244068143));
#57784=CARTESIAN_POINT('Ctrl Pts',(19.4508698780133,15.8829943829871,35.5368233312554));
#57785=CARTESIAN_POINT('Ctrl Pts',(17.5509231341999,16.0087171779061,37.165419328537));
#57786=CARTESIAN_POINT('Ctrl Pts',(17.8828910109209,16.1344399728252,39.6457257371314));
#57787=CARTESIAN_POINT('Ctrl Pts',(20.144241575452,16.2601627677443,40.717367550418));
#57788=CARTESIAN_POINT('Ctrl Pts',(22.2741406181319,16.3858855626634,39.4037265721894));
#57789=CARTESIAN_POINT('Ctrl Pts',(22.3315495051783,16.5116083575824,36.9019618407693));
#57790=CARTESIAN_POINT('Ctrl Pts',(20.2641498564961,16.6373311525015,35.4920039533422));
#57791=CARTESIAN_POINT('Ctrl Pts',(17.9560227994754,16.7630539474206,36.4587883348557));
#57792=CARTESIAN_POINT('Ctrl Pts',(17.5106313150273,16.8887767423397,38.9212564010996));
#57793=CARTESIAN_POINT('Ctrl Pts',(19.3338735519126,17.0144995372588,40.6352897430527));
#57794=CARTESIAN_POINT('Ctrl Pts',(21.7641760976727,17.1402223321778,40.0388401745554));
#57795=CARTESIAN_POINT('Ctrl Pts',(22.5867339129275,17.2659451270969,37.6754694477643));
#57796=CARTESIAN_POINT('Ctrl Pts',(21.0519262570048,17.391667922016,35.6989856985238));
#57797=CARTESIAN_POINT('Ctrl Pts',(18.5584677618551,17.5173907169351,35.9106157640885));
#57798=CARTESIAN_POINT('Ctrl Pts',(17.3787193111763,17.6431135118542,38.1174950414426));
#57799=CARTESIAN_POINT('Ctrl Pts',(18.587819808286,17.7688363067732,40.3084305812485));
#57800=CARTESIAN_POINT('Ctrl Pts',(21.0838809805431,17.8945591016923,40.4867594235869));
#57801=CARTESIAN_POINT('Ctrl Pts',(22.5921700493026,18.0202818966114,38.489965333854));
#57802=CARTESIAN_POINT('Ctrl Pts',(21.7381395384649,18.1460046915305,36.1377845503528));
#57803=CARTESIAN_POINT('Ctrl Pts',(19.3000921670417,18.2717274864495,35.5738274897759));
#57804=CARTESIAN_POINT('Ctrl Pts',(17.4998910580062,18.3974502813686,37.312044541547));
#57805=CARTESIAN_POINT('Ctrl Pts',(17.978111577537,18.5231730762877,39.7683482048675));
#57806=CARTESIAN_POINT('Ctrl Pts',(20.2989375265839,18.6488958712068,40.7042378695672));
#57807=CARTESIAN_POINT('Ctrl Pts',(22.3473330575957,18.7746186661259,39.2668102007657));
#57808=CARTESIAN_POINT('Ctrl Pts',(22.2565360433367,18.9003414610449,36.7660346304049));
#57809=CARTESIAN_POINT('Ctrl Pts',(20.1092924347572,19.026064255964,35.480940304005));
#57810=CARTESIAN_POINT('Ctrl Pts',(17.8624474620928,19.1517870508831,36.5826708710764));
#57811=CARTESIAN_POINT('Ctrl Pts',(17.5636159856029,19.2775098458022,39.0671873812369));
#57812=CARTESIAN_POINT('Ctrl Pts',(19.4851317460922,19.4032326407212,40.6702780445947));
#57813=CARTESIAN_POINT('Ctrl Pts',(21.8758618861422,19.5289554356404,39.9309999405283));
#57814=CARTESIAN_POINT('Ctrl Pts',(22.5570647266494,19.6546782305594,37.5230786143868));
#57815=CARTESIAN_POINT('Ctrl Pts',(20.9079406351558,19.7804010254785,35.640922422434));
#57816=CARTESIAN_POINT('Ctrl Pts',(18.431383675432,19.9061238203976,35.999794827407));
#57817=CARTESIAN_POINT('Ctrl Pts',(17.3843527335073,20.0318466153166,38.2726449087205));
#57818=CARTESIAN_POINT('Ctrl Pts',(18.7210357382066,20.1575694102357,40.3881588326942));
#57819=CARTESIAN_POINT('Ctrl Pts',(21.2232780187304,20.2832922051548,40.4184071172065));
#57820=CARTESIAN_POINT('Ctrl Pts',(22.6107075074267,20.4090150000739,38.3358244456626));
#57821=CARTESIAN_POINT('Ctrl Pts',(21.6189317058165,20.534737794993,36.0383270834549));
#57822=CARTESIAN_POINT('Ctrl Pts',(19.1517610640266,20.660460589912,35.6196939448752));
#57823=CARTESIAN_POINT('Ctrl Pts',(17.4576452053814,20.7861833848311,37.4614315506035));
#57824=CARTESIAN_POINT('Ctrl Pts',(18.080392516306,20.9119061797502,39.8851227001952));
#57825=CARTESIAN_POINT('Ctrl Pts',(20.4526467244417,21.0376289746693,40.6819650732079));
#57826=CARTESIAN_POINT('Ctrl Pts',(22.4121717690902,21.1633517695884,39.1258166429392));
#57827=CARTESIAN_POINT('Ctrl Pts',(22.1738395607332,21.2890745645074,36.6347562261618));
#57828=CARTESIAN_POINT('Ctrl Pts',(19.9536010856973,21.4147973594266,35.4791225704681));
#57829=CARTESIAN_POINT('Ctrl Pts',(17.7772456994095,21.5405201543456,36.7117620238512));
#57830=CARTESIAN_POINT('Ctrl Pts',(17.6234268263395,21.6662429492647,39.2099425611065));
#57831=CARTESIAN_POINT('Ctrl Pts',(19.6420258819895,21.7919823967325,40.6960636777901));
#57832=CARTESIAN_POINT('Ctrl Pts',(21.1957550240706,21.8758142458938,40.1098185863196));
#57833=CARTESIAN_POINT('Ctrl Pts',(21.6779259041872,21.9177384967489,39.5529549508008));
#57834=CARTESIAN_POINT('Ctrl Pts',(18.9080039791026,0.12675513256823,36.0004966849229));
#57835=CARTESIAN_POINT('Ctrl Pts',(18.2115290830147,0.16866273087459,36.3627479896582));
#57836=CARTESIAN_POINT('Ctrl Pts',(17.2192736957306,0.252477927487309,37.8285544616862));
#57837=CARTESIAN_POINT('Ctrl Pts',(18.260316732765,0.378200722406389,40.2896669677291));
#57838=CARTESIAN_POINT('Ctrl Pts',(20.8891071501034,0.503923517325469,40.7489098883695));
#57839=CARTESIAN_POINT('Ctrl Pts',(22.7064403355186,0.629646312244547,38.7972650707732));
#57840=CARTESIAN_POINT('Ctrl Pts',(22.0579280756295,0.755369107163628,36.2085764107035));
#57841=CARTESIAN_POINT('Ctrl Pts',(19.5336507759943,0.881091902082706,35.3444239829199));
#57842=CARTESIAN_POINT('Ctrl Pts',(17.4345338599763,1.00681469700178,36.9910810799666));
#57843=CARTESIAN_POINT('Ctrl Pts',(17.6733164611056,1.13253749192086,39.6485481925792));
#57844=CARTESIAN_POINT('Ctrl Pts',(20.0325164509972,1.25826028683994,40.8946649575679));
#57845=CARTESIAN_POINT('Ctrl Pts',(22.3620608920454,1.38398308175902,39.5939812684537));
#57846=CARTESIAN_POINT('Ctrl Pts',(22.5390024274368,1.5097058766781,36.9317589832509));
#57847=CARTESIAN_POINT('Ctrl Pts',(20.4020716216036,1.63542867159718,35.33420414241));
#57848=CARTESIAN_POINT('Ctrl Pts',(17.8987243836568,1.76115146651626,36.2571910565391));
#57849=CARTESIAN_POINT('Ctrl Pts',(17.3103288377261,1.88687426143534,38.8595872415529));
#57850=CARTESIAN_POINT('Ctrl Pts',(19.1731092749576,2.01259705635442,40.7697474494891));
#57851=CARTESIAN_POINT('Ctrl Pts',(21.7894587369895,2.1383198512735,40.2468906535202));
#57852=CARTESIAN_POINT('Ctrl Pts',(22.77502288537,2.26404264619258,37.7675097067451));
#57853=CARTESIAN_POINT('Ctrl Pts',(21.2316282608502,2.38976544111166,35.5911370802761));
#57854=CARTESIAN_POINT('Ctrl Pts',(18.5658152186384,2.51548823603074,35.7011636835708));
#57855=CARTESIAN_POINT('Ctrl Pts',(17.2070162410056,2.64121103094982,37.9973193192089));
#57856=CARTESIAN_POINT('Ctrl Pts',(18.3935442032701,2.76693382586889,40.3870507902624));
#57857=CARTESIAN_POINT('Ctrl Pts',(21.0440818136342,2.89265662078798,40.692526713073));
#57858=CARTESIAN_POINT('Ctrl Pts',(22.7431174571279,3.01837941570705,38.6353580075387));
#57859=CARTESIAN_POINT('Ctrl Pts',(21.9422707779827,3.14410221062614,36.0903020628022));
#57860=CARTESIAN_POINT('Ctrl Pts',(19.3713765334573,3.26982500554521,35.3767420031119));
#57861=CARTESIAN_POINT('Ctrl Pts',(17.373365044879,3.3955478004643,37.1449657645987));
#57862=CARTESIAN_POINT('Ctrl Pts',(17.7690820021981,3.52127059538337,39.7835398613493));
#57863=CARTESIAN_POINT('Ctrl Pts',(20.1978990902937,3.64699339030245,40.8878553636448));
#57864=CARTESIAN_POINT('Ctrl Pts',(22.4463650105696,3.77271618522153,39.4515175963588));
#57865=CARTESIAN_POINT('Ctrl Pts',(22.4653877024197,3.89843898014061,36.7835027326575));
#57866=CARTESIAN_POINT('Ctrl Pts',(20.2376312363324,4.02416177505969,35.3152499261521));
#57867=CARTESIAN_POINT('Ctrl Pts',(17.7933145478616,4.14988456997877,36.3848204485987));
#57868=CARTESIAN_POINT('Ctrl Pts',(17.3600141702051,4.27560736489784,39.0174837310305));
#57869=CARTESIAN_POINT('Ctrl Pts',(19.3326092765973,4.40133015981694,40.8140175387337));
#57870=CARTESIAN_POINT('Ctrl Pts',(21.913416862547,4.527052954736,40.1371886236553));
#57871=CARTESIAN_POINT('Ctrl Pts',(22.7504722901491,4.65277574965509,37.6038107625591));
#57872=CARTESIAN_POINT('Ctrl Pts',(21.0809427250616,4.77849854457416,35.5226245125383));
#57873=CARTESIAN_POINT('Ctrl Pts',(18.4263187737112,4.90422133949325,35.7902751297487));
#57874=CARTESIAN_POINT('Ctrl Pts',(17.2058360639291,5.02994413441233,38.1628448613054));
#57875=CARTESIAN_POINT('Ctrl Pts',(18.5317558081385,5.1556669293314,40.4781422521153));
#57876=CARTESIAN_POINT('Ctrl Pts',(21.1957289732478,5.28138972425049,40.6261697885866));
#57877=CARTESIAN_POINT('Ctrl Pts',(22.7699997223748,5.40711251916956,38.4720256930304));
#57878=CARTESIAN_POINT('Ctrl Pts',(21.8198895647289,5.53283531408866,35.978843817532));
#57879=CARTESIAN_POINT('Ctrl Pts',(19.2112613817822,5.65855810900771,35.4187329542988));
#57880=CARTESIAN_POINT('Ctrl Pts',(17.3214335265685,5.78428090392682,37.302138341791));
#57881=CARTESIAN_POINT('Ctrl Pts',(17.8726608124202,5.91000369884587,39.9126581473677));
#57882=CARTESIAN_POINT('Ctrl Pts',(20.3625938620227,6.03572649376497,40.8712501275516));
#57883=CARTESIAN_POINT('Ctrl Pts',(22.5220846322238,6.16144928868404,39.30432167054));
#57884=CARTESIAN_POINT('Ctrl Pts',(22.3831266916095,6.28717208360312,36.6398600238435));
#57885=CARTESIAN_POINT('Ctrl Pts',(20.0723564327029,6.4128948785222,35.3060661917509));
#57886=CARTESIAN_POINT('Ctrl Pts',(17.695645662784,6.53861767344128,36.5184650915059));
#57887=CARTESIAN_POINT('Ctrl Pts',(17.418959685041,6.66434046836036,39.1721625206974));
#57888=CARTESIAN_POINT('Ctrl Pts',(19.4944504378819,6.79006326327943,40.8487672179494));
#57889=CARTESIAN_POINT('Ctrl Pts',(22.0306631365517,6.91578605819852,40.0203408041494));
#57890=CARTESIAN_POINT('Ctrl Pts',(22.7162737544373,7.04150885311759,37.4418522436515));
#57891=CARTESIAN_POINT('Ctrl Pts',(20.9264654948829,7.16723164803668,35.463152779355));
#57892=CARTESIAN_POINT('Ctrl Pts',(18.2923424192746,7.29295444295576,35.887488493765));
#57893=CARTESIAN_POINT('Ctrl Pts',(17.2144571141139,7.41867723787484,38.3281499706796));
#57894=CARTESIAN_POINT('Ctrl Pts',(18.6751176504306,7.54440003279391,40.5608917769847));
#57895=CARTESIAN_POINT('Ctrl Pts',(21.3431818120828,7.670122827713,40.5509516922863));
#57896=CARTESIAN_POINT('Ctrl Pts',(22.7871655186511,7.79584562263208,38.3073884034218));
#57897=CARTESIAN_POINT('Ctrl Pts',(21.6911246315466,7.92156841755115,35.8748260609994));
#57898=CARTESIAN_POINT('Ctrl Pts',(19.0539129290207,8.04729121247024,35.4701291224934));
#57899=CARTESIAN_POINT('Ctrl Pts',(17.2788977526653,8.1730140073893,37.4621096193065));
#57900=CARTESIAN_POINT('Ctrl Pts',(17.9837017990567,8.2987368023084,40.0354180796676));
#57901=CARTESIAN_POINT('Ctrl Pts',(20.5260167447122,8.42445959722746,40.8449240358367));
#57902=CARTESIAN_POINT('Ctrl Pts',(22.58895740875,8.55018239214656,39.1529012840289));
#57903=CARTESIAN_POINT('Ctrl Pts',(22.2925062655231,8.67590518706562,36.5013391226503));
#57904=CARTESIAN_POINT('Ctrl Pts',(19.90682782072,8.80162798198472,35.3066828817265));
#57905=CARTESIAN_POINT('Ctrl Pts',(17.6060598791625,8.92735077690378,36.6576573652298));
#57906=CARTESIAN_POINT('Ctrl Pts',(17.4869588468777,9.05307357182287,39.3230804311022));
#57907=CARTESIAN_POINT('Ctrl Pts',(19.6580649411979,9.17879636674194,40.8738749059382));
#57908=CARTESIAN_POINT('Ctrl Pts',(22.1407863497089,9.30451916166103,39.8967569070777));
#57909=CARTESIAN_POINT('Ctrl Pts',(22.6725472064794,9.4302419565801,37.2822023432595));
#57910=CARTESIAN_POINT('Ctrl Pts',(20.7687384543469,9.55596475149919,35.4129304499065));
#57911=CARTESIAN_POINT('Ctrl Pts',(18.1643561025926,9.68168754641826,35.9924627974476));
#57912=CARTESIAN_POINT('Ctrl Pts',(17.2328491554166,9.80741034133735,38.4926547867434));
#57913=CARTESIAN_POINT('Ctrl Pts',(18.8231268502398,9.93313313625642,40.6350091060201));
#57914=CARTESIAN_POINT('Ctrl Pts',(21.4859231034409,10.0588559311755,40.4671362674954));
#57915=CARTESIAN_POINT('Ctrl Pts',(22.7945546320177,10.1845787260945,38.1420236469132));
#57916=CARTESIAN_POINT('Ctrl Pts',(21.5564276540805,10.3103015210136,35.7786136607956));
#57917=CARTESIAN_POINT('Ctrl Pts',(18.8998831142219,10.4360243159327,35.5307502231475));
#57918=CARTESIAN_POINT('Ctrl Pts',(17.2459069281592,10.5617471108518,37.6243184575056));
#57919=CARTESIAN_POINT('Ctrl Pts',(18.1018154579225,10.6874699057709,40.1513890470726));
#57920=CARTESIAN_POINT('Ctrl Pts',(20.6875944915874,10.81319270069,40.8089694338198));
#57921=CARTESIAN_POINT('Ctrl Pts',(22.6467487670819,10.938915495609,38.9977875818823));
#57922=CARTESIAN_POINT('Ctrl Pts',(22.1938442980656,11.0646382905281,36.3684259259055));
#57923=CARTESIAN_POINT('Ctrl Pts',(19.7416260335514,11.1903610854472,35.3170978328922));
#57924=CARTESIAN_POINT('Ctrl Pts',(17.5248714416295,11.3160838803663,36.8019090179151));
#57925=CARTESIAN_POINT('Ctrl Pts',(17.5637731315797,11.4418066752854,39.4697080797815));
#57926=CARTESIAN_POINT('Ctrl Pts',(19.8228788675921,11.5675294702044,40.8892525311785));
#57927=CARTESIAN_POINT('Ctrl Pts',(22.2434002171962,11.6932522651235,39.7668704339915));
#57928=CARTESIAN_POINT('Ctrl Pts',(22.6194460281224,11.8189750600426,37.1254210734962));
#57929=CARTESIAN_POINT('Ctrl Pts',(20.6083148706532,11.9446978549617,35.3721336916239));
#57930=CARTESIAN_POINT('Ctrl Pts',(18.0428087678081,12.0704206498807,36.1048298170676));
#57931=CARTESIAN_POINT('Ctrl Pts',(17.2609476731339,12.1961434447998,38.6557822675478));
#57932=CARTESIAN_POINT('Ctrl Pts',(18.9752642281328,12.3218662397189,40.7002342540793));
#57933=CARTESIAN_POINT('Ctrl Pts',(21.6234521464007,12.447589034638,40.3750175178618));
#57934=CARTESIAN_POINT('Ctrl Pts',(22.7921411433041,12.5733118295571,37.976511481911));
#57935=CARTESIAN_POINT('Ctrl Pts',(21.4162711158012,12.6990346244761,35.6905441060732));
#57936=CARTESIAN_POINT('Ctrl Pts',(18.7497122356375,12.8247574193952,35.6003836125284));
#57937=CARTESIAN_POINT('Ctrl Pts',(17.2225767766511,12.9504802143143,37.7881958681579));
#57938=CARTESIAN_POINT('Ctrl Pts',(18.2265874757008,13.0762030092334,40.2601642522943));
#57939=CARTESIAN_POINT('Ctrl Pts',(20.8467603281295,13.2019258041525,40.7635124412958));
#57940=CARTESIAN_POINT('Ctrl Pts',(22.6952559895186,13.3276485990715,38.839524664359));
#57941=CARTESIAN_POINT('Ctrl Pts',(22.0874868708618,13.4533713939906,36.2415866600212));
#57942=CARTESIAN_POINT('Ctrl Pts',(19.5773305579474,13.5790941889097,35.3372745121915));
#57943=CARTESIAN_POINT('Ctrl Pts',(17.4523651390159,13.7048169838288,36.9507140506687));
#57944=CARTESIAN_POINT('Ctrl Pts',(17.6491330937556,13.8305397787478,39.6115311334393));
#57945=CARTESIAN_POINT('Ctrl Pts',(19.988314090833,13.956262573667,40.8948461527887));
#57946=CARTESIAN_POINT('Ctrl Pts',(22.3381447951075,14.081985368586,39.6311369943095));
#57947=CARTESIAN_POINT('Ctrl Pts',(22.5571564850828,14.2077081635051,36.972058384033));
#57948=CARTESIAN_POINT('Ctrl Pts',(20.4457574698038,14.3334309584241,35.3409056093809));
#57949=CARTESIAN_POINT('Ctrl Pts',(17.9281267727182,14.4591537533433,36.2241953970884));
#57950=CARTESIAN_POINT('Ctrl Pts',(17.2986541046595,14.5848765482623,38.8169602024926));
#57951=CARTESIAN_POINT('Ctrl Pts',(19.1309961240551,14.7105993431814,40.7563384275775));
#57952=CARTESIAN_POINT('Ctrl Pts',(21.7552865233107,14.8363221381005,40.274918573031));
#57953=CARTESIAN_POINT('Ctrl Pts',(22.779933518428,14.9620449330196,37.8114324838938));
#57954=CARTESIAN_POINT('Ctrl Pts',(21.2711466509595,15.0877677279387,35.6109263229093));
#57955=CARTESIAN_POINT('Ctrl Pts',(18.6039270553319,15.2134905228577,35.6787850340383));
#57956=CARTESIAN_POINT('Ctrl Pts',(17.2089891345057,15.3392133177768,37.9531670100962));
#57957=CARTESIAN_POINT('Ctrl Pts',(18.3575801832093,15.4649361126959,40.3613621389871));
#57958=CARTESIAN_POINT('Ctrl Pts',(21.0029559402006,15.590658907615,40.70871251008));
#57959=CARTESIAN_POINT('Ctrl Pts',(22.7343089247975,15.7163817025341,38.6786676783821));
#57960=CARTESIAN_POINT('Ctrl Pts',(21.9738070592936,15.8421044974531,36.1212662455716));
#57961=CARTESIAN_POINT('Ctrl Pts',(19.414517701543,15.9678272923722,35.3671421448555));
#57962=CARTESIAN_POINT('Ctrl Pts',(17.3887953053845,16.0935500872913,37.1035504924735));
#57963=CARTESIAN_POINT('Ctrl Pts',(17.7427393119042,16.2192728822104,39.7480521121034));
#57964=CARTESIAN_POINT('Ctrl Pts',(20.1537903053346,16.3449956771294,40.8906361497366));
#57965=CARTESIAN_POINT('Ctrl Pts',(22.4246877430453,16.4707184720485,39.4900327071537));
#57966=CARTESIAN_POINT('Ctrl Pts',(22.4858970735737,16.5964412669676,36.8226522330121));
#57967=CARTESIAN_POINT('Ctrl Pts',(20.2816364627001,16.7221640618867,35.3193557435175));
#57968=CARTESIAN_POINT('Ctrl Pts',(17.8207123932173,16.8478868568058,36.3501408327656));
#57969=CARTESIAN_POINT('Ctrl Pts',(17.3458361852168,16.9736096517248,38.9756232194996));
#57970=CARTESIAN_POINT('Ctrl Pts',(19.289776269278,17.0993324466439,40.8031248270383));
#57971=CARTESIAN_POINT('Ctrl Pts',(21.8809637919903,17.225055241563,40.1671905551865));
#57972=CARTESIAN_POINT('Ctrl Pts',(22.7579745786992,17.3507780364821,37.6473657088982));
#57973=CARTESIAN_POINT('Ctrl Pts',(21.1215633200564,17.4765008314011,35.5400395906704));
#57974=CARTESIAN_POINT('Ctrl Pts',(18.4630389514322,17.6022236263203,35.7656794750045));
#57975=CARTESIAN_POINT('Ctrl Pts',(17.2051916637884,17.7279464212393,38.1186532056162));
#57976=CARTESIAN_POINT('Ctrl Pts',(18.4943340906363,17.8536692161584,40.4546277301526));
#57977=CARTESIAN_POINT('Ctrl Pts',(21.1556334324663,17.9793920110775,40.6447618646919));
#57978=CARTESIAN_POINT('Ctrl Pts',(22.7637705849502,18.1051148059966,38.5157808702195));
#57979=CARTESIAN_POINT('Ctrl Pts',(21.8532036238288,18.2308376009156,36.0078867366249));
#57980=CARTESIAN_POINT('Ctrl Pts',(19.2537585713457,18.3565603958347,35.4065959626586));
#57981=CARTESIAN_POINT('Ctrl Pts',(17.3343849278281,18.4822831907538,37.259882231141));
#57982=CARTESIAN_POINT('Ctrl Pts',(17.8442634388288,18.6080059856729,39.8787921341454));
#57983=CARTESIAN_POINT('Ctrl Pts',(20.3187270614952,18.733728780592,40.8766372896946));
#57984=CARTESIAN_POINT('Ctrl Pts',(22.5027254903318,18.859451575511,39.3440525311847));
#57985=CARTESIAN_POINT('Ctrl Pts',(22.405917753016,18.9851743704301,36.6777267001364));
#57986=CARTESIAN_POINT('Ctrl Pts',(20.1165275466479,19.1108971653492,35.3075596853814));
#57987=CARTESIAN_POINT('Ctrl Pts',(17.7209424089894,19.2366199602683,36.4822243392808));
#57988=CARTESIAN_POINT('Ctrl Pts',(17.4023284180584,19.3623427551874,39.1312147673787));
#57989=CARTESIAN_POINT('Ctrl Pts',(19.4510476904639,19.4880655501064,40.8404293390032));
#57990=CARTESIAN_POINT('Ctrl Pts',(22.0000431313306,19.6137883450255,40.0522113443288));
#57991=CARTESIAN_POINT('Ctrl Pts',(22.7263413051272,19.7395111399446,37.4848866682896));
#57992=CARTESIAN_POINT('Ctrl Pts',(20.9680459123426,19.8652339348637,35.4781325508272));
#57993=CARTESIAN_POINT('Ctrl Pts',(18.3275419534764,19.9909567297828,35.8607621537274));
#57994=CARTESIAN_POINT('Ctrl Pts',(17.2111980162402,20.1166795247018,38.2840739269754));
#57995=CARTESIAN_POINT('Ctrl Pts',(18.636368857476,20.2424023196209,40.5396339573463));
#57996=CARTESIAN_POINT('Ctrl Pts',(21.3042584942653,20.36812511454,40.5718846652048));
#57997=CARTESIAN_POINT('Ctrl Pts',(22.7835352147811,20.4938479094591,38.3514359219257));
#57998=CARTESIAN_POINT('Ctrl Pts',(21.7261042842396,20.6195707043781,35.901845228453));
#57999=CARTESIAN_POINT('Ctrl Pts',(19.095608013493,20.7452934992973,35.4554987572394));
#58000=CARTESIAN_POINT('Ctrl Pts',(17.2893424180392,20.8710162942162,37.4191585955583));
#58001=CARTESIAN_POINT('Ctrl Pts',(17.953315331488,20.9967390891354,40.0032970505363));
#58002=CARTESIAN_POINT('Ctrl Pts',(20.4826117417423,21.1224618840544,40.8528900438537));
#58003=CARTESIAN_POINT('Ctrl Pts',(22.5718564964719,21.2481846789736,39.1937252608371));
#58004=CARTESIAN_POINT('Ctrl Pts',(22.3177467990465,21.3739074738926,36.5377577223358));
#58005=CARTESIAN_POINT('Ctrl Pts',(19.9505294976469,21.4996302688117,35.3056216186709));
#58006=CARTESIAN_POINT('Ctrl Pts',(17.6301003264828,21.6253530637308,36.6198612705124));
#58007=CARTESIAN_POINT('Ctrl Pts',(17.466098710572,21.7510758586498,39.2834202783864));
#58008=CARTESIAN_POINT('Ctrl Pts',(19.6183281502704,21.8768153061177,40.8679219699589));
#58009=CARTESIAN_POINT('Ctrl Pts',(21.2749134892681,21.960647155279,40.2428677070976));
#58010=CARTESIAN_POINT('Ctrl Pts',(21.789003873016,22.002571406134,39.6491399398589));
#58011=CARTESIAN_POINT('Ctrl Pts',(17.8632119920882,21.75,39.1124570460077));
#58012=CARTESIAN_POINT('Ctrl Pts',(17.8700018959015,21.75,39.1256475418322));
#58013=CARTESIAN_POINT('Ctrl Pts',(17.8767917997148,21.75,39.1388380376567));
#58014=CARTESIAN_POINT('Ctrl Pts',(17.883581703528,21.75,39.1520285334812));
#58015=CARTESIAN_POINT('Ctrl Pts',(18.7894999003326,0.125000000000002,39.6065358483297));
#58016=CARTESIAN_POINT('Ctrl Pts',(18.7303882588618,0.125000000000002,39.5691127845715));
#58017=CARTESIAN_POINT('Ctrl Pts',(18.6736284073276,0.124999999999993,39.5282205607498));
#58018=CARTESIAN_POINT('Ctrl Pts',(18.6193051004316,0.125,39.4842200364387));
#58019=CARTESIAN_POINT('Ctrl Pts',(18.5728930747577,0.125000000000007,39.44662745269));
#58020=CARTESIAN_POINT('Ctrl Pts',(18.5282595960142,0.124999999999996,39.4067648264074));
#58021=CARTESIAN_POINT('Ctrl Pts',(18.4854679692591,0.125000000000011,39.3648290378955));
#58022=CARTESIAN_POINT('Ctrl Pts',(18.4735851139617,0.125000000000015,39.3531838412892));
#58023=CARTESIAN_POINT('Ctrl Pts',(18.4618427346802,0.125000000000011,39.34137695956));
#58024=CARTESIAN_POINT('Ctrl Pts',(18.4502475884037,0.125000000000005,39.3294177166378));
#58025=CARTESIAN_POINT('Ctrl Pts',(18.3993536433843,0.12499999999998,39.2769256620104));
#58026=CARTESIAN_POINT('Ctrl Pts',(18.3513818001719,0.125000000000007,39.2215941156987));
#58027=CARTESIAN_POINT('Ctrl Pts',(18.3064347445308,0.124999999999996,39.1637898014797));
#58028=CARTESIAN_POINT('Ctrl Pts',(18.2713288207951,0.124999999999988,39.1186417085152));
#58029=CARTESIAN_POINT('Ctrl Pts',(18.2380684235828,0.125000000000006,39.0719839207988));
#58030=CARTESIAN_POINT('Ctrl Pts',(18.2067137449448,0.125,39.0239722527309));
#58031=CARTESIAN_POINT('Ctrl Pts',(18.1984121807502,0.124999999999998,39.0112605311675));
#58032=CARTESIAN_POINT('Ctrl Pts',(18.190244268825,0.125000000000026,38.9984538246221));
#58033=CARTESIAN_POINT('Ctrl Pts',(18.1822112672552,0.125000000000005,38.9855548636928));
#58034=CARTESIAN_POINT('Ctrl Pts',(18.1745479872583,0.124999999999984,38.9732495817366));
#58035=CARTESIAN_POINT('Ctrl Pts',(18.1670119998787,0.124999999999989,38.960867533343));
#58036=CARTESIAN_POINT('Ctrl Pts',(18.1596062445286,0.124999999999994,38.9484152505001));
#58037=CARTESIAN_POINT('Ctrl Pts',(18.1209741842544,0.125000000000019,38.883458022156));
#58038=CARTESIAN_POINT('Ctrl Pts',(18.0858635979701,0.124999999999999,38.8165609525249));
#58039=CARTESIAN_POINT('Ctrl Pts',(18.0543793695552,0.125000000000003,38.7480970247487));
#58040=CARTESIAN_POINT('Ctrl Pts',(18.0223692110303,0.125000000000007,38.6784894373409));
#58041=CARTESIAN_POINT('Ctrl Pts',(17.9941068720973,0.125000000000014,38.607261439698));
#58042=CARTESIAN_POINT('Ctrl Pts',(17.9697368784911,0.125000000000005,38.5347637724566));
#58043=CARTESIAN_POINT('Ctrl Pts',(17.9523900077114,0.124999999999998,38.4831590126941));
#58044=CARTESIAN_POINT('Ctrl Pts',(17.9370159956698,0.125000000000009,38.4309100395559));
#58045=CARTESIAN_POINT('Ctrl Pts',(17.9236803055237,0.125000000000006,38.3781343478896));
#58046=CARTESIAN_POINT('Ctrl Pts',(17.9125026607243,0.125000000000004,38.3338990717977));
#58047=CARTESIAN_POINT('Ctrl Pts',(17.9027571739107,0.124999999999998,38.2892935789823));
#58048=CARTESIAN_POINT('Ctrl Pts',(17.8944894387071,0.124999999999992,38.2443844913444));
#58049=CARTESIAN_POINT('Ctrl Pts',(17.8922469722116,0.12499999999999,38.2322037523763));
#58050=CARTESIAN_POINT('Ctrl Pts',(17.8901140385265,0.125000000000003,38.2200045883144));
#58051=CARTESIAN_POINT('Ctrl Pts',(17.8880928384044,0.125000000000004,38.2077979591711));
#58052=CARTESIAN_POINT('Ctrl Pts',(17.8752443028934,0.125000000000006,38.1302018288823));
#58053=CARTESIAN_POINT('Ctrl Pts',(17.8668864697125,0.125000000000001,38.0521935532589));
#58054=CARTESIAN_POINT('Ctrl Pts',(17.8631561393029,0.125000000000009,37.9741425264019));
#58055=CARTESIAN_POINT('Ctrl Pts',(17.8618719786648,0.125000000000011,37.9472735776917));
#58056=CARTESIAN_POINT('Ctrl Pts',(17.861136579869,0.124999999999983,37.920399299391));
#58057=CARTESIAN_POINT('Ctrl Pts',(17.8609567607682,0.124999999999984,37.893534042365));
#58058=CARTESIAN_POINT('Ctrl Pts',(17.8604471216823,0.124999999999988,37.8173931598032));
#58059=CARTESIAN_POINT('Ctrl Pts',(17.864396119628,0.124999999999993,37.7413254308285));
#58060=CARTESIAN_POINT('Ctrl Pts',(17.8725735026586,0.125,37.6655923866698));
#58061=CARTESIAN_POINT('Ctrl Pts',(17.8807508856893,0.125000000000007,37.5898593425112));
#58062=CARTESIAN_POINT('Ctrl Pts',(17.8931569243958,0.124999999999979,37.5144602026434));
#58063=CARTESIAN_POINT('Ctrl Pts',(17.9096135186795,0.124999999999975,37.4396529031886));
#58064=CARTESIAN_POINT('Ctrl Pts',(17.913388066869,0.124999999999975,37.4224948113105));
#58065=CARTESIAN_POINT('Ctrl Pts',(17.9173773022217,0.124999999999984,37.4053627429111));
#58066=CARTESIAN_POINT('Ctrl Pts',(17.9215715350817,0.124999999999988,37.3882904321903));
#58067=CARTESIAN_POINT('Ctrl Pts',(17.9402979407093,0.125000000000007,37.3120660006368));
#58068=CARTESIAN_POINT('Ctrl Pts',(17.9631261749276,0.124999999999991,37.2369326093909));
#58069=CARTESIAN_POINT('Ctrl Pts',(17.9897910243411,0.124999999999986,37.1631633241872));
#58070=CARTESIAN_POINT('Ctrl Pts',(18.0169444069738,0.12499999999998,37.0880424938904));
#58071=CARTESIAN_POINT('Ctrl Pts',(18.0480764496311,0.124999999999978,37.0143353847301));
#58072=CARTESIAN_POINT('Ctrl Pts',(18.0829617098189,0.124999999999994,36.9423267037387));
#58073=CARTESIAN_POINT('Ctrl Pts',(18.1182336230504,0.125000000000011,36.8695199098616));
#58074=CARTESIAN_POINT('Ctrl Pts',(18.1573426808453,0.125000000000015,36.7984484679073));
#58075=CARTESIAN_POINT('Ctrl Pts',(18.2001077312806,0.125,36.7294163768159));
#58076=CARTESIAN_POINT('Ctrl Pts',(18.2183117477341,0.124999999999993,36.7000311356142));
#58077=CARTESIAN_POINT('Ctrl Pts',(18.237178840091,0.124999999999991,36.6710156254998));
#58078=CARTESIAN_POINT('Ctrl Pts',(18.2566976515838,0.124999999999997,36.6423944743196));
#58079=CARTESIAN_POINT('Ctrl Pts',(18.2653932320242,0.125,36.6296438249024));
#58080=CARTESIAN_POINT('Ctrl Pts',(18.2742193927629,0.125000000000004,36.6169699325046));
#58081=CARTESIAN_POINT('Ctrl Pts',(18.283161973467,0.124999999999999,36.6043931101447));
#58082=CARTESIAN_POINT('Ctrl Pts',(18.3314585616185,0.124999999999973,36.5364689135547));
#58083=CARTESIAN_POINT('Ctrl Pts',(18.383226098352,0.12499999999998,36.4712564282192));
#58084=CARTESIAN_POINT('Ctrl Pts',(18.4382186185833,0.124999999999998,36.4090539912327));
#58085=CARTESIAN_POINT('Ctrl Pts',(18.4931810653168,0.125000000000015,36.3468855705967));
#58086=CARTESIAN_POINT('Ctrl Pts',(18.5513653889031,0.124999999999998,36.2877229691864));
#58087=CARTESIAN_POINT('Ctrl Pts',(18.6125750949098,0.125000000000011,36.23187952165));
#58088=CARTESIAN_POINT('Ctrl Pts',(18.6730802615304,0.125000000000024,36.1766788464909));
#58089=CARTESIAN_POINT('Ctrl Pts',(18.736542045183,0.125000000000005,36.1247204853757));
#58090=CARTESIAN_POINT('Ctrl Pts',(18.802811802905,0.125000000000003,36.0763355898799));
#58091=CARTESIAN_POINT('Ctrl Pts',(18.8375759192312,0.125000000000002,36.0509536027825));
#58092=CARTESIAN_POINT('Ctrl Pts',(18.8731134037565,0.124999999999986,36.0265555500945));
#58093=CARTESIAN_POINT('Ctrl Pts',(18.9094067387628,0.124999999999998,36.0031936714508));
#58094=CARTESIAN_POINT('Origin',(20.,0.125,38.1));
#58095=CARTESIAN_POINT('',(21.1298171225045,0.125,36.0240655813356));
#58096=CARTESIAN_POINT('',(20.,0.125,40.46347));
#58097=CARTESIAN_POINT('Origin',(20.,0.125,38.1));
#58098=CARTESIAN_POINT('Ctrl Pts',(21.1298171225045,0.125000000000001,36.0240655813356));
#58099=CARTESIAN_POINT('Ctrl Pts',(21.1990795490775,0.124999999999983,36.0708787850807));
#58100=CARTESIAN_POINT('Ctrl Pts',(21.2656055745096,0.124999999999974,36.1216762809117));
#58101=CARTESIAN_POINT('Ctrl Pts',(21.3292135975137,0.124999999999986,36.1760987535025));
#58102=CARTESIAN_POINT('Ctrl Pts',(21.3840237393438,0.124999999999996,36.2229938352951));
#58103=CARTESIAN_POINT('Ctrl Pts',(21.4366668305791,0.125000000000016,36.2725815275598));
#58104=CARTESIAN_POINT('Ctrl Pts',(21.4870006796613,0.124999999999999,36.3246488141442));
#58105=CARTESIAN_POINT('Ctrl Pts',(21.4981487712734,0.124999999999995,36.3361808326848));
#58106=CARTESIAN_POINT('Ctrl Pts',(21.5091811000541,0.124999999999995,36.3478321489414));
#58107=CARTESIAN_POINT('Ctrl Pts',(21.5200905103336,0.124999999999994,36.3595940943587));
#58108=CARTESIAN_POINT('Ctrl Pts',(21.5765602420148,0.124999999999991,36.4204767529757));
#58109=CARTESIAN_POINT('Ctrl Pts',(21.6297871336939,0.124999999999987,36.4843697963929));
#58110=CARTESIAN_POINT('Ctrl Pts',(21.679573757162,0.124999999999998,36.5509334434494));
#58111=CARTESIAN_POINT('Ctrl Pts',(21.7155347807542,0.125000000000005,36.5990125601968));
#58112=CARTESIAN_POINT('Ctrl Pts',(21.7497000611184,0.125000000000016,36.6484856808021));
#58113=CARTESIAN_POINT('Ctrl Pts',(21.7819792229568,0.124999999999998,36.6992303718909));
#58114=CARTESIAN_POINT('Ctrl Pts',(21.7899338814766,0.124999999999994,36.71173555066));
#58115=CARTESIAN_POINT('Ctrl Pts',(21.7977739294712,0.124999999999996,36.724317963909));
#58116=CARTESIAN_POINT('Ctrl Pts',(21.805497878986,0.124999999999994,36.736975798943));
#58117=CARTESIAN_POINT('Ctrl Pts',(21.8128135352517,0.124999999999993,36.748964532168));
#58118=CARTESIAN_POINT('Ctrl Pts',(21.8200197531888,0.12500000000002,36.7610122599784));
#58119=CARTESIAN_POINT('Ctrl Pts',(21.8271155484798,0.125000000000018,36.7731169252624));
#58120=CARTESIAN_POINT('Ctrl Pts',(21.8680753538153,0.125000000000005,36.8429899575797));
#58121=CARTESIAN_POINT('Ctrl Pts',(21.9053620001245,0.125000000000023,36.9147624502371));
#58122=CARTESIAN_POINT('Ctrl Pts',(21.9387994467918,0.125000000000017,36.988118275587));
#58123=CARTESIAN_POINT('Ctrl Pts',(21.9716838232338,0.125000000000011,37.0602607629909));
#58124=CARTESIAN_POINT('Ctrl Pts',(22.0008454994912,0.125000000000007,37.1339355659331));
#58125=CARTESIAN_POINT('Ctrl Pts',(22.0260689714308,0.125000000000008,37.2088524461688));
#58126=CARTESIAN_POINT('Ctrl Pts',(22.0443784407949,0.125000000000009,37.2632338702174));
#58127=CARTESIAN_POINT('Ctrl Pts',(22.0606118324242,0.124999999999994,37.3182700210257));
#58128=CARTESIAN_POINT('Ctrl Pts',(22.0746694285563,0.12500000000001,37.3738493642667));
#58129=CARTESIAN_POINT('Ctrl Pts',(22.0852126256554,0.125000000000022,37.4155338716975));
#58130=CARTESIAN_POINT('Ctrl Pts',(22.0945316433851,0.125000000000003,37.457523925268));
#58131=CARTESIAN_POINT('Ctrl Pts',(22.1025786506068,0.125000000000016,37.4997713275294));
#58132=CARTESIAN_POINT('Ctrl Pts',(22.104914689879,0.12500000000002,37.5120357120529));
#58133=CARTESIAN_POINT('Ctrl Pts',(22.1071434994731,0.124999999999998,37.5243217754371));
#58134=CARTESIAN_POINT('Ctrl Pts',(22.1092638278586,0.125000000000007,37.5366283146355));
#58135=CARTESIAN_POINT('Ctrl Pts',(22.1115374551523,0.125000000000018,37.5498246117773));
#58136=CARTESIAN_POINT('Ctrl Pts',(22.1136847973057,0.12500000000001,37.5630356275134));
#58137=CARTESIAN_POINT('Ctrl Pts',(22.115704161457,0.125000000000008,37.5762552059159));
#58138=CARTESIAN_POINT('Ctrl Pts',(22.1272139470258,0.124999999999996,37.6516029398159));
#58139=CARTESIAN_POINT('Ctrl Pts',(22.1345787609411,0.125000000000017,37.7272779645949));
#58140=CARTESIAN_POINT('Ctrl Pts',(22.1376065452356,0.125000000000015,37.8030135753196));
#58141=CARTESIAN_POINT('Ctrl Pts',(22.1386716922244,0.125000000000014,37.8296566746506));
#58142=CARTESIAN_POINT('Ctrl Pts',(22.1391996378238,0.125000000000004,37.8563072559143));
#58143=CARTESIAN_POINT('Ctrl Pts',(22.139180474393,0.125000000000001,37.8829535563851));
#58144=CARTESIAN_POINT('Ctrl Pts',(22.1391246242936,0.124999999999991,37.9606118082407));
#58145=CARTESIAN_POINT('Ctrl Pts',(22.1344253216884,0.124999999999991,38.038235169254));
#58146=CARTESIAN_POINT('Ctrl Pts',(22.1252506920211,0.125000000000001,38.1154926420498));
#58147=CARTESIAN_POINT('Ctrl Pts',(22.1164517360991,0.12500000000001,38.1895866515542));
#58148=CARTESIAN_POINT('Ctrl Pts',(22.1035356471174,0.125000000000017,38.2633447580134));
#58149=CARTESIAN_POINT('Ctrl Pts',(22.0866122802599,0.125000000000001,38.3364515381243));
#58150=CARTESIAN_POINT('Ctrl Pts',(22.0830468966271,0.124999999999997,38.3518535393601));
#58151=CARTESIAN_POINT('Ctrl Pts',(22.0793025198156,0.125000000000007,38.3672300166854));
#58152=CARTESIAN_POINT('Ctrl Pts',(22.0753868276315,0.125000000000004,38.3825525151837));
#58153=CARTESIAN_POINT('Ctrl Pts',(22.0566063195045,0.124999999999987,38.456042537903));
#58154=CARTESIAN_POINT('Ctrl Pts',(22.0338646030691,0.124999999999995,38.5284059841618));
#58155=CARTESIAN_POINT('Ctrl Pts',(22.0073469685367,0.125000000000004,38.5993445283026));
#58156=CARTESIAN_POINT('Ctrl Pts',(21.9809376237444,0.125000000000013,38.6699933815777));
#58157=CARTESIAN_POINT('Ctrl Pts',(21.950782486382,0.125000000000022,38.739229785024));
#58158=CARTESIAN_POINT('Ctrl Pts',(21.9170213476871,0.125000000000023,38.8067321116329));
#58159=CARTESIAN_POINT('Ctrl Pts',(21.8835439844181,0.125000000000023,38.8736670550841));
#58160=CARTESIAN_POINT('Ctrl Pts',(21.8465203603964,0.125000000000007,38.9388977000179));
#58161=CARTESIAN_POINT('Ctrl Pts',(21.8060536812907,0.125000000000008,39.0020721563215));
#58162=CARTESIAN_POINT('Ctrl Pts',(21.7912130945568,0.125000000000008,39.0252405017074));
#58163=CARTESIAN_POINT('Ctrl Pts',(21.7759091563608,0.125000000000006,39.0481318698271));
#58164=CARTESIAN_POINT('Ctrl Pts',(21.7601460791288,0.125000000000019,39.0707272944136));
#58165=CARTESIAN_POINT('Ctrl Pts',(21.7533802017367,0.125000000000025,39.0804257733415));
#58166=CARTESIAN_POINT('Ctrl Pts',(21.7465304429989,0.125000000000001,39.0900685762855));
#58167=CARTESIAN_POINT('Ctrl Pts',(21.7396044503488,0.125000000000002,39.0996444763858));
#58168=CARTESIAN_POINT('Ctrl Pts',(21.6966889753724,0.12500000000001,39.15897955251));
#58169=CARTESIAN_POINT('Ctrl Pts',(21.6507769855365,0.125000000000004,39.2158537293796));
#58170=CARTESIAN_POINT('Ctrl Pts',(21.6020040083035,0.12500000000001,39.2699748866719));
#58171=CARTESIAN_POINT('Ctrl Pts',(21.5546149694859,0.125000000000016,39.3225603503708));
#58172=CARTESIAN_POINT('Ctrl Pts',(21.5045243298926,0.125000000000015,39.3725472978381));
#58173=CARTESIAN_POINT('Ctrl Pts',(21.4518289233424,0.125000000000007,39.4196284362144));
#58174=CARTESIAN_POINT('Ctrl Pts',(21.3998272581665,0.125,39.466089745733));
#58175=CARTESIAN_POINT('Ctrl Pts',(21.3452884405721,0.124999999999977,39.5097217501793));
#58176=CARTESIAN_POINT('Ctrl Pts',(21.2882869596872,0.124999999999972,39.5501829399227));
#58177=CARTESIAN_POINT('Ctrl Pts',(21.2621895577287,0.12499999999997,39.5687075802664));
#58178=CARTESIAN_POINT('Ctrl Pts',(21.2355757334482,0.124999999999981,39.5865668821878));
#58179=CARTESIAN_POINT('Ctrl Pts',(21.2084517554459,0.124999999999999,39.6037243469665));
#58180=CARTESIAN_POINT('Origin',(20.,0.125,38.1));
#58181=CARTESIAN_POINT('Ctrl Pts',(21.4817071279173,-0.127571370348389,
39.9452406715398));
#58182=CARTESIAN_POINT('Ctrl Pts',(22.0940973315942,-0.0856471207638085,
39.4535296222823));
#58183=CARTESIAN_POINT('Ctrl Pts',(22.7801769572279,-0.00181527287286855,
37.8212744373185));
#58184=CARTESIAN_POINT('Ctrl Pts',(21.2766046668293,0.123924173324431,35.6117430346468));
#58185=CARTESIAN_POINT('Ctrl Pts',(18.6087965704713,0.249646968243511,35.6768240224488));
#58186=CARTESIAN_POINT('Ctrl Pts',(17.2093803185729,0.37536976316259,37.9469002644723));
#58187=CARTESIAN_POINT('Ctrl Pts',(18.352852044017,0.501092558081669,40.3581971702879));
#58188=CARTESIAN_POINT('Ctrl Pts',(20.9975643581775,0.626815353000749,40.7106596417877));
#58189=CARTESIAN_POINT('Ctrl Pts',(22.7330915324132,0.752538147919828,38.6844033171128));
#58190=CARTESIAN_POINT('Ctrl Pts',(21.9779124571561,0.878260942838908,36.1253306736311));
#58191=CARTESIAN_POINT('Ctrl Pts',(19.4201843152843,1.00398373775798,35.3659513962466));
#58192=CARTESIAN_POINT('Ctrl Pts',(17.390869413503,1.12970653267706,37.0981277714779));
#58193=CARTESIAN_POINT('Ctrl Pts',(17.7393253384899,1.25542932759614,39.7433712754338));
#58194=CARTESIAN_POINT('Ctrl Pts',(20.148002280105,1.38115212251522,40.8909464790416));
#58195=CARTESIAN_POINT('Ctrl Pts',(22.4217990278434,1.5068749174343,39.4950599053239));
#58196=CARTESIAN_POINT('Ctrl Pts',(22.488540977682,1.63259771235338,36.8278104747239));
#58197=CARTESIAN_POINT('Ctrl Pts',(20.2874031381624,1.75832050727246,35.31994644143));
#58198=CARTESIAN_POINT('Ctrl Pts',(17.8243466987466,1.88404330219154,36.3456244965799));
#58199=CARTESIAN_POINT('Ctrl Pts',(17.3440259713813,2.00976609711062,38.9701163209587));
#58200=CARTESIAN_POINT('Ctrl Pts',(19.2841712887778,2.13548889202969,40.8016456505112));
#58201=CARTESIAN_POINT('Ctrl Pts',(21.87667199869,2.26121168694878,40.171087277866));
#58202=CARTESIAN_POINT('Ctrl Pts',(22.7589072219985,2.38693448186786,37.6530870516505));
#58203=CARTESIAN_POINT('Ctrl Pts',(21.1268704479201,2.51265727678694,35.5423715711052));
#58204=CARTESIAN_POINT('Ctrl Pts',(18.467884028376,2.63838007170603,35.7624968697667));
#58205=CARTESIAN_POINT('Ctrl Pts',(17.2051592290664,2.7641028666251,38.1128564263638));
#58206=CARTESIAN_POINT('Ctrl Pts',(18.489453703936,2.88982566154418,40.4514995436837));
#58207=CARTESIAN_POINT('Ctrl Pts',(21.1503527309155,3.01554845646325,40.6471530808971));
#58208=CARTESIAN_POINT('Ctrl Pts',(22.7629020249366,3.14127125138234,38.5215123030072));
#58209=CARTESIAN_POINT('Ctrl Pts',(21.8575387491212,3.26699404630141,36.0117351662413));
#58210=CARTESIAN_POINT('Ctrl Pts',(19.2593466568257,3.3927168412205,35.4050542034166));
#58211=CARTESIAN_POINT('Ctrl Pts',(17.3361333895618,3.51843963613957,37.2543553330546));
#58212=CARTESIAN_POINT('Ctrl Pts',(17.8405788528435,3.64416243105865,39.8743169192987));
#58213=CARTESIAN_POINT('Ctrl Pts',(20.3129672980339,3.76988522597773,40.8772921508858));
#58214=CARTESIAN_POINT('Ctrl Pts',(22.5001395877116,3.89560802089681,39.3492406745362));
#58215=CARTESIAN_POINT('Ctrl Pts',(22.408862320693,4.02133081581589,36.6827200202844));
#58216=CARTESIAN_POINT('Ctrl Pts',(20.1223191118479,4.14705361073498,35.3078076255658));
#58217=CARTESIAN_POINT('Ctrl Pts',(17.7243029566375,4.27277640565405,36.477500943669));
#58218=CARTESIAN_POINT('Ctrl Pts',(17.4001953724141,4.39849920057313,39.1258246045731));
#58219=CARTESIAN_POINT('Ctrl Pts',(19.4453649798832,4.52422199549221,40.8392846174551));
#58220=CARTESIAN_POINT('Ctrl Pts',(21.9959895315176,4.6499447904113,40.0563552875276));
#58221=CARTESIAN_POINT('Ctrl Pts',(22.727611062039,4.77566758533037,37.490542769993));
#58222=CARTESIAN_POINT('Ctrl Pts',(20.9734816986179,4.90139038024944,35.4801462629716));
#58223=CARTESIAN_POINT('Ctrl Pts',(18.3321902920983,5.02711317516853,35.8572982812701));
#58224=CARTESIAN_POINT('Ctrl Pts',(17.2108221363827,5.1528359700876,38.2782892763806));
#58225=CARTESIAN_POINT('Ctrl Pts',(18.6313124825418,5.27855876500669,40.5368000944927));
#58226=CARTESIAN_POINT('Ctrl Pts',(21.2991273711915,5.40428155992577,40.5745844690344));
#58227=CARTESIAN_POINT('Ctrl Pts',(22.7830098916132,5.53000435484485,38.3572084060612));
#58228=CARTESIAN_POINT('Ctrl Pts',(21.7306549615396,5.65572714976392,35.9054308794062));
#58229=CARTESIAN_POINT('Ctrl Pts',(19.1011040823716,5.78144994468301,35.4536276999946));
#58230=CARTESIAN_POINT('Ctrl Pts',(17.2907430656818,5.90717273960207,37.4135401797522));
#58231=CARTESIAN_POINT('Ctrl Pts',(17.9494062952009,6.03289553452117,39.9990433588531));
#58232=CARTESIAN_POINT('Ctrl Pts',(20.4768349091098,6.15861832944025,40.8538933694716));
#58233=CARTESIAN_POINT('Ctrl Pts',(22.5697100714367,6.28434112435933,39.1990406588125));
#58234=CARTESIAN_POINT('Ctrl Pts',(22.3207340819822,6.4100639192784,36.5426003911355));
#58235=CARTESIAN_POINT('Ctrl Pts',(19.9568059649405,6.53578671419749,35.3054634559017));
#58236=CARTESIAN_POINT('Ctrl Pts',(17.6322418220212,6.66150950911657,36.6150685431375));
#58237=CARTESIAN_POINT('Ctrl Pts',(17.4654842261801,6.78723230403565,39.2779346387738));
#58238=CARTESIAN_POINT('Ctrl Pts',(19.60850420023,6.91295509895471,40.8673148103763));
#58239=CARTESIAN_POINT('Ctrl Pts',(22.1083056259307,7.03867789387381,39.9347609132075));
#58240=CARTESIAN_POINT('Ctrl Pts',(22.6867471234151,7.16440068879287,37.3301363005141));
#58241=CARTESIAN_POINT('Ctrl Pts',(20.8166782167678,7.29012348371197,35.4271107559007));
#58242=CARTESIAN_POINT('Ctrl Pts',(18.2023468176975,7.41584627863103,35.9599665289712));
#58243=CARTESIAN_POINT('Ctrl Pts',(17.2262687851341,7.54156907355013,38.4430967336541));
#58244=CARTESIAN_POINT('Ctrl Pts',(18.7779722764348,7.66729186846919,40.6135529562361));
#58245=CARTESIAN_POINT('Ctrl Pts',(21.4433449959297,7.79301466338828,40.4933356312248));
#58246=CARTESIAN_POINT('Ctrl Pts',(22.7933556523239,7.91873745830735,38.1920022858178));
#58247=CARTESIAN_POINT('Ctrl Pts',(21.5977004670959,8.04446025322644,35.8068245949324));
#58248=CARTESIAN_POINT('Ctrl Pts',(18.9460146110701,8.17018304814552,35.5114840118539));
#58249=CARTESIAN_POINT('Ctrl Pts',(17.2548561407841,8.2959058430646,37.5751329566698));
#58250=CARTESIAN_POINT('Ctrl Pts',(18.0654267098815,8.42162863798366,40.1171084269631));
#58251=CARTESIAN_POINT('Ctrl Pts',(20.6390299020081,8.54735143290277,40.8208346155739));
#58252=CARTESIAN_POINT('Ctrl Pts',(22.6302666518364,8.67307422782184,39.0449854820062));
#58253=CARTESIAN_POINT('Ctrl Pts',(22.2244652857459,8.79879702274091,36.4079437321775));
#58254=CARTESIAN_POINT('Ctrl Pts',(19.7914443319572,8.92451981766,35.3129218248688));
#58255=CARTESIAN_POINT('Ctrl Pts',(17.5484861937545,9.05024261257907,36.7578449125555));
#58256=CARTESIAN_POINT('Ctrl Pts',(17.5396635304358,9.17596540749815,39.4259127714512));
#58257=CARTESIAN_POINT('Ctrl Pts',(19.7730166903984,9.30168820241722,40.8856379517316));
#58258=CARTESIAN_POINT('Ctrl Pts',(22.2132263089687,9.42741099733632,39.8067306542786));
#58259=CARTESIAN_POINT('Ctrl Pts',(22.6364587446177,9.55313379225539,37.1724303212727));
#58260=CARTESIAN_POINT('Ctrl Pts',(20.657010031006,9.67885658717447,35.3834510790116));
#58261=CARTESIAN_POINT('Ctrl Pts',(18.0788090632215,9.80457938209355,36.0701414814314));
#58262=CARTESIAN_POINT('Ctrl Pts',(17.2514449926014,9.93030217701264,38.606700692983));
#58263=CARTESIAN_POINT('Ctrl Pts',(18.9289186394175,10.0560249719317,40.6814888998364));
#58264=CARTESIAN_POINT('Ctrl Pts',(21.5824997256729,10.1817477668508,40.4036915677257));
#58265=CARTESIAN_POINT('Ctrl Pts',(22.7939030166767,10.3074705617699,38.0264734444553));
#58266=CARTESIAN_POINT('Ctrl Pts',(21.4591416370836,10.433193356689,35.7162621990046));
#58267=CARTESIAN_POINT('Ctrl Pts',(18.7946222581744,10.558916151608,35.5784201935143));
#58268=CARTESIAN_POINT('Ctrl Pts',(17.2285984972737,10.6846389465271,37.7385668365352));
#58269=CARTESIAN_POINT('Ctrl Pts',(18.1882331261458,10.8103617414462,40.228097980773));
#58270=CARTESIAN_POINT('Ctrl Pts',(20.7989833370656,10.9360845363653,40.7782318510646));
#58271=CARTESIAN_POINT('Ctrl Pts',(22.6815969114991,11.0618073312843,38.8876155313373));
#58272=CARTESIAN_POINT('Ctrl Pts',(22.1203936189598,11.1875301262034,36.2792223854518));
#58273=CARTESIAN_POINT('Ctrl Pts',(19.6268142603477,11.3132529211225,35.3301565703662));
#58274=CARTESIAN_POINT('Ctrl Pts',(17.4733298657346,11.4389757160416,36.9053292279559));
#58275=CARTESIAN_POINT('Ctrl Pts',(17.6224730826451,11.5646985109607,39.5692399321481));
#58276=CARTESIAN_POINT('Ctrl Pts',(19.9383253815204,11.6904213058798,40.8941897685019));
#58277=CARTESIAN_POINT('Ctrl Pts',(22.3103835449902,11.8161441007988,39.6727136090224));
#58278=CARTESIAN_POINT('Ctrl Pts',(22.5769223247629,11.9418668957179,37.0179780255909));
#58279=CARTESIAN_POINT('Ctrl Pts',(20.4950372175861,12.067589690637,35.3493203795843));
#58280=CARTESIAN_POINT('Ctrl Pts',(17.9620103683644,12.1933124855561,36.1874366723398));
#58281=CARTESIAN_POINT('Ctrl Pts',(17.286262446915,12.3190352804751,38.7685272723994));
#58282=CARTESIAN_POINT('Ctrl Pts',(19.0836220892193,12.4447580753942,40.7403696229124));
#58283=CARTESIAN_POINT('Ctrl Pts',(21.7161034402651,12.5704808703133,40.3059667275995));
#58284=CARTESIAN_POINT('Ctrl Pts',(22.7846500646538,12.6962036652324,37.8612025159488));
#58285=CARTESIAN_POINT('Ctrl Pts',(21.3154645013911,12.8219264601515,35.6340613619667));
#58286=CARTESIAN_POINT('Ctrl Pts',(18.6474580703767,12.9476492550705,35.6542014495105));
#58287=CARTESIAN_POINT('Ctrl Pts',(17.212062240429,13.0733720499896,37.9032685339766));
#58288=CARTESIAN_POINT('Ctrl Pts',(18.3173947696519,13.1990948449087,40.331622696553));
#58289=CARTESIAN_POINT('Ctrl Pts',(20.956134137445,13.3248176398278,40.7262345158379));
#58290=CARTESIAN_POINT('Ctrl Pts',(22.7235207966499,13.4505404347469,38.7274828214233));
#58291=CARTESIAN_POINT('Ctrl Pts',(22.0088841391277,13.5762632296659,36.1568878734034));
#58292=CARTESIAN_POINT('Ctrl Pts',(19.4634932314263,13.701986024585,35.3571072371964));
#58293=CARTESIAN_POINT('Ctrl Pts',(17.4070364676536,13.8277088195041,37.0570041510691));
#58294=CARTESIAN_POINT('Ctrl Pts',(17.7136224075105,13.9534316144232,39.707413364859));
#58295=CARTESIAN_POINT('Ctrl Pts',(20.1038504118531,14.0791544093423,40.8929402630424));
#58296=CARTESIAN_POINT('Ctrl Pts',(22.3994365305938,14.2048772042613,39.5331798758766));
#58297=CARTESIAN_POINT('Ctrl Pts',(22.5083467027926,14.3305999991804,36.8673211936783));
#58298=CARTESIAN_POINT('Ctrl Pts',(20.3313279368224,14.4563227940995,35.3248383796171));
#58299=CARTESIAN_POINT('Ctrl Pts',(17.8523604338763,14.5820455890186,36.3114406593615));
#58300=CARTESIAN_POINT('Ctrl Pts',(17.3305990171115,14.7077683839377,38.9280088245419));
#58301=CARTESIAN_POINT('Ctrl Pts',(19.2415399646442,14.8334911788567,40.7899885865433));
#58302=CARTESIAN_POINT('Ctrl Pts',(21.8436874911296,14.9592139737758,40.2005039052613));
#58303=CARTESIAN_POINT('Ctrl Pts',(22.7656292533077,15.0849367686949,37.6967692295793));
#58304=CARTESIAN_POINT('Ctrl Pts',(21.1671730436487,15.210659563614,35.5605104238951));
#58305=CARTESIAN_POINT('Ctrl Pts',(18.5050382630183,15.3363823585331,35.7385619580589));
#58306=CARTESIAN_POINT('Ctrl Pts',(17.2053053753228,15.4621051534521,38.0686603164341));
#58307=CARTESIAN_POINT('Ctrl Pts',(18.452458573503,15.5878279483712,40.4273194353679));
#58308=CARTESIAN_POINT('Ctrl Pts',(21.1099310572534,15.7135507432903,40.6650250036032));
#58309=CARTESIAN_POINT('Ctrl Pts',(22.7558912487344,15.8392735382094,38.5651490579532));
#58310=CARTESIAN_POINT('Ctrl Pts',(21.8903279937497,15.9649963331285,36.0413693150515));
#58311=CARTESIAN_POINT('Ctrl Pts',(19.3020541347117,16.0907191280475,35.3936792891285));
#58312=CARTESIAN_POINT('Ctrl Pts',(17.3498385402515,16.2164419229666,37.2123376440172));
#58313=CARTESIAN_POINT('Ctrl Pts',(17.8127917758874,16.3421647178857,39.8399483915737));
#58314=CARTESIAN_POINT('Ctrl Pts',(20.2690111607896,16.4678875128048,40.8818938183072));
#58315=CARTESIAN_POINT('Ctrl Pts',(22.4800728900715,16.5936103077239,39.3886189044468));
#58316=CARTESIAN_POINT('Ctrl Pts',(22.4309724249204,16.7193331026429,36.7209882922026));
#58317=CARTESIAN_POINT('Ctrl Pts',(20.1664564401246,16.845055897562,35.3100909558722));
#58318=CARTESIAN_POINT('Ctrl Pts',(17.7502438844354,16.9707786924811,36.4417184673749));
#58319=CARTESIAN_POINT('Ctrl Pts',(17.3842991815377,17.0965014874002,39.0845859278207));
#58320=CARTESIAN_POINT('Ctrl Pts',(19.4021183290917,17.2222242823192,40.8301717397549));
#58321=CARTESIAN_POINT('Ctrl Pts',(21.9648043451713,17.3479470772383,40.0876730380422));
#58322=CARTESIAN_POINT('Ctrl Pts',(22.7369073029115,17.4736698721574,37.5337503763873));
#58323=CARTESIAN_POINT('Ctrl Pts',(21.0147874333784,17.5993926670765,35.4958673831745));
#58324=CARTESIAN_POINT('Ctrl Pts',(18.3678624093392,17.7251154619956,35.8312058034916));
#58325=CARTESIAN_POINT('Ctrl Pts',(17.2083516033483,17.8508382569146,38.2341620307038));
#58326=CARTESIAN_POINT('Ctrl Pts',(18.5929507675084,17.9765610518337,40.5148525168716));
#58327=CARTESIAN_POINT('Ctrl Pts',(21.2598346151463,18.1022838467528,40.5948180221049));
#58328=CARTESIAN_POINT('Ctrl Pts',(22.7785947203223,18.2280066416719,38.4011836673442));
#58329=CARTESIAN_POINT('Ctrl Pts',(21.7651410481622,18.353729436591,35.9330719207845));
#58330=CARTESIAN_POINT('Ctrl Pts',(19.143063258592,18.47945223151,35.4397444404324));
#58331=CARTESIAN_POINT('Ctrl Pts',(17.301936719196,18.6051750264291,37.3707848357136));
#58332=CARTESIAN_POINT('Ctrl Pts',(17.9196333271384,18.7308978213482,39.9663801121273));
#58333=CARTESIAN_POINT('Ctrl Pts',(20.4332282839357,18.8566206162673,40.8610891830162));
#58334=CARTESIAN_POINT('Ctrl Pts',(22.5520097742367,18.9823434111863,39.2395377775908));
#58335=CARTESIAN_POINT('Ctrl Pts',(22.3450708948629,19.1080662061055,36.5794926225918));
#58336=CARTESIAN_POINT('Ctrl Pts',(20.0010010672759,19.2337890010245,35.3051298347038));
#58337=CARTESIAN_POINT('Ctrl Pts',(17.6560188969823,19.3595117959436,36.5778131218862));
#58338=CARTESIAN_POINT('Ctrl Pts',(17.4471746169796,19.4852345908627,39.237709333944));
#58339=CARTESIAN_POINT('Ctrl Pts',(19.5647938291461,19.6109573857818,40.8607781586984));
#58340=CARTESIAN_POINT('Ctrl Pts',(22.0790293183196,19.7366801807008,39.9678698530205));
#58341=CARTESIAN_POINT('Ctrl Pts',(22.6985846456872,19.8624029756199,37.372717893521));
#58342=CARTESIAN_POINT('Ctrl Pts',(20.8588428161005,19.988125770539,35.4403587830203));
#58343=CARTESIAN_POINT('Ctrl Pts',(18.2364104968719,20.1138485654581,35.9318084182521));
#58344=CARTESIAN_POINT('Ctrl Pts',(17.2211925474339,20.2395713603771,38.3991923551073));
#58345=CARTESIAN_POINT('Ctrl Pts',(18.7383740669321,20.3652941552962,40.5939164138209));
#58346=CARTESIAN_POINT('Ctrl Pts',(21.4053276546846,20.4910169502153,40.5158569002854));
#58347=CARTESIAN_POINT('Ctrl Pts',(22.7915347766057,20.6167397451344,38.2361674958629));
#58348=CARTESIAN_POINT('Ctrl Pts',(21.6337949755707,20.7424625400534,35.8323645322771));
#58349=CARTESIAN_POINT('Ctrl Pts',(18.9870152307706,20.8681853349726,35.4951624966401));
#58350=CARTESIAN_POINT('Ctrl Pts',(17.2636212567748,20.9939081298916,37.5317484821045));
#58351=CARTESIAN_POINT('Ctrl Pts',(18.0335354157021,21.1196309248107,40.086345359573));
#58352=CARTESIAN_POINT('Ctrl Pts',(20.5963850122518,21.2453537197298,40.8304436732054));
#58353=CARTESIAN_POINT('Ctrl Pts',(22.6141023677897,21.3710765146489,39.0867611723361));
#58354=CARTESIAN_POINT('Ctrl Pts',(22.2526978385088,21.4967993095679,36.4427448448181));
#58355=CARTESIAN_POINT('Ctrl Pts',(19.8316106131819,21.6225368858548,35.3109838910756));
#58356=CARTESIAN_POINT('Ctrl Pts',(18.3297609408629,21.7063668638354,36.2486441106533));
#58357=CARTESIAN_POINT('Ctrl Pts',(17.9420413053583,21.7482892435095,36.9315928900642));
#58358=CARTESIAN_POINT('Ctrl Pts',(21.3897090577788,-0.0427385219042173,
39.8306710798006));
#58359=CARTESIAN_POINT('Ctrl Pts',(21.9640764188518,-0.00081427231963721,
39.3694899961113));
#58360=CARTESIAN_POINT('Ctrl Pts',(22.6075578816433,0.0830175755713031,
37.8385802957988));
#58361=CARTESIAN_POINT('Ctrl Pts',(21.1973412527138,0.208757021768603,35.7662370196645));
#58362=CARTESIAN_POINT('Ctrl Pts',(18.6951753347191,0.334479816687684,35.8272771783663));
#58363=CARTESIAN_POINT('Ctrl Pts',(17.3826477749713,0.460202611606761,37.9564061107638));
#58364=CARTESIAN_POINT('Ctrl Pts',(18.4551222095092,0.585925406525842,40.2179874232035));
#58365=CARTESIAN_POINT('Ctrl Pts',(20.9356263448805,0.71164820144492,40.5485657675615));
#58366=CARTESIAN_POINT('Ctrl Pts',(22.5633959550915,0.837370996364001,38.648118159038));
#58367=CARTESIAN_POINT('Ctrl Pts',(21.855105375019,0.963093791283079,36.2479363922409));
#58368=CARTESIAN_POINT('Ctrl Pts',(19.456184630748,1.08881658620216,35.5357063974009));
#58369=CARTESIAN_POINT('Ctrl Pts',(17.5528683498476,1.21453938112124,37.1603332571726));
#58370=CARTESIAN_POINT('Ctrl Pts',(17.8796889111226,1.34026217604032,39.6413356011684));
#58371=CARTESIAN_POINT('Ctrl Pts',(20.1388129309487,1.46598497095939,40.7176587320276));
#58372=CARTESIAN_POINT('Ctrl Pts',(22.2714313656875,1.59170776587848,39.4084416954231));
#58373=CARTESIAN_POINT('Ctrl Pts',(22.3340293585545,1.71743056079755,36.906799756054));
#58374=CARTESIAN_POINT('Ctrl Pts',(20.2695584956116,1.84315335571663,35.4925578552857));
#58375=CARTESIAN_POINT('Ctrl Pts',(17.9594313596992,1.96887615063571,36.4545523390475));
#58376=CARTESIAN_POINT('Ctrl Pts',(17.5089333814672,2.09459894555479,38.9160914594892));
#58377=CARTESIAN_POINT('Ctrl Pts',(19.3286165497482,2.22032174047387,40.633902524112));
#58378=CARTESIAN_POINT('Ctrl Pts',(21.7601508597217,2.34604453539295,40.0424950418823));
#58379=CARTESIAN_POINT('Ctrl Pts',(22.5876087681188,2.47176733031203,37.6808355371598));
#58380=CARTESIAN_POINT('Ctrl Pts',(21.0569039177257,2.59749012523111,35.701172777603));
#58381=CARTESIAN_POINT('Ctrl Pts',(18.5630119453321,2.72321292015019,35.9076306636672));
#58382=CARTESIAN_POINT('Ctrl Pts',(17.3786887697062,2.84893571506927,38.1120581806159));
#58383=CARTESIAN_POINT('Ctrl Pts',(18.5832423761198,2.97465850998835,40.3054967231031));
#58384=CARTESIAN_POINT('Ctrl Pts',(21.0789282036058,3.10038130490743,40.4890022808));
#58385=CARTESIAN_POINT('Ctrl Pts',(22.5913555367767,3.22610409982651,38.4953409242742));
#58386=CARTESIAN_POINT('Ctrl Pts',(21.7422055790859,3.35182689474558,36.1413939436233));
#58387=CARTESIAN_POINT('Ctrl Pts',(19.3053332603386,3.47754968966468,35.5723813409743));
#58388=CARTESIAN_POINT('Ctrl Pts',(17.501530844058,3.60327248458374,37.306860768114));
#58389=CARTESIAN_POINT('Ctrl Pts',(17.9746556716773,3.72899527950283,39.7641509294657));
#58390=CARTESIAN_POINT('Ctrl Pts',(20.293535396214,3.8547180744219,40.7048521907358));
#58391=CARTESIAN_POINT('Ctrl Pts',(22.3449078196972,3.98044086934098,39.2716762699177));
#58392=CARTESIAN_POINT('Ctrl Pts',(22.259297888858,4.10616366426007,36.7707178577268));
#58393=CARTESIAN_POINT('Ctrl Pts',(20.1147244111011,4.23188645917914,35.4811727292785));
#58394=CARTESIAN_POINT('Ctrl Pts',(17.865599257549,4.35760925409822,36.5782406777038));
#58395=CARTESIAN_POINT('Ctrl Pts',(17.5616152670535,4.48333204901731,39.0621319340425));
#58396=CARTESIAN_POINT('Ctrl Pts',(19.479801847008,4.60905484393638,40.6692045161871));
#58397=CARTESIAN_POINT('Ctrl Pts',(21.8720600575641,4.73477763885547,39.9348866736791));
#58398=CARTESIAN_POINT('Ctrl Pts',(22.55825576296,4.86050043377454,37.5283835064896));
#58399=CARTESIAN_POINT('Ctrl Pts',(20.9130389593609,4.98622322869362,35.6428109915879));
#58400=CARTESIAN_POINT('Ctrl Pts',(18.4357433300734,5.1119460236127,35.9965459275369));
#58401=CARTESIAN_POINT('Ctrl Pts',(17.3840000714084,5.23766881853178,38.2672194306302));
#58402=CARTESIAN_POINT('Ctrl Pts',(18.7162932509112,5.36339161345086,40.3855010275026));
#58403=CARTESIAN_POINT('Ctrl Pts',(21.2184655394692,5.48911440836994,40.4209393989282));
#58404=CARTESIAN_POINT('Ctrl Pts',(22.6102149212844,5.61483720328902,38.3412385314921));
#58405=CARTESIAN_POINT('Ctrl Pts',(21.6231999095005,5.7405599982081,36.0416900092141));
#58406=CARTESIAN_POINT('Ctrl Pts',(19.1569158471387,5.86628279312718,35.6179389460439));
#58407=CARTESIAN_POINT('Ctrl Pts',(17.4589587709116,5.99200558804625,37.4561619485894));
#58408=CARTESIAN_POINT('Ctrl Pts',(18.0767261007989,6.11772838296534,39.8811331991244));
#58409=CARTESIAN_POINT('Ctrl Pts',(20.4472285917842,6.24345117788442,40.6829062218869));
#58410=CARTESIAN_POINT('Ctrl Pts',(22.4101587249301,6.3691739728035,39.1308020590856));
#58411=CARTESIAN_POINT('Ctrl Pts',(22.1766414655508,6.49489676772258,36.6392981499235));
#58412=CARTESIAN_POINT('Ctrl Pts',(19.9594878497692,6.62061956264165,35.4789741073284));
#58413=CARTESIAN_POINT('Ctrl Pts',(17.7792541288559,6.74634235756073,36.7072668094111));
#58414=CARTESIAN_POINT('Ctrl Pts',(17.6228503854794,6.87206515247981,39.2047975717553));
#58415=CARTESIAN_POINT('Ctrl Pts',(19.6328118770762,6.99778794739889,40.6954943357201));
#58416=CARTESIAN_POINT('Ctrl Pts',(21.977402530985,7.12351074231797,39.8208420017032));
#58417=CARTESIAN_POINT('Ctrl Pts',(22.519929035247,7.24923353723705,37.3779365528634));
#58418=CARTESIAN_POINT('Ctrl Pts',(20.7659712865986,7.37495633215614,35.5930684188678));
#58419=CARTESIAN_POINT('Ctrl Pts',(18.3139617383752,7.5006791270752,36.0928395817203));
#58420=CARTESIAN_POINT('Ctrl Pts',(17.3984876494714,7.6264019219943,38.4217941180613));
#58421=CARTESIAN_POINT('Ctrl Pts',(18.8538470495971,7.75212471691336,40.4574883623582));
#58422=CARTESIAN_POINT('Ctrl Pts',(21.3537288014283,7.87784751183246,40.3447352397454));
#58423=CARTESIAN_POINT('Ctrl Pts',(22.6199183215705,8.00357030675152,38.186289933772));
#58424=CARTESIAN_POINT('Ctrl Pts',(21.4985004586309,8.12929310167061,35.9492061140465));
#58425=CARTESIAN_POINT('Ctrl Pts',(19.0114557633118,8.25501589658968,35.6722030034448));
#58426=CARTESIAN_POINT('Ctrl Pts',(17.4253000379226,8.38073869150878,37.6077215527263));
#58427=CARTESIAN_POINT('Ctrl Pts',(18.1855428960556,8.50646148642784,39.9918676968322));
#58428=CARTESIAN_POINT('Ctrl Pts',(20.599353020769,8.63218428134693,40.6519000609089));
#58429=CARTESIAN_POINT('Ctrl Pts',(22.4669553932489,8.75790707626599,38.9863120511942));
#58430=CARTESIAN_POINT('Ctrl Pts',(22.0863499257514,8.8836298711851,36.5130022206416));
#58431=CARTESIAN_POINT('Ctrl Pts',(19.8043933949771,9.00935266610415,35.4859693918313));
#58432=CARTESIAN_POINT('Ctrl Pts',(17.7006988239315,9.13507546102325,36.8411783024981));
#58433=CARTESIAN_POINT('Ctrl Pts',(17.6924239530769,9.26079825594232,39.3435878545717));
#58434=CARTESIAN_POINT('Ctrl Pts',(19.7871099116859,9.3865210508614,40.7126798071462));
#58435=CARTESIAN_POINT('Ctrl Pts',(22.0758087685058,9.51224384578049,39.7007610443055));
#58436=CARTESIAN_POINT('Ctrl Pts',(22.4727630236925,9.63796664069955,37.2300224180872));
#58437=CARTESIAN_POINT('Ctrl Pts',(20.6162167772143,9.76368943561865,35.5521195381551));
#58438=CARTESIAN_POINT('Ctrl Pts',(18.1980943492413,9.88941223053771,36.1961738550658));
#58439=CARTESIAN_POINT('Ctrl Pts',(17.4221006853397,10.0151350254568,38.5752400318213));
#58440=CARTESIAN_POINT('Ctrl Pts',(18.9954212675538,10.1408578203759,40.5212062148211));
#58441=CARTESIAN_POINT('Ctrl Pts',(21.484243519697,10.266580615295,40.2606571080598));
#58442=CARTESIAN_POINT('Ctrl Pts',(22.6204317004865,10.3923034102141,38.0310386524419));
#58443=CARTESIAN_POINT('Ctrl Pts',(21.3685446411314,10.5180262051331,35.8642666684951));
#58444=CARTESIAN_POINT('Ctrl Pts',(18.8694632466171,10.6437490000522,35.7349831684274));
#58445=CARTESIAN_POINT('Ctrl Pts',(17.4006727115538,10.7694717949713,37.7610079471273));
#58446=CARTESIAN_POINT('Ctrl Pts',(18.3007243552118,10.8951945898904,40.0959659935483));
#58447=CARTESIAN_POINT('Ctrl Pts',(20.7493750685367,11.0209173848094,40.6119424696889));
#58448=CARTESIAN_POINT('Ctrl Pts',(22.5150985960771,11.1466401797285,38.8387130812318));
#58449=CARTESIAN_POINT('Ctrl Pts',(21.9887399897083,11.2723629746476,36.3922730845633));
#58450=CARTESIAN_POINT('Ctrl Pts',(19.6499850794686,11.3980857695667,35.5021340450715));
#58451=CARTESIAN_POINT('Ctrl Pts',(17.6302088952332,11.5238085644857,36.9795054287771));
#58452=CARTESIAN_POINT('Ctrl Pts',(17.7700919230879,11.6495313594049,39.4780159407255));
#58453=CARTESIAN_POINT('Ctrl Pts',(19.9421547117366,11.7752541543239,40.7207006481087));
#58454=CARTESIAN_POINT('Ctrl Pts',(22.1669335855388,11.900976949243,39.5750650155964));
#58455=CARTESIAN_POINT('Ctrl Pts',(22.4169231749254,12.0266997441621,37.0851599481297));
#58456=CARTESIAN_POINT('Ctrl Pts',(20.4643007327528,12.1524225390811,35.5201079879311));
#58457=CARTESIAN_POINT('Ctrl Pts',(18.0885475966331,12.2781453340003,36.3061862766624));
#58458=CARTESIAN_POINT('Ctrl Pts',(17.4547563503607,12.4038681289193,38.7270189218375));
#58459=CARTESIAN_POINT('Ctrl Pts',(19.1405192976627,12.5295909238384,40.5764310785245));
#58460=CARTESIAN_POINT('Ctrl Pts',(21.6095518811291,12.6553137187575,40.1689999290297));
#58461=CARTESIAN_POINT('Ctrl Pts',(22.6117532572266,12.7810365136766,37.8760292703545));
#58462=CARTESIAN_POINT('Ctrl Pts',(21.2337883096637,12.9067593085956,35.787169618993));
#58463=CARTESIAN_POINT('Ctrl Pts',(18.7314363714608,13.0324821035147,35.8060592237987));
#58464=CARTESIAN_POINT('Ctrl Pts',(17.3851631783365,13.1582048984338,37.9154834412742));
#58465=CARTESIAN_POINT('Ctrl Pts',(18.4218664503776,13.2839276933529,40.1930629383581));
#58466=CARTESIAN_POINT('Ctrl Pts',(20.8967684950848,13.409650488272,40.5631736095118));
#58467=CARTESIAN_POINT('Ctrl Pts',(22.5544194590421,13.535373283191,38.6885228896471));
#58468=CARTESIAN_POINT('Ctrl Pts',(21.8841540487817,13.6610960781101,36.2775342294486));
#58469=CARTESIAN_POINT('Ctrl Pts',(19.4968045291821,13.7868188730292,35.5274113654686));
#58470=CARTESIAN_POINT('Ctrl Pts',(17.5680316038858,13.9125416679483,37.1217629711195));
#58471=CARTESIAN_POINT('Ctrl Pts',(17.855581855605,14.0382644628674,39.6076102899493));
#58472=CARTESIAN_POINT('Ctrl Pts',(20.097402418661,14.1639872577864,40.7195287234941));
#58473=CARTESIAN_POINT('Ctrl Pts',(22.2504573389066,14.2897100527055,39.4441948259583));
#58474=CARTESIAN_POINT('Ctrl Pts',(22.3526053612365,14.4154328476246,36.9438572844788));
#58475=CARTESIAN_POINT('Ctrl Pts',(20.3107560368861,14.5411556425437,35.4971460567465));
#58476=CARTESIAN_POINT('Ctrl Pts',(17.9857057432925,14.6668784374627,36.4224909503174));
#58477=CARTESIAN_POINT('Ctrl Pts',(17.4963400965896,14.7926012323818,38.876598385542));
#58478=CARTESIAN_POINT('Ctrl Pts',(19.2886321721494,14.9183240273009,40.6229692383917));
#58479=CARTESIAN_POINT('Ctrl Pts',(21.7292143351823,15.04404682222,40.070085213226));
#58480=CARTESIAN_POINT('Ctrl Pts',(22.5939134336097,15.1697696171391,37.72180552184));
#58481=CARTESIAN_POINT('Ctrl Pts',(21.0947041558975,15.2954924120581,35.7181854028005));
#58482=CARTESIAN_POINT('Ctrl Pts',(18.597859301766,15.4212152069772,35.8851818524476));
#58483=CARTESIAN_POINT('Ctrl Pts',(17.3788258418525,15.5469380018963,38.0706061735827));
#58484=CARTESIAN_POINT('Ctrl Pts',(18.5485442452357,15.6726607968154,40.2828179393466));
#58485=CARTESIAN_POINT('Ctrl Pts',(21.0410162809591,15.7983835917345,40.5057645494));
#58486=CARTESIAN_POINT('Ctrl Pts',(22.5847800543438,15.9241063866536,38.5362683062499));
#58487=CARTESIAN_POINT('Ctrl Pts',(21.7729589644207,16.0498291815726,36.1691881306424));
#58488=CARTESIAN_POINT('Ctrl Pts',(19.3453890633611,16.1755519764917,35.5617126864745));
#58489=CARTESIAN_POINT('Ctrl Pts',(17.5143850523512,16.3012747714108,37.2674519254743));
#58490=CARTESIAN_POINT('Ctrl Pts',(17.9485938732237,16.4269975663299,39.7319163175226));
#58491=CARTESIAN_POINT('Ctrl Pts',(20.2523084621442,16.5527203612489,40.7091681441222));
#58492=CARTESIAN_POINT('Ctrl Pts',(22.3260870480718,16.678443156168,39.3086095354431));
#58493=CARTESIAN_POINT('Ctrl Pts',(22.2800351935076,16.8041659510871,36.8066100817083));
#58494=CARTESIAN_POINT('Ctrl Pts',(20.1561212861896,16.9298887460062,35.4833142893404));
#58495=CARTESIAN_POINT('Ctrl Pts',(17.8899295328436,17.0556115409253,36.5446799081842));
#58496=CARTESIAN_POINT('Ctrl Pts',(17.5467060585947,17.1813343358443,39.0234537354066));
#58497=CARTESIAN_POINT('Ctrl Pts',(19.439240347916,17.3070571307634,40.6606574501416));
#58498=CARTESIAN_POINT('Ctrl Pts',(21.8428111357511,17.4327799256825,39.9642599288516));
#58499=CARTESIAN_POINT('Ctrl Pts',(22.5669748072978,17.5585027206016,37.5689083854212));
#58500=CARTESIAN_POINT('Ctrl Pts',(20.9517800524239,17.6842255155207,35.6575559993785));
#58501=CARTESIAN_POINT('Ctrl Pts',(18.4692005926496,17.8099483104397,35.9720735118851));
#58502=CARTESIAN_POINT('Ctrl Pts',(17.3816829318936,17.9356711053588,38.2258320121205));
#58503=CARTESIAN_POINT('Ctrl Pts',(18.6803133856264,18.0613939002779,40.3649161583056));
#58504=CARTESIAN_POINT('Ctrl Pts',(21.181612440802,18.187116695197,40.439916666057));
#58505=CARTESIAN_POINT('Ctrl Pts',(22.6060738846253,18.3128394901161,38.3824834022036));
#58506=CARTESIAN_POINT('Ctrl Pts',(21.6555447811986,18.4385622850351,36.0676148393279));
#58507=CARTESIAN_POINT('Ctrl Pts',(19.1962698099778,18.5642850799542,35.604917687523));
#58508=CARTESIAN_POINT('Ctrl Pts',(17.4694574189812,18.6900078748733,37.416061251387));
#58509=CARTESIAN_POINT('Ctrl Pts',(18.0488017137092,18.8157306697924,39.8504979885785));
#58510=CARTESIAN_POINT('Ctrl Pts',(20.4063294688456,18.9414534647115,40.6896552528342));
#58511=CARTESIAN_POINT('Ctrl Pts',(22.393557425739,19.0671762596305,39.1687847425188));
#58512=CARTESIAN_POINT('Ctrl Pts',(22.1994672242047,19.1928990545496,36.6738997707503));
#58513=CARTESIAN_POINT('Ctrl Pts',(20.0009389117691,19.3186218494687,35.4786612004172));
#58514=CARTESIAN_POINT('Ctrl Pts',(17.8015549032927,19.4443446443878,36.6723245489679));
#58515=CARTESIAN_POINT('Ctrl Pts',(17.6056776060072,19.5700674393069,39.1670698255491));
#58516=CARTESIAN_POINT('Ctrl Pts',(19.5918154497326,19.6957902342259,40.6893635397801));
#58517=CARTESIAN_POINT('Ctrl Pts',(21.9499439670764,19.821513029145,39.8518952325912));
#58518=CARTESIAN_POINT('Ctrl Pts',(22.5310315747525,19.9472358240641,37.4178742871035));
#58519=CARTESIAN_POINT('Ctrl Pts',(20.8055179179848,20.0729586189832,35.6054938860462));
#58520=CARTESIAN_POINT('Ctrl Pts',(18.3459104295828,20.1986814139022,36.066429786708));
#58521=CARTESIAN_POINT('Ctrl Pts',(17.3937265915144,20.3244042088213,38.3806157290309));
#58522=CARTESIAN_POINT('Ctrl Pts',(18.8167074628455,20.4501270037404,40.4390710379465));
#58523=CARTESIAN_POINT('Ctrl Pts',(21.318071928025,20.5758497986595,40.3658581803161));
#58524=CARTESIAN_POINT('Ctrl Pts',(22.6182105026428,20.7015725935786,38.2277129594711));
#58525=CARTESIAN_POINT('Ctrl Pts',(21.5323538864901,20.8272953884976,35.9731602960804));
#58526=CARTESIAN_POINT('Ctrl Pts',(19.0499106856773,20.9530181834167,35.6568948787136));
#58527=CARTESIAN_POINT('Ctrl Pts',(17.4335209345191,21.0787409783358,37.5670307872341));
#58528=CARTESIAN_POINT('Ctrl Pts',(18.1556317081086,21.2044637732549,39.9630146849301));
#58529=CARTESIAN_POINT('Ctrl Pts',(20.5593559198267,21.3301865681739,40.6609124994508));
#58530=CARTESIAN_POINT('Ctrl Pts',(22.4517947373209,21.455909363093,39.0254939206425));
#58531=CARTESIAN_POINT('Ctrl Pts',(22.1128295407574,21.5816321580121,36.5456425586315));
#58532=CARTESIAN_POINT('Ctrl Pts',(19.8420657823089,21.707369734299,35.4841517828753));
#58533=CARTESIAN_POINT('Ctrl Pts',(18.433464815411,21.7911997122795,36.3635933916213));
#58534=CARTESIAN_POINT('Ctrl Pts',(18.0698183975814,21.8331220919537,37.004138400054));
#58535=CARTESIAN_POINT('Ctrl Pts',(21.2977109876404,0.0420943265399541,
39.7161014880613));
#58536=CARTESIAN_POINT('Ctrl Pts',(21.8340555061094,0.0840185761245343,
39.2854503699403));
#58537=CARTESIAN_POINT('Ctrl Pts',(22.4349388060586,0.167850424015474,37.8558861542791));
#58538=CARTESIAN_POINT('Ctrl Pts',(21.1180778385984,0.293589870212774,35.9207310046821));
#58539=CARTESIAN_POINT('Ctrl Pts',(18.7815540989668,0.419312665131854,35.9777303342837));
#58540=CARTESIAN_POINT('Ctrl Pts',(17.5559152313698,0.545035460050933,37.9659119570555));
#58541=CARTESIAN_POINT('Ctrl Pts',(18.5573923750011,0.670758254970012,40.0777776761189));
#58542=CARTESIAN_POINT('Ctrl Pts',(20.8736883315835,0.796481049889092,40.3864718933352));
#58543=CARTESIAN_POINT('Ctrl Pts',(22.3937003777697,0.922203844808171,38.6118330009634));
#58544=CARTESIAN_POINT('Ctrl Pts',(21.7322982928821,1.04792663972725,36.3705421108507));
#58545=CARTESIAN_POINT('Ctrl Pts',(19.4921849462116,1.17364943464633,35.7054613985552));
#58546=CARTESIAN_POINT('Ctrl Pts',(17.7148672861923,1.29937222956541,37.2225387428673));
#58547=CARTESIAN_POINT('Ctrl Pts',(18.0200524837552,1.42509502448449,39.539299926903));
#58548=CARTESIAN_POINT('Ctrl Pts',(20.1296235817924,1.55081781940357,40.5443709850134));
#58549=CARTESIAN_POINT('Ctrl Pts',(22.1210637035315,1.67654061432265,39.3218234855224));
#58550=CARTESIAN_POINT('Ctrl Pts',(22.1795177394272,1.80226340924173,36.9857890373839));
#58551=CARTESIAN_POINT('Ctrl Pts',(20.2517138530609,1.92798620416081,35.6651692691415));
#58552=CARTESIAN_POINT('Ctrl Pts',(18.0945160206517,2.05370899907988,36.563480181515));
#58553=CARTESIAN_POINT('Ctrl Pts',(17.6738407915532,2.17943179399897,38.8620665980196));
#58554=CARTESIAN_POINT('Ctrl Pts',(19.3730618107187,2.30515458891804,40.4661593977127));
#58555=CARTESIAN_POINT('Ctrl Pts',(21.6436297207534,2.43087738383713,39.9139028058985));
#58556=CARTESIAN_POINT('Ctrl Pts',(22.416310314239,2.55660017875621,37.7085840226691));
#58557=CARTESIAN_POINT('Ctrl Pts',(20.9869373875313,2.68232297367528,35.8599739841007));
#58558=CARTESIAN_POINT('Ctrl Pts',(18.658139862288,2.80804576859437,36.0527644575676));
#58559=CARTESIAN_POINT('Ctrl Pts',(17.5522183103459,2.93376856351344,38.1112599348682));
#58560=CARTESIAN_POINT('Ctrl Pts',(18.6770310483036,3.05949135843252,40.1594939025224));
#58561=CARTESIAN_POINT('Ctrl Pts',(21.0075036762963,3.1852141533516,40.3308514807028));
#58562=CARTESIAN_POINT('Ctrl Pts',(22.4198090486167,3.31093694827068,38.4691695455411));
#58563=CARTESIAN_POINT('Ctrl Pts',(21.6268724090507,3.43665974318976,36.2710527210051));
#58564=CARTESIAN_POINT('Ctrl Pts',(19.3513198638514,3.56238253810884,35.7397084785321));
#58565=CARTESIAN_POINT('Ctrl Pts',(17.6669282985544,3.68810533302792,37.3593662031733));
#58566=CARTESIAN_POINT('Ctrl Pts',(18.1087324905111,3.813828127947,39.6539849396328));
#58567=CARTESIAN_POINT('Ctrl Pts',(20.2741034943941,3.93955092286608,40.5324122305857));
#58568=CARTESIAN_POINT('Ctrl Pts',(22.1896760516827,4.06527371778516,39.1941118652993));
#58569=CARTESIAN_POINT('Ctrl Pts',(22.1097334570229,4.19099651270424,36.8587156951692));
#58570=CARTESIAN_POINT('Ctrl Pts',(20.1071297103542,4.31671930762331,35.6545378329912));
#58571=CARTESIAN_POINT('Ctrl Pts',(18.0068955584607,4.4424421025424,36.6789804117387));
#58572=CARTESIAN_POINT('Ctrl Pts',(17.723035161693,4.56816489746147,38.9984392635119));
#58573=CARTESIAN_POINT('Ctrl Pts',(19.5142387141328,4.69388769238056,40.499124414919));
#58574=CARTESIAN_POINT('Ctrl Pts',(21.7481305836104,4.81961048729963,39.8134180598305));
#58575=CARTESIAN_POINT('Ctrl Pts',(22.3889004638811,4.94533328221871,37.5662242429861));
#58576=CARTESIAN_POINT('Ctrl Pts',(20.8525962201039,5.07105607713779,35.8054757202043));
#58577=CARTESIAN_POINT('Ctrl Pts',(18.5392963680484,5.19677887205687,36.1357935738037));
#58578=CARTESIAN_POINT('Ctrl Pts',(17.5571780064341,5.32250166697596,38.2561495848798));
#58579=CARTESIAN_POINT('Ctrl Pts',(18.8012740192805,5.44822446189503,40.2342019605124));
#58580=CARTESIAN_POINT('Ctrl Pts',(21.137803707747,5.57394725681411,40.267294328822));
#58581=CARTESIAN_POINT('Ctrl Pts',(22.4374199509555,5.6996700517332,38.325268656923));
#58582=CARTESIAN_POINT('Ctrl Pts',(21.5157448574613,5.82539284665227,36.1779491390219));
#58583=CARTESIAN_POINT('Ctrl Pts',(19.212727611906,5.95111564157135,35.7822501920932));
#58584=CARTESIAN_POINT('Ctrl Pts',(17.6271744761412,6.07683843649043,37.4987837174265));
#58585=CARTESIAN_POINT('Ctrl Pts',(18.2040459063968,6.2025612314095,39.7632230393958));
#58586=CARTESIAN_POINT('Ctrl Pts',(20.4176222744586,6.32828402632859,40.5119190743023));
#58587=CARTESIAN_POINT('Ctrl Pts',(22.2506073784236,6.45400682124767,39.0625634593587));
#58588=CARTESIAN_POINT('Ctrl Pts',(22.0325488491192,6.57972961616675,36.7359959087116));
#58589=CARTESIAN_POINT('Ctrl Pts',(19.9621697345979,6.70545241108583,35.652484758755));
#58590=CARTESIAN_POINT('Ctrl Pts',(17.9262664356906,6.8311752060049,36.7994650756846));
#58591=CARTESIAN_POINT('Ctrl Pts',(17.7802165447788,6.95689800092399,39.1316605047367));
#58592=CARTESIAN_POINT('Ctrl Pts',(19.6571195539224,7.08262079584305,40.5236738610639));
#58593=CARTESIAN_POINT('Ctrl Pts',(21.8464994360391,7.20834359076215,39.7069230901989));
#58594=CARTESIAN_POINT('Ctrl Pts',(22.3531109470789,7.33406638568122,37.4257368052129));
#58595=CARTESIAN_POINT('Ctrl Pts',(20.7152643564292,7.45978918060031,35.759026081835));
#58596=CARTESIAN_POINT('Ctrl Pts',(18.4255766590528,7.58551197551937,36.2257126344692));
#58597=CARTESIAN_POINT('Ctrl Pts',(17.5707065138088,7.71123477043847,38.4004915024686));
#58598=CARTESIAN_POINT('Ctrl Pts',(18.9297218227593,7.83695756535754,40.3014237684802));
#58599=CARTESIAN_POINT('Ctrl Pts',(21.2641126069269,7.96268036027662,40.1961348482662));
#58600=CARTESIAN_POINT('Ctrl Pts',(22.4464809908173,8.0884031551957,38.180577581726));
#58601=CARTESIAN_POINT('Ctrl Pts',(21.3993004501658,8.21412595011479,36.0915876331608));
#58602=CARTESIAN_POINT('Ctrl Pts',(19.0768969155535,8.33984874503385,35.8329219950357));
#58603=CARTESIAN_POINT('Ctrl Pts',(17.5957439350612,8.46557153995296,37.6403101487827));
#58604=CARTESIAN_POINT('Ctrl Pts',(18.3056590822296,8.59129433487201,39.8666269667012));
#58605=CARTESIAN_POINT('Ctrl Pts',(20.5596761395299,8.7170171297911,40.4829655062439));
#58606=CARTESIAN_POINT('Ctrl Pts',(22.3036441346612,8.84273992471017,38.9276386203823));
#58607=CARTESIAN_POINT('Ctrl Pts',(21.9482345657571,8.96846271962927,36.6180607091055));
#58608=CARTESIAN_POINT('Ctrl Pts',(19.817342457997,9.09418551454833,35.6590169587937));
#58609=CARTESIAN_POINT('Ctrl Pts',(17.8529114541085,9.21990830946742,36.9245116924406));
#58610=CARTESIAN_POINT('Ctrl Pts',(17.8451843757182,9.34563110438649,39.2612629376924));
#58611=CARTESIAN_POINT('Ctrl Pts',(19.8012031329734,9.47135389930557,40.5397216625606));
#58612=CARTESIAN_POINT('Ctrl Pts',(21.9383912280429,9.59707669422467,39.5947914343325));
#58613=CARTESIAN_POINT('Ctrl Pts',(22.3090673027673,9.72279948914372,37.2876145149019));
#58614=CARTESIAN_POINT('Ctrl Pts',(20.5754235234226,9.84852228406283,35.7207879972984));
#58615=CARTESIAN_POINT('Ctrl Pts',(18.3173796352609,9.97424507898189,36.3222062287001));
#58616=CARTESIAN_POINT('Ctrl Pts',(17.592756378078,10.099967873901,38.5437793706595));
#58617=CARTESIAN_POINT('Ctrl Pts',(19.0619238956901,10.2256906688201,40.3609235298059));
#58618=CARTESIAN_POINT('Ctrl Pts',(21.3859873137211,10.3514134637392,40.1176226483937));
#58619=CARTESIAN_POINT('Ctrl Pts',(22.4469603842963,10.4771362586582,38.0356038604284));
#58620=CARTESIAN_POINT('Ctrl Pts',(21.2779476451792,10.6028590535773,36.0122711379855));
#58621=CARTESIAN_POINT('Ctrl Pts',(18.9443042350597,10.7285818484964,35.8915461433405));
#58622=CARTESIAN_POINT('Ctrl Pts',(17.572746925834,10.8543046434155,37.7834490577195));
#58623=CARTESIAN_POINT('Ctrl Pts',(18.4132155842779,10.9800274383345,39.9638340063237));
#58624=CARTESIAN_POINT('Ctrl Pts',(20.6997668000079,11.1057502332536,40.4456530883133));
#58625=CARTESIAN_POINT('Ctrl Pts',(22.348600280655,11.2314730281727,38.7898106311262));
#58626=CARTESIAN_POINT('Ctrl Pts',(21.8570863604567,11.3571958230918,36.505323783675));
#58627=CARTESIAN_POINT('Ctrl Pts',(19.6731558985896,11.4829186180109,35.6741115197767));
#58628=CARTESIAN_POINT('Ctrl Pts',(17.7870879247318,11.6086414129299,37.0536816295986));
#58629=CARTESIAN_POINT('Ctrl Pts',(17.9177107635305,11.734364207849,39.3867919493028));
#58630=CARTESIAN_POINT('Ctrl Pts',(19.9459840419529,11.8600870027681,40.5472115277155));
#58631=CARTESIAN_POINT('Ctrl Pts',(22.0234836260872,11.9858097976872,39.4774164221702));
#58632=CARTESIAN_POINT('Ctrl Pts',(22.256924025088,12.1115325926063,37.1523418706686));
#58633=CARTESIAN_POINT('Ctrl Pts',(20.4335642479196,12.2372553875253,35.6908955962779));
#58634=CARTESIAN_POINT('Ctrl Pts',(18.2150848249019,12.3629781824444,36.4249358809851));
#58635=CARTESIAN_POINT('Ctrl Pts',(17.6232502538064,12.4887009773635,38.6855105712756));
#58636=CARTESIAN_POINT('Ctrl Pts',(19.1974165061062,12.6144237722826,40.4124925341364));
#58637=CARTESIAN_POINT('Ctrl Pts',(21.5030003219933,12.7401465672016,40.03203313046));
#58638=CARTESIAN_POINT('Ctrl Pts',(22.4388564497993,12.8658693621208,37.8908560247601));
#58639=CARTESIAN_POINT('Ctrl Pts',(21.1521121179363,12.9915921570398,35.9402778760194));
#58640=CARTESIAN_POINT('Ctrl Pts',(18.815414672545,13.1173149519589,35.9579169980868));
#58641=CARTESIAN_POINT('Ctrl Pts',(17.5582641162439,13.243037746878,37.9276983485718));
#58642=CARTESIAN_POINT('Ctrl Pts',(18.5263381311034,13.3687605417971,40.054503180163));
#58643=CARTESIAN_POINT('Ctrl Pts',(20.8374028527246,13.4944833367161,40.4001127031856));
#58644=CARTESIAN_POINT('Ctrl Pts',(22.3853181214344,13.6202061316352,38.649562957871));
#58645=CARTESIAN_POINT('Ctrl Pts',(21.7594239584356,13.7459289265543,36.3981805854939));
#58646=CARTESIAN_POINT('Ctrl Pts',(19.530115826938,13.8716517214733,35.6977154937408));
#58647=CARTESIAN_POINT('Ctrl Pts',(17.729026740118,13.9973745163925,37.1865217911697));
#58648=CARTESIAN_POINT('Ctrl Pts',(17.9975413036994,14.1230973113115,39.5078072150396));
#58649=CARTESIAN_POINT('Ctrl Pts',(20.0909544254689,14.2488201062306,40.5461171839458));
#58650=CARTESIAN_POINT('Ctrl Pts',(22.1014781472193,14.3745429011497,39.3552097760401));
#58651=CARTESIAN_POINT('Ctrl Pts',(22.1968640196805,14.5002656960688,37.0203933752795));
#58652=CARTESIAN_POINT('Ctrl Pts',(20.2901841369496,14.6259884909878,35.6694537338759));
#58653=CARTESIAN_POINT('Ctrl Pts',(18.1190510527088,14.7517112859069,36.5335412412735));
#58654=CARTESIAN_POINT('Ctrl Pts',(17.6620811760677,14.877434080826,38.8251879465421));
#58655=CARTESIAN_POINT('Ctrl Pts',(19.3357243796546,15.0031568757451,40.45594989024));
#58656=CARTESIAN_POINT('Ctrl Pts',(21.614741179235,15.1288796706642,39.9396665211908));
#58657=CARTESIAN_POINT('Ctrl Pts',(22.4221976139118,15.2546024655832,37.7468418141005));
#58658=CARTESIAN_POINT('Ctrl Pts',(21.0222352681462,15.3803252605023,35.8758603817059));
#58659=CARTESIAN_POINT('Ctrl Pts',(18.6906803405137,15.5060480554214,36.0318017468361));
#58660=CARTESIAN_POINT('Ctrl Pts',(17.5523463083822,15.6317708503405,38.0725520307311));
#58661=CARTESIAN_POINT('Ctrl Pts',(18.6446299169683,15.7574936452595,40.1383164433252));
#58662=CARTESIAN_POINT('Ctrl Pts',(20.9721015046648,15.8832164401786,40.3465040951967));
#58663=CARTESIAN_POINT('Ctrl Pts',(22.4136688599532,16.0089392350977,38.5073875545465));
#58664=CARTESIAN_POINT('Ctrl Pts',(21.6555899350916,16.1346620300168,36.2970069462334));
#58665=CARTESIAN_POINT('Ctrl Pts',(19.3887239920105,16.2603848249359,35.7297460838206));
#58666=CARTESIAN_POINT('Ctrl Pts',(17.678931564451,16.3861076198549,37.3225662069312));
#58667=CARTESIAN_POINT('Ctrl Pts',(18.08439597056,16.511830414774,39.6238842434713));
#58668=CARTESIAN_POINT('Ctrl Pts',(20.2356057634987,16.6375532096931,40.5364424699371));
#58669=CARTESIAN_POINT('Ctrl Pts',(22.1721012060722,16.7632760046122,39.2286001664393));
#58670=CARTESIAN_POINT('Ctrl Pts',(22.1290979620948,16.8889987995313,36.8922318712142));
#58671=CARTESIAN_POINT('Ctrl Pts',(20.1457861322546,17.0147215944504,35.6565376228087));
#58672=CARTESIAN_POINT('Ctrl Pts',(18.0296151812518,17.1404443893694,36.6476413489935));
#58673=CARTESIAN_POINT('Ctrl Pts',(17.7091129356516,17.2661671842885,38.9623215429927));
#58674=CARTESIAN_POINT('Ctrl Pts',(19.4763623667403,17.3918899792076,40.4911431605282));
#58675=CARTESIAN_POINT('Ctrl Pts',(21.720817926331,17.5176127741267,39.840846819661));
#58676=CARTESIAN_POINT('Ctrl Pts',(22.397042311684,17.6433355690457,37.6040663944551));
#58677=CARTESIAN_POINT('Ctrl Pts',(20.8887726714696,17.7690583639648,35.8192446155825));
#58678=CARTESIAN_POINT('Ctrl Pts',(18.57053877596,17.8947811588839,36.1129412202786));
#58679=CARTESIAN_POINT('Ctrl Pts',(17.555014260439,18.020503953803,38.2175019935372));
#58680=CARTESIAN_POINT('Ctrl Pts',(18.7676760037445,18.1462267487221,40.2149797997396));
#58681=CARTESIAN_POINT('Ctrl Pts',(21.1033902664578,18.2719495436411,40.2850153100092));
#58682=CARTESIAN_POINT('Ctrl Pts',(22.4335530489282,18.3976723385602,38.3637831370628));
#58683=CARTESIAN_POINT('Ctrl Pts',(21.5459485142351,18.5233951334793,36.2021577578715));
#58684=CARTESIAN_POINT('Ctrl Pts',(19.2494763613636,18.6491179283984,35.7700909346134));
#58685=CARTESIAN_POINT('Ctrl Pts',(17.6369781187664,18.7748407233175,37.4613376670606));
#58686=CARTESIAN_POINT('Ctrl Pts',(18.1779701002801,18.9005635182365,39.7346158650296));
#58687=CARTESIAN_POINT('Ctrl Pts',(20.3794306537555,19.0262863131556,40.5182213226522));
#58688=CARTESIAN_POINT('Ctrl Pts',(22.2351050772414,19.1520091080747,39.0980317074466));
#58689=CARTESIAN_POINT('Ctrl Pts',(22.0538635535465,19.2777319029938,36.7683069189088));
#58690=CARTESIAN_POINT('Ctrl Pts',(20.0008767562623,19.4034546979128,35.6521925661306));
#58691=CARTESIAN_POINT('Ctrl Pts',(17.947090909603,19.529177492832,36.7668359760495));
#58692=CARTESIAN_POINT('Ctrl Pts',(17.7641805950347,19.654900287751,39.0964303171541));
#58693=CARTESIAN_POINT('Ctrl Pts',(19.6188370703191,19.7806230826701,40.5179489208616));
#58694=CARTESIAN_POINT('Ctrl Pts',(21.8208586158333,19.9063458775892,39.7359206121618));
#58695=CARTESIAN_POINT('Ctrl Pts',(22.3634785038178,20.0320686725083,37.4630306806861));
#58696=CARTESIAN_POINT('Ctrl Pts',(20.7521930198691,20.1577914674273,35.770628989072));
#58697=CARTESIAN_POINT('Ctrl Pts',(18.4554103622938,20.2835142623465,36.2010511551641));
#58698=CARTESIAN_POINT('Ctrl Pts',(17.5662606355948,20.4092370572655,38.3620391029544));
#58699=CARTESIAN_POINT('Ctrl Pts',(18.8950408587589,20.5349598521846,40.2842256620722));
#58700=CARTESIAN_POINT('Ctrl Pts',(21.2308162013654,20.6606826471036,40.215859460347));
#58701=CARTESIAN_POINT('Ctrl Pts',(22.4448862286797,20.7864054420227,38.2192584230794));
#58702=CARTESIAN_POINT('Ctrl Pts',(21.4309127974096,20.9121282369418,36.1139560598838));
#58703=CARTESIAN_POINT('Ctrl Pts',(19.1128061405839,21.0378510318609,35.8186272607871));
#58704=CARTESIAN_POINT('Ctrl Pts',(17.6034206122633,21.16357382678,37.6023130923634));
#58705=CARTESIAN_POINT('Ctrl Pts',(18.277728000515,21.2892966216991,39.8396840102872));
#58706=CARTESIAN_POINT('Ctrl Pts',(20.5223268274015,21.4150194166181,40.4913813256959));
#58707=CARTESIAN_POINT('Ctrl Pts',(22.2894871068521,21.5407422115372,38.9642266689488));
#58708=CARTESIAN_POINT('Ctrl Pts',(21.972961243006,21.6664650064563,36.6485402724449));
#58709=CARTESIAN_POINT('Ctrl Pts',(19.8525209514359,21.7922025827432,35.6573196746751));
#58710=CARTESIAN_POINT('Ctrl Pts',(18.537168689959,21.8760325607237,36.4785426725894));
#58711=CARTESIAN_POINT('Ctrl Pts',(18.1975954898047,21.9179549403979,37.0766839100436));
#58712=CARTESIAN_POINT('Ctrl Pts',(21.2057129175019,0.126927174984125,39.6015318963221));
#58713=CARTESIAN_POINT('Ctrl Pts',(21.7040345933669,0.168851424568706,39.2014107437692));
#58714=CARTESIAN_POINT('Ctrl Pts',(22.2623197304739,0.252683272459645,37.8731920127594));
#58715=CARTESIAN_POINT('Ctrl Pts',(21.0388144244828,0.378422718656945,36.0752249896998));
#58716=CARTESIAN_POINT('Ctrl Pts',(18.8679328632146,0.504145513576025,36.1281834902012));
#58717=CARTESIAN_POINT('Ctrl Pts',(17.7291826877682,0.629868308495104,37.9754178033472));
#58718=CARTESIAN_POINT('Ctrl Pts',(18.6596625404933,0.755591103414184,39.9375679290345));
#58719=CARTESIAN_POINT('Ctrl Pts',(20.8117503182865,0.881313898333262,40.2243780191089));
#58720=CARTESIAN_POINT('Ctrl Pts',(22.2240048004479,1.00703669325235,38.5755478428887));
#58721=CARTESIAN_POINT('Ctrl Pts',(21.6094912107451,1.13275948817143,36.4931478294605));
#58722=CARTESIAN_POINT('Ctrl Pts',(19.5281852616754,1.2584822830905,35.8752163997095));
#58723=CARTESIAN_POINT('Ctrl Pts',(17.876866222537,1.38420507800959,37.2847442285619));
#58724=CARTESIAN_POINT('Ctrl Pts',(18.160416056388,1.50992787292866,39.4372642526377));
#58725=CARTESIAN_POINT('Ctrl Pts',(20.1204342326361,1.63565066784774,40.3710832379994));
#58726=CARTESIAN_POINT('Ctrl Pts',(21.9706960413755,1.76137346276682,39.2352052756217));
#58727=CARTESIAN_POINT('Ctrl Pts',(22.0250061202997,1.8870962576859,37.064778318714));
#58728=CARTESIAN_POINT('Ctrl Pts',(20.23386921051,2.01281905260498,35.8377806829972));
#58729=CARTESIAN_POINT('Ctrl Pts',(18.2296006816042,2.13854184752406,36.6724080239824));
#58730=CARTESIAN_POINT('Ctrl Pts',(17.8387482016392,2.26426464244315,38.8080417365501));
#58731=CARTESIAN_POINT('Ctrl Pts',(19.4175070716892,2.38998743736221,40.2984162713134));
#58732=CARTESIAN_POINT('Ctrl Pts',(21.5271085817852,2.5157102322813,39.7853105699147));
#58733=CARTESIAN_POINT('Ctrl Pts',(22.2450118603592,2.64143302720037,37.7363325081784));
#58734=CARTESIAN_POINT('Ctrl Pts',(20.9169708573369,2.76715582211946,36.0187751905983));
#58735=CARTESIAN_POINT('Ctrl Pts',(18.7532677792441,2.89287861703854,36.1978982514681));
#58736=CARTESIAN_POINT('Ctrl Pts',(17.7257478509857,3.01860141195762,38.1104616891203));
#58737=CARTESIAN_POINT('Ctrl Pts',(18.7708197204874,3.1443242068767,40.0134910819418));
#58738=CARTESIAN_POINT('Ctrl Pts',(20.9360791489867,3.27004700179578,40.1727006806057));
#58739=CARTESIAN_POINT('Ctrl Pts',(22.2482625604568,3.39576979671486,38.442998166808));
#58740=CARTESIAN_POINT('Ctrl Pts',(21.5115392390155,3.52149259163393,36.400711498387));
#58741=CARTESIAN_POINT('Ctrl Pts',(19.3973064673642,3.64721538655302,35.90703561609));
#58742=CARTESIAN_POINT('Ctrl Pts',(17.8323257530507,3.77293818147209,37.4118716382326));
#58743=CARTESIAN_POINT('Ctrl Pts',(18.2428093093449,3.89866097639118,39.5438189498));
#58744=CARTESIAN_POINT('Ctrl Pts',(20.2546715925742,4.02438377131025,40.3599722704356));
#58745=CARTESIAN_POINT('Ctrl Pts',(22.0344442836683,4.15010656622933,39.1165474606809));
#58746=CARTESIAN_POINT('Ctrl Pts',(21.9601690251878,4.27582936114841,36.9467135326116));
#58747=CARTESIAN_POINT('Ctrl Pts',(20.0995350096073,4.40155215606749,35.8279029367039));
#58748=CARTESIAN_POINT('Ctrl Pts',(18.1481918593724,4.52727495098657,36.7797201457734));
#58749=CARTESIAN_POINT('Ctrl Pts',(17.8844550563323,4.65299774590565,38.9347465929813));
#58750=CARTESIAN_POINT('Ctrl Pts',(19.5486755812576,4.77872054082473,40.329044313651));
#58751=CARTESIAN_POINT('Ctrl Pts',(21.6242011096567,4.90444333574381,39.6919494459819));
#58752=CARTESIAN_POINT('Ctrl Pts',(22.2195451648021,5.03016613066288,37.6040649794827));
#58753=CARTESIAN_POINT('Ctrl Pts',(20.7921534808469,5.15588892558196,35.9681404488207));
#58754=CARTESIAN_POINT('Ctrl Pts',(18.6428494060235,5.28161172050103,36.2750412200706));
#58755=CARTESIAN_POINT('Ctrl Pts',(17.7303559414599,5.40733451542013,38.2450797391293));
#58756=CARTESIAN_POINT('Ctrl Pts',(18.8862547876498,5.53305731033921,40.0829028935224));
#58757=CARTESIAN_POINT('Ctrl Pts',(21.0571418760249,5.65878010525829,40.1136492587158));
#58758=CARTESIAN_POINT('Ctrl Pts',(22.2646249806265,5.78450290017737,38.3092987823539));
#58759=CARTESIAN_POINT('Ctrl Pts',(21.4082898054222,5.91022569509645,36.3142082688297));
#58760=CARTESIAN_POINT('Ctrl Pts',(19.2685393766731,6.03594849001553,35.9465614381426));
#58761=CARTESIAN_POINT('Ctrl Pts',(17.7953901813709,6.1616712849346,37.5414054862636));
#58762=CARTESIAN_POINT('Ctrl Pts',(18.3313657119948,6.28739407985369,39.6453128796672));
#58763=CARTESIAN_POINT('Ctrl Pts',(20.3880159571329,6.41311687477276,40.3409319267177));
#58764=CARTESIAN_POINT('Ctrl Pts',(22.0910560319171,6.53883966969183,38.9943248596318));
#58765=CARTESIAN_POINT('Ctrl Pts',(21.8884562326876,6.66456246461093,36.8326936674997));
#58766=CARTESIAN_POINT('Ctrl Pts',(19.9648516194267,6.79028525952999,35.8259954101816));
#58767=CARTESIAN_POINT('Ctrl Pts',(18.0732787425253,6.91600805444907,36.8916633419583));
#58768=CARTESIAN_POINT('Ctrl Pts',(17.9375827040782,7.04173084936815,39.058523437718));
#58769=CARTESIAN_POINT('Ctrl Pts',(19.6814272307687,7.16745364428724,40.3518533864079));
#58770=CARTESIAN_POINT('Ctrl Pts',(21.7155963410933,7.29317643920632,39.5930041786945));
#58771=CARTESIAN_POINT('Ctrl Pts',(22.1862928589108,7.41889923412539,37.4735370575624));
#58772=CARTESIAN_POINT('Ctrl Pts',(20.6645574262598,7.54462202904449,35.9249837448021));
#58773=CARTESIAN_POINT('Ctrl Pts',(18.5371915797305,7.67034482396355,36.3585856872182));
#58774=CARTESIAN_POINT('Ctrl Pts',(17.742925378146,7.79606761888264,38.3791888868759));
#58775=CARTESIAN_POINT('Ctrl Pts',(19.0055965959216,7.92179041380171,40.1453591746023));
#58776=CARTESIAN_POINT('Ctrl Pts',(21.1744964124255,8.0475132087208,40.0475344567868));
#58777=CARTESIAN_POINT('Ctrl Pts',(22.273043660064,8.17323600363987,38.1748652296802));
#58778=CARTESIAN_POINT('Ctrl Pts',(21.3001004417008,8.29895879855895,36.2339691522749));
#58779=CARTESIAN_POINT('Ctrl Pts',(19.1423380677952,8.42468159347804,35.9936409866267));
#58780=CARTESIAN_POINT('Ctrl Pts',(17.7661878321998,8.55040438839711,37.6728987448391));
#58781=CARTESIAN_POINT('Ctrl Pts',(18.4257752684035,8.6761271833162,39.7413862365702));
#58782=CARTESIAN_POINT('Ctrl Pts',(20.5199992582908,8.80184997823527,40.3140309515788));
#58783=CARTESIAN_POINT('Ctrl Pts',(22.1403328760735,8.92757277315435,38.8689651895704));
#58784=CARTESIAN_POINT('Ctrl Pts',(21.8101192057626,9.05329556807344,36.7231191975695));
#58785=CARTESIAN_POINT('Ctrl Pts',(19.8302915210169,9.1790183629925,35.8320645257562));
#58786=CARTESIAN_POINT('Ctrl Pts',(18.0051240842855,9.30474115791159,37.0078450823832));
#58787=CARTESIAN_POINT('Ctrl Pts',(17.9979447983593,9.43046395283067,39.1789380208129));
#58788=CARTESIAN_POINT('Ctrl Pts',(19.8152963542609,9.55618674774975,40.3667635179752));
#58789=CARTESIAN_POINT('Ctrl Pts',(21.80097368758,9.68190954266882,39.4888218243594));
#58790=CARTESIAN_POINT('Ctrl Pts',(22.1453715818421,9.8076323375879,37.3452066117164));
#58791=CARTESIAN_POINT('Ctrl Pts',(20.5346302696308,9.93335513250699,35.8894564564418));
#58792=CARTESIAN_POINT('Ctrl Pts',(18.4366649212808,10.0590779274261,36.4482386023345));
#58793=CARTESIAN_POINT('Ctrl Pts',(17.7634120708163,10.1848007223452,38.5123187094979));
#58794=CARTESIAN_POINT('Ctrl Pts',(19.1284265238265,10.3105235172642,40.2006408447907));
#58795=CARTESIAN_POINT('Ctrl Pts',(21.2877311077452,10.4362463121833,39.9745881887277));
#58796=CARTESIAN_POINT('Ctrl Pts',(22.2734890681061,10.5619691071024,38.0401690684149));
#58797=CARTESIAN_POINT('Ctrl Pts',(21.187350649227,10.6876919020215,36.1602756074759));
#58798=CARTESIAN_POINT('Ctrl Pts',(19.0191452235023,10.8134146969406,36.0481091182536));
#58799=CARTESIAN_POINT('Ctrl Pts',(17.744821140114,10.9391374918596,37.8058901683115));
#58800=CARTESIAN_POINT('Ctrl Pts',(18.5257068133439,11.0648602867787,39.8317020190991));
#58801=CARTESIAN_POINT('Ctrl Pts',(20.650158531479,11.1905830816978,40.2793637069377));
#58802=CARTESIAN_POINT('Ctrl Pts',(22.1821019652329,11.3163058766169,38.7409081810206));
#58803=CARTESIAN_POINT('Ctrl Pts',(21.7254327312052,11.442028671536,36.6183744827865));
#58804=CARTESIAN_POINT('Ctrl Pts',(19.6963267177105,11.567751466455,35.8460889944819));
#58805=CARTESIAN_POINT('Ctrl Pts',(17.9439669542304,11.6934742613741,37.1278578304199));
#58806=CARTESIAN_POINT('Ctrl Pts',(18.0653296039732,11.8191970562932,39.2955679578802));
#58807=CARTESIAN_POINT('Ctrl Pts',(19.9498133721693,11.9449198512123,40.3737224073222));
#58808=CARTESIAN_POINT('Ctrl Pts',(21.8800336666357,12.0706426461313,39.3797678287443));
#58809=CARTESIAN_POINT('Ctrl Pts',(22.0969248752505,12.1963654410504,37.2195237932074));
#58810=CARTESIAN_POINT('Ctrl Pts',(20.4028277630863,12.3220882359695,35.8616832046247));
#58811=CARTESIAN_POINT('Ctrl Pts',(18.3416220531705,12.4478110308886,36.5436854853077));
#58812=CARTESIAN_POINT('Ctrl Pts',(17.791744157252,12.5735338258077,38.6440022207137));
#58813=CARTESIAN_POINT('Ctrl Pts',(19.2543137145497,12.6992566207267,40.2485539897483));
#58814=CARTESIAN_POINT('Ctrl Pts',(21.3964487628574,12.8249794156458,39.8950663318903));
#58815=CARTESIAN_POINT('Ctrl Pts',(22.2659596423722,12.9507022105649,37.9056827791656));
#58816=CARTESIAN_POINT('Ctrl Pts',(21.070435926209,13.076425005484,36.0933861330457));
#58817=CARTESIAN_POINT('Ctrl Pts',(18.899392973629,13.2021478004031,36.1097747723749));
#58818=CARTESIAN_POINT('Ctrl Pts',(17.7313650541513,13.3278705953222,37.9399132558693));
#58819=CARTESIAN_POINT('Ctrl Pts',(18.6308098118291,13.4535933902412,39.915943421968));
#58820=CARTESIAN_POINT('Ctrl Pts',(20.7780372103644,13.5793161851603,40.2370517968595));
#58821=CARTESIAN_POINT('Ctrl Pts',(22.2162167838267,13.7050389800794,38.6106030260947));
#58822=CARTESIAN_POINT('Ctrl Pts',(21.6346938680896,13.8307617749985,36.5188269415392));
#58823=CARTESIAN_POINT('Ctrl Pts',(19.5634271246938,13.9564845699175,35.868019622013));
#58824=CARTESIAN_POINT('Ctrl Pts',(17.8900218763501,14.0822073648366,37.2512806112199));
#58825=CARTESIAN_POINT('Ctrl Pts',(18.1395007517939,14.2079301597557,39.4080041401299));
#58826=CARTESIAN_POINT('Ctrl Pts',(20.0845064322766,14.3336529546748,40.3727056443974));
#58827=CARTESIAN_POINT('Ctrl Pts',(21.9524989555321,14.4593757495939,39.266224726122));
#58828=CARTESIAN_POINT('Ctrl Pts',(22.0411226781244,14.5850985445129,37.09692946608));
#58829=CARTESIAN_POINT('Ctrl Pts',(20.2696122370133,14.710821339432,35.8417614110053));
#58830=CARTESIAN_POINT('Ctrl Pts',(18.252396362125,14.8365441343511,36.6445915322294));
#58831=CARTESIAN_POINT('Ctrl Pts',(17.8278222555458,14.9622669292702,38.7737775075423));
#58832=CARTESIAN_POINT('Ctrl Pts',(19.3828165871599,15.0879897241893,40.2889305420883));
#58833=CARTESIAN_POINT('Ctrl Pts',(21.5002680232876,15.2137125191083,39.8092478291555));
#58834=CARTESIAN_POINT('Ctrl Pts',(22.2504817942136,15.3394353140274,37.771878106361));
#58835=CARTESIAN_POINT('Ctrl Pts',(20.949766380395,15.4651581089465,36.0335353606114));
#58836=CARTESIAN_POINT('Ctrl Pts',(18.7835013792615,15.5908809038656,36.1784216412247));
#58837=CARTESIAN_POINT('Ctrl Pts',(17.7258667749119,15.7166036987847,38.0744978878796));
#58838=CARTESIAN_POINT('Ctrl Pts',(18.740715588701,15.8423264937037,39.9938149473038));
#58839=CARTESIAN_POINT('Ctrl Pts',(20.9031867283705,15.9680492886228,40.1872436409934));
#58840=CARTESIAN_POINT('Ctrl Pts',(22.2425576655626,16.0937720835419,38.4785068028433));
#58841=CARTESIAN_POINT('Ctrl Pts',(21.5382209057625,16.219494878461,36.4248257618243));
#58842=CARTESIAN_POINT('Ctrl Pts',(19.43205892066,16.34521767338,35.8977794811667));
#58843=CARTESIAN_POINT('Ctrl Pts',(17.8434780765507,16.4709404682991,37.3776804883882));
#58844=CARTESIAN_POINT('Ctrl Pts',(18.2201980678962,16.5966632632182,39.5158521694202));
#58845=CARTESIAN_POINT('Ctrl Pts',(20.2189030648533,16.7223860581373,40.363716795752));
#58846=CARTESIAN_POINT('Ctrl Pts',(22.0181153640725,16.8481088530564,39.1485907974356));
#58847=CARTESIAN_POINT('Ctrl Pts',(21.9781607306821,16.9738316479754,36.9778536607199));
#58848=CARTESIAN_POINT('Ctrl Pts',(20.1354509783197,17.0995544428945,35.829760956277));
#58849=CARTESIAN_POINT('Ctrl Pts',(18.1693008296599,17.2252772378136,36.7506027898027));
#58850=CARTESIAN_POINT('Ctrl Pts',(17.8715198127086,17.3510000327327,38.9011893505787));
#58851=CARTESIAN_POINT('Ctrl Pts',(19.5134843855647,17.4767228276518,40.3216288709148));
#58852=CARTESIAN_POINT('Ctrl Pts',(21.5988247169108,17.6024456225708,39.7174337104706));
#58853=CARTESIAN_POINT('Ctrl Pts',(22.2271098160703,17.7281684174899,37.6392244034891));
#58854=CARTESIAN_POINT('Ctrl Pts',(20.8257652905152,17.853891212409,35.9809332317864));
#58855=CARTESIAN_POINT('Ctrl Pts',(18.6718769592704,17.9796140073281,36.2538089286721));
#58856=CARTESIAN_POINT('Ctrl Pts',(17.7283455889843,18.1053368022472,38.2091719749538));
#58857=CARTESIAN_POINT('Ctrl Pts',(18.8550386218625,18.2310595971662,40.0650434411737));
#58858=CARTESIAN_POINT('Ctrl Pts',(21.0251680921135,18.3567823920853,40.1301139539612));
#58859=CARTESIAN_POINT('Ctrl Pts',(22.2610322132312,18.4825051870044,38.3450828719222));
#58860=CARTESIAN_POINT('Ctrl Pts',(21.4363522472715,18.6082279819235,36.3367006764149));
#58861=CARTESIAN_POINT('Ctrl Pts',(19.3026829127495,18.7339507768426,35.9352641817039));
#58862=CARTESIAN_POINT('Ctrl Pts',(17.8044988185514,18.8596735717616,37.5066140827342));
#58863=CARTESIAN_POINT('Ctrl Pts',(18.3071384868509,18.9853963666807,39.6187337414808));
#58864=CARTESIAN_POINT('Ctrl Pts',(20.3525318386655,19.1111191615998,40.3467873924701));
#58865=CARTESIAN_POINT('Ctrl Pts',(22.0766527287437,19.2368419565189,39.0272786723744));
#58866=CARTESIAN_POINT('Ctrl Pts',(21.9082598828883,19.362564751438,36.8627140670674));
#58867=CARTESIAN_POINT('Ctrl Pts',(20.0008146007556,19.488287546357,35.825723931844));
#58868=CARTESIAN_POINT('Ctrl Pts',(18.0926269159133,19.6140103412761,36.8613474031311));
#58869=CARTESIAN_POINT('Ctrl Pts',(17.9226835840622,19.7397331361952,39.0257908087591));
#58870=CARTESIAN_POINT('Ctrl Pts',(19.6458586909056,19.8654559311143,40.3465343019432));
#58871=CARTESIAN_POINT('Ctrl Pts',(21.6917732645902,19.9911787260334,39.6199459917325));
#58872=CARTESIAN_POINT('Ctrl Pts',(22.195925432883,20.1169015209524,37.5081870742687));
#58873=CARTESIAN_POINT('Ctrl Pts',(20.6988681217534,20.2426243158715,35.9357640920978));
#58874=CARTESIAN_POINT('Ctrl Pts',(18.5649102950046,20.3683471107906,36.33567252362));
#58875=CARTESIAN_POINT('Ctrl Pts',(17.7387946796753,20.4940699057097,38.3434624768781));
#58876=CARTESIAN_POINT('Ctrl Pts',(18.9733742546723,20.6197927006287,40.1293802861978));
#58877=CARTESIAN_POINT('Ctrl Pts',(21.1435604747057,20.7455154955478,40.0658607403778));
#58878=CARTESIAN_POINT('Ctrl Pts',(22.2715619547167,20.8712382904669,38.2108038866874));
#58879=CARTESIAN_POINT('Ctrl Pts',(21.329471708329,20.996961085386,36.2547518236871));
#58880=CARTESIAN_POINT('Ctrl Pts',(19.1757015954905,21.1226838803051,35.9803596428606));
#58881=CARTESIAN_POINT('Ctrl Pts',(17.7733202900077,21.2484066752241,37.6375953974928));
#58882=CARTESIAN_POINT('Ctrl Pts',(18.3998242929215,21.3741294701433,39.7163533356445));
#58883=CARTESIAN_POINT('Ctrl Pts',(20.4852977349763,21.4998522650623,40.3218501519411));
#58884=CARTESIAN_POINT('Ctrl Pts',(22.1271794763833,21.6255750599814,38.9029594172551));
#58885=CARTESIAN_POINT('Ctrl Pts',(21.8330929452547,21.7512978549005,36.7514379862583));
#58886=CARTESIAN_POINT('Ctrl Pts',(19.8629761205629,21.8770354311873,35.8304875664748));
#58887=CARTESIAN_POINT('Ctrl Pts',(18.6408725645071,21.9608654091679,36.5934919535574));
#58888=CARTESIAN_POINT('Ctrl Pts',(18.3253725820279,22.002787788842,37.1492294200333));
#58889=CARTESIAN_POINT('Ctrl Pts',(21.0904144288932,0.125,36.00310066666));
#58890=CARTESIAN_POINT('Ctrl Pts',(21.103548660097,0.125,36.0100889715519));
#58891=CARTESIAN_POINT('Ctrl Pts',(21.1166828913007,0.125,36.0170772764437));
#58892=CARTESIAN_POINT('Ctrl Pts',(21.1298171225045,0.125,36.0240655813356));
#58893=CARTESIAN_POINT('Origin',(20.,0.125,38.1));
#58894=CARTESIAN_POINT('',(20.,-0.075,40.66347));
#58895=CARTESIAN_POINT('Origin',(20.,-0.075,38.1));
#58896=CARTESIAN_POINT('Origin',(20.,0.125,40.66347));
#58897=CARTESIAN_POINT('Origin',(20.,-0.075,38.1));
#58898=CARTESIAN_POINT('',(16.0376,-0.075,38.1));
#58899=CARTESIAN_POINT('Origin',(20.,-0.075,38.1));
#58900=CARTESIAN_POINT('Origin',(20.,21.95,38.1));
#58901=CARTESIAN_POINT('',(18.03653,22.15,38.1));
#58902=CARTESIAN_POINT('',(17.83653,21.95,38.1));
#58903=CARTESIAN_POINT('Origin',(20.,22.15,38.1));
#58904=CARTESIAN_POINT('Origin',(20.,22.15,38.1));
#58905=CARTESIAN_POINT('Origin',(24.2323742019726,-4.901,38.6431964418851));
#58906=CARTESIAN_POINT('',(23.9131875668744,-0.674999999999999,38.7225566853387));
#58907=CARTESIAN_POINT('',(23.9131875668744,-4.501,38.7225566853387));
#58908=CARTESIAN_POINT('',(23.9131875668744,-0.0750000000000001,38.7225566853387));
#58909=CARTESIAN_POINT('',(23.7544810775837,-0.674999999999999,38.7620163125374));
#58910=CARTESIAN_POINT('',(23.7544810775837,-0.674999999999999,38.7620163125374));
#58911=CARTESIAN_POINT('',(23.7544810775837,-4.651,38.7620163125374));
#58912=CARTESIAN_POINT('',(23.7544810775837,-4.901,38.7620163125374));
#58913=CARTESIAN_POINT('Ctrl Pts',(23.9131875668744,-4.50099999999998,38.7225566853387));
#58914=CARTESIAN_POINT('Ctrl Pts',(23.8323033520823,-4.57771996783978,38.7426671482203));
#58915=CARTESIAN_POINT('Ctrl Pts',(23.7544810775837,-4.651,38.7620163125374));
#58916=CARTESIAN_POINT('Origin',(23.7544810775837,-4.901,38.7620163125374));
#58917=CARTESIAN_POINT('',(23.8901204070909,-4.501,38.8533770492488));
#58918=CARTESIAN_POINT('Ctrl Pts',(23.7544810775837,-4.651,38.7620163125374));
#58919=CARTESIAN_POINT('Ctrl Pts',(23.82099229071,-4.57771996783967,38.8068153649425));
#58920=CARTESIAN_POINT('Ctrl Pts',(23.8901204070909,-4.50099999999998,38.8533770492489));
#58921=CARTESIAN_POINT('',(23.8901204070909,-0.674999999999999,38.8533770492488));
#58922=CARTESIAN_POINT('',(24.1629149309058,-0.674999999999999,39.03711954309));
#58923=CARTESIAN_POINT('',(23.8901204070909,-0.0750000000000001,38.8533770492488));
#58924=CARTESIAN_POINT('Origin',(23.9760628220115,-0.674999999999999,38.8010871525125));
#58925=CARTESIAN_POINT('Origin',(20.,-0.674999999999999,38.1));
#58926=CARTESIAN_POINT('Origin',(20.,-4.701,38.1));
#58927=CARTESIAN_POINT('',(16.1876,-4.651,38.1));
#58928=CARTESIAN_POINT('',(16.0381567112477,-4.501,38.0335807605545));
#58929=CARTESIAN_POINT('Ctrl Pts',(16.1876,-4.651,38.1));
#58930=CARTESIAN_POINT('Ctrl Pts',(16.1143199678399,-4.57771996783992,38.0674310968177));
#58931=CARTESIAN_POINT('Ctrl Pts',(16.0381567112477,-4.50099999999999,38.0335807605545));
#58932=CARTESIAN_POINT('',(16.0868124331256,-4.501,37.4774433146613));
#58933=CARTESIAN_POINT('Origin',(20.,-4.501,38.1));
#58934=CARTESIAN_POINT('',(16.2455189224163,-4.65100000000001,37.4379836874626));
#58935=CARTESIAN_POINT('Ctrl Pts',(16.0868124331256,-4.50099999999999,37.4774433146613));
#58936=CARTESIAN_POINT('Ctrl Pts',(16.1676966479178,-4.57771996783991,37.4573328517796));
#58937=CARTESIAN_POINT('Ctrl Pts',(16.2455189224163,-4.65100000000001,37.4379836874626));
#58938=CARTESIAN_POINT('',(16.1098795929091,-4.501,37.3466229507511));
#58939=CARTESIAN_POINT('Ctrl Pts',(16.2455189224163,-4.65100000000001,37.4379836874626));
#58940=CARTESIAN_POINT('Ctrl Pts',(16.1790077092902,-4.57771996783988,37.3931846350576));
#58941=CARTESIAN_POINT('Ctrl Pts',(16.1098795929091,-4.50099999999999,37.3466229507511));
#58942=CARTESIAN_POINT('',(16.2543683790546,-4.501,36.8073834597322));
#58943=CARTESIAN_POINT('Origin',(20.,-4.501,38.1));
#58944=CARTESIAN_POINT('',(16.4175158525158,-4.651,36.7960824055852));
#58945=CARTESIAN_POINT('Ctrl Pts',(16.2543683790546,-4.50099999999999,36.8073834597322));
#58946=CARTESIAN_POINT('Ctrl Pts',(16.3375159261096,-4.57771996783986,36.8016239164704));
#58947=CARTESIAN_POINT('Ctrl Pts',(16.4175158525158,-4.651,36.7960824055852));
#58948=CARTESIAN_POINT('',(16.299801814644,-4.501,36.682556121362));
#58949=CARTESIAN_POINT('Ctrl Pts',(16.4175158525158,-4.651,36.7960824055852));
#58950=CARTESIAN_POINT('Ctrl Pts',(16.3597943679782,-4.57771996783973,36.7404144004953));
#58951=CARTESIAN_POINT('Ctrl Pts',(16.299801814644,-4.50099999999999,36.682556121362));
#58952=CARTESIAN_POINT('',(16.5357334464049,-4.501,36.1765991042837));
#58953=CARTESIAN_POINT('Origin',(20.,-4.501,38.1));
#58954=CARTESIAN_POINT('',(16.6983647506122,-4.651,36.1938));
#58955=CARTESIAN_POINT('Ctrl Pts',(16.5357334464049,-4.50099999999999,36.1765991042837));
#58956=CARTESIAN_POINT('Ctrl Pts',(16.61861792958,-4.57771996783963,36.1853654814492));
#58957=CARTESIAN_POINT('Ctrl Pts',(16.6983647506122,-4.651,36.1938));
#58958=CARTESIAN_POINT('',(16.6021526858504,-4.501,36.0615576069641));
#58959=CARTESIAN_POINT('Ctrl Pts',(16.6983647506122,-4.651,36.1938));
#58960=CARTESIAN_POINT('Ctrl Pts',(16.6511868327625,-4.57771996783981,36.1289544863906));
#58961=CARTESIAN_POINT('Ctrl Pts',(16.6021526858504,-4.50099999999999,36.061557606964));
#58962=CARTESIAN_POINT('',(16.9223584999828,-4.501,35.6042563117636));
#58963=CARTESIAN_POINT('Origin',(20.,-4.501,38.1));
#58964=CARTESIAN_POINT('',(17.0795321650532,-4.651,35.649436516831));
#58965=CARTESIAN_POINT('Ctrl Pts',(16.9223584999827,-4.50099999999999,35.6042563117636));
#58966=CARTESIAN_POINT('Ctrl Pts',(17.0024615161987,-4.57771996783983,35.6272822474223));
#58967=CARTESIAN_POINT('Ctrl Pts',(17.0795321650532,-4.651,35.649436516831));
#58968=CARTESIAN_POINT('',(17.0077454283034,-4.501,35.5024961331769));
#58969=CARTESIAN_POINT('Ctrl Pts',(17.0795321650532,-4.651,35.649436516831));
#58970=CARTESIAN_POINT('Ctrl Pts',(17.0443312910519,-4.57771996783965,35.5773837928196));
#58971=CARTESIAN_POINT('Ctrl Pts',(17.0077454283034,-4.50099999999999,35.5024961331769));
#58972=CARTESIAN_POINT('',(17.4024961331769,-4.501,35.1077454283034));
#58973=CARTESIAN_POINT('Origin',(20.,-4.501,38.1));
#58974=CARTESIAN_POINT('',(17.549436516831,-4.651,35.1795321650532));
#58975=CARTESIAN_POINT('Ctrl Pts',(17.4024961331769,-4.50099999999999,35.1077454283034));
#58976=CARTESIAN_POINT('Ctrl Pts',(17.4773837928199,-4.57771996783995,35.1443312910521));
#58977=CARTESIAN_POINT('Ctrl Pts',(17.549436516831,-4.651,35.1795321650532));
#58978=CARTESIAN_POINT('',(17.5042563117636,-4.501,35.0223584999828));
#58979=CARTESIAN_POINT('Ctrl Pts',(17.549436516831,-4.651,35.1795321650532));
#58980=CARTESIAN_POINT('Ctrl Pts',(17.5272822474223,-4.57771996783968,35.1024615161985));
#58981=CARTESIAN_POINT('Ctrl Pts',(17.5042563117636,-4.501,35.0223584999827));
#58982=CARTESIAN_POINT('',(17.961557606964,-4.501,34.7021526858504));
#58983=CARTESIAN_POINT('Origin',(20.,-4.501,38.1));
#58984=CARTESIAN_POINT('',(18.0938,-4.651,34.7983647506122));
#58985=CARTESIAN_POINT('Ctrl Pts',(17.961557606964,-4.501,34.7021526858504));
#58986=CARTESIAN_POINT('Ctrl Pts',(18.0289544863906,-4.57771996783974,34.7511868327624));
#58987=CARTESIAN_POINT('Ctrl Pts',(18.0938,-4.651,34.7983647506122));
#58988=CARTESIAN_POINT('',(18.0765991042837,-4.501,34.6357334464049));
#58989=CARTESIAN_POINT('Ctrl Pts',(18.0938,-4.651,34.7983647506122));
#58990=CARTESIAN_POINT('Ctrl Pts',(18.0853654814492,-4.57771996783983,34.7186179295802));
#58991=CARTESIAN_POINT('Ctrl Pts',(18.0765991042837,-4.50099999999999,34.6357334464049));
#58992=CARTESIAN_POINT('',(18.582556121362,-4.501,34.399801814644));
#58993=CARTESIAN_POINT('Origin',(20.,-4.501,38.1));
#58994=CARTESIAN_POINT('',(18.6960824055852,-4.65100000000001,34.5175158525158));
#58995=CARTESIAN_POINT('Ctrl Pts',(18.582556121362,-4.50099999999999,34.399801814644));
#58996=CARTESIAN_POINT('Ctrl Pts',(18.6404144004955,-4.57771996784003,34.4597943679785));
#58997=CARTESIAN_POINT('Ctrl Pts',(18.6960824055852,-4.65100000000001,34.5175158525158));
#58998=CARTESIAN_POINT('',(18.7073834597322,-4.501,34.3543683790546));
#58999=CARTESIAN_POINT('Ctrl Pts',(18.6960824055852,-4.65100000000001,34.5175158525158));
#59000=CARTESIAN_POINT('Ctrl Pts',(18.7016239164704,-4.57771996783996,34.4375159261097));
#59001=CARTESIAN_POINT('Ctrl Pts',(18.7073834597322,-4.501,34.3543683790546));
#59002=CARTESIAN_POINT('',(19.2466229507512,-4.501,34.2098795929091));
#59003=CARTESIAN_POINT('Origin',(20.,-4.501,38.1));
#59004=CARTESIAN_POINT('',(19.3379836874626,-4.651,34.3455189224163));
#59005=CARTESIAN_POINT('Ctrl Pts',(19.2466229507511,-4.501,34.2098795929091));
#59006=CARTESIAN_POINT('Ctrl Pts',(19.2931846350574,-4.57771996783949,34.2790077092898));
#59007=CARTESIAN_POINT('Ctrl Pts',(19.3379836874626,-4.651,34.3455189224163));
#59008=CARTESIAN_POINT('',(19.3774433146613,-4.501,34.1868124331256));
#59009=CARTESIAN_POINT('Ctrl Pts',(19.3379836874626,-4.651,34.3455189224163));
#59010=CARTESIAN_POINT('Ctrl Pts',(19.3573328517797,-4.57771996783973,34.2676966479176));
#59011=CARTESIAN_POINT('Ctrl Pts',(19.3774433146613,-4.501,34.1868124331256));
#59012=CARTESIAN_POINT('',(19.9335807605545,-4.501,34.1381567112477));
#59013=CARTESIAN_POINT('Origin',(20.,-4.501,38.1));
#59014=CARTESIAN_POINT('',(20.,-4.65100000000001,34.2876));
#59015=CARTESIAN_POINT('Ctrl Pts',(19.9335807605545,-4.501,34.1381567112477));
#59016=CARTESIAN_POINT('Ctrl Pts',(19.9674310968175,-4.57771996783948,34.2143199678395));
#59017=CARTESIAN_POINT('Ctrl Pts',(20.,-4.65100000000001,34.2876));
#59018=CARTESIAN_POINT('',(20.0664192394455,-4.501,34.1381567112477));
#59019=CARTESIAN_POINT('Ctrl Pts',(20.,-4.65100000000001,34.2876));
#59020=CARTESIAN_POINT('Ctrl Pts',(20.0325689031823,-4.57771996783993,34.2143199678399));
#59021=CARTESIAN_POINT('Ctrl Pts',(20.0664192394455,-4.501,34.1381567112477));
#59022=CARTESIAN_POINT('',(20.6225566853387,-4.501,34.1868124331256));
#59023=CARTESIAN_POINT('Origin',(20.,-4.501,38.1));
#59024=CARTESIAN_POINT('',(20.6620163125374,-4.651,34.3455189224163));
#59025=CARTESIAN_POINT('Ctrl Pts',(20.6225566853387,-4.501,34.1868124331256));
#59026=CARTESIAN_POINT('Ctrl Pts',(20.6426671482203,-4.57771996783972,34.2676966479176));
#59027=CARTESIAN_POINT('Ctrl Pts',(20.6620163125374,-4.651,34.3455189224163));
#59028=CARTESIAN_POINT('',(20.7533770492488,-4.501,34.2098795929091));
#59029=CARTESIAN_POINT('Ctrl Pts',(20.6620163125374,-4.651,34.3455189224163));
#59030=CARTESIAN_POINT('Ctrl Pts',(20.7068153649425,-4.57771996783977,34.2790077092901));
#59031=CARTESIAN_POINT('Ctrl Pts',(20.7533770492489,-4.501,34.2098795929091));
#59032=CARTESIAN_POINT('',(21.2926165402678,-4.501,34.3543683790546));
#59033=CARTESIAN_POINT('Origin',(20.,-4.501,38.1));
#59034=CARTESIAN_POINT('',(21.3039175944148,-4.65100000000001,34.5175158525158));
#59035=CARTESIAN_POINT('Ctrl Pts',(21.2926165402678,-4.501,34.3543683790546));
#59036=CARTESIAN_POINT('Ctrl Pts',(21.2983760835296,-4.57771996783983,34.4375159261096));
#59037=CARTESIAN_POINT('Ctrl Pts',(21.3039175944148,-4.65100000000001,34.5175158525158));
#59038=CARTESIAN_POINT('',(21.417443878638,-4.501,34.399801814644));
#59039=CARTESIAN_POINT('Ctrl Pts',(21.3039175944148,-4.65100000000001,34.5175158525158));
#59040=CARTESIAN_POINT('Ctrl Pts',(21.3595855995048,-4.57771996783964,34.4597943679781));
#59041=CARTESIAN_POINT('Ctrl Pts',(21.417443878638,-4.501,34.399801814644));
#59042=CARTESIAN_POINT('',(21.9234008957163,-4.501,34.6357334464049));
#59043=CARTESIAN_POINT('Origin',(20.,-4.501,38.1));
#59044=CARTESIAN_POINT('',(21.9062,-4.651,34.7983647506122));
#59045=CARTESIAN_POINT('Ctrl Pts',(21.9234008957163,-4.501,34.6357334464049));
#59046=CARTESIAN_POINT('Ctrl Pts',(21.9146345185508,-4.57771996784004,34.7186179295804));
#59047=CARTESIAN_POINT('Ctrl Pts',(21.9062,-4.651,34.7983647506122));
#59048=CARTESIAN_POINT('',(22.038442393036,-4.501,34.7021526858504));
#59049=CARTESIAN_POINT('Ctrl Pts',(21.9062,-4.651,34.7983647506122));
#59050=CARTESIAN_POINT('Ctrl Pts',(21.9710455136096,-4.57771996783961,34.7511868327624));
#59051=CARTESIAN_POINT('Ctrl Pts',(22.038442393036,-4.501,34.7021526858504));
#59052=CARTESIAN_POINT('',(22.4957436882363,-4.501,35.0223584999827));
#59053=CARTESIAN_POINT('Origin',(20.,-4.501,38.1));
#59054=CARTESIAN_POINT('',(22.450563483169,-4.651,35.1795321650532));
#59055=CARTESIAN_POINT('Ctrl Pts',(22.4957436882364,-4.501,35.0223584999827));
#59056=CARTESIAN_POINT('Ctrl Pts',(22.4727177525778,-4.57771996783958,35.1024615161984));
#59057=CARTESIAN_POINT('Ctrl Pts',(22.450563483169,-4.651,35.1795321650532));
#59058=CARTESIAN_POINT('',(22.5975038668231,-4.501,35.1077454283034));
#59059=CARTESIAN_POINT('Ctrl Pts',(22.450563483169,-4.651,35.1795321650532));
#59060=CARTESIAN_POINT('Ctrl Pts',(22.5226162071807,-4.57771996783934,35.1443312910517));
#59061=CARTESIAN_POINT('Ctrl Pts',(22.5975038668231,-4.501,35.1077454283034));
#59062=CARTESIAN_POINT('',(22.9922545716966,-4.501,35.5024961331769));
#59063=CARTESIAN_POINT('Origin',(20.,-4.501,38.1));
#59064=CARTESIAN_POINT('',(22.9204678349468,-4.651,35.649436516831));
#59065=CARTESIAN_POINT('Ctrl Pts',(22.9922545716966,-4.501,35.5024961331769));
#59066=CARTESIAN_POINT('Ctrl Pts',(22.9556687089481,-4.57771996783959,35.5773837928195));
#59067=CARTESIAN_POINT('Ctrl Pts',(22.9204678349468,-4.651,35.649436516831));
#59068=CARTESIAN_POINT('',(23.0776415000172,-4.501,35.6042563117636));
#59069=CARTESIAN_POINT('Ctrl Pts',(22.9204678349468,-4.651,35.649436516831));
#59070=CARTESIAN_POINT('Ctrl Pts',(22.9975384838016,-4.57771996783957,35.6272822474222));
#59071=CARTESIAN_POINT('Ctrl Pts',(23.0776415000173,-4.501,35.6042563117636));
#59072=CARTESIAN_POINT('',(23.3978473141496,-4.501,36.061557606964));
#59073=CARTESIAN_POINT('Origin',(20.,-4.501,38.1));
#59074=CARTESIAN_POINT('',(23.3016352493878,-4.651,36.1938));
#59075=CARTESIAN_POINT('Ctrl Pts',(23.3978473141496,-4.501,36.061557606964));
#59076=CARTESIAN_POINT('Ctrl Pts',(23.3488131672376,-4.5777199678397,36.1289544863905));
#59077=CARTESIAN_POINT('Ctrl Pts',(23.3016352493878,-4.651,36.1938));
#59078=CARTESIAN_POINT('',(23.4642665535951,-4.501,36.1765991042837));
#59079=CARTESIAN_POINT('Ctrl Pts',(23.3016352493878,-4.651,36.1938));
#59080=CARTESIAN_POINT('Ctrl Pts',(23.3813820704202,-4.57771996783943,36.1853654814491));
#59081=CARTESIAN_POINT('Ctrl Pts',(23.4642665535951,-4.501,36.1765991042837));
#59082=CARTESIAN_POINT('',(23.700198185356,-4.501,36.682556121362));
#59083=CARTESIAN_POINT('Origin',(20.,-4.501,38.1));
#59084=CARTESIAN_POINT('',(23.5824841474842,-4.651,36.7960824055852));
#59085=CARTESIAN_POINT('Ctrl Pts',(23.700198185356,-4.501,36.682556121362));
#59086=CARTESIAN_POINT('Ctrl Pts',(23.6402056320216,-4.57771996784001,36.7404144004955));
#59087=CARTESIAN_POINT('Ctrl Pts',(23.5824841474842,-4.651,36.7960824055852));
#59088=CARTESIAN_POINT('',(23.7456316209454,-4.501,36.8073834597322));
#59089=CARTESIAN_POINT('Ctrl Pts',(23.5824841474842,-4.651,36.7960824055852));
#59090=CARTESIAN_POINT('Ctrl Pts',(23.6624840738904,-4.57771996783986,36.8016239164704));
#59091=CARTESIAN_POINT('Ctrl Pts',(23.7456316209454,-4.501,36.8073834597322));
#59092=CARTESIAN_POINT('',(23.8901204070909,-4.501,37.3466229507511));
#59093=CARTESIAN_POINT('Origin',(20.,-4.501,38.1));
#59094=CARTESIAN_POINT('',(23.7544810775837,-4.651,37.4379836874626));
#59095=CARTESIAN_POINT('Ctrl Pts',(23.8901204070909,-4.501,37.3466229507511));
#59096=CARTESIAN_POINT('Ctrl Pts',(23.8209922907099,-4.57771996783982,37.3931846350576));
#59097=CARTESIAN_POINT('Ctrl Pts',(23.7544810775837,-4.651,37.4379836874626));
#59098=CARTESIAN_POINT('',(23.9131875668744,-4.501,37.4774433146613));
#59099=CARTESIAN_POINT('Ctrl Pts',(23.7544810775837,-4.651,37.4379836874626));
#59100=CARTESIAN_POINT('Ctrl Pts',(23.8323033520825,-4.57771996783966,37.4573328517797));
#59101=CARTESIAN_POINT('Ctrl Pts',(23.9131875668744,-4.501,37.4774433146613));
#59102=CARTESIAN_POINT('',(23.9618432887523,-4.501,38.0335807605545));
#59103=CARTESIAN_POINT('Origin',(20.,-4.501,38.1));
#59104=CARTESIAN_POINT('',(23.8124,-4.651,38.1));
#59105=CARTESIAN_POINT('Ctrl Pts',(23.9618432887523,-4.501,38.0335807605545));
#59106=CARTESIAN_POINT('Ctrl Pts',(23.8856800321604,-4.57771996783957,38.0674310968176));
#59107=CARTESIAN_POINT('Ctrl Pts',(23.8124,-4.651,38.1));
#59108=CARTESIAN_POINT('',(23.9618432887523,-4.501,38.1664192394455));
#59109=CARTESIAN_POINT('Ctrl Pts',(23.8124,-4.651,38.1));
#59110=CARTESIAN_POINT('Ctrl Pts',(23.8856800321601,-4.57771996783995,38.1325689031822));
#59111=CARTESIAN_POINT('Ctrl Pts',(23.9618432887523,-4.501,38.1664192394455));
#59112=CARTESIAN_POINT('Origin',(20.,-4.501,38.1));
#59113=CARTESIAN_POINT('',(23.7456316209454,-4.501,39.3926165402678));
#59114=CARTESIAN_POINT('Origin',(20.,-4.501,38.1));
#59115=CARTESIAN_POINT('',(23.5824841474842,-4.65100000000001,39.4039175944148));
#59116=CARTESIAN_POINT('Ctrl Pts',(23.7456316209454,-4.50099999999998,39.3926165402678));
#59117=CARTESIAN_POINT('Ctrl Pts',(23.6624840738902,-4.57771996784001,39.3983760835296));
#59118=CARTESIAN_POINT('Ctrl Pts',(23.5824841474842,-4.65100000000001,39.4039175944148));
#59119=CARTESIAN_POINT('',(23.700198185356,-4.501,39.517443878638));
#59120=CARTESIAN_POINT('Ctrl Pts',(23.5824841474842,-4.65100000000001,39.4039175944148));
#59121=CARTESIAN_POINT('Ctrl Pts',(23.6402056320216,-4.57771996783998,39.4595855995045));
#59122=CARTESIAN_POINT('Ctrl Pts',(23.700198185356,-4.50099999999998,39.517443878638));
#59123=CARTESIAN_POINT('',(23.4642665535951,-4.501,40.0234008957163));
#59124=CARTESIAN_POINT('Origin',(20.,-4.501,38.1));
#59125=CARTESIAN_POINT('',(23.3016352493878,-4.651,40.0062));
#59126=CARTESIAN_POINT('Ctrl Pts',(23.4642665535951,-4.50099999999998,40.0234008957163));
#59127=CARTESIAN_POINT('Ctrl Pts',(23.3813820704201,-4.57771996783958,40.0146345185508));
#59128=CARTESIAN_POINT('Ctrl Pts',(23.3016352493878,-4.651,40.0062));
#59129=CARTESIAN_POINT('',(23.3978473141496,-4.501,40.1384423930359));
#59130=CARTESIAN_POINT('Ctrl Pts',(23.3016352493878,-4.651,40.0062));
#59131=CARTESIAN_POINT('Ctrl Pts',(23.3488131672377,-4.57771996783948,40.0710455136097));
#59132=CARTESIAN_POINT('Ctrl Pts',(23.3978473141496,-4.50099999999999,40.138442393036));
#59133=CARTESIAN_POINT('',(23.0776415000172,-4.501,40.5957436882364));
#59134=CARTESIAN_POINT('Origin',(20.,-4.501,38.1));
#59135=CARTESIAN_POINT('',(22.9204678349468,-4.651,40.550563483169));
#59136=CARTESIAN_POINT('Ctrl Pts',(23.0776415000173,-4.50099999999999,40.5957436882364));
#59137=CARTESIAN_POINT('Ctrl Pts',(22.9975384838016,-4.5777199678396,40.5727177525777));
#59138=CARTESIAN_POINT('Ctrl Pts',(22.9204678349468,-4.651,40.550563483169));
#59139=CARTESIAN_POINT('',(22.9922545716966,-4.501,40.6975038668231));
#59140=CARTESIAN_POINT('Ctrl Pts',(22.9204678349468,-4.651,40.550563483169));
#59141=CARTESIAN_POINT('Ctrl Pts',(22.955668708948,-4.57771996783992,40.6226162071801));
#59142=CARTESIAN_POINT('Ctrl Pts',(22.9922545716966,-4.50099999999998,40.6975038668231));
#59143=CARTESIAN_POINT('',(22.5975038668231,-4.501,41.0922545716966));
#59144=CARTESIAN_POINT('Origin',(20.,-4.501,38.1));
#59145=CARTESIAN_POINT('',(22.450563483169,-4.65100000000001,41.0204678349468));
#59146=CARTESIAN_POINT('Ctrl Pts',(22.5975038668231,-4.50099999999999,41.0922545716966));
#59147=CARTESIAN_POINT('Ctrl Pts',(22.5226162071807,-4.57771996783933,41.0556687089482));
#59148=CARTESIAN_POINT('Ctrl Pts',(22.450563483169,-4.65100000000001,41.0204678349468));
#59149=CARTESIAN_POINT('',(22.4957436882364,-4.501,41.1776415000172));
#59150=CARTESIAN_POINT('Ctrl Pts',(22.450563483169,-4.65100000000001,41.0204678349468));
#59151=CARTESIAN_POINT('Ctrl Pts',(22.4727177525775,-4.57771996784042,41.0975384838007));
#59152=CARTESIAN_POINT('Ctrl Pts',(22.4957436882364,-4.50099999999999,41.1776415000173));
#59153=CARTESIAN_POINT('',(22.038442393036,-4.501,41.4978473141496));
#59154=CARTESIAN_POINT('Origin',(20.,-4.501,38.1));
#59155=CARTESIAN_POINT('',(21.9062,-4.651,41.4016352493878));
#59156=CARTESIAN_POINT('Ctrl Pts',(22.038442393036,-4.50099999999999,41.4978473141496));
#59157=CARTESIAN_POINT('Ctrl Pts',(21.9710455136096,-4.57771996783954,41.4488131672377));
#59158=CARTESIAN_POINT('Ctrl Pts',(21.9062,-4.651,41.4016352493878));
#59159=CARTESIAN_POINT('',(21.9234008957163,-4.501,41.5642665535951));
#59160=CARTESIAN_POINT('Ctrl Pts',(21.9062,-4.651,41.4016352493878));
#59161=CARTESIAN_POINT('Ctrl Pts',(21.9146345185508,-4.57771996784014,41.4813820704194));
#59162=CARTESIAN_POINT('Ctrl Pts',(21.9234008957163,-4.50099999999999,41.5642665535951));
#59163=CARTESIAN_POINT('',(21.417443878638,-4.501,41.800198185356));
#59164=CARTESIAN_POINT('Origin',(20.,-4.501,38.1));
#59165=CARTESIAN_POINT('',(21.3039175944148,-4.65100000000001,41.6824841474842));
#59166=CARTESIAN_POINT('Ctrl Pts',(21.417443878638,-4.50099999999999,41.800198185356));
#59167=CARTESIAN_POINT('Ctrl Pts',(21.3595855995046,-4.57771996783985,41.7402056320217));
#59168=CARTESIAN_POINT('Ctrl Pts',(21.3039175944148,-4.65100000000001,41.6824841474842));
#59169=CARTESIAN_POINT('',(21.2926165402678,-4.501,41.8456316209454));
#59170=CARTESIAN_POINT('Ctrl Pts',(21.3039175944148,-4.65100000000001,41.6824841474842));
#59171=CARTESIAN_POINT('Ctrl Pts',(21.2983760835296,-4.57771996783928,41.762484073891));
#59172=CARTESIAN_POINT('Ctrl Pts',(21.2926165402678,-4.50099999999999,41.8456316209454));
#59173=CARTESIAN_POINT('',(20.7533770492488,-4.501,41.9901204070909));
#59174=CARTESIAN_POINT('Origin',(20.,-4.501,38.1));
#59175=CARTESIAN_POINT('',(20.6620163125374,-4.651,41.8544810775837));
#59176=CARTESIAN_POINT('Ctrl Pts',(20.7533770492489,-4.50099999999999,41.9901204070909));
#59177=CARTESIAN_POINT('Ctrl Pts',(20.7068153649426,-4.57771996783958,41.9209922907101));
#59178=CARTESIAN_POINT('Ctrl Pts',(20.6620163125374,-4.651,41.8544810775837));
#59179=CARTESIAN_POINT('',(20.6225566853387,-4.501,42.0131875668744));
#59180=CARTESIAN_POINT('Ctrl Pts',(20.6620163125374,-4.651,41.8544810775837));
#59181=CARTESIAN_POINT('Ctrl Pts',(20.6426671482204,-4.57771996783993,41.9323033520822));
#59182=CARTESIAN_POINT('Ctrl Pts',(20.6225566853387,-4.50099999999999,42.0131875668744));
#59183=CARTESIAN_POINT('',(20.0664192394455,-4.501,42.0618432887523));
#59184=CARTESIAN_POINT('Origin',(20.,-4.501,38.1));
#59185=CARTESIAN_POINT('',(20.,-4.651,41.9124));
#59186=CARTESIAN_POINT('Ctrl Pts',(20.0664192394455,-4.50099999999999,42.0618432887523));
#59187=CARTESIAN_POINT('Ctrl Pts',(20.0325689031823,-4.5777199678398,41.9856800321602));
#59188=CARTESIAN_POINT('Ctrl Pts',(20.,-4.651,41.9124));
#59189=CARTESIAN_POINT('',(19.9335807605545,-4.501,42.0618432887523));
#59190=CARTESIAN_POINT('Ctrl Pts',(20.,-4.651,41.9124));
#59191=CARTESIAN_POINT('Ctrl Pts',(19.9674310968177,-4.57771996783988,41.9856800321601));
#59192=CARTESIAN_POINT('Ctrl Pts',(19.9335807605545,-4.50099999999999,42.0618432887523));
#59193=CARTESIAN_POINT('',(19.3774433146613,-4.501,42.0131875668744));
#59194=CARTESIAN_POINT('Origin',(20.,-4.501,38.1));
#59195=CARTESIAN_POINT('',(19.3379836874626,-4.651,41.8544810775837));
#59196=CARTESIAN_POINT('Ctrl Pts',(19.3774433146613,-4.50099999999999,42.0131875668744));
#59197=CARTESIAN_POINT('Ctrl Pts',(19.3573328517796,-4.57771996784008,41.932303352082));
#59198=CARTESIAN_POINT('Ctrl Pts',(19.3379836874626,-4.651,41.8544810775837));
#59199=CARTESIAN_POINT('',(19.2466229507511,-4.501,41.9901204070909));
#59200=CARTESIAN_POINT('Ctrl Pts',(19.3379836874626,-4.651,41.8544810775837));
#59201=CARTESIAN_POINT('Ctrl Pts',(19.2931846350574,-4.57771996783954,41.9209922907101));
#59202=CARTESIAN_POINT('Ctrl Pts',(19.2466229507511,-4.50099999999999,41.9901204070909));
#59203=CARTESIAN_POINT('',(18.7073834597322,-4.501,41.8456316209454));
#59204=CARTESIAN_POINT('Origin',(20.,-4.501,38.1));
#59205=CARTESIAN_POINT('',(18.6960824055852,-4.65100000000001,41.6824841474842));
#59206=CARTESIAN_POINT('Ctrl Pts',(18.7073834597322,-4.50099999999999,41.8456316209454));
#59207=CARTESIAN_POINT('Ctrl Pts',(18.7016239164704,-4.57771996784026,41.76248407389));
#59208=CARTESIAN_POINT('Ctrl Pts',(18.6960824055852,-4.65100000000001,41.6824841474842));
#59209=CARTESIAN_POINT('',(18.582556121362,-4.501,41.800198185356));
#59210=CARTESIAN_POINT('Ctrl Pts',(18.6960824055852,-4.65100000000001,41.6824841474842));
#59211=CARTESIAN_POINT('Ctrl Pts',(18.6404144004953,-4.57771996783977,41.7402056320217));
#59212=CARTESIAN_POINT('Ctrl Pts',(18.582556121362,-4.50099999999999,41.800198185356));
#59213=CARTESIAN_POINT('',(18.0765991042837,-4.501,41.5642665535951));
#59214=CARTESIAN_POINT('Origin',(20.,-4.501,38.1));
#59215=CARTESIAN_POINT('',(18.0938,-4.651,41.4016352493878));
#59216=CARTESIAN_POINT('Ctrl Pts',(18.0765991042837,-4.50099999999999,41.5642665535951));
#59217=CARTESIAN_POINT('Ctrl Pts',(18.0853654814492,-4.57771996783993,41.4813820704197));
#59218=CARTESIAN_POINT('Ctrl Pts',(18.0938,-4.651,41.4016352493878));
#59219=CARTESIAN_POINT('',(17.961557606964,-4.501,41.4978473141496));
#59220=CARTESIAN_POINT('Ctrl Pts',(18.0938,-4.651,41.4016352493878));
#59221=CARTESIAN_POINT('Ctrl Pts',(18.0289544863912,-4.57771996784051,41.448813167237));
#59222=CARTESIAN_POINT('Ctrl Pts',(17.961557606964,-4.50099999999999,41.4978473141496));
#59223=CARTESIAN_POINT('',(17.5042563117637,-4.501,41.1776415000173));
#59224=CARTESIAN_POINT('Origin',(20.,-4.501,38.1));
#59225=CARTESIAN_POINT('',(17.549436516831,-4.65100000000001,41.0204678349468));
#59226=CARTESIAN_POINT('Ctrl Pts',(17.5042563117636,-4.50099999999999,41.1776415000173));
#59227=CARTESIAN_POINT('Ctrl Pts',(17.5272822474223,-4.57771996783969,41.0975384838015));
#59228=CARTESIAN_POINT('Ctrl Pts',(17.549436516831,-4.65100000000001,41.0204678349468));
#59229=CARTESIAN_POINT('',(17.4024961331769,-4.501,41.0922545716966));
#59230=CARTESIAN_POINT('Ctrl Pts',(17.549436516831,-4.65100000000001,41.0204678349468));
#59231=CARTESIAN_POINT('Ctrl Pts',(17.4773837928199,-4.57771996783993,41.055668708948));
#59232=CARTESIAN_POINT('Ctrl Pts',(17.4024961331769,-4.50099999999999,41.0922545716966));
#59233=CARTESIAN_POINT('',(17.0077454283034,-4.501,40.6975038668231));
#59234=CARTESIAN_POINT('Origin',(20.,-4.501,38.1));
#59235=CARTESIAN_POINT('',(17.0795321650532,-4.651,40.550563483169));
#59236=CARTESIAN_POINT('Ctrl Pts',(17.0077454283034,-4.50099999999999,40.6975038668231));
#59237=CARTESIAN_POINT('Ctrl Pts',(17.044331291052,-4.57771996783985,40.6226162071802));
#59238=CARTESIAN_POINT('Ctrl Pts',(17.0795321650532,-4.651,40.550563483169));
#59239=CARTESIAN_POINT('',(16.9223584999828,-4.501,40.5957436882364));
#59240=CARTESIAN_POINT('Ctrl Pts',(17.0795321650532,-4.651,40.550563483169));
#59241=CARTESIAN_POINT('Ctrl Pts',(17.0024615161981,-4.57771996783934,40.5727177525778));
#59242=CARTESIAN_POINT('Ctrl Pts',(16.9223584999827,-4.50099999999999,40.5957436882364));
#59243=CARTESIAN_POINT('',(16.6021526858504,-4.501,40.1384423930359));
#59244=CARTESIAN_POINT('Origin',(20.,-4.501,38.1));
#59245=CARTESIAN_POINT('',(16.6983647506122,-4.65100000000001,40.0062));
#59246=CARTESIAN_POINT('Ctrl Pts',(16.6021526858504,-4.50099999999999,40.1384423930359));
#59247=CARTESIAN_POINT('Ctrl Pts',(16.6511868327624,-4.57771996783963,40.0710455136095));
#59248=CARTESIAN_POINT('Ctrl Pts',(16.6983647506122,-4.65100000000001,40.0062));
#59249=CARTESIAN_POINT('',(16.5357334464049,-4.501,40.0234008957163));
#59250=CARTESIAN_POINT('Ctrl Pts',(16.6983647506122,-4.65100000000001,40.0062));
#59251=CARTESIAN_POINT('Ctrl Pts',(16.6186179295803,-4.57771996783988,40.0146345185508));
#59252=CARTESIAN_POINT('Ctrl Pts',(16.5357334464049,-4.50099999999999,40.0234008957163));
#59253=CARTESIAN_POINT('',(16.299801814644,-4.501,39.517443878638));
#59254=CARTESIAN_POINT('Origin',(20.,-4.501,38.1));
#59255=CARTESIAN_POINT('',(16.4175158525158,-4.651,39.4039175944148));
#59256=CARTESIAN_POINT('Ctrl Pts',(16.299801814644,-4.50099999999999,39.517443878638));
#59257=CARTESIAN_POINT('Ctrl Pts',(16.3597943679784,-4.57771996783994,39.4595855995045));
#59258=CARTESIAN_POINT('Ctrl Pts',(16.4175158525158,-4.651,39.4039175944148));
#59259=CARTESIAN_POINT('',(16.2543683790546,-4.501,39.3926165402678));
#59260=CARTESIAN_POINT('Ctrl Pts',(16.4175158525158,-4.651,39.4039175944148));
#59261=CARTESIAN_POINT('Ctrl Pts',(16.3375159261095,-4.57771996783976,39.3983760835296));
#59262=CARTESIAN_POINT('Ctrl Pts',(16.2543683790546,-4.50099999999999,39.3926165402678));
#59263=CARTESIAN_POINT('',(16.1098795929091,-4.501,38.8533770492488));
#59264=CARTESIAN_POINT('Origin',(20.,-4.501,38.1));
#59265=CARTESIAN_POINT('',(16.2455189224163,-4.651,38.7620163125374));
#59266=CARTESIAN_POINT('Ctrl Pts',(16.1098795929091,-4.50099999999999,38.8533770492489));
#59267=CARTESIAN_POINT('Ctrl Pts',(16.1790077092901,-4.57771996783979,38.8068153649424));
#59268=CARTESIAN_POINT('Ctrl Pts',(16.2455189224163,-4.651,38.7620163125374));
#59269=CARTESIAN_POINT('',(16.0868124331256,-4.501,38.7225566853387));
#59270=CARTESIAN_POINT('Ctrl Pts',(16.2455189224163,-4.651,38.7620163125374));
#59271=CARTESIAN_POINT('Ctrl Pts',(16.1676966479176,-4.5777199678397,38.7426671482203));
#59272=CARTESIAN_POINT('Ctrl Pts',(16.0868124331256,-4.50099999999999,38.7225566853387));
#59273=CARTESIAN_POINT('',(16.0381567112477,-4.501,38.1664192394455));
#59274=CARTESIAN_POINT('Origin',(20.,-4.501,38.1));
#59275=CARTESIAN_POINT('Ctrl Pts',(16.0381567112477,-4.50099999999999,38.1664192394455));
#59276=CARTESIAN_POINT('Ctrl Pts',(16.1143199678397,-4.57771996783974,38.1325689031823));
#59277=CARTESIAN_POINT('Ctrl Pts',(16.1876,-4.651,38.1));
#59278=CARTESIAN_POINT('',(16.4376,-4.901,38.1));
#59279=CARTESIAN_POINT('',(16.2376,-4.701,38.1));
#59280=CARTESIAN_POINT('Origin',(20.,-4.901,38.1));
#59281=CARTESIAN_POINT('Origin',(23.793914987161,-0.674999999999999,39.4808721266631));
#59282=CARTESIAN_POINT('',(23.700198185356,-0.674999999999999,39.517443878638));
#59283=CARTESIAN_POINT('',(23.7456316209454,-0.674999999999999,39.3926165402678));
#59284=CARTESIAN_POINT('Origin',(20.,-0.674999999999999,38.1));
#59285=CARTESIAN_POINT('',(23.5824841474842,-0.674999999999999,39.4039175944148));
#59286=CARTESIAN_POINT('',(23.9369417981727,-0.674999999999999,39.7457651830685));
#59287=CARTESIAN_POINT('',(23.5824841474842,-0.674999999999999,39.4039175944148));
#59288=CARTESIAN_POINT('Origin',(24.073749855503,-4.901,39.3698881347541));
#59289=CARTESIAN_POINT('',(23.7456316209454,-0.0750000000000001,39.3926165402678));
#59290=CARTESIAN_POINT('',(23.5824841474842,-4.901,39.4039175944148));
#59291=CARTESIAN_POINT('Origin',(23.5824841474842,-4.901,39.4039175944148));
#59292=CARTESIAN_POINT('',(23.700198185356,-0.0750000000000001,39.517443878638));
#59293=CARTESIAN_POINT('Origin',(20.,-0.075,38.1));
#59294=CARTESIAN_POINT('',(16.0381567112477,-0.674999999999999,38.0335807605545));
#59295=CARTESIAN_POINT('',(16.0376,-0.674999999999999,38.1));
#59296=CARTESIAN_POINT('Origin',(20.,-0.674999999999999,38.1));
#59297=CARTESIAN_POINT('',(16.0376,-0.075,38.1));
#59298=CARTESIAN_POINT('',(16.0381567112477,-0.674999999999999,38.1664192394455));
#59299=CARTESIAN_POINT('Origin',(20.,-0.674999999999999,38.1));
#59300=CARTESIAN_POINT('',(16.0381567112477,-0.0750000000000001,38.1664192394455));
#59301=CARTESIAN_POINT('',(16.0868124331256,-0.674999999999999,38.7225566853387));
#59302=CARTESIAN_POINT('',(16.0868124331256,-0.0750000000000001,38.7225566853387));
#59303=CARTESIAN_POINT('',(16.1098795929091,-0.674999999999999,38.8533770492488));
#59304=CARTESIAN_POINT('Origin',(20.,-0.674999999999999,38.1));
#59305=CARTESIAN_POINT('',(16.1098795929091,-0.0750000000000001,38.8533770492488));
#59306=CARTESIAN_POINT('',(16.2543683790546,-0.674999999999999,39.3926165402678));
#59307=CARTESIAN_POINT('',(16.2543683790546,-0.0750000000000001,39.3926165402678));
#59308=CARTESIAN_POINT('',(16.299801814644,-0.674999999999999,39.517443878638));
#59309=CARTESIAN_POINT('Origin',(20.,-0.674999999999999,38.1));
#59310=CARTESIAN_POINT('',(16.299801814644,-0.0750000000000001,39.517443878638));
#59311=CARTESIAN_POINT('',(16.5357334464049,-0.674999999999999,40.0234008957163));
#59312=CARTESIAN_POINT('',(16.5357334464049,-0.0750000000000001,40.0234008957163));
#59313=CARTESIAN_POINT('',(16.6021526858504,-0.674999999999999,40.1384423930359));
#59314=CARTESIAN_POINT('Origin',(20.,-0.674999999999999,38.1));
#59315=CARTESIAN_POINT('',(16.6021526858504,-0.0750000000000001,40.1384423930359));
#59316=CARTESIAN_POINT('',(16.9223584999828,-0.674999999999999,40.5957436882364));
#59317=CARTESIAN_POINT('',(16.9223584999828,-0.0750000000000001,40.5957436882364));
#59318=CARTESIAN_POINT('',(17.0077454283034,-0.674999999999999,40.6975038668231));
#59319=CARTESIAN_POINT('Origin',(20.,-0.674999999999999,38.1));
#59320=CARTESIAN_POINT('',(17.0077454283034,-0.0750000000000001,40.6975038668231));
#59321=CARTESIAN_POINT('',(17.4024961331769,-0.674999999999999,41.0922545716966));
#59322=CARTESIAN_POINT('',(17.4024961331769,-0.0750000000000001,41.0922545716966));
#59323=CARTESIAN_POINT('',(17.5042563117636,-0.674999999999999,41.1776415000172));
#59324=CARTESIAN_POINT('Origin',(20.,-0.674999999999999,38.1));
#59325=CARTESIAN_POINT('',(17.5042563117637,-0.0750000000000001,41.1776415000173));
#59326=CARTESIAN_POINT('',(17.9615576069641,-0.674999999999999,41.4978473141496));
#59327=CARTESIAN_POINT('',(17.961557606964,-0.0750000000000001,41.4978473141496));
#59328=CARTESIAN_POINT('',(18.0765991042837,-0.674999999999999,41.5642665535951));
#59329=CARTESIAN_POINT('Origin',(20.,-0.674999999999999,38.1));
#59330=CARTESIAN_POINT('',(18.0765991042837,-0.0750000000000001,41.5642665535951));
#59331=CARTESIAN_POINT('',(18.582556121362,-0.674999999999999,41.800198185356));
#59332=CARTESIAN_POINT('',(18.582556121362,-0.0750000000000001,41.800198185356));
#59333=CARTESIAN_POINT('',(18.7073834597322,-0.674999999999999,41.8456316209454));
#59334=CARTESIAN_POINT('Origin',(20.,-0.674999999999999,38.1));
#59335=CARTESIAN_POINT('',(18.7073834597322,-0.0750000000000001,41.8456316209454));
#59336=CARTESIAN_POINT('',(19.2466229507512,-0.674999999999999,41.9901204070909));
#59337=CARTESIAN_POINT('',(19.2466229507511,-0.0750000000000001,41.9901204070909));
#59338=CARTESIAN_POINT('',(19.3774433146613,-0.674999999999999,42.0131875668744));
#59339=CARTESIAN_POINT('Origin',(20.,-0.674999999999999,38.1));
#59340=CARTESIAN_POINT('',(19.3774433146613,-0.0750000000000001,42.0131875668744));
#59341=CARTESIAN_POINT('',(19.9335807605545,-0.674999999999999,42.0618432887523));
#59342=CARTESIAN_POINT('',(19.9335807605545,-0.0750000000000001,42.0618432887523));
#59343=CARTESIAN_POINT('',(20.0664192394455,-0.674999999999999,42.0618432887523));
#59344=CARTESIAN_POINT('Origin',(20.,-0.674999999999999,38.1));
#59345=CARTESIAN_POINT('',(20.0664192394455,-0.0750000000000001,42.0618432887523));
#59346=CARTESIAN_POINT('',(20.6225566853387,-0.674999999999999,42.0131875668744));
#59347=CARTESIAN_POINT('',(20.6225566853387,-0.0750000000000001,42.0131875668744));
#59348=CARTESIAN_POINT('',(20.7533770492489,-0.674999999999999,41.9901204070909));
#59349=CARTESIAN_POINT('Origin',(20.,-0.674999999999999,38.1));
#59350=CARTESIAN_POINT('',(20.7533770492488,-0.0750000000000001,41.9901204070909));
#59351=CARTESIAN_POINT('',(21.2926165402678,-0.674999999999999,41.8456316209454));
#59352=CARTESIAN_POINT('',(21.2926165402678,-0.0750000000000001,41.8456316209454));
#59353=CARTESIAN_POINT('',(21.417443878638,-0.674999999999999,41.800198185356));
#59354=CARTESIAN_POINT('Origin',(20.,-0.674999999999999,38.1));
#59355=CARTESIAN_POINT('',(21.417443878638,-0.0750000000000001,41.800198185356));
#59356=CARTESIAN_POINT('',(21.9234008957163,-0.674999999999999,41.5642665535951));
#59357=CARTESIAN_POINT('',(21.9234008957163,-0.0750000000000001,41.5642665535951));
#59358=CARTESIAN_POINT('',(22.038442393036,-0.674999999999999,41.4978473141496));
#59359=CARTESIAN_POINT('Origin',(20.,-0.674999999999999,38.1));
#59360=CARTESIAN_POINT('',(22.038442393036,-0.0750000000000001,41.4978473141496));
#59361=CARTESIAN_POINT('',(22.4957436882364,-0.674999999999999,41.1776415000172));
#59362=CARTESIAN_POINT('',(22.4957436882364,-0.0750000000000001,41.1776415000172));
#59363=CARTESIAN_POINT('',(22.5975038668231,-0.674999999999999,41.0922545716966));
#59364=CARTESIAN_POINT('Origin',(20.,-0.674999999999999,38.1));
#59365=CARTESIAN_POINT('',(22.5975038668231,-0.0750000000000001,41.0922545716966));
#59366=CARTESIAN_POINT('',(22.9922545716966,-0.674999999999999,40.6975038668231));
#59367=CARTESIAN_POINT('',(22.9922545716966,-0.0750000000000001,40.6975038668231));
#59368=CARTESIAN_POINT('',(23.0776415000173,-0.674999999999999,40.5957436882363));
#59369=CARTESIAN_POINT('Origin',(20.,-0.674999999999999,38.1));
#59370=CARTESIAN_POINT('',(23.0776415000172,-0.0750000000000001,40.5957436882364));
#59371=CARTESIAN_POINT('',(23.3978473141496,-0.674999999999999,40.1384423930359));
#59372=CARTESIAN_POINT('',(23.3978473141496,-0.0750000000000001,40.1384423930359));
#59373=CARTESIAN_POINT('',(23.4642665535951,-0.674999999999999,40.0234008957163));
#59374=CARTESIAN_POINT('Origin',(20.,-0.674999999999999,38.1));
#59375=CARTESIAN_POINT('',(23.4642665535951,-0.0750000000000001,40.0234008957163));
#59376=CARTESIAN_POINT('',(23.9618432887523,-0.674999999999999,38.1664192394455));
#59377=CARTESIAN_POINT('',(23.9618432887523,-0.0750000000000001,38.1664192394455));
#59378=CARTESIAN_POINT('',(23.9618432887523,-0.674999999999999,38.0335807605545));
#59379=CARTESIAN_POINT('Origin',(20.,-0.674999999999999,38.1));
#59380=CARTESIAN_POINT('',(23.9618432887523,-0.0750000000000001,38.0335807605545));
#59381=CARTESIAN_POINT('',(23.9131875668744,-0.674999999999999,37.4774433146613));
#59382=CARTESIAN_POINT('',(23.9131875668744,-0.0750000000000001,37.4774433146613));
#59383=CARTESIAN_POINT('',(23.8901204070909,-0.674999999999999,37.3466229507511));
#59384=CARTESIAN_POINT('Origin',(20.,-0.674999999999999,38.1));
#59385=CARTESIAN_POINT('',(23.8901204070909,-0.0750000000000001,37.3466229507511));
#59386=CARTESIAN_POINT('',(23.7456316209454,-0.674999999999999,36.8073834597322));
#59387=CARTESIAN_POINT('',(23.7456316209454,-0.0750000000000001,36.8073834597322));
#59388=CARTESIAN_POINT('',(23.700198185356,-0.674999999999999,36.682556121362));
#59389=CARTESIAN_POINT('Origin',(20.,-0.674999999999999,38.1));
#59390=CARTESIAN_POINT('',(23.700198185356,-0.0750000000000001,36.682556121362));
#59391=CARTESIAN_POINT('',(23.4642665535951,-0.674999999999999,36.1765991042837));
#59392=CARTESIAN_POINT('',(23.4642665535951,-0.0750000000000001,36.1765991042837));
#59393=CARTESIAN_POINT('',(23.3978473141496,-0.674999999999999,36.061557606964));
#59394=CARTESIAN_POINT('Origin',(20.,-0.674999999999999,38.1));
#59395=CARTESIAN_POINT('',(23.3978473141496,-0.0750000000000001,36.061557606964));
#59396=CARTESIAN_POINT('',(23.0776415000172,-0.674999999999999,35.6042563117636));
#59397=CARTESIAN_POINT('',(23.0776415000172,-0.0750000000000001,35.6042563117636));
#59398=CARTESIAN_POINT('',(22.9922545716966,-0.674999999999999,35.5024961331769));
#59399=CARTESIAN_POINT('Origin',(20.,-0.674999999999999,38.1));
#59400=CARTESIAN_POINT('',(22.9922545716966,-0.0750000000000001,35.5024961331769));
#59401=CARTESIAN_POINT('',(22.5975038668231,-0.674999999999999,35.1077454283034));
#59402=CARTESIAN_POINT('',(22.5975038668231,-0.0750000000000001,35.1077454283034));
#59403=CARTESIAN_POINT('',(22.4957436882364,-0.674999999999999,35.0223584999828));
#59404=CARTESIAN_POINT('Origin',(20.,-0.674999999999999,38.1));
#59405=CARTESIAN_POINT('',(22.4957436882363,-0.0750000000000001,35.0223584999827));
#59406=CARTESIAN_POINT('',(22.038442393036,-0.674999999999999,34.7021526858504));
#59407=CARTESIAN_POINT('',(22.038442393036,-0.0750000000000001,34.7021526858504));
#59408=CARTESIAN_POINT('',(21.9234008957163,-0.674999999999999,34.6357334464049));
#59409=CARTESIAN_POINT('Origin',(20.,-0.674999999999999,38.1));
#59410=CARTESIAN_POINT('',(21.9234008957163,-0.0750000000000001,34.6357334464049));
#59411=CARTESIAN_POINT('',(21.417443878638,-0.674999999999999,34.399801814644));
#59412=CARTESIAN_POINT('',(21.417443878638,-0.0750000000000001,34.399801814644));
#59413=CARTESIAN_POINT('',(21.2926165402678,-0.674999999999999,34.3543683790546));
#59414=CARTESIAN_POINT('Origin',(20.,-0.674999999999999,38.1));
#59415=CARTESIAN_POINT('',(21.2926165402678,-0.0750000000000001,34.3543683790546));
#59416=CARTESIAN_POINT('',(20.7533770492489,-0.674999999999999,34.2098795929091));
#59417=CARTESIAN_POINT('',(20.7533770492488,-0.0750000000000001,34.2098795929091));
#59418=CARTESIAN_POINT('',(20.6225566853387,-0.674999999999999,34.1868124331256));
#59419=CARTESIAN_POINT('Origin',(20.,-0.674999999999999,38.1));
#59420=CARTESIAN_POINT('',(20.6225566853387,-0.0750000000000001,34.1868124331256));
#59421=CARTESIAN_POINT('',(20.0664192394455,-0.674999999999999,34.1381567112477));
#59422=CARTESIAN_POINT('',(20.0664192394455,-0.0750000000000001,34.1381567112477));
#59423=CARTESIAN_POINT('',(19.9335807605545,-0.674999999999999,34.1381567112477));
#59424=CARTESIAN_POINT('Origin',(20.,-0.674999999999999,38.1));
#59425=CARTESIAN_POINT('',(19.9335807605545,-0.0750000000000001,34.1381567112477));
#59426=CARTESIAN_POINT('',(19.3774433146613,-0.674999999999999,34.1868124331256));
#59427=CARTESIAN_POINT('',(19.3774433146613,-0.0750000000000001,34.1868124331256));
#59428=CARTESIAN_POINT('',(19.2466229507511,-0.674999999999999,34.2098795929091));
#59429=CARTESIAN_POINT('Origin',(20.,-0.674999999999999,38.1));
#59430=CARTESIAN_POINT('',(19.2466229507512,-0.0750000000000001,34.2098795929091));
#59431=CARTESIAN_POINT('',(18.7073834597322,-0.674999999999999,34.3543683790546));
#59432=CARTESIAN_POINT('',(18.7073834597322,-0.0750000000000001,34.3543683790546));
#59433=CARTESIAN_POINT('',(18.582556121362,-0.674999999999999,34.399801814644));
#59434=CARTESIAN_POINT('Origin',(20.,-0.674999999999999,38.1));
#59435=CARTESIAN_POINT('',(18.582556121362,-0.0750000000000001,34.399801814644));
#59436=CARTESIAN_POINT('',(18.0765991042837,-0.674999999999999,34.6357334464049));
#59437=CARTESIAN_POINT('',(18.0765991042837,-0.0750000000000001,34.6357334464049));
#59438=CARTESIAN_POINT('',(17.961557606964,-0.674999999999999,34.7021526858504));
#59439=CARTESIAN_POINT('Origin',(20.,-0.674999999999999,38.1));
#59440=CARTESIAN_POINT('',(17.961557606964,-0.0750000000000001,34.7021526858504));
#59441=CARTESIAN_POINT('',(17.5042563117636,-0.674999999999999,35.0223584999828));
#59442=CARTESIAN_POINT('',(17.5042563117636,-0.0750000000000001,35.0223584999828));
#59443=CARTESIAN_POINT('',(17.4024961331769,-0.674999999999999,35.1077454283034));
#59444=CARTESIAN_POINT('Origin',(20.,-0.674999999999999,38.1));
#59445=CARTESIAN_POINT('',(17.4024961331769,-0.0750000000000001,35.1077454283034));
#59446=CARTESIAN_POINT('',(17.0077454283034,-0.674999999999999,35.5024961331769));
#59447=CARTESIAN_POINT('',(17.0077454283034,-0.0750000000000001,35.5024961331769));
#59448=CARTESIAN_POINT('',(16.9223584999828,-0.674999999999999,35.6042563117636));
#59449=CARTESIAN_POINT('Origin',(20.,-0.674999999999999,38.1));
#59450=CARTESIAN_POINT('',(16.9223584999828,-0.0750000000000001,35.6042563117636));
#59451=CARTESIAN_POINT('',(16.6021526858504,-0.674999999999999,36.0615576069641));
#59452=CARTESIAN_POINT('',(16.6021526858504,-0.0750000000000001,36.0615576069641));
#59453=CARTESIAN_POINT('',(16.5357334464049,-0.674999999999999,36.1765991042837));
#59454=CARTESIAN_POINT('Origin',(20.,-0.674999999999999,38.1));
#59455=CARTESIAN_POINT('',(16.5357334464049,-0.0750000000000001,36.1765991042837));
#59456=CARTESIAN_POINT('',(16.299801814644,-0.674999999999999,36.682556121362));
#59457=CARTESIAN_POINT('',(16.299801814644,-0.0750000000000001,36.682556121362));
#59458=CARTESIAN_POINT('',(16.2543683790546,-0.674999999999999,36.8073834597322));
#59459=CARTESIAN_POINT('Origin',(20.,-0.674999999999999,38.1));
#59460=CARTESIAN_POINT('',(16.2543683790546,-0.0750000000000001,36.8073834597322));
#59461=CARTESIAN_POINT('',(16.1098795929091,-0.674999999999999,37.3466229507511));
#59462=CARTESIAN_POINT('',(16.1098795929091,-0.0750000000000001,37.3466229507511));
#59463=CARTESIAN_POINT('',(16.0868124331256,-0.674999999999999,37.4774433146613));
#59464=CARTESIAN_POINT('Origin',(20.,-0.674999999999999,38.1));
#59465=CARTESIAN_POINT('',(16.0868124331256,-0.0750000000000001,37.4774433146613));
#59466=CARTESIAN_POINT('',(16.0381567112477,-0.0750000000000001,38.0335807605545));
#59467=CARTESIAN_POINT('Origin',(23.7913466810908,-4.901,40.0579949192431));
#59468=CARTESIAN_POINT('',(23.3016352493878,-0.674999999999999,40.0062));
#59469=CARTESIAN_POINT('',(23.3016352493878,-0.674999999999999,40.0062));
#59470=CARTESIAN_POINT('',(23.3016352493878,-4.901,40.0062));
#59471=CARTESIAN_POINT('Origin',(23.3016352493878,-4.901,40.0062));
#59472=CARTESIAN_POINT('',(23.5913466810908,-0.674999999999999,40.4044050807569));
#59473=CARTESIAN_POINT('Origin',(23.4964909652393,-0.674999999999999,40.1187));
#59474=CARTESIAN_POINT('Origin',(23.0928278346486,-0.674999999999999,40.6951906953484));
#59475=CARTESIAN_POINT('',(22.9204678349468,-0.674999999999999,40.550563483169));
#59476=CARTESIAN_POINT('',(23.136630312413,-0.674999999999999,40.9930267961517));
#59477=CARTESIAN_POINT('',(22.9204678349468,-0.674999999999999,40.550563483169));
#59478=CARTESIAN_POINT('Origin',(23.3937453562876,-4.901,40.6866090189041));
#59479=CARTESIAN_POINT('',(22.9204678349468,-4.901,40.550563483169));
#59480=CARTESIAN_POINT('Origin',(22.9204678349468,-4.901,40.550563483169));
#59481=CARTESIAN_POINT('Origin',(22.8930267961517,-4.901,41.236630312413));
#59482=CARTESIAN_POINT('',(22.450563483169,-0.674999999999999,41.0204678349468));
#59483=CARTESIAN_POINT('',(22.450563483169,-0.674999999999999,41.0204678349468));
#59484=CARTESIAN_POINT('',(22.450563483169,-4.901,41.0204678349468));
#59485=CARTESIAN_POINT('Origin',(22.450563483169,-4.901,41.0204678349468));
#59486=CARTESIAN_POINT('',(22.5866090189041,-0.674999999999999,41.4937453562876));
#59487=CARTESIAN_POINT('Origin',(22.5951906953484,-0.674999999999999,41.1928278346486));
#59488=CARTESIAN_POINT('Origin',(22.0187,-0.674999999999999,41.5964909652393));
#59489=CARTESIAN_POINT('',(21.9062,-0.674999999999999,41.4016352493878));
#59490=CARTESIAN_POINT('',(21.9579949192431,-0.674999999999999,41.8913466810908));
#59491=CARTESIAN_POINT('',(21.9062,-0.674999999999999,41.4016352493878));
#59492=CARTESIAN_POINT('Origin',(22.3044050807569,-4.901,41.6913466810908));
#59493=CARTESIAN_POINT('',(21.9062,-4.901,41.4016352493878));
#59494=CARTESIAN_POINT('Origin',(21.9062,-4.901,41.4016352493878));
#59495=CARTESIAN_POINT('Origin',(21.6457651830685,-4.901,42.0369417981727));
#59496=CARTESIAN_POINT('',(21.3039175944148,-0.674999999999999,41.6824841474842));
#59497=CARTESIAN_POINT('',(21.3039175944148,-0.674999999999999,41.6824841474842));
#59498=CARTESIAN_POINT('',(21.3039175944148,-4.901,41.6824841474842));
#59499=CARTESIAN_POINT('Origin',(21.3039175944148,-4.901,41.6824841474842));
#59500=CARTESIAN_POINT('',(21.2698881347541,-0.674999999999999,42.173749855503));
#59501=CARTESIAN_POINT('Origin',(21.3808721266631,-0.674999999999999,41.893914987161));
#59502=CARTESIAN_POINT('Origin',(20.7010871525125,-0.674999999999999,42.0760628220115));
#59503=CARTESIAN_POINT('',(20.6620163125374,-0.674999999999999,41.8544810775837));
#59504=CARTESIAN_POINT('',(20.5431964418851,-0.674999999999999,42.3323742019726));
#59505=CARTESIAN_POINT('',(20.6620163125374,-0.674999999999999,41.8544810775837));
#59506=CARTESIAN_POINT('Origin',(20.93711954309,-4.901,42.2629149309058));
#59507=CARTESIAN_POINT('',(20.6620163125374,-4.901,41.8544810775837));
#59508=CARTESIAN_POINT('Origin',(20.6620163125374,-4.901,41.8544810775837));
#59509=CARTESIAN_POINT('Origin',(20.2,-4.901,42.3624));
#59510=CARTESIAN_POINT('',(20.,-0.674999999999999,41.9124));
#59511=CARTESIAN_POINT('',(20.,-0.674999999999999,41.9124));
#59512=CARTESIAN_POINT('',(20.,-4.901,41.9124));
#59513=CARTESIAN_POINT('Origin',(20.,-4.901,41.9124));
#59514=CARTESIAN_POINT('',(19.8,-0.674999999999999,42.3624));
#59515=CARTESIAN_POINT('Origin',(20.,-0.674999999999999,42.1374));
#59516=CARTESIAN_POINT('Origin',(19.2989128474875,-0.674999999999999,42.0760628220115));
#59517=CARTESIAN_POINT('',(19.3379836874626,-0.674999999999999,41.8544810775837));
#59518=CARTESIAN_POINT('',(19.06288045691,-0.674999999999999,42.2629149309059));
#59519=CARTESIAN_POINT('',(19.3379836874626,-0.674999999999999,41.8544810775837));
#59520=CARTESIAN_POINT('Origin',(19.4568035581149,-4.901,42.3323742019726));
#59521=CARTESIAN_POINT('',(19.3379836874626,-4.901,41.8544810775837));
#59522=CARTESIAN_POINT('Origin',(19.3379836874626,-4.901,41.8544810775837));
#59523=CARTESIAN_POINT('Origin',(18.7301118652459,-4.901,42.173749855503));
#59524=CARTESIAN_POINT('',(18.6960824055852,-0.674999999999999,41.6824841474842));
#59525=CARTESIAN_POINT('',(18.6960824055852,-0.674999999999999,41.6824841474842));
#59526=CARTESIAN_POINT('',(18.6960824055852,-4.901,41.6824841474842));
#59527=CARTESIAN_POINT('Origin',(18.6960824055852,-4.901,41.6824841474842));
#59528=CARTESIAN_POINT('',(18.3542348169315,-0.674999999999999,42.0369417981727));
#59529=CARTESIAN_POINT('Origin',(18.6191278733369,-0.674999999999999,41.893914987161));
#59530=CARTESIAN_POINT('Origin',(17.9813,-0.674999999999999,41.5964909652393));
#59531=CARTESIAN_POINT('',(18.0938,-0.674999999999999,41.4016352493878));
#59532=CARTESIAN_POINT('',(17.6955949192431,-0.674999999999999,41.6913466810908));
#59533=CARTESIAN_POINT('',(18.0938,-0.674999999999999,41.4016352493878));
#59534=CARTESIAN_POINT('Origin',(18.0420050807569,-4.901,41.8913466810908));
#59535=CARTESIAN_POINT('',(18.0938,-4.901,41.4016352493878));
#59536=CARTESIAN_POINT('Origin',(18.0938,-4.901,41.4016352493878));
#59537=CARTESIAN_POINT('Origin',(17.4133909810959,-4.901,41.4937453562876));
#59538=CARTESIAN_POINT('',(17.549436516831,-0.674999999999999,41.0204678349468));
#59539=CARTESIAN_POINT('',(17.549436516831,-0.674999999999999,41.0204678349468));
#59540=CARTESIAN_POINT('',(17.549436516831,-4.901,41.0204678349468));
#59541=CARTESIAN_POINT('Origin',(17.549436516831,-4.901,41.0204678349468));
#59542=CARTESIAN_POINT('',(17.1069732038483,-0.674999999999999,41.236630312413));
#59543=CARTESIAN_POINT('Origin',(17.4048093046516,-0.674999999999999,41.1928278346486));
#59544=CARTESIAN_POINT('Origin',(16.9071721653514,-0.674999999999999,40.6951906953484));
#59545=CARTESIAN_POINT('',(17.0795321650532,-0.674999999999999,40.550563483169));
#59546=CARTESIAN_POINT('',(16.6062546437124,-0.674999999999999,40.6866090189041));
#59547=CARTESIAN_POINT('',(17.0795321650532,-0.674999999999999,40.550563483169));
#59548=CARTESIAN_POINT('Origin',(16.863369687587,-4.901,40.9930267961517));
#59549=CARTESIAN_POINT('',(17.0795321650532,-4.901,40.550563483169));
#59550=CARTESIAN_POINT('Origin',(17.0795321650532,-4.901,40.550563483169));
#59551=CARTESIAN_POINT('Origin',(16.4086533189092,-4.901,40.4044050807569));
#59552=CARTESIAN_POINT('',(16.6983647506122,-0.674999999999999,40.0062));
#59553=CARTESIAN_POINT('',(16.6983647506122,-0.674999999999999,40.0062));
#59554=CARTESIAN_POINT('',(16.6983647506122,-4.901,40.0062));
#59555=CARTESIAN_POINT('Origin',(16.6983647506122,-4.901,40.0062));
#59556=CARTESIAN_POINT('',(16.2086533189092,-0.674999999999999,40.0579949192431));
#59557=CARTESIAN_POINT('Origin',(16.5035090347607,-0.674999999999999,40.1187));
#59558=CARTESIAN_POINT('Origin',(16.206085012839,-0.674999999999999,39.480872126663));
#59559=CARTESIAN_POINT('',(16.4175158525158,-0.674999999999999,39.4039175944148));
#59560=CARTESIAN_POINT('',(15.926250144497,-0.674999999999999,39.3698881347541));
#59561=CARTESIAN_POINT('',(16.4175158525158,-0.674999999999999,39.4039175944148));
#59562=CARTESIAN_POINT('Origin',(16.0630582018273,-4.901,39.7457651830685));
#59563=CARTESIAN_POINT('',(16.4175158525158,-4.901,39.4039175944148));
#59564=CARTESIAN_POINT('Origin',(16.4175158525158,-4.901,39.4039175944148));
#59565=CARTESIAN_POINT('Origin',(15.8370850690942,-4.901,39.03711954309));
#59566=CARTESIAN_POINT('',(16.2455189224163,-0.674999999999999,38.7620163125374));
#59567=CARTESIAN_POINT('',(16.2455189224163,-0.674999999999999,38.7620163125374));
#59568=CARTESIAN_POINT('',(16.2455189224163,-4.901,38.7620163125374));
#59569=CARTESIAN_POINT('Origin',(16.2455189224163,-4.901,38.7620163125374));
#59570=CARTESIAN_POINT('',(15.7676257980274,-0.674999999999999,38.6431964418851));
#59571=CARTESIAN_POINT('Origin',(16.0239371779885,-0.674999999999999,38.8010871525125));
#59572=CARTESIAN_POINT('Origin',(15.9626,-0.674999999999999,38.1));
#59573=CARTESIAN_POINT('',(16.1876,-0.674999999999999,38.1));
#59574=CARTESIAN_POINT('',(15.7376,-0.674999999999999,37.9));
#59575=CARTESIAN_POINT('',(16.1876,-0.674999999999999,38.1));
#59576=CARTESIAN_POINT('Origin',(15.7376,-4.901,38.3));
#59577=CARTESIAN_POINT('',(16.1876,-4.901,38.1));
#59578=CARTESIAN_POINT('Origin',(16.1876,-4.901,38.1));
#59579=CARTESIAN_POINT('Origin',(15.7676257980274,-4.901,37.5568035581149));
#59580=CARTESIAN_POINT('',(16.2455189224163,-0.674999999999999,37.4379836874626));
#59581=CARTESIAN_POINT('',(16.2455189224163,-0.674999999999999,37.4379836874626));
#59582=CARTESIAN_POINT('',(16.2455189224163,-4.901,37.4379836874626));
#59583=CARTESIAN_POINT('Origin',(16.2455189224163,-4.901,37.4379836874626));
#59584=CARTESIAN_POINT('',(15.8370850690942,-0.674999999999999,37.16288045691));
#59585=CARTESIAN_POINT('Origin',(16.0239371779885,-0.674999999999999,37.3989128474875));
#59586=CARTESIAN_POINT('Origin',(16.206085012839,-0.674999999999999,36.7191278733369));
#59587=CARTESIAN_POINT('',(16.4175158525158,-0.674999999999999,36.7960824055852));
#59588=CARTESIAN_POINT('',(16.0630582018273,-0.674999999999999,36.4542348169315));
#59589=CARTESIAN_POINT('',(16.4175158525158,-0.674999999999999,36.7960824055852));
#59590=CARTESIAN_POINT('Origin',(15.926250144497,-4.901,36.8301118652458));
#59591=CARTESIAN_POINT('',(16.4175158525158,-4.901,36.7960824055852));
#59592=CARTESIAN_POINT('Origin',(16.4175158525158,-4.901,36.7960824055852));
#59593=CARTESIAN_POINT('Origin',(16.2086533189092,-4.901,36.1420050807569));
#59594=CARTESIAN_POINT('',(16.6983647506122,-0.674999999999999,36.1938));
#59595=CARTESIAN_POINT('',(16.6983647506122,-0.674999999999999,36.1938));
#59596=CARTESIAN_POINT('',(16.6983647506122,-4.901,36.1938));
#59597=CARTESIAN_POINT('Origin',(16.6983647506122,-4.901,36.1938));
#59598=CARTESIAN_POINT('',(16.4086533189092,-0.674999999999999,35.7955949192431));
#59599=CARTESIAN_POINT('Origin',(16.5035090347607,-0.674999999999999,36.0813));
#59600=CARTESIAN_POINT('Origin',(16.9071721653514,-0.674999999999999,35.5048093046516));
#59601=CARTESIAN_POINT('',(17.0795321650532,-0.674999999999999,35.649436516831));
#59602=CARTESIAN_POINT('',(16.863369687587,-0.674999999999999,35.2069732038483));
#59603=CARTESIAN_POINT('',(17.0795321650532,-0.674999999999999,35.649436516831));
#59604=CARTESIAN_POINT('Origin',(16.6062546437124,-4.901,35.5133909810959));
#59605=CARTESIAN_POINT('',(17.0795321650532,-4.901,35.649436516831));
#59606=CARTESIAN_POINT('Origin',(17.0795321650532,-4.901,35.649436516831));
#59607=CARTESIAN_POINT('Origin',(17.1069732038483,-4.901,34.963369687587));
#59608=CARTESIAN_POINT('',(17.549436516831,-0.674999999999999,35.1795321650532));
#59609=CARTESIAN_POINT('',(17.549436516831,-0.674999999999999,35.1795321650532));
#59610=CARTESIAN_POINT('',(17.549436516831,-4.901,35.1795321650532));
#59611=CARTESIAN_POINT('Origin',(17.549436516831,-4.901,35.1795321650532));
#59612=CARTESIAN_POINT('',(17.4133909810959,-0.674999999999999,34.7062546437124));
#59613=CARTESIAN_POINT('Origin',(17.4048093046516,-0.674999999999999,35.0071721653514));
#59614=CARTESIAN_POINT('Origin',(17.9813,-0.674999999999999,34.6035090347607));
#59615=CARTESIAN_POINT('',(18.0938,-0.674999999999999,34.7983647506122));
#59616=CARTESIAN_POINT('',(18.0420050807569,-0.674999999999999,34.3086533189092));
#59617=CARTESIAN_POINT('',(18.0938,-0.674999999999999,34.7983647506122));
#59618=CARTESIAN_POINT('Origin',(17.6955949192431,-4.901,34.5086533189092));
#59619=CARTESIAN_POINT('',(18.0938,-4.901,34.7983647506122));
#59620=CARTESIAN_POINT('Origin',(18.0938,-4.901,34.7983647506122));
#59621=CARTESIAN_POINT('Origin',(18.3542348169315,-4.901,34.1630582018273));
#59622=CARTESIAN_POINT('',(18.6960824055852,-0.674999999999999,34.5175158525158));
#59623=CARTESIAN_POINT('',(18.6960824055852,-0.674999999999999,34.5175158525158));
#59624=CARTESIAN_POINT('',(18.6960824055852,-4.901,34.5175158525158));
#59625=CARTESIAN_POINT('Origin',(18.6960824055852,-4.901,34.5175158525158));
#59626=CARTESIAN_POINT('',(18.7301118652459,-0.674999999999999,34.026250144497));
#59627=CARTESIAN_POINT('Origin',(18.6191278733369,-0.674999999999999,34.306085012839));
#59628=CARTESIAN_POINT('Origin',(19.2989128474875,-0.674999999999999,34.1239371779885));
#59629=CARTESIAN_POINT('',(19.3379836874626,-0.674999999999999,34.3455189224163));
#59630=CARTESIAN_POINT('',(19.4568035581149,-0.674999999999999,33.8676257980274));
#59631=CARTESIAN_POINT('',(19.3379836874626,-0.674999999999999,34.3455189224163));
#59632=CARTESIAN_POINT('Origin',(19.06288045691,-4.901,33.9370850690941));
#59633=CARTESIAN_POINT('',(19.3379836874626,-4.901,34.3455189224163));
#59634=CARTESIAN_POINT('Origin',(19.3379836874626,-4.901,34.3455189224163));
#59635=CARTESIAN_POINT('Origin',(19.8,-4.901,33.8376));
#59636=CARTESIAN_POINT('',(20.,-0.674999999999999,34.2876));
#59637=CARTESIAN_POINT('',(20.,-0.674999999999999,34.2876));
#59638=CARTESIAN_POINT('',(20.,-4.901,34.2876));
#59639=CARTESIAN_POINT('Origin',(20.,-4.901,34.2876));
#59640=CARTESIAN_POINT('',(20.2,-0.674999999999999,33.8376));
#59641=CARTESIAN_POINT('Origin',(20.,-0.674999999999999,34.0626));
#59642=CARTESIAN_POINT('Origin',(20.7010871525125,-0.674999999999999,34.1239371779885));
#59643=CARTESIAN_POINT('',(20.6620163125374,-0.674999999999999,34.3455189224163));
#59644=CARTESIAN_POINT('',(20.93711954309,-0.674999999999999,33.9370850690941));
#59645=CARTESIAN_POINT('',(20.6620163125374,-0.674999999999999,34.3455189224163));
#59646=CARTESIAN_POINT('Origin',(20.5431964418851,-4.901,33.8676257980274));
#59647=CARTESIAN_POINT('',(20.6620163125374,-4.901,34.3455189224163));
#59648=CARTESIAN_POINT('Origin',(20.6620163125374,-4.901,34.3455189224163));
#59649=CARTESIAN_POINT('Origin',(21.2698881347541,-4.901,34.026250144497));
#59650=CARTESIAN_POINT('',(21.3039175944148,-0.674999999999999,34.5175158525158));
#59651=CARTESIAN_POINT('',(21.3039175944148,-0.674999999999999,34.5175158525158));
#59652=CARTESIAN_POINT('',(21.3039175944148,-4.901,34.5175158525158));
#59653=CARTESIAN_POINT('Origin',(21.3039175944148,-4.901,34.5175158525158));
#59654=CARTESIAN_POINT('',(21.6457651830685,-0.674999999999999,34.1630582018273));
#59655=CARTESIAN_POINT('Origin',(21.3808721266631,-0.674999999999999,34.306085012839));
#59656=CARTESIAN_POINT('Origin',(22.0187,-0.674999999999999,34.6035090347607));
#59657=CARTESIAN_POINT('',(21.9062,-0.674999999999999,34.7983647506122));
#59658=CARTESIAN_POINT('',(22.3044050807569,-0.674999999999999,34.5086533189092));
#59659=CARTESIAN_POINT('',(21.9062,-0.674999999999999,34.7983647506122));
#59660=CARTESIAN_POINT('Origin',(21.9579949192431,-4.901,34.3086533189092));
#59661=CARTESIAN_POINT('',(21.9062,-4.901,34.7983647506122));
#59662=CARTESIAN_POINT('Origin',(21.9062,-4.901,34.7983647506122));
#59663=CARTESIAN_POINT('Origin',(22.5866090189041,-4.901,34.7062546437124));
#59664=CARTESIAN_POINT('',(22.450563483169,-0.674999999999999,35.1795321650532));
#59665=CARTESIAN_POINT('',(22.450563483169,-0.674999999999999,35.1795321650532));
#59666=CARTESIAN_POINT('',(22.450563483169,-4.901,35.1795321650532));
#59667=CARTESIAN_POINT('Origin',(22.450563483169,-4.901,35.1795321650532));
#59668=CARTESIAN_POINT('',(22.8930267961517,-0.674999999999999,34.963369687587));
#59669=CARTESIAN_POINT('Origin',(22.5951906953484,-0.674999999999999,35.0071721653514));
#59670=CARTESIAN_POINT('Origin',(23.0928278346486,-0.674999999999999,35.5048093046516));
#59671=CARTESIAN_POINT('',(22.9204678349468,-0.674999999999999,35.649436516831));
#59672=CARTESIAN_POINT('',(23.3937453562876,-0.674999999999999,35.5133909810959));
#59673=CARTESIAN_POINT('',(22.9204678349468,-0.674999999999999,35.649436516831));
#59674=CARTESIAN_POINT('Origin',(23.136630312413,-4.901,35.2069732038483));
#59675=CARTESIAN_POINT('',(22.9204678349468,-4.901,35.649436516831));
#59676=CARTESIAN_POINT('Origin',(22.9204678349468,-4.901,35.649436516831));
#59677=CARTESIAN_POINT('Origin',(23.5913466810908,-4.901,35.7955949192431));
#59678=CARTESIAN_POINT('',(23.3016352493878,-0.674999999999999,36.1938));
#59679=CARTESIAN_POINT('',(23.3016352493878,-0.674999999999999,36.1938));
#59680=CARTESIAN_POINT('',(23.3016352493878,-4.901,36.1938));
#59681=CARTESIAN_POINT('Origin',(23.3016352493878,-4.901,36.1938));
#59682=CARTESIAN_POINT('',(23.7913466810908,-0.674999999999999,36.1420050807569));
#59683=CARTESIAN_POINT('Origin',(23.4964909652393,-0.674999999999999,36.0813));
#59684=CARTESIAN_POINT('Origin',(23.793914987161,-0.674999999999999,36.7191278733369));
#59685=CARTESIAN_POINT('',(23.5824841474842,-0.674999999999999,36.7960824055852));
#59686=CARTESIAN_POINT('',(24.073749855503,-0.674999999999999,36.8301118652458));
#59687=CARTESIAN_POINT('',(23.5824841474842,-0.674999999999999,36.7960824055852));
#59688=CARTESIAN_POINT('Origin',(23.9369417981727,-4.901,36.4542348169315));
#59689=CARTESIAN_POINT('',(23.5824841474842,-4.901,36.7960824055852));
#59690=CARTESIAN_POINT('Origin',(23.5824841474842,-4.901,36.7960824055852));
#59691=CARTESIAN_POINT('Origin',(24.1629149309058,-4.901,37.16288045691));
#59692=CARTESIAN_POINT('',(23.7544810775837,-0.674999999999999,37.4379836874626));
#59693=CARTESIAN_POINT('',(23.7544810775837,-0.674999999999999,37.4379836874626));
#59694=CARTESIAN_POINT('',(23.7544810775837,-4.901,37.4379836874626));
#59695=CARTESIAN_POINT('Origin',(23.7544810775837,-4.901,37.4379836874626));
#59696=CARTESIAN_POINT('',(24.2323742019726,-0.674999999999999,37.5568035581149));
#59697=CARTESIAN_POINT('Origin',(23.9760628220115,-0.674999999999999,37.3989128474875));
#59698=CARTESIAN_POINT('Origin',(24.0374,-0.674999999999999,38.1));
#59699=CARTESIAN_POINT('',(23.8124,-0.674999999999999,38.1));
#59700=CARTESIAN_POINT('',(24.2624,-0.674999999999999,38.3));
#59701=CARTESIAN_POINT('',(23.8124,-0.674999999999999,38.1));
#59702=CARTESIAN_POINT('Origin',(24.2624,-4.901,37.9));
#59703=CARTESIAN_POINT('',(23.8124,-4.901,38.1));
#59704=CARTESIAN_POINT('Origin',(23.8124,-4.901,38.1));
#59705=CARTESIAN_POINT('Origin',(20.,-4.901,38.1));
#59706=CARTESIAN_POINT('',(22.2913588808463,-4.901,38.1));
#59707=CARTESIAN_POINT('',(21.1456794404232,-4.901,36.115625));
#59708=CARTESIAN_POINT('',(22.0049390207405,-4.901,37.60390625));
#59709=CARTESIAN_POINT('',(18.8543205595768,-4.901,36.115625));
#59710=CARTESIAN_POINT('',(20.5728397202116,-4.901,36.115625));
#59711=CARTESIAN_POINT('',(17.7086411191537,-4.901,38.1));
#59712=CARTESIAN_POINT('',(18.567900699471,-4.901,36.61171875));
#59713=CARTESIAN_POINT('',(18.8543205595768,-4.901,40.084375));
#59714=CARTESIAN_POINT('',(17.9950609792595,-4.901,38.59609375));
#59715=CARTESIAN_POINT('',(21.1456794404232,-4.901,40.084375));
#59716=CARTESIAN_POINT('',(19.4271602797884,-4.901,40.084375));
#59717=CARTESIAN_POINT('',(21.432099300529,-4.901,39.58828125));
#59718=CARTESIAN_POINT('Origin',(20.,-2.501,38.1));
#59719=CARTESIAN_POINT('',(22.2913588808463,-2.501,38.1));
#59720=CARTESIAN_POINT('',(21.1456794404232,-2.501,36.115625));
#59721=CARTESIAN_POINT('',(21.1456794404232,-2.501,36.115625));
#59722=CARTESIAN_POINT('Origin',(20.,-2.501,38.1));
#59723=CARTESIAN_POINT('Origin',(20.,-2.501,38.1));
#59724=CARTESIAN_POINT('',(18.8543205595768,-2.501,36.115625));
#59725=CARTESIAN_POINT('',(18.8543205595768,-2.501,36.115625));
#59726=CARTESIAN_POINT('Origin',(20.,-2.501,38.1));
#59727=CARTESIAN_POINT('Origin',(20.,-2.501,38.1));
#59728=CARTESIAN_POINT('',(17.7086411191537,-2.501,38.1));
#59729=CARTESIAN_POINT('',(17.7086411191537,-2.501,38.1));
#59730=CARTESIAN_POINT('Origin',(20.,-2.501,38.1));
#59731=CARTESIAN_POINT('Origin',(20.,-2.501,38.1));
#59732=CARTESIAN_POINT('',(18.8543205595768,-2.501,40.084375));
#59733=CARTESIAN_POINT('',(18.8543205595768,-2.501,40.084375));
#59734=CARTESIAN_POINT('Origin',(20.,-2.501,38.1));
#59735=CARTESIAN_POINT('Origin',(20.,-2.501,38.1));
#59736=CARTESIAN_POINT('',(21.1456794404232,-2.501,40.084375));
#59737=CARTESIAN_POINT('',(21.1456794404232,-2.501,40.084375));
#59738=CARTESIAN_POINT('Origin',(20.,-2.501,38.1));
#59739=CARTESIAN_POINT('Origin',(20.,-2.501,38.1));
#59740=CARTESIAN_POINT('',(22.2913588808463,-2.501,38.1));
#59741=CARTESIAN_POINT('Origin',(20.,-2.501,38.1));
#59742=CARTESIAN_POINT('Origin',(20.,-1.81260634222019,38.1));
#59743=CARTESIAN_POINT('',(20.,-1.12421268444038,38.1));
#59744=CARTESIAN_POINT('',(18.8543205595768,-1.81260634222019,38.1));
#59745=CARTESIAN_POINT('Origin',(22.2913588808463,-4.901,38.1));
#59746=CARTESIAN_POINT('',(22.2913588808463,-4.901,38.1));
#59747=CARTESIAN_POINT('',(21.1456794404232,-4.901,36.115625));
#59748=CARTESIAN_POINT('Origin',(21.1456794404232,-4.901,40.084375));
#59749=CARTESIAN_POINT('',(21.1456794404232,-4.901,40.084375));
#59750=CARTESIAN_POINT('Origin',(18.8543205595768,-4.901,40.084375));
#59751=CARTESIAN_POINT('',(18.8543205595768,-4.901,40.084375));
#59752=CARTESIAN_POINT('Origin',(17.7086411191537,-4.901,38.1));
#59753=CARTESIAN_POINT('',(17.7086411191537,-4.901,38.1));
#59754=CARTESIAN_POINT('Origin',(18.8543205595768,-4.901,36.115625));
#59755=CARTESIAN_POINT('',(18.8543205595768,-4.901,36.115625));
#59756=CARTESIAN_POINT('Origin',(21.1456794404232,-4.901,36.115625));
#71781=UNCERTAINTY_MEASURE_WITH_UNIT(LENGTH_MEASURE(0.01),#71796,
'DISTANCE_ACCURACY_VALUE',
'Maximum model space distance between geometric entities at asserted c
onnectivities');
#71783=UNCERTAINTY_MEASURE_WITH_UNIT(LENGTH_MEASURE(0.01),#71796,
'DISTANCE_ACCURACY_VALUE',
'Maximum model space distance between geometric entities at asserted c
onnectivities');
#71793=(
GEOMETRIC_REPRESENTATION_CONTEXT(3)
GLOBAL_UNCERTAINTY_ASSIGNED_CONTEXT((#71781))
GLOBAL_UNIT_ASSIGNED_CONTEXT((#71796,#71798,#71799))
REPRESENTATION_CONTEXT('','3D')
);
#71795=(
GEOMETRIC_REPRESENTATION_CONTEXT(3)
GLOBAL_UNCERTAINTY_ASSIGNED_CONTEXT((#71783))
GLOBAL_UNIT_ASSIGNED_CONTEXT((#71796,#71798,#71799))
REPRESENTATION_CONTEXT('','3D')
);
#71796=(
LENGTH_UNIT()
NAMED_UNIT(*)
SI_UNIT(.MILLI.,.METRE.)
);
#71798=(
NAMED_UNIT(*)
PLANE_ANGLE_UNIT()
SI_UNIT($,.RADIAN.)
);
#71799=(
NAMED_UNIT(*)
SI_UNIT($,.STERADIAN.)
SOLID_ANGLE_UNIT()
);
#71809=SHAPE_DEFINITION_REPRESENTATION(#71820,#72025);
#71820=PRODUCT_DEFINITION_SHAPE('',$,#72037);
#72025=SHAPE_REPRESENTATION('',(#14358),#71793);
#72027=PRODUCT_DEFINITION_CONTEXT('part definition',#72062,'design');
#72037=PRODUCT_DEFINITION('ASME B18.3 SHCS 10-32 UNF x 0.875',
'ASME B18.3 SHCS 10-32 UNF x 0.875',#72048,#72027);
#72048=PRODUCT_DEFINITION_FORMATION('',$,#72073);
#72062=APPLICATION_CONTEXT(
'Core Data for Automotive Mechanical Design Process');
#72063=PRODUCT_CONTEXT('part definition',#72062,'mechanical');
#72073=PRODUCT('ASME B18.3 SHCS 10-32 UNF x 0.875',
'ASME B18.3 SHCS 10-32 UNF x 0.875',$,(#72063));
#72084=PRESENTATION_STYLE_ASSIGNMENT((#72095));
#72095=SURFACE_STYLE_USAGE(.BOTH.,#72106);
#72106=SURFACE_SIDE_STYLE('',(#72117));
#72117=SURFACE_STYLE_FILL_AREA(#72128);
#72128=FILL_AREA_STYLE('Opaque(201,205,211)',(#72139));
#72139=FILL_AREA_STYLE_COLOUR('Opaque(201,205,211)',#72150);
#72150=COLOUR_RGB('Opaque(201,205,211)', 0.31764706, 0.68627451, 0.89019608);
ENDSEC;
END-ISO-10303-21;
